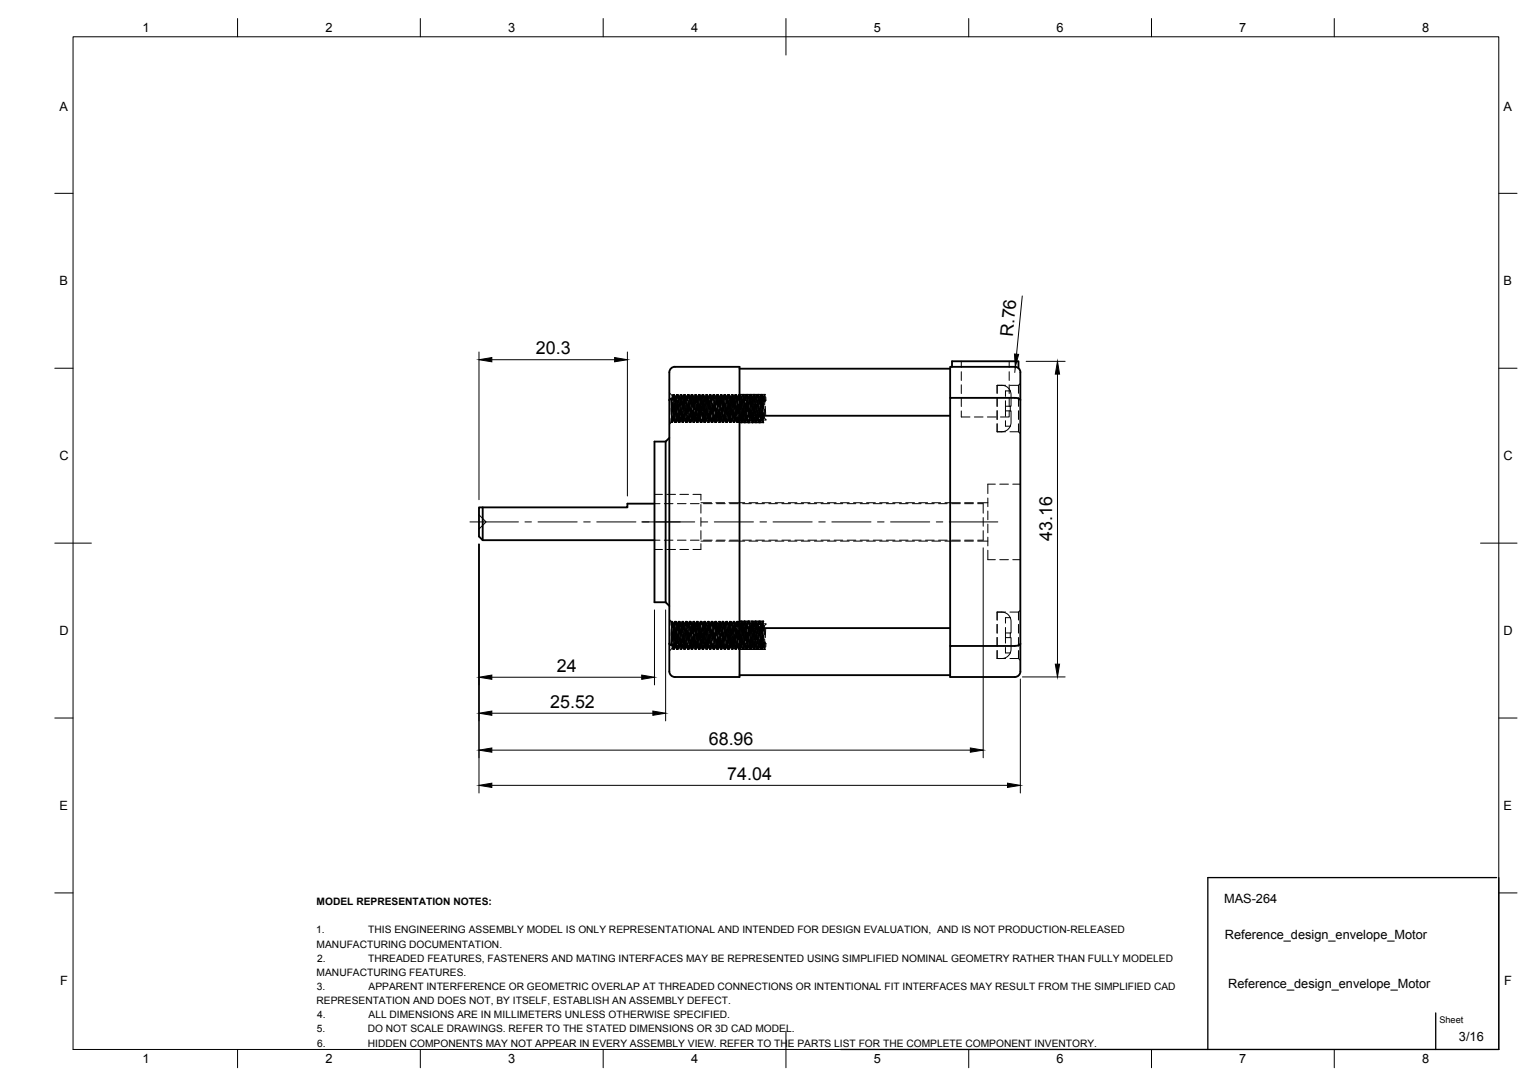
ISO-10303-21;
HEADER;
/* Generated by software containing ST-Developer
 * from STEP Tools, Inc. (www.steptools.com) 
 */

FILE_DESCRIPTION(
/* description */ (''),
/* implementation_level */ '2;1');

FILE_NAME(
/* name */ 'Reference_design_envelope_Motor.step',
/* time_stamp */ '2026-10-12T15:37:13-07:00',
/* author */ (''),
/* organization */ (''),
/* preprocessor_version */ 'ST-DEVELOPER v20.2',
/* originating_system */ 'Autodesk Translation Framework v15.15.0.0',
/* authorisation */ '');

FILE_SCHEMA (('AUTOMOTIVE_DESIGN { 1 0 10303 214 3 1 1 }'));
ENDSEC;

DATA;
#10=MECHANICAL_DESIGN_GEOMETRIC_PRESENTATION_REPRESENTATION('',(#326,#327,#328,#329,#330,#331,#332,#333),#36460);
#106=SHAPE_REPRESENTATION_RELATIONSHIP('SRR','None',#36517,#119);
#119=ADVANCED_BREP_SHAPE_REPRESENTATION('',(#358,#359,#360,#361,#362,#363,
#364,#365),#36446);
#132=FACE_BOUND('',#1845,.T.);
#133=FACE_BOUND('',#1846,.T.);
#134=FACE_BOUND('',#1847,.T.);
#135=FACE_BOUND('',#1848,.T.);
#136=FACE_BOUND('',#1849,.T.);
#137=FACE_BOUND('',#1863,.T.);
#138=FACE_BOUND('',#1865,.T.);
#139=FACE_BOUND('',#1883,.T.);
#140=FACE_BOUND('',#1884,.T.);
#141=FACE_BOUND('',#1885,.T.);
#142=FACE_BOUND('',#1886,.T.);
#143=FACE_BOUND('',#1887,.T.);
#144=FACE_BOUND('',#1893,.T.);
#145=FACE_BOUND('',#1917,.T.);
#146=FACE_BOUND('',#1920,.T.);
#147=FACE_BOUND('',#1921,.T.);
#148=FACE_BOUND('',#1922,.T.);
#149=FACE_BOUND('',#1923,.T.);
#150=FACE_BOUND('',#1924,.T.);
#151=FACE_BOUND('',#1945,.T.);
#152=FACE_BOUND('',#1947,.T.);
#153=FACE_BOUND('',#1954,.T.);
#154=FACE_BOUND('',#1956,.T.);
#155=FACE_BOUND('',#1957,.T.);
#156=FACE_BOUND('',#1958,.T.);
#157=FACE_BOUND('',#1959,.T.);
#158=FACE_BOUND('',#1960,.T.);
#265=(
BOUNDED_CURVE()
B_SPLINE_CURVE(2,(#24742,#24743,#24744,#24745,#24746,#24747,#24748,#24749,
#24750,#24751,#24752,#24753,#24754,#24755,#24756,#24757,#24758,#24759,#24760,
#24761,#24762,#24763,#24764,#24765,#24766,#24767,#24768,#24769,#24770,#24771,
#24772,#24773,#24774,#24775,#24776,#24777,#24778,#24779,#24780,#24781,#24782,
#24783,#24784,#24785,#24786,#24787,#24788,#24789,#24790,#24791,#24792,#24793,
#24794,#24795,#24796,#24797,#24798,#24799,#24800,#24801,#24802,#24803,#24804,
#24805,#24806,#24807,#24808,#24809,#24810,#24811,#24812,#24813,#24814,#24815,
#24816,#24817,#24818,#24819,#24820,#24821,#24822,#24823,#24824,#24825,#24826,
#24827,#24828,#24829,#24830,#24831,#24832,#24833,#24834,#24835,#24836,#24837,
#24838,#24839,#24840,#24841,#24842,#24843,#24844,#24845,#24846,#24847,#24848,
#24849,#24850,#24851,#24852,#24853,#24854,#24855,#24856,#24857,#24858,#24859,
#24860,#24861,#24862,#24863,#24864,#24865,#24866,#24867,#24868,#24869,#24870,
#24871,#24872,#24873,#24874,#24875,#24876,#24877,#24878,#24879,#24880,#24881,
#24882,#24883,#24884,#24885,#24886,#24887,#24888,#24889,#24890,#24891,#24892,
#24893,#24894,#24895,#24896,#24897,#24898,#24899,#24900,#24901,#24902,#24903,
#24904,#24905,#24906,#24907,#24908,#24909,#24910,#24911,#24912,#24913,#24914,
#24915,#24916,#24917,#24918,#24919,#24920,#24921,#24922,#24923,#24924,#24925,
#24926,#24927,#24928,#24929,#24930,#24931,#24932,#24933,#24934,#24935,#24936,
#24937,#24938,#24939,#24940,#24941,#24942,#24943,#24944,#24945,#24946,#24947,
#24948,#24949,#24950,#24951,#24952,#24953,#24954,#24955,#24956,#24957,#24958,
#24959,#24960,#24961,#24962,#24963,#24964,#24965,#24966,#24967,#24968,#24969,
#24970,#24971,#24972,#24973,#24974,#24975,#24976,#24977,#24978,#24979,#24980,
#24981,#24982,#24983,#24984,#24985,#24986,#24987,#24988,#24989,#24990,#24991,
#24992,#24993,#24994,#24995,#24996,#24997,#24998,#24999,#25000,#25001,#25002,
#25003,#25004,#25005,#25006,#25007,#25008,#25009,#25010,#25011,#25012,#25013,
#25014,#25015,#25016,#25017,#25018,#25019,#25020,#25021,#25022,#25023,#25024,
#25025,#25026,#25027,#25028,#25029,#25030,#25031,#25032,#25033,#25034,#25035,
#25036,#25037,#25038,#25039,#25040,#25041,#25042),.UNSPECIFIED.,.F.,.F.)
B_SPLINE_CURVE_WITH_KNOTS((3,2,2,2,2,2,2,2,2,2,2,2,2,2,2,2,2,2,2,2,2,2,
2,2,2,2,2,2,2,2,2,2,2,2,2,2,2,2,2,2,2,2,2,2,2,2,2,2,2,2,2,2,2,2,2,2,2,2,
2,2,2,2,2,2,2,2,2,2,2,2,2,2,2,2,2,2,2,2,2,2,2,2,2,2,2,2,2,2,2,2,2,2,2,2,
2,2,2,2,2,2,2,2,2,2,2,2,2,2,2,2,2,2,2,2,2,2,2,2,2,2,2,2,2,2,2,2,2,2,2,2,
2,2,2,2,2,2,2,2,2,2,2,2,2,2,2,2,2,2,2,2,3),(0.0578262804341777,0.063130434027066,
0.0694434774297724,0.0757565208324788,0.0820695642351851,0.0883826076378915,
0.0946956510405978,0.101008694443304,0.107321737846011,0.113634781248717,
0.119947824651423,0.12626086805413,0.132573911456836,0.138886954859542,
0.145199998262249,0.151513041664955,0.157826085067661,0.164139128470368,
0.170452171873074,0.17676521527578,0.183078258678487,0.189391302081193,
0.195704345483899,0.202017388886606,0.208330432289312,0.214643475692019,
0.220956519094725,0.227269562497431,0.233582605900138,0.239895649302844,
0.24620869270555,0.252521736108257,0.258834779510963,0.265147822913669,
0.271460866316376,0.277773909719082,0.284086953121788,0.290399996524495,
0.296713039927201,0.303026083329907,0.309339126732614,0.31565217013532,
0.321965213538027,0.328278256940733,0.334591300343439,0.340904343746146,
0.347217387148852,0.353530430551558,0.359843473954265,0.366156517356971,
0.372469560759677,0.378782604162384,0.38509564756509,0.391408690967797,
0.397721734370503,0.404034777773209,0.410347821175916,0.416660864578622,
0.422973907981328,0.429286951384035,0.435599994786741,0.441913038189447,
0.448226081592154,0.45453912499486,0.460852168397566,0.467165211800273,
0.473478255202979,0.479791298605685,0.486104342008392,0.492417385411098,
0.498730428813805,0.505043472216511,0.511356515619217,0.517669559021924,
0.52398260242463,0.530295645827336,0.536608689230043,0.542921732632749,
0.549234776035455,0.555547819438162,0.561860862840868,0.568173906243575,
0.574486949646281,0.580799993048987,0.587113036451693,0.5934260798544,0.599739123257106,
0.606052166659813,0.612365210062519,0.618678253465225,0.624991296867932,
0.631304340270638,0.637617383673344,0.643930427076051,0.650243470478757,
0.656556513881463,0.66286955728417,0.669182600686876,0.675495644089582,
0.681808687492289,0.688121730894995,0.694434774297702,0.700747817700408,
0.707060861103114,0.71337390450582,0.719686947908527,0.725999991311233,
0.732313034713939,0.738626078116646,0.744939121519352,0.751252164922059,
0.757565208324765,0.763878251727471,0.770191295130178,0.776504338532884,
0.78281738193559,0.789130425338297,0.795443468741003,0.80175651214371,0.808069555546416,
0.814382598949122,0.820695642351829,0.827008685754535,0.833321729157241,
0.839634772559948,0.845947815962654,0.85226085936536,0.858573902768067,
0.864886946170773,0.871199989573479,0.877513032976186,0.883826076378892,
0.890139119781598,0.896452163184305,0.902765206587011,0.909078249989718,
0.915391293392424,0.92170433679513,0.928017380197837,0.934330423600543,
0.940643467003249,0.946956510405956,0.953269553808662,0.959582597211368,
0.965895640614075,0.972208684016781,0.978521727419488,0.984834770822194,
0.9911478142249,0.997460857627607,1.),.UNSPECIFIED.)
CURVE()
GEOMETRIC_REPRESENTATION_ITEM()
RATIONAL_B_SPLINE_CURVE((0.964022189566827,0.887435933741894,1.,0.866025403784439,
1.,0.866025403784439,1.,0.866025403784439,1.,0.866025403784439,1.,0.866025403784439,
1.,0.866025403784439,1.,0.866025403784439,1.,0.866025403784439,1.,0.866025403784439,
1.,0.866025403784439,1.,0.866025403784439,1.,0.866025403784439,1.,0.866025403784439,
1.,0.866025403784439,1.,0.866025403784439,1.,0.866025403784439,1.,0.866025403784439,
1.,0.866025403784439,1.,0.866025403784439,1.,0.866025403784439,1.,0.866025403784439,
1.,0.866025403784439,1.,0.866025403784439,1.,0.866025403784439,1.,0.866025403784439,
1.,0.866025403784439,1.,0.866025403784439,1.,0.866025403784439,1.,0.866025403784439,
1.,0.866025403784439,1.,0.866025403784439,1.,0.866025403784439,1.,0.866025403784439,
1.,0.866025403784439,1.,0.866025403784439,1.,0.866025403784439,1.,0.866025403784439,
1.,0.866025403784439,1.,0.866025403784439,1.,0.866025403784439,1.,0.866025403784439,
1.,0.866025403784439,1.,0.866025403784439,1.,0.866025403784439,1.,0.866025403784439,
1.,0.866025403784439,1.,0.866025403784439,1.,0.866025403784439,1.,0.866025403784439,
1.,0.866025403784439,1.,0.866025403784439,1.,0.866025403784439,1.,0.866025403784439,
1.,0.866025403784439,1.,0.866025403784439,1.,0.866025403784439,1.,0.866025403784439,
1.,0.866025403784439,1.,0.866025403784439,1.,0.866025403784439,1.,0.866025403784439,
1.,0.866025403784439,1.,0.866025403784439,1.,0.866025403784439,1.,0.866025403784439,
1.,0.866025403784439,1.,0.866025403784439,1.,0.866025403784439,1.,0.866025403784439,
1.,0.866025403784439,1.,0.866025403784439,1.,0.866025403784439,1.,0.866025403784439,
1.,0.866025403784439,1.,0.866025403784439,1.,0.866025403784439,1.,0.866025403784439,
1.,0.866025403784439,1.,0.866025403784439,1.,0.866025403784439,1.,0.866025403784439,
1.,0.866025403784439,1.,0.866025403784439,1.,0.866025403784439,1.,0.866025403784439,
1.,0.866025403784439,1.,0.866025403784439,1.,0.866025403784439,1.,0.866025403784439,
1.,0.866025403784439,1.,0.866025403784439,1.,0.866025403784439,1.,0.866025403784439,
1.,0.866025403784439,1.,0.866025403784439,1.,0.866025403784439,1.,0.866025403784439,
1.,0.866025403784439,1.,0.866025403784439,1.,0.866025403784439,1.,0.866025403784439,
1.,0.866025403784439,1.,0.866025403784439,1.,0.866025403784439,1.,0.866025403784439,
1.,0.866025403784439,1.,0.866025403784439,1.,0.866025403784439,1.,0.866025403784439,
1.,0.866025403784439,1.,0.866025403784439,1.,0.866025403784439,1.,0.866025403784439,
1.,0.866025403784439,1.,0.866025403784439,1.,0.866025403784439,1.,0.866025403784439,
1.,0.866025403784439,1.,0.866025403784439,1.,0.866025403784439,1.,0.866025403784439,
1.,0.866025403784439,1.,0.866025403784439,1.,0.866025403784439,1.,0.866025403784439,
1.,0.866025403784439,1.,0.866025403784439,1.,0.866025403784439,1.,0.866025403784439,
1.,0.866025403784439,1.,0.866025403784439,1.,0.866025403784439,1.,0.866025403784439,
1.,0.866025403784439,1.,0.866025403784439,1.,0.866025403784439,1.,0.866025403784439,
1.,0.866025403784439,1.,0.866025403784439,1.,0.866025403784439,1.,0.866025403784439,
1.,0.866025403784439,1.,0.866025403784439,1.,0.866025403784439,1.,0.866025403784439,
1.,0.866025403784439,1.,0.866025403784439,1.,0.866025403784439,1.,0.946114646712328,
0.93557529156098))
REPRESENTATION_ITEM('')
);
#266=(
BOUNDED_CURVE()
B_SPLINE_CURVE(2,(#25685,#25686,#25687,#25688,#25689,#25690,#25691,#25692,
#25693,#25694,#25695,#25696,#25697,#25698,#25699,#25700,#25701,#25702,#25703,
#25704,#25705,#25706,#25707,#25708,#25709,#25710,#25711,#25712,#25713,#25714,
#25715,#25716,#25717,#25718,#25719,#25720,#25721,#25722,#25723,#25724,#25725,
#25726,#25727,#25728,#25729,#25730,#25731,#25732,#25733,#25734,#25735,#25736,
#25737,#25738,#25739,#25740,#25741,#25742,#25743,#25744,#25745,#25746,#25747,
#25748,#25749,#25750,#25751,#25752,#25753,#25754,#25755,#25756,#25757,#25758,
#25759,#25760,#25761,#25762,#25763,#25764,#25765,#25766,#25767,#25768,#25769,
#25770,#25771,#25772,#25773,#25774,#25775,#25776,#25777,#25778,#25779,#25780,
#25781,#25782,#25783,#25784,#25785,#25786,#25787,#25788,#25789,#25790,#25791,
#25792,#25793,#25794,#25795,#25796,#25797,#25798,#25799,#25800,#25801,#25802,
#25803,#25804,#25805,#25806,#25807,#25808,#25809,#25810,#25811,#25812,#25813,
#25814,#25815,#25816,#25817,#25818,#25819,#25820,#25821,#25822,#25823,#25824,
#25825,#25826,#25827,#25828,#25829,#25830,#25831,#25832,#25833,#25834,#25835,
#25836,#25837,#25838,#25839,#25840,#25841,#25842,#25843,#25844,#25845,#25846,
#25847,#25848,#25849,#25850,#25851,#25852,#25853,#25854,#25855,#25856,#25857,
#25858,#25859,#25860,#25861,#25862,#25863,#25864,#25865,#25866,#25867,#25868,
#25869,#25870,#25871,#25872,#25873,#25874,#25875,#25876,#25877,#25878,#25879,
#25880,#25881,#25882,#25883,#25884,#25885,#25886,#25887,#25888,#25889,#25890,
#25891,#25892,#25893,#25894,#25895,#25896,#25897,#25898,#25899,#25900,#25901,
#25902,#25903,#25904,#25905,#25906,#25907,#25908,#25909,#25910,#25911,#25912,
#25913,#25914,#25915,#25916,#25917,#25918,#25919,#25920,#25921,#25922,#25923,
#25924,#25925,#25926,#25927,#25928,#25929,#25930,#25931,#25932,#25933,#25934,
#25935,#25936,#25937,#25938,#25939,#25940,#25941,#25942,#25943,#25944,#25945,
#25946,#25947,#25948,#25949,#25950,#25951,#25952,#25953,#25954,#25955,#25956,
#25957,#25958,#25959,#25960,#25961,#25962,#25963,#25964,#25965,#25966,#25967,
#25968,#25969,#25970,#25971,#25972,#25973,#25974,#25975,#25976,#25977,#25978,
#25979,#25980,#25981,#25982,#25983,#25984,#25985),.UNSPECIFIED.,.F.,.F.)
B_SPLINE_CURVE_WITH_KNOTS((3,2,2,2,2,2,2,2,2,2,2,2,2,2,2,2,2,2,2,2,2,2,
2,2,2,2,2,2,2,2,2,2,2,2,2,2,2,2,2,2,2,2,2,2,2,2,2,2,2,2,2,2,2,2,2,2,2,2,
2,2,2,2,2,2,2,2,2,2,2,2,2,2,2,2,2,2,2,2,2,2,2,2,2,2,2,2,2,2,2,2,2,2,2,2,
2,2,2,2,2,2,2,2,2,2,2,2,2,2,2,2,2,2,2,2,2,2,2,2,2,2,2,2,2,2,2,2,2,2,2,2,
2,2,2,2,2,2,2,2,2,2,2,2,2,2,2,2,2,2,2,2,3),(0.0624132680173737,0.063130431687086,
0.0694434748554471,0.0757565180238082,0.0820695611921693,0.0883826043605304,
0.0946956475288915,0.101008690697253,0.107321733865614,0.113634777033975,
0.119947820202336,0.126260863370697,0.132573906539058,0.138886949707419,
0.14519999287578,0.151513036044142,0.157826079212503,0.164139122380864,
0.170452165549225,0.176765208717586,0.183078251885947,0.189391295054308,
0.195704338222669,0.20201738139103,0.208330424559392,0.214643467727753,
0.220956510896114,0.227269554064475,0.233582597232836,0.239895640401197,
0.246208683569558,0.252521726737919,0.258834769906281,0.265147813074642,
0.271460856243003,0.277773899411364,0.284086942579725,0.290399985748086,
0.296713028916447,0.303026072084808,0.309339115253169,0.31565215842153,
0.321965201589892,0.328278244758253,0.334591287926614,0.340904331094975,
0.347217374263336,0.353530417431697,0.359843460600058,0.366156503768419,
0.37246954693678,0.378782590105142,0.385095633273503,0.391408676441864,
0.397721719610225,0.404034762778586,0.410347805946947,0.416660849115308,
0.422973892283669,0.42928693545203,0.435599978620392,0.441913021788753,
0.448226064957114,0.454539108125475,0.460852151293836,0.467165194462197,
0.473478237630558,0.479791280798919,0.48610432396728,0.492417367135642,
0.498730410304003,0.505043453472364,0.511356496640725,0.517669539809086,
0.523982582977447,0.530295626145808,0.536608669314169,0.542921712482531,
0.549234755650892,0.555547798819253,0.561860841987614,0.568173885155975,
0.574486928324336,0.580799971492697,0.587113014661058,0.593426057829419,
0.599739100997781,0.606052144166142,0.612365187334503,0.618678230502864,
0.624991273671225,0.631304316839586,0.637617360007947,0.643930403176308,
0.650243446344669,0.656556489513031,0.662869532681392,0.669182575849753,
0.675495619018114,0.681808662186475,0.688121705354836,0.694434748523197,
0.700747791691558,0.707060834859919,0.713373878028281,0.719686921196642,
0.725999964365003,0.732313007533364,0.738626050701725,0.744939093870086,
0.751252137038447,0.757565180206808,0.763878223375169,0.770191266543531,
0.776504309711892,0.782817352880253,0.789130396048614,0.795443439216975,
0.801756482385336,0.808069525553697,0.814382568722058,0.820695611890419,
0.827008655058781,0.833321698227142,0.839634741395503,0.845947784563864,
0.852260827732225,0.858573870900586,0.864886914068947,0.871199957237308,
0.87751300040567,0.88382604357403,0.890139086742392,0.896452129910753,0.902765173079114,
0.909078216247475,0.915391259415836,0.921704302584197,0.928017345752558,
0.934330388920919,0.940643432089281,0.946956475257642,0.953269518426003,
0.959582561594364,0.965895604762725,0.972208647931086,0.978521691099447,
0.984834734267808,0.99114777743617,0.997460820604531,1.),.UNSPECIFIED.)
CURVE()
GEOMETRIC_REPRESENTATION_ITEM()
RATIONAL_B_SPLINE_CURVE((0.973018780871376,0.984780444152242,1.,0.866025403784439,
1.,0.866025403784439,1.,0.866025403784439,1.,0.866025403784439,1.,0.866025403784439,
1.,0.866025403784439,1.,0.866025403784439,1.,0.866025403784439,1.,0.866025403784439,
1.,0.866025403784439,1.,0.866025403784439,1.,0.866025403784439,1.,0.866025403784439,
1.,0.866025403784439,1.,0.866025403784439,1.,0.866025403784439,1.,0.866025403784439,
1.,0.866025403784439,1.,0.866025403784439,1.,0.866025403784439,1.,0.866025403784439,
1.,0.866025403784439,1.,0.866025403784439,1.,0.866025403784439,1.,0.866025403784439,
1.,0.866025403784439,1.,0.866025403784439,1.,0.866025403784439,1.,0.866025403784439,
1.,0.866025403784439,1.,0.866025403784439,1.,0.866025403784439,1.,0.866025403784439,
1.,0.866025403784439,1.,0.866025403784439,1.,0.866025403784439,1.,0.866025403784439,
1.,0.866025403784439,1.,0.866025403784439,1.,0.866025403784439,1.,0.866025403784439,
1.,0.866025403784439,1.,0.866025403784439,1.,0.866025403784439,1.,0.866025403784439,
1.,0.866025403784439,1.,0.866025403784439,1.,0.866025403784439,1.,0.866025403784439,
1.,0.866025403784439,1.,0.866025403784439,1.,0.866025403784439,1.,0.866025403784439,
1.,0.866025403784439,1.,0.866025403784439,1.,0.866025403784439,1.,0.866025403784439,
1.,0.866025403784439,1.,0.866025403784439,1.,0.866025403784439,1.,0.866025403784439,
1.,0.866025403784439,1.,0.866025403784439,1.,0.866025403784439,1.,0.866025403784439,
1.,0.866025403784439,1.,0.866025403784439,1.,0.866025403784439,1.,0.866025403784439,
1.,0.866025403784439,1.,0.866025403784439,1.,0.866025403784439,1.,0.866025403784439,
1.,0.866025403784439,1.,0.866025403784439,1.,0.866025403784439,1.,0.866025403784439,
1.,0.866025403784439,1.,0.866025403784439,1.,0.866025403784439,1.,0.866025403784439,
1.,0.866025403784439,1.,0.866025403784439,1.,0.866025403784439,1.,0.866025403784439,
1.,0.866025403784439,1.,0.866025403784439,1.,0.866025403784439,1.,0.866025403784439,
1.,0.866025403784439,1.,0.866025403784439,1.,0.866025403784439,1.,0.866025403784439,
1.,0.866025403784439,1.,0.866025403784439,1.,0.866025403784439,1.,0.866025403784439,
1.,0.866025403784439,1.,0.866025403784439,1.,0.866025403784439,1.,0.866025403784439,
1.,0.866025403784439,1.,0.866025403784439,1.,0.866025403784439,1.,0.866025403784439,
1.,0.866025403784439,1.,0.866025403784439,1.,0.866025403784439,1.,0.866025403784439,
1.,0.866025403784439,1.,0.866025403784439,1.,0.866025403784439,1.,0.866025403784439,
1.,0.866025403784439,1.,0.866025403784439,1.,0.866025403784439,1.,0.866025403784439,
1.,0.866025403784439,1.,0.866025403784439,1.,0.866025403784439,1.,0.866025403784439,
1.,0.866025403784439,1.,0.866025403784439,1.,0.866025403784439,1.,0.866025403784439,
1.,0.866025403784439,1.,0.866025403784439,1.,0.866025403784439,1.,0.866025403784439,
1.,0.866025403784439,1.,0.866025403784439,1.,0.866025403784439,1.,0.866025403784439,
1.,0.866025403784439,1.,0.866025403784439,1.,0.866025403784439,1.,0.866025403784439,
1.,0.866025403784439,1.,0.866025403784439,1.,0.866025403784439,1.,0.866025403784439,
1.,0.866025403784439,1.,0.866025403784439,1.,0.866025403784439,1.,0.866025403784439,
1.,0.866025403784439,1.,0.866025403784439,1.,0.866025403784439,1.,0.946114646713198,
0.93557529156132))
REPRESENTATION_ITEM('')
);
#267=(
BOUNDED_CURVE()
B_SPLINE_CURVE(2,(#27292,#27293,#27294,#27295,#27296,#27297,#27298,#27299,
#27300,#27301,#27302,#27303,#27304,#27305,#27306,#27307,#27308,#27309,#27310,
#27311,#27312,#27313,#27314,#27315,#27316,#27317,#27318,#27319,#27320,#27321,
#27322,#27323,#27324,#27325,#27326,#27327,#27328,#27329,#27330,#27331,#27332,
#27333,#27334,#27335,#27336,#27337,#27338,#27339,#27340,#27341,#27342,#27343,
#27344,#27345,#27346,#27347,#27348,#27349,#27350,#27351,#27352,#27353,#27354,
#27355,#27356,#27357,#27358,#27359,#27360,#27361,#27362,#27363,#27364,#27365,
#27366,#27367,#27368,#27369,#27370,#27371,#27372,#27373,#27374,#27375,#27376,
#27377,#27378,#27379,#27380,#27381,#27382,#27383,#27384,#27385,#27386,#27387,
#27388,#27389,#27390,#27391,#27392,#27393,#27394,#27395,#27396,#27397,#27398,
#27399,#27400,#27401,#27402,#27403,#27404,#27405,#27406,#27407,#27408,#27409,
#27410,#27411,#27412,#27413,#27414,#27415,#27416,#27417,#27418,#27419,#27420,
#27421,#27422,#27423,#27424,#27425,#27426,#27427,#27428,#27429,#27430,#27431,
#27432,#27433,#27434,#27435,#27436,#27437,#27438,#27439,#27440,#27441,#27442,
#27443,#27444,#27445,#27446,#27447,#27448,#27449,#27450,#27451,#27452,#27453,
#27454,#27455,#27456,#27457,#27458,#27459,#27460,#27461,#27462,#27463,#27464,
#27465,#27466,#27467,#27468,#27469,#27470,#27471,#27472,#27473,#27474,#27475,
#27476,#27477,#27478,#27479,#27480,#27481,#27482,#27483,#27484,#27485,#27486,
#27487,#27488,#27489,#27490,#27491,#27492,#27493,#27494,#27495,#27496,#27497,
#27498,#27499,#27500,#27501,#27502,#27503,#27504,#27505,#27506,#27507,#27508,
#27509,#27510,#27511,#27512,#27513,#27514,#27515,#27516,#27517,#27518,#27519,
#27520,#27521,#27522,#27523,#27524,#27525,#27526,#27527,#27528,#27529,#27530,
#27531,#27532,#27533,#27534,#27535,#27536,#27537,#27538,#27539,#27540,#27541,
#27542,#27543,#27544,#27545,#27546,#27547,#27548,#27549,#27550,#27551,#27552,
#27553,#27554,#27555,#27556,#27557,#27558,#27559,#27560,#27561,#27562,#27563,
#27564,#27565,#27566,#27567,#27568,#27569,#27570,#27571,#27572,#27573,#27574,
#27575,#27576,#27577,#27578,#27579,#27580,#27581,#27582,#27583,#27584,#27585,
#27586,#27587,#27588,#27589,#27590,#27591,#27592),.UNSPECIFIED.,.F.,.F.)
B_SPLINE_CURVE_WITH_KNOTS((3,2,2,2,2,2,2,2,2,2,2,2,2,2,2,2,2,2,2,2,2,2,
2,2,2,2,2,2,2,2,2,2,2,2,2,2,2,2,2,2,2,2,2,2,2,2,2,2,2,2,2,2,2,2,2,2,2,2,
2,2,2,2,2,2,2,2,2,2,2,2,2,2,2,2,2,2,2,2,2,2,2,2,2,2,2,2,2,2,2,2,2,2,2,2,
2,2,2,2,2,2,2,2,2,2,2,2,2,2,2,2,2,2,2,2,2,2,2,2,2,2,2,2,2,2,2,2,2,2,2,2,
2,2,2,2,2,2,2,2,2,2,2,2,2,2,2,2,2,2,2,2,3),(0.0578262804341777,0.0631304340270661,
0.0694434774297724,0.0757565208324788,0.0820695642351851,0.0883826076378915,
0.0946956510405978,0.101008694443304,0.107321737846011,0.113634781248717,
0.119947824651423,0.12626086805413,0.132573911456836,0.138886954859542,
0.145199998262249,0.151513041664955,0.157826085067661,0.164139128470368,
0.170452171873074,0.17676521527578,0.183078258678487,0.189391302081193,
0.195704345483899,0.202017388886606,0.208330432289312,0.214643475692019,
0.220956519094725,0.227269562497431,0.233582605900138,0.239895649302844,
0.24620869270555,0.252521736108257,0.258834779510963,0.265147822913669,
0.271460866316376,0.277773909719082,0.284086953121788,0.290399996524495,
0.296713039927201,0.303026083329908,0.309339126732614,0.31565217013532,
0.321965213538027,0.328278256940733,0.334591300343439,0.340904343746146,
0.347217387148852,0.353530430551558,0.359843473954265,0.366156517356971,
0.372469560759677,0.378782604162384,0.38509564756509,0.391408690967797,
0.397721734370503,0.404034777773209,0.410347821175916,0.416660864578622,
0.422973907981328,0.429286951384035,0.435599994786741,0.441913038189447,
0.448226081592154,0.45453912499486,0.460852168397566,0.467165211800273,
0.473478255202979,0.479791298605685,0.486104342008392,0.492417385411098,
0.498730428813805,0.505043472216511,0.511356515619217,0.517669559021924,
0.52398260242463,0.530295645827336,0.536608689230043,0.542921732632749,
0.549234776035455,0.555547819438162,0.561860862840868,0.568173906243575,
0.574486949646281,0.580799993048987,0.587113036451693,0.5934260798544,0.599739123257106,
0.606052166659813,0.612365210062519,0.618678253465225,0.624991296867932,
0.631304340270638,0.637617383673344,0.643930427076051,0.650243470478757,
0.656556513881463,0.66286955728417,0.669182600686876,0.675495644089582,
0.681808687492289,0.688121730894995,0.694434774297702,0.700747817700408,
0.707060861103114,0.71337390450582,0.719686947908527,0.725999991311233,
0.732313034713939,0.738626078116646,0.744939121519352,0.751252164922059,
0.757565208324765,0.763878251727471,0.770191295130178,0.776504338532884,
0.78281738193559,0.789130425338297,0.795443468741003,0.80175651214371,0.808069555546416,
0.814382598949122,0.820695642351829,0.827008685754535,0.833321729157241,
0.839634772559948,0.845947815962654,0.85226085936536,0.858573902768067,
0.864886946170773,0.871199989573479,0.877513032976186,0.883826076378892,
0.890139119781598,0.896452163184305,0.902765206587011,0.909078249989718,
0.915391293392424,0.92170433679513,0.928017380197837,0.934330423600543,
0.940643467003249,0.946956510405956,0.953269553808662,0.959582597211368,
0.965895640614075,0.972208684016781,0.978521727419488,0.984834770822194,
0.9911478142249,0.997460857627607,1.),.UNSPECIFIED.)
CURVE()
GEOMETRIC_REPRESENTATION_ITEM()
RATIONAL_B_SPLINE_CURVE((0.964022189566827,0.887435933741894,1.,0.866025403784439,
1.,0.866025403784439,1.,0.866025403784439,1.,0.866025403784439,1.,0.866025403784439,
1.,0.866025403784439,1.,0.866025403784439,1.,0.866025403784439,1.,0.866025403784439,
1.,0.866025403784439,1.,0.866025403784439,1.,0.866025403784439,1.,0.866025403784439,
1.,0.866025403784439,1.,0.866025403784439,1.,0.866025403784439,1.,0.866025403784439,
1.,0.866025403784439,1.,0.866025403784439,1.,0.866025403784439,1.,0.866025403784439,
1.,0.866025403784439,1.,0.866025403784439,1.,0.866025403784439,1.,0.866025403784439,
1.,0.866025403784439,1.,0.866025403784439,1.,0.866025403784439,1.,0.866025403784439,
1.,0.866025403784439,1.,0.866025403784439,1.,0.866025403784439,1.,0.866025403784439,
1.,0.866025403784439,1.,0.866025403784439,1.,0.866025403784439,1.,0.866025403784439,
1.,0.866025403784439,1.,0.866025403784439,1.,0.866025403784439,1.,0.866025403784439,
1.,0.866025403784439,1.,0.866025403784439,1.,0.866025403784439,1.,0.866025403784439,
1.,0.866025403784439,1.,0.866025403784439,1.,0.866025403784439,1.,0.866025403784439,
1.,0.866025403784439,1.,0.866025403784439,1.,0.866025403784439,1.,0.866025403784439,
1.,0.866025403784439,1.,0.866025403784439,1.,0.866025403784439,1.,0.866025403784439,
1.,0.866025403784439,1.,0.866025403784439,1.,0.866025403784439,1.,0.866025403784439,
1.,0.866025403784439,1.,0.866025403784439,1.,0.866025403784439,1.,0.866025403784439,
1.,0.866025403784439,1.,0.866025403784439,1.,0.866025403784439,1.,0.866025403784439,
1.,0.866025403784439,1.,0.866025403784439,1.,0.866025403784439,1.,0.866025403784439,
1.,0.866025403784439,1.,0.866025403784439,1.,0.866025403784439,1.,0.866025403784439,
1.,0.866025403784439,1.,0.866025403784439,1.,0.866025403784439,1.,0.866025403784439,
1.,0.866025403784439,1.,0.866025403784439,1.,0.866025403784439,1.,0.866025403784439,
1.,0.866025403784439,1.,0.866025403784439,1.,0.866025403784439,1.,0.866025403784439,
1.,0.866025403784439,1.,0.866025403784439,1.,0.866025403784439,1.,0.866025403784439,
1.,0.866025403784439,1.,0.866025403784439,1.,0.866025403784439,1.,0.866025403784439,
1.,0.866025403784439,1.,0.866025403784439,1.,0.866025403784439,1.,0.866025403784439,
1.,0.866025403784439,1.,0.866025403784439,1.,0.866025403784439,1.,0.866025403784439,
1.,0.866025403784439,1.,0.866025403784439,1.,0.866025403784439,1.,0.866025403784439,
1.,0.866025403784439,1.,0.866025403784439,1.,0.866025403784439,1.,0.866025403784439,
1.,0.866025403784439,1.,0.866025403784439,1.,0.866025403784439,1.,0.866025403784439,
1.,0.866025403784439,1.,0.866025403784439,1.,0.866025403784439,1.,0.866025403784439,
1.,0.866025403784439,1.,0.866025403784439,1.,0.866025403784439,1.,0.866025403784439,
1.,0.866025403784439,1.,0.866025403784439,1.,0.866025403784439,1.,0.866025403784439,
1.,0.866025403784439,1.,0.866025403784439,1.,0.866025403784439,1.,0.866025403784439,
1.,0.866025403784439,1.,0.866025403784439,1.,0.866025403784439,1.,0.866025403784439,
1.,0.866025403784439,1.,0.866025403784439,1.,0.866025403784439,1.,0.866025403784439,
1.,0.866025403784439,1.,0.866025403784439,1.,0.866025403784439,1.,0.866025403784439,
1.,0.866025403784439,1.,0.866025403784439,1.,0.866025403784439,1.,0.946114646712328,
0.93557529156098))
REPRESENTATION_ITEM('')
);
#268=(
BOUNDED_CURVE()
B_SPLINE_CURVE(2,(#28234,#28235,#28236,#28237,#28238,#28239,#28240,#28241,
#28242,#28243,#28244,#28245,#28246,#28247,#28248,#28249,#28250,#28251,#28252,
#28253,#28254,#28255,#28256,#28257,#28258,#28259,#28260,#28261,#28262,#28263,
#28264,#28265,#28266,#28267,#28268,#28269,#28270,#28271,#28272,#28273,#28274,
#28275,#28276,#28277,#28278,#28279,#28280,#28281,#28282,#28283,#28284,#28285,
#28286,#28287,#28288,#28289,#28290,#28291,#28292,#28293,#28294,#28295,#28296,
#28297,#28298,#28299,#28300,#28301,#28302,#28303,#28304,#28305,#28306,#28307,
#28308,#28309,#28310,#28311,#28312,#28313,#28314,#28315,#28316,#28317,#28318,
#28319,#28320,#28321,#28322,#28323,#28324,#28325,#28326,#28327,#28328,#28329,
#28330,#28331,#28332,#28333,#28334,#28335,#28336,#28337,#28338,#28339,#28340,
#28341,#28342,#28343,#28344,#28345,#28346,#28347,#28348,#28349,#28350,#28351,
#28352,#28353,#28354,#28355,#28356,#28357,#28358,#28359,#28360,#28361,#28362,
#28363,#28364,#28365,#28366,#28367,#28368,#28369,#28370,#28371,#28372,#28373,
#28374,#28375,#28376,#28377,#28378,#28379,#28380,#28381,#28382,#28383,#28384,
#28385,#28386,#28387,#28388,#28389,#28390,#28391,#28392,#28393,#28394,#28395,
#28396,#28397,#28398,#28399,#28400,#28401,#28402,#28403,#28404,#28405,#28406,
#28407,#28408,#28409,#28410,#28411,#28412,#28413,#28414,#28415,#28416,#28417,
#28418,#28419,#28420,#28421,#28422,#28423,#28424,#28425,#28426,#28427,#28428,
#28429,#28430,#28431,#28432,#28433,#28434,#28435,#28436,#28437,#28438,#28439,
#28440,#28441,#28442,#28443,#28444,#28445,#28446,#28447,#28448,#28449,#28450,
#28451,#28452,#28453,#28454,#28455,#28456,#28457,#28458,#28459,#28460,#28461,
#28462,#28463,#28464,#28465,#28466,#28467,#28468,#28469,#28470,#28471,#28472,
#28473,#28474,#28475,#28476,#28477,#28478,#28479,#28480,#28481,#28482,#28483,
#28484,#28485,#28486,#28487,#28488,#28489,#28490,#28491,#28492,#28493,#28494,
#28495,#28496,#28497,#28498,#28499,#28500,#28501,#28502,#28503,#28504,#28505,
#28506,#28507,#28508,#28509,#28510,#28511,#28512,#28513,#28514,#28515,#28516,
#28517,#28518,#28519,#28520,#28521,#28522,#28523,#28524,#28525,#28526,#28527,
#28528,#28529,#28530,#28531,#28532,#28533,#28534),.UNSPECIFIED.,.F.,.F.)
B_SPLINE_CURVE_WITH_KNOTS((3,2,2,2,2,2,2,2,2,2,2,2,2,2,2,2,2,2,2,2,2,2,
2,2,2,2,2,2,2,2,2,2,2,2,2,2,2,2,2,2,2,2,2,2,2,2,2,2,2,2,2,2,2,2,2,2,2,2,
2,2,2,2,2,2,2,2,2,2,2,2,2,2,2,2,2,2,2,2,2,2,2,2,2,2,2,2,2,2,2,2,2,2,2,2,
2,2,2,2,2,2,2,2,2,2,2,2,2,2,2,2,2,2,2,2,2,2,2,2,2,2,2,2,2,2,2,2,2,2,2,2,
2,2,2,2,2,2,2,2,2,2,2,2,2,2,2,2,2,2,2,2,3),(0.0624132680173737,0.0631304316871764,
0.0694434748563336,0.0757565180254908,0.082069561194648,0.0883826043638051,
0.0946956475329623,0.101008690702119,0.107321733871277,0.113634777040434,
0.119947820209591,0.126260863378748,0.132573906547905,0.138886949717063,
0.14519999288622,0.151513036055377,0.157826079224534,0.164139122393691,
0.170452165562848,0.176765208732006,0.183078251901163,0.18939129507032,
0.195704338239477,0.202017381408634,0.208330424577791,0.214643467746949,
0.220956510916106,0.227269554085263,0.23358259725442,0.239895640423577,
0.246208683592735,0.252521726761892,0.258834769931049,0.265147813100206,
0.271460856269363,0.27777389943852,0.284086942607678,0.290399985776835,
0.296713028945992,0.303026072115149,0.309339115284306,0.315652158453464,
0.321965201622621,0.328278244791778,0.334591287960935,0.340904331130092,
0.347217374299249,0.353530417468407,0.359843460637564,0.366156503806721,
0.372469546975878,0.378782590145035,0.385095633314192,0.39140867648335,
0.397721719652507,0.404034762821664,0.410347805990821,0.416660849159978,
0.422973892329136,0.429286935498293,0.43559997866745,0.441913021836607,
0.448226065005764,0.454539108174921,0.460852151344079,0.467165194513236,
0.473478237682393,0.47979128085155,0.486104324020707,0.492417367189865,
0.498730410359022,0.505043453528179,0.511356496697336,0.517669539866493,
0.52398258303565,0.530295626204808,0.536608669373965,0.542921712543122,
0.549234755712279,0.555547798881436,0.561860842050594,0.568173885219751,
0.574486928388908,0.580799971558065,0.587113014727222,0.593426057896379,
0.599739101065537,0.606052144234694,0.612365187403851,0.618678230573008,
0.624991273742165,0.631304316911322,0.63761736008048,0.643930403249637,
0.650243446418794,0.656556489587951,0.662869532757108,0.669182575926266,
0.675495619095423,0.68180866226458,0.688121705433737,0.694434748602894,
0.700747791772051,0.707060834941208,0.713373878110366,0.719686921279523,
0.72599996444868,0.732313007617837,0.738626050786994,0.744939093956152,
0.751252137125309,0.757565180294466,0.763878223463623,0.77019126663278,
0.776504309801938,0.782817352971095,0.789130396140252,0.795443439309409,
0.801756482478566,0.808069525647723,0.814382568816881,0.820695611986038,
0.827008655155195,0.833321698324352,0.839634741493509,0.845947784662667,
0.852260827831824,0.858573871000981,0.864886914170138,0.871199957339295,
0.877513000508452,0.883826043677609,0.890139086846767,0.896452130015924,
0.902765173185081,0.909078216354238,0.915391259523395,0.921704302692553,
0.92801734586171,0.934330389030867,0.940643432200024,0.946956475369181,
0.953269518538338,0.959582561707496,0.965895604876653,0.97220864804581,
0.978521691214967,0.984834734384124,0.991147777553281,0.997460820722439,
1.),.UNSPECIFIED.)
CURVE()
GEOMETRIC_REPRESENTATION_ITEM()
RATIONAL_B_SPLINE_CURVE((0.973018780871375,0.984780444152242,1.,0.866025403784439,
1.,0.866025403784439,1.,0.866025403784439,1.,0.866025403784439,1.,0.866025403784439,
1.,0.866025403784439,1.,0.866025403784439,1.,0.866025403784439,1.,0.866025403784439,
1.,0.866025403784439,1.,0.866025403784439,1.,0.866025403784439,1.,0.866025403784439,
1.,0.866025403784439,1.,0.866025403784439,1.,0.866025403784439,1.,0.866025403784439,
1.,0.866025403784439,1.,0.866025403784439,1.,0.866025403784439,1.,0.866025403784439,
1.,0.866025403784439,1.,0.866025403784439,1.,0.866025403784439,1.,0.866025403784439,
1.,0.866025403784439,1.,0.866025403784439,1.,0.866025403784439,1.,0.866025403784439,
1.,0.866025403784439,1.,0.866025403784439,1.,0.866025403784439,1.,0.866025403784439,
1.,0.866025403784439,1.,0.866025403784439,1.,0.866025403784439,1.,0.866025403784439,
1.,0.866025403784439,1.,0.866025403784439,1.,0.866025403784439,1.,0.866025403784439,
1.,0.866025403784439,1.,0.866025403784439,1.,0.866025403784439,1.,0.866025403784439,
1.,0.866025403784439,1.,0.866025403784439,1.,0.866025403784439,1.,0.866025403784439,
1.,0.866025403784439,1.,0.866025403784439,1.,0.866025403784439,1.,0.866025403784439,
1.,0.866025403784439,1.,0.866025403784439,1.,0.866025403784439,1.,0.866025403784439,
1.,0.866025403784439,1.,0.866025403784439,1.,0.866025403784439,1.,0.866025403784439,
1.,0.866025403784439,1.,0.866025403784439,1.,0.866025403784439,1.,0.866025403784439,
1.,0.866025403784439,1.,0.866025403784439,1.,0.866025403784439,1.,0.866025403784439,
1.,0.866025403784439,1.,0.866025403784439,1.,0.866025403784439,1.,0.866025403784439,
1.,0.866025403784439,1.,0.866025403784439,1.,0.866025403784439,1.,0.866025403784439,
1.,0.866025403784439,1.,0.866025403784439,1.,0.866025403784439,1.,0.866025403784439,
1.,0.866025403784439,1.,0.866025403784439,1.,0.866025403784439,1.,0.866025403784439,
1.,0.866025403784439,1.,0.866025403784439,1.,0.866025403784439,1.,0.866025403784439,
1.,0.866025403784439,1.,0.866025403784439,1.,0.866025403784439,1.,0.866025403784439,
1.,0.866025403784439,1.,0.866025403784439,1.,0.866025403784439,1.,0.866025403784439,
1.,0.866025403784439,1.,0.866025403784439,1.,0.866025403784439,1.,0.866025403784439,
1.,0.866025403784439,1.,0.866025403784439,1.,0.866025403784439,1.,0.866025403784439,
1.,0.866025403784439,1.,0.866025403784439,1.,0.866025403784439,1.,0.866025403784439,
1.,0.866025403784439,1.,0.866025403784439,1.,0.866025403784439,1.,0.866025403784439,
1.,0.866025403784439,1.,0.866025403784439,1.,0.866025403784439,1.,0.866025403784439,
1.,0.866025403784439,1.,0.866025403784439,1.,0.866025403784439,1.,0.866025403784439,
1.,0.866025403784439,1.,0.866025403784439,1.,0.866025403784439,1.,0.866025403784439,
1.,0.866025403784439,1.,0.866025403784439,1.,0.866025403784439,1.,0.866025403784439,
1.,0.866025403784439,1.,0.866025403784439,1.,0.866025403784439,1.,0.866025403784439,
1.,0.866025403784439,1.,0.866025403784439,1.,0.866025403784439,1.,0.866025403784439,
1.,0.866025403784439,1.,0.866025403784439,1.,0.866025403784439,1.,0.866025403784439,
1.,0.866025403784439,1.,0.866025403784439,1.,0.866025403784439,1.,0.866025403784439,
1.,0.866025403784439,1.,0.866025403784439,1.,0.866025403784439,1.,0.946114646713198,
0.93557529156132))
REPRESENTATION_ITEM('')
);
#269=(
BOUNDED_CURVE()
B_SPLINE_CURVE(2,(#29818,#29819,#29820,#29821,#29822,#29823,#29824,#29825,
#29826,#29827,#29828,#29829,#29830,#29831,#29832,#29833,#29834,#29835,#29836,
#29837,#29838,#29839,#29840,#29841,#29842,#29843,#29844,#29845,#29846,#29847,
#29848,#29849,#29850,#29851,#29852,#29853,#29854,#29855,#29856,#29857,#29858,
#29859,#29860,#29861,#29862,#29863,#29864,#29865,#29866,#29867,#29868,#29869,
#29870,#29871,#29872,#29873,#29874,#29875,#29876,#29877,#29878,#29879,#29880,
#29881,#29882,#29883,#29884,#29885,#29886,#29887,#29888,#29889,#29890,#29891,
#29892,#29893,#29894,#29895,#29896,#29897,#29898,#29899,#29900,#29901,#29902,
#29903,#29904,#29905,#29906,#29907,#29908,#29909,#29910,#29911,#29912,#29913,
#29914,#29915,#29916,#29917,#29918,#29919,#29920,#29921,#29922,#29923,#29924,
#29925,#29926,#29927,#29928,#29929,#29930,#29931,#29932,#29933,#29934,#29935,
#29936,#29937,#29938,#29939,#29940,#29941,#29942,#29943,#29944,#29945,#29946,
#29947,#29948,#29949,#29950,#29951,#29952,#29953,#29954,#29955,#29956,#29957,
#29958,#29959,#29960,#29961,#29962,#29963,#29964,#29965,#29966,#29967,#29968,
#29969,#29970,#29971,#29972,#29973,#29974,#29975,#29976,#29977,#29978,#29979,
#29980,#29981,#29982,#29983,#29984,#29985,#29986,#29987,#29988,#29989,#29990,
#29991,#29992,#29993,#29994,#29995,#29996,#29997,#29998,#29999,#30000,#30001,
#30002,#30003,#30004,#30005,#30006,#30007,#30008,#30009,#30010,#30011,#30012,
#30013,#30014,#30015,#30016,#30017,#30018,#30019,#30020,#30021,#30022,#30023,
#30024,#30025,#30026,#30027,#30028,#30029,#30030,#30031,#30032,#30033,#30034,
#30035,#30036,#30037,#30038,#30039,#30040,#30041,#30042,#30043,#30044,#30045,
#30046,#30047,#30048,#30049,#30050,#30051,#30052,#30053,#30054,#30055,#30056,
#30057,#30058,#30059,#30060,#30061,#30062,#30063,#30064,#30065,#30066,#30067,
#30068,#30069,#30070,#30071,#30072,#30073,#30074,#30075,#30076,#30077,#30078,
#30079,#30080,#30081,#30082,#30083,#30084,#30085,#30086,#30087,#30088,#30089,
#30090,#30091,#30092,#30093,#30094,#30095,#30096,#30097,#30098,#30099,#30100,
#30101,#30102,#30103,#30104,#30105,#30106,#30107,#30108,#30109,#30110,#30111,
#30112,#30113,#30114,#30115,#30116,#30117,#30118),.UNSPECIFIED.,.F.,.F.)
B_SPLINE_CURVE_WITH_KNOTS((3,2,2,2,2,2,2,2,2,2,2,2,2,2,2,2,2,2,2,2,2,2,
2,2,2,2,2,2,2,2,2,2,2,2,2,2,2,2,2,2,2,2,2,2,2,2,2,2,2,2,2,2,2,2,2,2,2,2,
2,2,2,2,2,2,2,2,2,2,2,2,2,2,2,2,2,2,2,2,2,2,2,2,2,2,2,2,2,2,2,2,2,2,2,2,
2,2,2,2,2,2,2,2,2,2,2,2,2,2,2,2,2,2,2,2,2,2,2,2,2,2,2,2,2,2,2,2,2,2,2,2,
2,2,2,2,2,2,2,2,2,2,2,2,2,2,2,2,2,2,2,2,3),(0.0578262804341777,0.063130434027066,
0.0694434774297724,0.0757565208324788,0.0820695642351851,0.0883826076378915,
0.0946956510405978,0.101008694443304,0.107321737846011,0.113634781248717,
0.119947824651423,0.12626086805413,0.132573911456836,0.138886954859542,
0.145199998262249,0.151513041664955,0.157826085067661,0.164139128470368,
0.170452171873074,0.17676521527578,0.183078258678487,0.189391302081193,
0.195704345483899,0.202017388886606,0.208330432289312,0.214643475692019,
0.220956519094725,0.227269562497431,0.233582605900138,0.239895649302844,
0.24620869270555,0.252521736108257,0.258834779510963,0.265147822913669,
0.271460866316376,0.277773909719082,0.284086953121788,0.290399996524495,
0.296713039927201,0.303026083329907,0.309339126732614,0.31565217013532,
0.321965213538027,0.328278256940733,0.334591300343439,0.340904343746146,
0.347217387148852,0.353530430551558,0.359843473954265,0.366156517356971,
0.372469560759677,0.378782604162384,0.38509564756509,0.391408690967797,
0.397721734370503,0.404034777773209,0.410347821175916,0.416660864578622,
0.422973907981328,0.429286951384035,0.435599994786741,0.441913038189447,
0.448226081592154,0.45453912499486,0.460852168397566,0.467165211800273,
0.473478255202979,0.479791298605685,0.486104342008392,0.492417385411098,
0.498730428813805,0.505043472216511,0.511356515619217,0.517669559021924,
0.52398260242463,0.530295645827336,0.536608689230043,0.542921732632749,
0.549234776035455,0.555547819438162,0.561860862840868,0.568173906243575,
0.574486949646281,0.580799993048987,0.587113036451693,0.5934260798544,0.599739123257106,
0.606052166659813,0.612365210062519,0.618678253465225,0.624991296867932,
0.631304340270638,0.637617383673344,0.643930427076051,0.650243470478757,
0.656556513881463,0.66286955728417,0.669182600686876,0.675495644089582,
0.681808687492289,0.688121730894995,0.694434774297702,0.700747817700408,
0.707060861103114,0.71337390450582,0.719686947908527,0.725999991311233,
0.732313034713939,0.738626078116646,0.744939121519352,0.751252164922059,
0.757565208324765,0.763878251727471,0.770191295130178,0.776504338532884,
0.78281738193559,0.789130425338297,0.795443468741003,0.80175651214371,0.808069555546416,
0.814382598949122,0.820695642351829,0.827008685754535,0.833321729157241,
0.839634772559948,0.845947815962654,0.85226085936536,0.858573902768067,
0.864886946170773,0.871199989573479,0.877513032976186,0.883826076378892,
0.890139119781598,0.896452163184305,0.902765206587011,0.909078249989718,
0.915391293392424,0.92170433679513,0.928017380197837,0.934330423600543,
0.940643467003249,0.946956510405956,0.953269553808662,0.959582597211368,
0.965895640614075,0.972208684016781,0.978521727419488,0.984834770822194,
0.9911478142249,0.997460857627607,1.),.UNSPECIFIED.)
CURVE()
GEOMETRIC_REPRESENTATION_ITEM()
RATIONAL_B_SPLINE_CURVE((0.964022189566827,0.887435933741894,1.,0.866025403784439,
1.,0.866025403784439,1.,0.866025403784439,1.,0.866025403784439,1.,0.866025403784439,
1.,0.866025403784439,1.,0.866025403784439,1.,0.866025403784439,1.,0.866025403784439,
1.,0.866025403784439,1.,0.866025403784439,1.,0.866025403784439,1.,0.866025403784439,
1.,0.866025403784439,1.,0.866025403784439,1.,0.866025403784439,1.,0.866025403784439,
1.,0.866025403784439,1.,0.866025403784439,1.,0.866025403784439,1.,0.866025403784439,
1.,0.866025403784439,1.,0.866025403784439,1.,0.866025403784439,1.,0.866025403784439,
1.,0.866025403784439,1.,0.866025403784439,1.,0.866025403784439,1.,0.866025403784439,
1.,0.866025403784439,1.,0.866025403784439,1.,0.866025403784439,1.,0.866025403784439,
1.,0.866025403784439,1.,0.866025403784439,1.,0.866025403784439,1.,0.866025403784439,
1.,0.866025403784439,1.,0.866025403784439,1.,0.866025403784439,1.,0.866025403784439,
1.,0.866025403784439,1.,0.866025403784439,1.,0.866025403784439,1.,0.866025403784439,
1.,0.866025403784439,1.,0.866025403784439,1.,0.866025403784439,1.,0.866025403784439,
1.,0.866025403784439,1.,0.866025403784439,1.,0.866025403784439,1.,0.866025403784439,
1.,0.866025403784439,1.,0.866025403784439,1.,0.866025403784439,1.,0.866025403784439,
1.,0.866025403784439,1.,0.866025403784439,1.,0.866025403784439,1.,0.866025403784439,
1.,0.866025403784439,1.,0.866025403784439,1.,0.866025403784439,1.,0.866025403784439,
1.,0.866025403784439,1.,0.866025403784439,1.,0.866025403784439,1.,0.866025403784439,
1.,0.866025403784439,1.,0.866025403784439,1.,0.866025403784439,1.,0.866025403784439,
1.,0.866025403784439,1.,0.866025403784439,1.,0.866025403784439,1.,0.866025403784439,
1.,0.866025403784439,1.,0.866025403784439,1.,0.866025403784439,1.,0.866025403784439,
1.,0.866025403784439,1.,0.866025403784439,1.,0.866025403784439,1.,0.866025403784439,
1.,0.866025403784439,1.,0.866025403784439,1.,0.866025403784439,1.,0.866025403784439,
1.,0.866025403784439,1.,0.866025403784439,1.,0.866025403784439,1.,0.866025403784439,
1.,0.866025403784439,1.,0.866025403784439,1.,0.866025403784439,1.,0.866025403784439,
1.,0.866025403784439,1.,0.866025403784439,1.,0.866025403784439,1.,0.866025403784439,
1.,0.866025403784439,1.,0.866025403784439,1.,0.866025403784439,1.,0.866025403784439,
1.,0.866025403784439,1.,0.866025403784439,1.,0.866025403784439,1.,0.866025403784439,
1.,0.866025403784439,1.,0.866025403784439,1.,0.866025403784439,1.,0.866025403784439,
1.,0.866025403784439,1.,0.866025403784439,1.,0.866025403784439,1.,0.866025403784439,
1.,0.866025403784439,1.,0.866025403784439,1.,0.866025403784439,1.,0.866025403784439,
1.,0.866025403784439,1.,0.866025403784439,1.,0.866025403784439,1.,0.866025403784439,
1.,0.866025403784439,1.,0.866025403784439,1.,0.866025403784439,1.,0.866025403784439,
1.,0.866025403784439,1.,0.866025403784439,1.,0.866025403784439,1.,0.866025403784439,
1.,0.866025403784439,1.,0.866025403784439,1.,0.866025403784439,1.,0.866025403784439,
1.,0.866025403784439,1.,0.866025403784439,1.,0.866025403784439,1.,0.866025403784439,
1.,0.866025403784439,1.,0.866025403784439,1.,0.866025403784439,1.,0.866025403784439,
1.,0.866025403784439,1.,0.866025403784439,1.,0.866025403784439,1.,0.946114646712328,
0.93557529156098))
REPRESENTATION_ITEM('')
);
#270=(
BOUNDED_CURVE()
B_SPLINE_CURVE(2,(#30760,#30761,#30762,#30763,#30764,#30765,#30766,#30767,
#30768,#30769,#30770,#30771,#30772,#30773,#30774,#30775,#30776,#30777,#30778,
#30779,#30780,#30781,#30782,#30783,#30784,#30785,#30786,#30787,#30788,#30789,
#30790,#30791,#30792,#30793,#30794,#30795,#30796,#30797,#30798,#30799,#30800,
#30801,#30802,#30803,#30804,#30805,#30806,#30807,#30808,#30809,#30810,#30811,
#30812,#30813,#30814,#30815,#30816,#30817,#30818,#30819,#30820,#30821,#30822,
#30823,#30824,#30825,#30826,#30827,#30828,#30829,#30830,#30831,#30832,#30833,
#30834,#30835,#30836,#30837,#30838,#30839,#30840,#30841,#30842,#30843,#30844,
#30845,#30846,#30847,#30848,#30849,#30850,#30851,#30852,#30853,#30854,#30855,
#30856,#30857,#30858,#30859,#30860,#30861,#30862,#30863,#30864,#30865,#30866,
#30867,#30868,#30869,#30870,#30871,#30872,#30873,#30874,#30875,#30876,#30877,
#30878,#30879,#30880,#30881,#30882,#30883,#30884,#30885,#30886,#30887,#30888,
#30889,#30890,#30891,#30892,#30893,#30894,#30895,#30896,#30897,#30898,#30899,
#30900,#30901,#30902,#30903,#30904,#30905,#30906,#30907,#30908,#30909,#30910,
#30911,#30912,#30913,#30914,#30915,#30916,#30917,#30918,#30919,#30920,#30921,
#30922,#30923,#30924,#30925,#30926,#30927,#30928,#30929,#30930,#30931,#30932,
#30933,#30934,#30935,#30936,#30937,#30938,#30939,#30940,#30941,#30942,#30943,
#30944,#30945,#30946,#30947,#30948,#30949,#30950,#30951,#30952,#30953,#30954,
#30955,#30956,#30957,#30958,#30959,#30960,#30961,#30962,#30963,#30964,#30965,
#30966,#30967,#30968,#30969,#30970,#30971,#30972,#30973,#30974,#30975,#30976,
#30977,#30978,#30979,#30980,#30981,#30982,#30983,#30984,#30985,#30986,#30987,
#30988,#30989,#30990,#30991,#30992,#30993,#30994,#30995,#30996,#30997,#30998,
#30999,#31000,#31001,#31002,#31003,#31004,#31005,#31006,#31007,#31008,#31009,
#31010,#31011,#31012,#31013,#31014,#31015,#31016,#31017,#31018,#31019,#31020,
#31021,#31022,#31023,#31024,#31025,#31026,#31027,#31028,#31029,#31030,#31031,
#31032,#31033,#31034,#31035,#31036,#31037,#31038,#31039,#31040,#31041,#31042,
#31043,#31044,#31045,#31046,#31047,#31048,#31049,#31050,#31051,#31052,#31053,
#31054,#31055,#31056,#31057,#31058,#31059,#31060),.UNSPECIFIED.,.F.,.F.)
B_SPLINE_CURVE_WITH_KNOTS((3,2,2,2,2,2,2,2,2,2,2,2,2,2,2,2,2,2,2,2,2,2,
2,2,2,2,2,2,2,2,2,2,2,2,2,2,2,2,2,2,2,2,2,2,2,2,2,2,2,2,2,2,2,2,2,2,2,2,
2,2,2,2,2,2,2,2,2,2,2,2,2,2,2,2,2,2,2,2,2,2,2,2,2,2,2,2,2,2,2,2,2,2,2,2,
2,2,2,2,2,2,2,2,2,2,2,2,2,2,2,2,2,2,2,2,2,2,2,2,2,2,2,2,2,2,2,2,2,2,2,2,
2,2,2,2,2,2,2,2,2,2,2,2,2,2,2,2,2,2,2,2,3),(0.0624132680173737,0.0631304316870872,
0.0694434748554592,0.0757565180238312,0.0820695611922032,0.0883826043605751,
0.0946956475289471,0.101008690697319,0.107321733865691,0.113634777034063,
0.119947820202435,0.126260863370807,0.132573906539179,0.138886949707551,
0.145199992875923,0.151513036044295,0.157826079212667,0.164139122381039,
0.170452165549411,0.176765208717783,0.183078251886155,0.189391295054527,
0.195704338222899,0.202017381391271,0.208330424559643,0.214643467728015,
0.220956510896387,0.227269554064759,0.233582597233131,0.239895640401503,
0.246208683569875,0.252521726738247,0.258834769906619,0.26514781307499,
0.271460856243362,0.277773899411734,0.284086942580106,0.290399985748478,
0.29671302891685,0.303026072085222,0.309339115253594,0.315652158421966,
0.321965201590338,0.32827824475871,0.334591287927082,0.340904331095454,
0.347217374263826,0.353530417432198,0.35984346060057,0.366156503768942,
0.372469546937314,0.378782590105686,0.385095633274058,0.39140867644243,
0.397721719610802,0.404034762779174,0.410347805947546,0.416660849115918,
0.42297389228429,0.429286935452662,0.435599978621034,0.441913021789406,
0.448226064957778,0.45453910812615,0.460852151294522,0.467165194462894,
0.473478237631266,0.479791280799638,0.48610432396801,0.492417367136382,
0.498730410304754,0.505043453473126,0.511356496641498,0.51766953980987,
0.523982582978242,0.530295626146613,0.536608669314985,0.542921712483357,
0.549234755651729,0.555547798820101,0.561860841988473,0.568173885156845,
0.574486928325217,0.580799971493589,0.587113014661961,0.593426057830333,
0.599739100998705,0.606052144167077,0.612365187335449,0.618678230503821,
0.624991273672193,0.631304316840565,0.637617360008937,0.643930403177309,
0.650243446345681,0.656556489514053,0.662869532682425,0.669182575850797,
0.675495619019169,0.681808662187541,0.688121705355913,0.694434748524285,
0.700747791692657,0.707060834861029,0.713373878029401,0.719686921197773,
0.725999964366145,0.732313007534517,0.738626050702889,0.744939093871261,
0.751252137039633,0.757565180208005,0.763878223376377,0.770191266544749,
0.776504309713121,0.782817352881493,0.789130396049865,0.795443439218236,
0.801756482386608,0.80806952555498,0.814382568723352,0.820695611891724,
0.827008655060096,0.833321698228468,0.83963474139684,0.845947784565212,
0.852260827733584,0.858573870901956,0.864886914070328,0.8711999572387,0.877513000407072,
0.883826043575444,0.890139086743816,0.896452129912188,0.90276517308056,
0.909078216248932,0.915391259417304,0.921704302585676,0.928017345754048,
0.93433038892242,0.940643432090792,0.946956475259164,0.953269518427536,
0.959582561595908,0.96589560476428,0.972208647932652,0.978521691101024,
0.984834734269396,0.991147777437768,0.99746082060614,1.),.UNSPECIFIED.)
CURVE()
GEOMETRIC_REPRESENTATION_ITEM()
RATIONAL_B_SPLINE_CURVE((0.973018780871376,0.984780444152242,1.,0.866025403784439,
1.,0.866025403784439,1.,0.866025403784439,1.,0.866025403784439,1.,0.866025403784439,
1.,0.866025403784439,1.,0.866025403784439,1.,0.866025403784439,1.,0.866025403784439,
1.,0.866025403784439,1.,0.866025403784439,1.,0.866025403784439,1.,0.866025403784439,
1.,0.866025403784439,1.,0.866025403784439,1.,0.866025403784439,1.,0.866025403784439,
1.,0.866025403784439,1.,0.866025403784439,1.,0.866025403784439,1.,0.866025403784439,
1.,0.866025403784439,1.,0.866025403784439,1.,0.866025403784439,1.,0.866025403784439,
1.,0.866025403784439,1.,0.866025403784439,1.,0.866025403784439,1.,0.866025403784439,
1.,0.866025403784439,1.,0.866025403784439,1.,0.866025403784439,1.,0.866025403784439,
1.,0.866025403784439,1.,0.866025403784439,1.,0.866025403784439,1.,0.866025403784439,
1.,0.866025403784439,1.,0.866025403784439,1.,0.866025403784439,1.,0.866025403784439,
1.,0.866025403784439,1.,0.866025403784439,1.,0.866025403784439,1.,0.866025403784439,
1.,0.866025403784439,1.,0.866025403784439,1.,0.866025403784439,1.,0.866025403784439,
1.,0.866025403784439,1.,0.866025403784439,1.,0.866025403784439,1.,0.866025403784439,
1.,0.866025403784439,1.,0.866025403784439,1.,0.866025403784439,1.,0.866025403784439,
1.,0.866025403784439,1.,0.866025403784439,1.,0.866025403784439,1.,0.866025403784439,
1.,0.866025403784439,1.,0.866025403784439,1.,0.866025403784439,1.,0.866025403784439,
1.,0.866025403784439,1.,0.866025403784439,1.,0.866025403784439,1.,0.866025403784439,
1.,0.866025403784439,1.,0.866025403784439,1.,0.866025403784439,1.,0.866025403784439,
1.,0.866025403784439,1.,0.866025403784439,1.,0.866025403784439,1.,0.866025403784439,
1.,0.866025403784439,1.,0.866025403784439,1.,0.866025403784439,1.,0.866025403784439,
1.,0.866025403784439,1.,0.866025403784439,1.,0.866025403784439,1.,0.866025403784439,
1.,0.866025403784439,1.,0.866025403784439,1.,0.866025403784439,1.,0.866025403784439,
1.,0.866025403784439,1.,0.866025403784439,1.,0.866025403784439,1.,0.866025403784439,
1.,0.866025403784439,1.,0.866025403784439,1.,0.866025403784439,1.,0.866025403784439,
1.,0.866025403784439,1.,0.866025403784439,1.,0.866025403784439,1.,0.866025403784439,
1.,0.866025403784439,1.,0.866025403784439,1.,0.866025403784439,1.,0.866025403784439,
1.,0.866025403784439,1.,0.866025403784439,1.,0.866025403784439,1.,0.866025403784439,
1.,0.866025403784439,1.,0.866025403784439,1.,0.866025403784439,1.,0.866025403784439,
1.,0.866025403784439,1.,0.866025403784439,1.,0.866025403784439,1.,0.866025403784439,
1.,0.866025403784439,1.,0.866025403784439,1.,0.866025403784439,1.,0.866025403784439,
1.,0.866025403784439,1.,0.866025403784439,1.,0.866025403784439,1.,0.866025403784439,
1.,0.866025403784439,1.,0.866025403784439,1.,0.866025403784439,1.,0.866025403784439,
1.,0.866025403784439,1.,0.866025403784439,1.,0.866025403784439,1.,0.866025403784439,
1.,0.866025403784439,1.,0.866025403784439,1.,0.866025403784439,1.,0.866025403784439,
1.,0.866025403784439,1.,0.866025403784439,1.,0.866025403784439,1.,0.866025403784439,
1.,0.866025403784439,1.,0.866025403784439,1.,0.866025403784439,1.,0.866025403784439,
1.,0.866025403784439,1.,0.866025403784439,1.,0.866025403784439,1.,0.946114646713198,
0.93557529156132))
REPRESENTATION_ITEM('')
);
#271=(
BOUNDED_CURVE()
B_SPLINE_CURVE(2,(#32344,#32345,#32346,#32347,#32348,#32349,#32350,#32351,
#32352,#32353,#32354,#32355,#32356,#32357,#32358,#32359,#32360,#32361,#32362,
#32363,#32364,#32365,#32366,#32367,#32368,#32369,#32370,#32371,#32372,#32373,
#32374,#32375,#32376,#32377,#32378,#32379,#32380,#32381,#32382,#32383,#32384,
#32385,#32386,#32387,#32388,#32389,#32390,#32391,#32392,#32393,#32394,#32395,
#32396,#32397,#32398,#32399,#32400,#32401,#32402,#32403,#32404,#32405,#32406,
#32407,#32408,#32409,#32410,#32411,#32412,#32413,#32414,#32415,#32416,#32417,
#32418,#32419,#32420,#32421,#32422,#32423,#32424,#32425,#32426,#32427,#32428,
#32429,#32430,#32431,#32432,#32433,#32434,#32435,#32436,#32437,#32438,#32439,
#32440,#32441,#32442,#32443,#32444,#32445,#32446,#32447,#32448,#32449,#32450,
#32451,#32452,#32453,#32454,#32455,#32456,#32457,#32458,#32459,#32460,#32461,
#32462,#32463,#32464,#32465,#32466,#32467,#32468,#32469,#32470,#32471,#32472,
#32473,#32474,#32475,#32476,#32477,#32478,#32479,#32480,#32481,#32482,#32483,
#32484,#32485,#32486,#32487,#32488,#32489,#32490,#32491,#32492,#32493,#32494,
#32495,#32496,#32497,#32498,#32499,#32500,#32501,#32502,#32503,#32504,#32505,
#32506,#32507,#32508,#32509,#32510,#32511,#32512,#32513,#32514,#32515,#32516,
#32517,#32518,#32519,#32520,#32521,#32522,#32523,#32524,#32525,#32526,#32527,
#32528,#32529,#32530,#32531,#32532,#32533,#32534,#32535,#32536,#32537,#32538,
#32539,#32540,#32541,#32542,#32543,#32544,#32545,#32546,#32547,#32548,#32549,
#32550,#32551,#32552,#32553,#32554,#32555,#32556,#32557,#32558,#32559,#32560,
#32561,#32562,#32563,#32564,#32565,#32566,#32567,#32568,#32569,#32570,#32571,
#32572,#32573,#32574,#32575,#32576,#32577,#32578,#32579,#32580,#32581,#32582,
#32583,#32584,#32585,#32586,#32587,#32588,#32589,#32590,#32591,#32592,#32593,
#32594,#32595,#32596,#32597,#32598,#32599,#32600,#32601,#32602,#32603,#32604,
#32605,#32606,#32607,#32608,#32609,#32610,#32611,#32612,#32613,#32614,#32615,
#32616,#32617,#32618,#32619,#32620,#32621,#32622,#32623,#32624,#32625,#32626,
#32627,#32628,#32629,#32630,#32631,#32632,#32633,#32634,#32635,#32636,#32637,
#32638,#32639,#32640,#32641,#32642,#32643,#32644),.UNSPECIFIED.,.F.,.F.)
B_SPLINE_CURVE_WITH_KNOTS((3,2,2,2,2,2,2,2,2,2,2,2,2,2,2,2,2,2,2,2,2,2,
2,2,2,2,2,2,2,2,2,2,2,2,2,2,2,2,2,2,2,2,2,2,2,2,2,2,2,2,2,2,2,2,2,2,2,2,
2,2,2,2,2,2,2,2,2,2,2,2,2,2,2,2,2,2,2,2,2,2,2,2,2,2,2,2,2,2,2,2,2,2,2,2,
2,2,2,2,2,2,2,2,2,2,2,2,2,2,2,2,2,2,2,2,2,2,2,2,2,2,2,2,2,2,2,2,2,2,2,2,
2,2,2,2,2,2,2,2,2,2,2,2,2,2,2,2,2,2,2,2,3),(0.0578262804341777,0.0631304340270661,
0.0694434774297724,0.0757565208324788,0.0820695642351851,0.0883826076378915,
0.0946956510405978,0.101008694443304,0.107321737846011,0.113634781248717,
0.119947824651423,0.12626086805413,0.132573911456836,0.138886954859542,
0.145199998262249,0.151513041664955,0.157826085067661,0.164139128470368,
0.170452171873074,0.17676521527578,0.183078258678487,0.189391302081193,
0.195704345483899,0.202017388886606,0.208330432289312,0.214643475692019,
0.220956519094725,0.227269562497431,0.233582605900138,0.239895649302844,
0.24620869270555,0.252521736108257,0.258834779510963,0.265147822913669,
0.271460866316376,0.277773909719082,0.284086953121788,0.290399996524495,
0.296713039927201,0.303026083329907,0.309339126732614,0.31565217013532,
0.321965213538027,0.328278256940733,0.334591300343439,0.340904343746146,
0.347217387148852,0.353530430551558,0.359843473954265,0.366156517356971,
0.372469560759677,0.378782604162384,0.38509564756509,0.391408690967796,
0.397721734370503,0.404034777773209,0.410347821175916,0.416660864578622,
0.422973907981328,0.429286951384035,0.435599994786741,0.441913038189447,
0.448226081592154,0.45453912499486,0.460852168397566,0.467165211800273,
0.473478255202979,0.479791298605685,0.486104342008392,0.492417385411098,
0.498730428813805,0.505043472216511,0.511356515619217,0.517669559021924,
0.52398260242463,0.530295645827336,0.536608689230043,0.542921732632749,
0.549234776035455,0.555547819438162,0.561860862840868,0.568173906243574,
0.574486949646281,0.580799993048987,0.587113036451694,0.5934260798544,0.599739123257106,
0.606052166659813,0.612365210062519,0.618678253465225,0.624991296867932,
0.631304340270638,0.637617383673344,0.643930427076051,0.650243470478757,
0.656556513881463,0.66286955728417,0.669182600686876,0.675495644089583,
0.681808687492289,0.688121730894995,0.694434774297702,0.700747817700408,
0.707060861103114,0.71337390450582,0.719686947908527,0.725999991311233,
0.73231303471394,0.738626078116646,0.744939121519352,0.751252164922059,
0.757565208324765,0.763878251727471,0.770191295130178,0.776504338532884,
0.78281738193559,0.789130425338297,0.795443468741003,0.80175651214371,0.808069555546416,
0.814382598949122,0.820695642351829,0.827008685754535,0.833321729157241,
0.839634772559948,0.845947815962654,0.85226085936536,0.858573902768067,
0.864886946170773,0.871199989573479,0.877513032976186,0.883826076378892,
0.890139119781598,0.896452163184305,0.902765206587011,0.909078249989718,
0.915391293392424,0.92170433679513,0.928017380197837,0.934330423600543,
0.940643467003249,0.946956510405956,0.953269553808662,0.959582597211368,
0.965895640614075,0.972208684016781,0.978521727419487,0.984834770822194,
0.9911478142249,0.997460857627607,1.),.UNSPECIFIED.)
CURVE()
GEOMETRIC_REPRESENTATION_ITEM()
RATIONAL_B_SPLINE_CURVE((0.964022189566828,0.887435933741894,1.,0.866025403784439,
1.,0.866025403784439,1.,0.866025403784439,1.,0.866025403784439,1.,0.866025403784439,
1.,0.866025403784439,1.,0.866025403784439,1.,0.866025403784439,1.,0.866025403784439,
1.,0.866025403784439,1.,0.866025403784439,1.,0.866025403784439,1.,0.866025403784439,
1.,0.866025403784439,1.,0.866025403784439,1.,0.866025403784439,1.,0.866025403784439,
1.,0.866025403784439,1.,0.866025403784439,1.,0.866025403784439,1.,0.866025403784439,
1.,0.866025403784439,1.,0.866025403784439,1.,0.866025403784439,1.,0.866025403784439,
1.,0.866025403784439,1.,0.866025403784439,1.,0.866025403784439,1.,0.866025403784439,
1.,0.866025403784439,1.,0.866025403784439,1.,0.866025403784439,1.,0.866025403784439,
1.,0.866025403784439,1.,0.866025403784439,1.,0.866025403784439,1.,0.866025403784439,
1.,0.866025403784439,1.,0.866025403784439,1.,0.866025403784439,1.,0.866025403784439,
1.,0.866025403784439,1.,0.866025403784439,1.,0.866025403784439,1.,0.866025403784439,
1.,0.866025403784439,1.,0.866025403784439,1.,0.866025403784439,1.,0.866025403784439,
1.,0.866025403784439,1.,0.866025403784439,1.,0.866025403784439,1.,0.866025403784439,
1.,0.866025403784439,1.,0.866025403784439,1.,0.866025403784439,1.,0.866025403784439,
1.,0.866025403784439,1.,0.866025403784439,1.,0.866025403784439,1.,0.866025403784439,
1.,0.866025403784439,1.,0.866025403784439,1.,0.866025403784439,1.,0.866025403784439,
1.,0.866025403784439,1.,0.866025403784439,1.,0.866025403784439,1.,0.866025403784439,
1.,0.866025403784439,1.,0.866025403784439,1.,0.866025403784439,1.,0.866025403784439,
1.,0.866025403784439,1.,0.866025403784439,1.,0.866025403784439,1.,0.866025403784439,
1.,0.866025403784439,1.,0.866025403784439,1.,0.866025403784439,1.,0.866025403784439,
1.,0.866025403784439,1.,0.866025403784439,1.,0.866025403784439,1.,0.866025403784439,
1.,0.866025403784439,1.,0.866025403784439,1.,0.866025403784439,1.,0.866025403784439,
1.,0.866025403784439,1.,0.866025403784439,1.,0.866025403784439,1.,0.866025403784439,
1.,0.866025403784439,1.,0.866025403784439,1.,0.866025403784439,1.,0.866025403784439,
1.,0.866025403784439,1.,0.866025403784439,1.,0.866025403784439,1.,0.866025403784439,
1.,0.866025403784439,1.,0.866025403784439,1.,0.866025403784439,1.,0.866025403784439,
1.,0.866025403784439,1.,0.866025403784439,1.,0.866025403784439,1.,0.866025403784439,
1.,0.866025403784439,1.,0.866025403784439,1.,0.866025403784439,1.,0.866025403784439,
1.,0.866025403784439,1.,0.866025403784439,1.,0.866025403784439,1.,0.866025403784439,
1.,0.866025403784439,1.,0.866025403784439,1.,0.866025403784439,1.,0.866025403784439,
1.,0.866025403784439,1.,0.866025403784439,1.,0.866025403784439,1.,0.866025403784439,
1.,0.866025403784439,1.,0.866025403784439,1.,0.866025403784439,1.,0.866025403784439,
1.,0.866025403784439,1.,0.866025403784439,1.,0.866025403784439,1.,0.866025403784439,
1.,0.866025403784439,1.,0.866025403784439,1.,0.866025403784439,1.,0.866025403784439,
1.,0.866025403784439,1.,0.866025403784439,1.,0.866025403784439,1.,0.866025403784439,
1.,0.866025403784439,1.,0.866025403784439,1.,0.866025403784439,1.,0.866025403784439,
1.,0.866025403784439,1.,0.866025403784439,1.,0.866025403784439,1.,0.946114646712328,
0.93557529156098))
REPRESENTATION_ITEM('')
);
#272=(
BOUNDED_CURVE()
B_SPLINE_CURVE(2,(#33286,#33287,#33288,#33289,#33290,#33291,#33292,#33293,
#33294,#33295,#33296,#33297,#33298,#33299,#33300,#33301,#33302,#33303,#33304,
#33305,#33306,#33307,#33308,#33309,#33310,#33311,#33312,#33313,#33314,#33315,
#33316,#33317,#33318,#33319,#33320,#33321,#33322,#33323,#33324,#33325,#33326,
#33327,#33328,#33329,#33330,#33331,#33332,#33333,#33334,#33335,#33336,#33337,
#33338,#33339,#33340,#33341,#33342,#33343,#33344,#33345,#33346,#33347,#33348,
#33349,#33350,#33351,#33352,#33353,#33354,#33355,#33356,#33357,#33358,#33359,
#33360,#33361,#33362,#33363,#33364,#33365,#33366,#33367,#33368,#33369,#33370,
#33371,#33372,#33373,#33374,#33375,#33376,#33377,#33378,#33379,#33380,#33381,
#33382,#33383,#33384,#33385,#33386,#33387,#33388,#33389,#33390,#33391,#33392,
#33393,#33394,#33395,#33396,#33397,#33398,#33399,#33400,#33401,#33402,#33403,
#33404,#33405,#33406,#33407,#33408,#33409,#33410,#33411,#33412,#33413,#33414,
#33415,#33416,#33417,#33418,#33419,#33420,#33421,#33422,#33423,#33424,#33425,
#33426,#33427,#33428,#33429,#33430,#33431,#33432,#33433,#33434,#33435,#33436,
#33437,#33438,#33439,#33440,#33441,#33442,#33443,#33444,#33445,#33446,#33447,
#33448,#33449,#33450,#33451,#33452,#33453,#33454,#33455,#33456,#33457,#33458,
#33459,#33460,#33461,#33462,#33463,#33464,#33465,#33466,#33467,#33468,#33469,
#33470,#33471,#33472,#33473,#33474,#33475,#33476,#33477,#33478,#33479,#33480,
#33481,#33482,#33483,#33484,#33485,#33486,#33487,#33488,#33489,#33490,#33491,
#33492,#33493,#33494,#33495,#33496,#33497,#33498,#33499,#33500,#33501,#33502,
#33503,#33504,#33505,#33506,#33507,#33508,#33509,#33510,#33511,#33512,#33513,
#33514,#33515,#33516,#33517,#33518,#33519,#33520,#33521,#33522,#33523,#33524,
#33525,#33526,#33527,#33528,#33529,#33530,#33531,#33532,#33533,#33534,#33535,
#33536,#33537,#33538,#33539,#33540,#33541,#33542,#33543,#33544,#33545,#33546,
#33547,#33548,#33549,#33550,#33551,#33552,#33553,#33554,#33555,#33556,#33557,
#33558,#33559,#33560,#33561,#33562,#33563,#33564,#33565,#33566,#33567,#33568,
#33569,#33570,#33571,#33572,#33573,#33574,#33575,#33576,#33577,#33578,#33579,
#33580,#33581,#33582,#33583,#33584,#33585,#33586),.UNSPECIFIED.,.F.,.F.)
B_SPLINE_CURVE_WITH_KNOTS((3,2,2,2,2,2,2,2,2,2,2,2,2,2,2,2,2,2,2,2,2,2,
2,2,2,2,2,2,2,2,2,2,2,2,2,2,2,2,2,2,2,2,2,2,2,2,2,2,2,2,2,2,2,2,2,2,2,2,
2,2,2,2,2,2,2,2,2,2,2,2,2,2,2,2,2,2,2,2,2,2,2,2,2,2,2,2,2,2,2,2,2,2,2,2,
2,2,2,2,2,2,2,2,2,2,2,2,2,2,2,2,2,2,2,2,2,2,2,2,2,2,2,2,2,2,2,2,2,2,2,2,
2,2,2,2,2,2,2,2,2,2,2,2,2,2,2,2,2,2,2,2,3),(0.0624132680173737,0.0631304316872321,
0.0694434748568796,0.0757565180265271,0.0820695611961746,0.088382604365822,
0.0946956475354695,0.101008690705117,0.107321733874764,0.113634777044412,
0.119947820214059,0.126260863383707,0.132573906553354,0.138886949723002,
0.145199992892649,0.151513036062297,0.157826079231944,0.164139122401592,
0.170452165571239,0.176765208740887,0.183078251910534,0.189391295080182,
0.195704338249829,0.202017381419477,0.208330424589124,0.214643467758772,
0.220956510928419,0.227269554098067,0.233582597267714,0.239895640437362,
0.246208683607009,0.252521726776657,0.258834769946304,0.265147813115952,
0.271460856285599,0.277773899455247,0.284086942624894,0.290399985794542,
0.296713028964189,0.303026072133836,0.309339115303484,0.315652158473131,
0.321965201642779,0.328278244812426,0.334591287982074,0.340904331151721,
0.347217374321369,0.353530417491016,0.359843460660664,0.366156503830311,
0.372469546999959,0.378782590169606,0.385095633339254,0.391408676508901,
0.397721719678549,0.404034762848196,0.410347806017844,0.416660849187491,
0.422973892357139,0.429286935526786,0.435599978696434,0.441913021866081,
0.448226065035729,0.454539108205376,0.460852151375024,0.467165194544671,
0.473478237714319,0.479791280883966,0.486104324053614,0.492417367223261,
0.498730410392908,0.505043453562556,0.511356496732204,0.517669539901851,
0.523982583071499,0.530295626241146,0.536608669410793,0.542921712580441,
0.549234755750089,0.555547798919736,0.561860842089383,0.568173885259031,
0.574486928428678,0.580799971598326,0.587113014767973,0.593426057937621,
0.599739101107268,0.606052144276916,0.612365187446563,0.618678230616211,
0.624991273785858,0.631304316955506,0.637617360125153,0.643930403294801,
0.650243446464448,0.656556489634096,0.662869532803743,0.669182575973391,
0.675495619143038,0.681808662312686,0.688121705482333,0.694434748651981,
0.700747791821628,0.707060834991275,0.713373878160923,0.719686921330571,
0.725999964500218,0.732313007669865,0.738626050839513,0.74493909400916,
0.751252137178808,0.757565180348455,0.763878223518103,0.77019126668775,
0.776504309857398,0.782817353027045,0.789130396196693,0.79544343936634,
0.801756482535988,0.808069525705635,0.814382568875283,0.82069561204493,
0.827008655214578,0.833321698384225,0.839634741553873,0.84594778472352,
0.852260827893168,0.858573871062815,0.864886914232463,0.87119995740211,
0.877513000571758,0.883826043741405,0.890139086911052,0.8964521300807,0.902765173250348,
0.909078216419995,0.915391259589642,0.92170430275929,0.928017345928937,
0.934330389098585,0.940643432268232,0.94695647543788,0.953269518607527,
0.959582561777175,0.965895604946822,0.97220864811647,0.978521691286117,
0.984834734455765,0.991147777625412,0.99746082079506,1.),.UNSPECIFIED.)
CURVE()
GEOMETRIC_REPRESENTATION_ITEM()
RATIONAL_B_SPLINE_CURVE((0.973018780871376,0.984780444152243,1.,0.866025403784439,
1.,0.866025403784439,1.,0.866025403784439,1.,0.866025403784439,1.,0.866025403784439,
1.,0.866025403784439,1.,0.866025403784439,1.,0.866025403784439,1.,0.866025403784439,
1.,0.866025403784439,1.,0.866025403784439,1.,0.866025403784439,1.,0.866025403784439,
1.,0.866025403784439,1.,0.866025403784439,1.,0.866025403784439,1.,0.866025403784439,
1.,0.866025403784439,1.,0.866025403784439,1.,0.866025403784439,1.,0.866025403784439,
1.,0.866025403784439,1.,0.866025403784439,1.,0.866025403784439,1.,0.866025403784439,
1.,0.866025403784439,1.,0.866025403784439,1.,0.866025403784439,1.,0.866025403784439,
1.,0.866025403784439,1.,0.866025403784439,1.,0.866025403784439,1.,0.866025403784439,
1.,0.866025403784439,1.,0.866025403784439,1.,0.866025403784439,1.,0.866025403784439,
1.,0.866025403784439,1.,0.866025403784439,1.,0.866025403784439,1.,0.866025403784439,
1.,0.866025403784439,1.,0.866025403784439,1.,0.866025403784439,1.,0.866025403784439,
1.,0.866025403784439,1.,0.866025403784439,1.,0.866025403784439,1.,0.866025403784439,
1.,0.866025403784439,1.,0.866025403784439,1.,0.866025403784439,1.,0.866025403784439,
1.,0.866025403784439,1.,0.866025403784439,1.,0.866025403784439,1.,0.866025403784439,
1.,0.866025403784439,1.,0.866025403784439,1.,0.866025403784439,1.,0.866025403784439,
1.,0.866025403784439,1.,0.866025403784439,1.,0.866025403784439,1.,0.866025403784439,
1.,0.866025403784439,1.,0.866025403784439,1.,0.866025403784439,1.,0.866025403784439,
1.,0.866025403784439,1.,0.866025403784439,1.,0.866025403784439,1.,0.866025403784439,
1.,0.866025403784439,1.,0.866025403784439,1.,0.866025403784439,1.,0.866025403784439,
1.,0.866025403784439,1.,0.866025403784439,1.,0.866025403784439,1.,0.866025403784439,
1.,0.866025403784439,1.,0.866025403784439,1.,0.866025403784439,1.,0.866025403784439,
1.,0.866025403784439,1.,0.866025403784439,1.,0.866025403784439,1.,0.866025403784439,
1.,0.866025403784439,1.,0.866025403784439,1.,0.866025403784439,1.,0.866025403784439,
1.,0.866025403784439,1.,0.866025403784439,1.,0.866025403784439,1.,0.866025403784439,
1.,0.866025403784439,1.,0.866025403784439,1.,0.866025403784439,1.,0.866025403784439,
1.,0.866025403784439,1.,0.866025403784439,1.,0.866025403784439,1.,0.866025403784439,
1.,0.866025403784439,1.,0.866025403784439,1.,0.866025403784439,1.,0.866025403784439,
1.,0.866025403784439,1.,0.866025403784439,1.,0.866025403784439,1.,0.866025403784439,
1.,0.866025403784439,1.,0.866025403784439,1.,0.866025403784439,1.,0.866025403784439,
1.,0.866025403784439,1.,0.866025403784439,1.,0.866025403784439,1.,0.866025403784439,
1.,0.866025403784439,1.,0.866025403784439,1.,0.866025403784439,1.,0.866025403784439,
1.,0.866025403784439,1.,0.866025403784439,1.,0.866025403784439,1.,0.866025403784439,
1.,0.866025403784439,1.,0.866025403784439,1.,0.866025403784439,1.,0.866025403784439,
1.,0.866025403784439,1.,0.866025403784439,1.,0.866025403784439,1.,0.866025403784439,
1.,0.866025403784439,1.,0.866025403784439,1.,0.866025403784439,1.,0.866025403784439,
1.,0.866025403784439,1.,0.866025403784439,1.,0.866025403784439,1.,0.866025403784439,
1.,0.866025403784439,1.,0.866025403784439,1.,0.866025403784439,1.,0.946114646713198,
0.93557529156132))
REPRESENTATION_ITEM('')
);
#273=(
BOUNDED_CURVE()
B_SPLINE_CURVE(2,(#34305,#34306,#34307),.UNSPECIFIED.,.F.,.F.)
B_SPLINE_CURVE_WITH_KNOTS((3,3),(3.14998285709622,4.30410895504795),
 .UNSPECIFIED.)
CURVE()
GEOMETRIC_REPRESENTATION_ITEM()
RATIONAL_B_SPLINE_CURVE((6.34638554216859,6.34638554216859,5.62867319679424))
REPRESENTATION_ITEM('')
);
#274=(
BOUNDED_CURVE()
B_SPLINE_CURVE(2,(#34312,#34313,#34314),.UNSPECIFIED.,.F.,.F.)
B_SPLINE_CURVE_WITH_KNOTS((3,3),(1.9958567591426,3.14998285709622),
 .UNSPECIFIED.)
CURVE()
GEOMETRIC_REPRESENTATION_ITEM()
RATIONAL_B_SPLINE_CURVE((5.62867319679188,6.34638554216859,6.34638554216859))
REPRESENTATION_ITEM('')
);
#289=(
BOUNDED_SURFACE()
B_SPLINE_SURFACE(1,2,((#24102,#24103,#24104,#24105,#24106,#24107,#24108,
#24109,#24110,#24111,#24112,#24113,#24114,#24115,#24116,#24117,#24118,#24119,
#24120,#24121,#24122,#24123,#24124,#24125,#24126,#24127,#24128,#24129,#24130,
#24131,#24132,#24133,#24134,#24135,#24136,#24137,#24138,#24139,#24140,#24141,
#24142,#24143,#24144,#24145,#24146,#24147,#24148,#24149,#24150,#24151,#24152,
#24153,#24154,#24155,#24156,#24157,#24158,#24159,#24160,#24161,#24162,#24163,
#24164,#24165,#24166,#24167,#24168,#24169,#24170,#24171,#24172,#24173,#24174,
#24175,#24176,#24177,#24178,#24179,#24180,#24181,#24182,#24183,#24184,#24185,
#24186,#24187,#24188,#24189,#24190,#24191,#24192,#24193,#24194,#24195,#24196,
#24197,#24198,#24199,#24200,#24201,#24202,#24203,#24204,#24205,#24206,#24207,
#24208,#24209,#24210,#24211,#24212,#24213,#24214,#24215,#24216,#24217,#24218,
#24219,#24220,#24221,#24222,#24223,#24224,#24225,#24226,#24227,#24228,#24229,
#24230,#24231,#24232,#24233,#24234,#24235,#24236,#24237,#24238,#24239,#24240,
#24241,#24242,#24243,#24244,#24245,#24246,#24247,#24248,#24249,#24250,#24251,
#24252,#24253,#24254,#24255,#24256,#24257,#24258,#24259,#24260,#24261,#24262,
#24263,#24264,#24265,#24266,#24267,#24268,#24269,#24270,#24271,#24272,#24273,
#24274,#24275,#24276,#24277,#24278,#24279,#24280,#24281,#24282,#24283,#24284,
#24285,#24286,#24287,#24288,#24289,#24290,#24291,#24292,#24293,#24294,#24295,
#24296,#24297,#24298,#24299,#24300,#24301,#24302,#24303,#24304,#24305,#24306,
#24307,#24308,#24309,#24310,#24311,#24312,#24313,#24314,#24315,#24316,#24317,
#24318,#24319,#24320,#24321,#24322,#24323,#24324,#24325,#24326,#24327,#24328,
#24329,#24330,#24331,#24332,#24333,#24334,#24335,#24336,#24337,#24338,#24339,
#24340,#24341,#24342,#24343,#24344,#24345,#24346,#24347,#24348,#24349,#24350,
#24351,#24352,#24353,#24354,#24355,#24356,#24357,#24358,#24359,#24360,#24361,
#24362,#24363,#24364,#24365,#24366,#24367,#24368,#24369,#24370,#24371,#24372,
#24373,#24374,#24375,#24376,#24377,#24378,#24379,#24380,#24381,#24382,#24383,
#24384,#24385,#24386,#24387,#24388,#24389,#24390,#24391,#24392,#24393,#24394,
#24395,#24396,#24397,#24398,#24399,#24400,#24401,#24402,#24403,#24404,#24405,
#24406,#24407,#24408,#24409,#24410,#24411,#24412,#24413,#24414,#24415,#24416,
#24417,#24418,#24419,#24420),(#24421,#24422,#24423,#24424,#24425,#24426,
#24427,#24428,#24429,#24430,#24431,#24432,#24433,#24434,#24435,#24436,#24437,
#24438,#24439,#24440,#24441,#24442,#24443,#24444,#24445,#24446,#24447,#24448,
#24449,#24450,#24451,#24452,#24453,#24454,#24455,#24456,#24457,#24458,#24459,
#24460,#24461,#24462,#24463,#24464,#24465,#24466,#24467,#24468,#24469,#24470,
#24471,#24472,#24473,#24474,#24475,#24476,#24477,#24478,#24479,#24480,#24481,
#24482,#24483,#24484,#24485,#24486,#24487,#24488,#24489,#24490,#24491,#24492,
#24493,#24494,#24495,#24496,#24497,#24498,#24499,#24500,#24501,#24502,#24503,
#24504,#24505,#24506,#24507,#24508,#24509,#24510,#24511,#24512,#24513,#24514,
#24515,#24516,#24517,#24518,#24519,#24520,#24521,#24522,#24523,#24524,#24525,
#24526,#24527,#24528,#24529,#24530,#24531,#24532,#24533,#24534,#24535,#24536,
#24537,#24538,#24539,#24540,#24541,#24542,#24543,#24544,#24545,#24546,#24547,
#24548,#24549,#24550,#24551,#24552,#24553,#24554,#24555,#24556,#24557,#24558,
#24559,#24560,#24561,#24562,#24563,#24564,#24565,#24566,#24567,#24568,#24569,
#24570,#24571,#24572,#24573,#24574,#24575,#24576,#24577,#24578,#24579,#24580,
#24581,#24582,#24583,#24584,#24585,#24586,#24587,#24588,#24589,#24590,#24591,
#24592,#24593,#24594,#24595,#24596,#24597,#24598,#24599,#24600,#24601,#24602,
#24603,#24604,#24605,#24606,#24607,#24608,#24609,#24610,#24611,#24612,#24613,
#24614,#24615,#24616,#24617,#24618,#24619,#24620,#24621,#24622,#24623,#24624,
#24625,#24626,#24627,#24628,#24629,#24630,#24631,#24632,#24633,#24634,#24635,
#24636,#24637,#24638,#24639,#24640,#24641,#24642,#24643,#24644,#24645,#24646,
#24647,#24648,#24649,#24650,#24651,#24652,#24653,#24654,#24655,#24656,#24657,
#24658,#24659,#24660,#24661,#24662,#24663,#24664,#24665,#24666,#24667,#24668,
#24669,#24670,#24671,#24672,#24673,#24674,#24675,#24676,#24677,#24678,#24679,
#24680,#24681,#24682,#24683,#24684,#24685,#24686,#24687,#24688,#24689,#24690,
#24691,#24692,#24693,#24694,#24695,#24696,#24697,#24698,#24699,#24700,#24701,
#24702,#24703,#24704,#24705,#24706,#24707,#24708,#24709,#24710,#24711,#24712,
#24713,#24714,#24715,#24716,#24717,#24718,#24719,#24720,#24721,#24722,#24723,
#24724,#24725,#24726,#24727,#24728,#24729,#24730,#24731,#24732,#24733,#24734,
#24735,#24736,#24737,#24738,#24739)),.UNSPECIFIED.,.F.,.F.,.F.)
B_SPLINE_SURFACE_WITH_KNOTS((2,2),(3,2,2,2,2,2,2,2,2,2,2,2,2,2,2,2,2,2,
2,2,2,2,2,2,2,2,2,2,2,2,2,2,2,2,2,2,2,2,2,2,2,2,2,2,2,2,2,2,2,2,2,2,2,2,
2,2,2,2,2,2,2,2,2,2,2,2,2,2,2,2,2,2,2,2,2,2,2,2,2,2,2,2,2,2,2,2,2,2,2,2,
2,2,2,2,2,2,2,2,2,2,2,2,2,2,2,2,2,2,2,2,2,2,2,2,2,2,2,2,2,2,2,2,2,2,2,2,
2,2,2,2,2,2,2,2,2,2,2,2,2,2,2,2,2,2,2,2,2,2,2,2,2,2,2,2,2,2,2,2,2,3),(-2.4733869132694E-5,
1.),(0.,0.00617283950617284,0.0123456790123457,0.0185185185185185,0.0246913580246914,
0.0308641975308642,0.037037037037037,0.0432098765432099,0.0493827160493827,
0.0555555555555556,0.0617283950617284,0.0679012345679012,0.0740740740740741,
0.0802469135802469,0.0864197530864197,0.0925925925925926,0.0987654320987654,
0.104938271604938,0.111111111111111,0.117283950617284,0.123456790123457,
0.12962962962963,0.135802469135802,0.141975308641975,0.148148148148148,
0.154320987654321,0.160493827160494,0.166666666666667,0.172839506172839,
0.179012345679012,0.185185185185185,0.191358024691358,0.197530864197531,
0.203703703703704,0.209876543209877,0.216049382716049,0.222222222222222,
0.228395061728395,0.234567901234568,0.240740740740741,0.246913580246914,
0.253086419753086,0.259259259259259,0.265432098765432,0.271604938271605,
0.277777777777778,0.283950617283951,0.290123456790123,0.296296296296296,
0.302469135802469,0.308641975308642,0.314814814814815,0.320987654320988,
0.327160493827161,0.333333333333333,0.339506172839506,0.345679012345679,
0.351851851851852,0.358024691358025,0.364197530864198,0.37037037037037,
0.376543209876543,0.382716049382716,0.388888888888889,0.395061728395062,
0.401234567901235,0.407407407407407,0.41358024691358,0.419753086419753,
0.425925925925926,0.432098765432099,0.438271604938272,0.444444444444444,
0.450617283950617,0.45679012345679,0.462962962962963,0.469135802469136,
0.475308641975309,0.481481481481481,0.487654320987654,0.493827160493827,
0.5,0.506172839506173,0.512345679012346,0.518518518518518,0.524691358024691,
0.530864197530864,0.537037037037037,0.54320987654321,0.549382716049383,
0.555555555555556,0.561728395061728,0.567901234567901,0.574074074074074,
0.580246913580247,0.58641975308642,0.592592592592593,0.598765432098765,
0.604938271604938,0.611111111111111,0.617283950617284,0.623456790123457,
0.62962962962963,0.635802469135803,0.641975308641975,0.648148148148148,
0.654320987654321,0.660493827160494,0.666666666666667,0.672839506172839,
0.679012345679012,0.685185185185185,0.691358024691358,0.697530864197531,
0.703703703703704,0.709876543209877,0.716049382716049,0.722222222222222,
0.728395061728395,0.734567901234568,0.740740740740741,0.746913580246914,
0.753086419753086,0.759259259259259,0.765432098765432,0.771604938271605,
0.777777777777778,0.783950617283951,0.790123456790123,0.796296296296296,
0.802469135802469,0.808641975308642,0.814814814814815,0.820987654320988,
0.827160493827161,0.833333333333333,0.839506172839506,0.845679012345679,
0.851851851851852,0.858024691358025,0.864197530864197,0.87037037037037,
0.876543209876543,0.882716049382716,0.888888888888889,0.895061728395062,
0.901234567901235,0.907407407407407,0.91358024691358,0.919753086419753,
0.925925925925926,0.932098765432099,0.938271604938272,0.944444444444444,
0.950617283950617,0.95679012345679,0.962962962962963,0.969135802469136,
0.975308641975309,0.977791447664447),.UNSPECIFIED.)
GEOMETRIC_REPRESENTATION_ITEM()
RATIONAL_B_SPLINE_SURFACE(((1.,0.866025403784439,1.,0.866025403784439,1.,
0.866025403784439,1.,0.866025403784439,1.,0.866025403784439,1.,0.866025403784439,
1.,0.866025403784439,1.,0.866025403784439,1.,0.866025403784439,1.,0.866025403784439,
1.,0.866025403784439,1.,0.866025403784439,1.,0.866025403784439,1.,0.866025403784439,
1.,0.866025403784439,1.,0.866025403784439,1.,0.866025403784439,1.,0.866025403784439,
1.,0.866025403784439,1.,0.866025403784439,1.,0.866025403784439,1.,0.866025403784439,
1.,0.866025403784439,1.,0.866025403784439,1.,0.866025403784439,1.,0.866025403784439,
1.,0.866025403784439,1.,0.866025403784439,1.,0.866025403784439,1.,0.866025403784439,
1.,0.866025403784439,1.,0.866025403784439,1.,0.866025403784439,1.,0.866025403784439,
1.,0.866025403784439,1.,0.866025403784439,1.,0.866025403784439,1.,0.866025403784439,
1.,0.866025403784439,1.,0.866025403784439,1.,0.866025403784439,1.,0.866025403784439,
1.,0.866025403784439,1.,0.866025403784439,1.,0.866025403784439,1.,0.866025403784439,
1.,0.866025403784439,1.,0.866025403784439,1.,0.866025403784439,1.,0.866025403784439,
1.,0.866025403784439,1.,0.866025403784439,1.,0.866025403784439,1.,0.866025403784439,
1.,0.866025403784439,1.,0.866025403784439,1.,0.866025403784439,1.,0.866025403784439,
1.,0.866025403784439,1.,0.866025403784439,1.,0.866025403784439,1.,0.866025403784439,
1.,0.866025403784439,1.,0.866025403784439,1.,0.866025403784439,1.,0.866025403784439,
1.,0.866025403784439,1.,0.866025403784439,1.,0.866025403784439,1.,0.866025403784439,
1.,0.866025403784439,1.,0.866025403784439,1.,0.866025403784439,1.,0.866025403784439,
1.,0.866025403784439,1.,0.866025403784439,1.,0.866025403784439,1.,0.866025403784439,
1.,0.866025403784439,1.,0.866025403784439,1.,0.866025403784439,1.,0.866025403784439,
1.,0.866025403784439,1.,0.866025403784439,1.,0.866025403784439,1.,0.866025403784439,
1.,0.866025403784439,1.,0.866025403784439,1.,0.866025403784439,1.,0.866025403784439,
1.,0.866025403784439,1.,0.866025403784439,1.,0.866025403784439,1.,0.866025403784439,
1.,0.866025403784439,1.,0.866025403784439,1.,0.866025403784439,1.,0.866025403784439,
1.,0.866025403784439,1.,0.866025403784439,1.,0.866025403784439,1.,0.866025403784439,
1.,0.866025403784439,1.,0.866025403784439,1.,0.866025403784439,1.,0.866025403784439,
1.,0.866025403784439,1.,0.866025403784439,1.,0.866025403784439,1.,0.866025403784439,
1.,0.866025403784439,1.,0.866025403784439,1.,0.866025403784439,1.,0.866025403784439,
1.,0.866025403784439,1.,0.866025403784439,1.,0.866025403784439,1.,0.866025403784439,
1.,0.866025403784439,1.,0.866025403784439,1.,0.866025403784439,1.,0.866025403784439,
1.,0.866025403784439,1.,0.866025403784439,1.,0.866025403784439,1.,0.866025403784439,
1.,0.866025403784439,1.,0.866025403784439,1.,0.866025403784439,1.,0.866025403784439,
1.,0.866025403784439,1.,0.866025403784439,1.,0.866025403784439,1.,0.866025403784439,
1.,0.866025403784439,1.,0.866025403784439,1.,0.866025403784439,1.,0.866025403784439,
1.,0.866025403784439,1.,0.866025403784439,1.,0.866025403784439,1.,0.866025403784439,
1.,0.866025403784439,1.,0.866025403784439,1.,0.866025403784439,1.,0.866025403784439,
1.,0.866025403784439,1.,0.866025403784439,1.,0.866025403784439,1.,0.866025403784439,
1.,0.866025403784439,1.,0.866025403784439,1.,0.866025403784439,1.,0.866025403784439,
1.,0.866025403784439,1.,0.866025403784439,1.,0.866025403784439,1.,0.866025403784439,
1.,0.9461134718712,0.935574832010768),(1.,0.866025403784439,1.,0.866025403784439,
1.,0.866025403784439,1.,0.866025403784439,1.,0.866025403784439,1.,0.866025403784439,
1.,0.866025403784439,1.,0.866025403784439,1.,0.866025403784439,1.,0.866025403784439,
1.,0.866025403784439,1.,0.866025403784439,1.,0.866025403784439,1.,0.866025403784439,
1.,0.866025403784439,1.,0.866025403784439,1.,0.866025403784439,1.,0.866025403784439,
1.,0.866025403784439,1.,0.866025403784439,1.,0.866025403784439,1.,0.866025403784439,
1.,0.866025403784439,1.,0.866025403784439,1.,0.866025403784439,1.,0.866025403784439,
1.,0.866025403784439,1.,0.866025403784439,1.,0.866025403784439,1.,0.866025403784439,
1.,0.866025403784439,1.,0.866025403784439,1.,0.866025403784439,1.,0.866025403784439,
1.,0.866025403784439,1.,0.866025403784439,1.,0.866025403784439,1.,0.866025403784439,
1.,0.866025403784439,1.,0.866025403784439,1.,0.866025403784439,1.,0.866025403784439,
1.,0.866025403784439,1.,0.866025403784439,1.,0.866025403784439,1.,0.866025403784439,
1.,0.866025403784439,1.,0.866025403784439,1.,0.866025403784439,1.,0.866025403784439,
1.,0.866025403784439,1.,0.866025403784439,1.,0.866025403784439,1.,0.866025403784439,
1.,0.866025403784439,1.,0.866025403784439,1.,0.866025403784439,1.,0.866025403784439,
1.,0.866025403784439,1.,0.866025403784439,1.,0.866025403784439,1.,0.866025403784439,
1.,0.866025403784439,1.,0.866025403784439,1.,0.866025403784439,1.,0.866025403784439,
1.,0.866025403784439,1.,0.866025403784439,1.,0.866025403784439,1.,0.866025403784439,
1.,0.866025403784439,1.,0.866025403784439,1.,0.866025403784439,1.,0.866025403784439,
1.,0.866025403784439,1.,0.866025403784439,1.,0.866025403784439,1.,0.866025403784439,
1.,0.866025403784439,1.,0.866025403784439,1.,0.866025403784439,1.,0.866025403784439,
1.,0.866025403784439,1.,0.866025403784439,1.,0.866025403784439,1.,0.866025403784439,
1.,0.866025403784439,1.,0.866025403784439,1.,0.866025403784439,1.,0.866025403784439,
1.,0.866025403784439,1.,0.866025403784439,1.,0.866025403784439,1.,0.866025403784439,
1.,0.866025403784439,1.,0.866025403784439,1.,0.866025403784439,1.,0.866025403784439,
1.,0.866025403784439,1.,0.866025403784439,1.,0.866025403784439,1.,0.866025403784439,
1.,0.866025403784439,1.,0.866025403784439,1.,0.866025403784439,1.,0.866025403784439,
1.,0.866025403784439,1.,0.866025403784439,1.,0.866025403784439,1.,0.866025403784439,
1.,0.866025403784439,1.,0.866025403784439,1.,0.866025403784439,1.,0.866025403784439,
1.,0.866025403784439,1.,0.866025403784439,1.,0.866025403784439,1.,0.866025403784439,
1.,0.866025403784439,1.,0.866025403784439,1.,0.866025403784439,1.,0.866025403784439,
1.,0.866025403784439,1.,0.866025403784439,1.,0.866025403784439,1.,0.866025403784439,
1.,0.866025403784439,1.,0.866025403784439,1.,0.866025403784439,1.,0.866025403784439,
1.,0.866025403784439,1.,0.866025403784439,1.,0.866025403784439,1.,0.866025403784439,
1.,0.866025403784439,1.,0.866025403784439,1.,0.866025403784439,1.,0.866025403784439,
1.,0.866025403784439,1.,0.866025403784439,1.,0.866025403784439,1.,0.866025403784439,
1.,0.866025403784439,1.,0.866025403784439,1.,0.866025403784439,1.,0.866025403784439,
1.,0.866025403784439,1.,0.866025403784439,1.,0.866025403784439,1.,0.866025403784439,
1.,0.866025403784439,1.,0.866025403784439,1.,0.866025403784439,1.,0.866025403784439,
1.,0.866025403784439,1.,0.866025403784439,1.,0.866025403784439,1.,0.866025403784439,
1.,0.9461134718712,0.935574832010768)))
REPRESENTATION_ITEM('')
SURFACE()
);
#290=(
BOUNDED_SURFACE()
B_SPLINE_SURFACE(1,2,((#25044,#25045,#25046,#25047,#25048,#25049,#25050,
#25051,#25052,#25053,#25054,#25055,#25056,#25057,#25058,#25059,#25060,#25061,
#25062,#25063,#25064,#25065,#25066,#25067,#25068,#25069,#25070,#25071,#25072,
#25073,#25074,#25075,#25076,#25077,#25078,#25079,#25080,#25081,#25082,#25083,
#25084,#25085,#25086,#25087,#25088,#25089,#25090,#25091,#25092,#25093,#25094,
#25095,#25096,#25097,#25098,#25099,#25100,#25101,#25102,#25103,#25104,#25105,
#25106,#25107,#25108,#25109,#25110,#25111,#25112,#25113,#25114,#25115,#25116,
#25117,#25118,#25119,#25120,#25121,#25122,#25123,#25124,#25125,#25126,#25127,
#25128,#25129,#25130,#25131,#25132,#25133,#25134,#25135,#25136,#25137,#25138,
#25139,#25140,#25141,#25142,#25143,#25144,#25145,#25146,#25147,#25148,#25149,
#25150,#25151,#25152,#25153,#25154,#25155,#25156,#25157,#25158,#25159,#25160,
#25161,#25162,#25163,#25164,#25165,#25166,#25167,#25168,#25169,#25170,#25171,
#25172,#25173,#25174,#25175,#25176,#25177,#25178,#25179,#25180,#25181,#25182,
#25183,#25184,#25185,#25186,#25187,#25188,#25189,#25190,#25191,#25192,#25193,
#25194,#25195,#25196,#25197,#25198,#25199,#25200,#25201,#25202,#25203,#25204,
#25205,#25206,#25207,#25208,#25209,#25210,#25211,#25212,#25213,#25214,#25215,
#25216,#25217,#25218,#25219,#25220,#25221,#25222,#25223,#25224,#25225,#25226,
#25227,#25228,#25229,#25230,#25231,#25232,#25233,#25234,#25235,#25236,#25237,
#25238,#25239,#25240,#25241,#25242,#25243,#25244,#25245,#25246,#25247,#25248,
#25249,#25250,#25251,#25252,#25253,#25254,#25255,#25256,#25257,#25258,#25259,
#25260,#25261,#25262,#25263,#25264,#25265,#25266,#25267,#25268,#25269,#25270,
#25271,#25272,#25273,#25274,#25275,#25276,#25277,#25278,#25279,#25280,#25281,
#25282,#25283,#25284,#25285,#25286,#25287,#25288,#25289,#25290,#25291,#25292,
#25293,#25294,#25295,#25296,#25297,#25298,#25299,#25300,#25301,#25302,#25303,
#25304,#25305,#25306,#25307,#25308,#25309,#25310,#25311,#25312,#25313,#25314,
#25315,#25316,#25317,#25318,#25319,#25320,#25321,#25322,#25323,#25324,#25325,
#25326,#25327,#25328,#25329,#25330,#25331,#25332,#25333,#25334,#25335,#25336,
#25337,#25338,#25339,#25340,#25341,#25342,#25343,#25344,#25345,#25346,#25347,
#25348,#25349,#25350,#25351,#25352,#25353,#25354,#25355,#25356,#25357,#25358,
#25359,#25360,#25361,#25362),(#25363,#25364,#25365,#25366,#25367,#25368,
#25369,#25370,#25371,#25372,#25373,#25374,#25375,#25376,#25377,#25378,#25379,
#25380,#25381,#25382,#25383,#25384,#25385,#25386,#25387,#25388,#25389,#25390,
#25391,#25392,#25393,#25394,#25395,#25396,#25397,#25398,#25399,#25400,#25401,
#25402,#25403,#25404,#25405,#25406,#25407,#25408,#25409,#25410,#25411,#25412,
#25413,#25414,#25415,#25416,#25417,#25418,#25419,#25420,#25421,#25422,#25423,
#25424,#25425,#25426,#25427,#25428,#25429,#25430,#25431,#25432,#25433,#25434,
#25435,#25436,#25437,#25438,#25439,#25440,#25441,#25442,#25443,#25444,#25445,
#25446,#25447,#25448,#25449,#25450,#25451,#25452,#25453,#25454,#25455,#25456,
#25457,#25458,#25459,#25460,#25461,#25462,#25463,#25464,#25465,#25466,#25467,
#25468,#25469,#25470,#25471,#25472,#25473,#25474,#25475,#25476,#25477,#25478,
#25479,#25480,#25481,#25482,#25483,#25484,#25485,#25486,#25487,#25488,#25489,
#25490,#25491,#25492,#25493,#25494,#25495,#25496,#25497,#25498,#25499,#25500,
#25501,#25502,#25503,#25504,#25505,#25506,#25507,#25508,#25509,#25510,#25511,
#25512,#25513,#25514,#25515,#25516,#25517,#25518,#25519,#25520,#25521,#25522,
#25523,#25524,#25525,#25526,#25527,#25528,#25529,#25530,#25531,#25532,#25533,
#25534,#25535,#25536,#25537,#25538,#25539,#25540,#25541,#25542,#25543,#25544,
#25545,#25546,#25547,#25548,#25549,#25550,#25551,#25552,#25553,#25554,#25555,
#25556,#25557,#25558,#25559,#25560,#25561,#25562,#25563,#25564,#25565,#25566,
#25567,#25568,#25569,#25570,#25571,#25572,#25573,#25574,#25575,#25576,#25577,
#25578,#25579,#25580,#25581,#25582,#25583,#25584,#25585,#25586,#25587,#25588,
#25589,#25590,#25591,#25592,#25593,#25594,#25595,#25596,#25597,#25598,#25599,
#25600,#25601,#25602,#25603,#25604,#25605,#25606,#25607,#25608,#25609,#25610,
#25611,#25612,#25613,#25614,#25615,#25616,#25617,#25618,#25619,#25620,#25621,
#25622,#25623,#25624,#25625,#25626,#25627,#25628,#25629,#25630,#25631,#25632,
#25633,#25634,#25635,#25636,#25637,#25638,#25639,#25640,#25641,#25642,#25643,
#25644,#25645,#25646,#25647,#25648,#25649,#25650,#25651,#25652,#25653,#25654,
#25655,#25656,#25657,#25658,#25659,#25660,#25661,#25662,#25663,#25664,#25665,
#25666,#25667,#25668,#25669,#25670,#25671,#25672,#25673,#25674,#25675,#25676,
#25677,#25678,#25679,#25680,#25681)),.UNSPECIFIED.,.F.,.F.,.F.)
B_SPLINE_SURFACE_WITH_KNOTS((2,2),(3,2,2,2,2,2,2,2,2,2,2,2,2,2,2,2,2,2,
2,2,2,2,2,2,2,2,2,2,2,2,2,2,2,2,2,2,2,2,2,2,2,2,2,2,2,2,2,2,2,2,2,2,2,2,
2,2,2,2,2,2,2,2,2,2,2,2,2,2,2,2,2,2,2,2,2,2,2,2,2,2,2,2,2,2,2,2,2,2,2,2,
2,2,2,2,2,2,2,2,2,2,2,2,2,2,2,2,2,2,2,2,2,2,2,2,2,2,2,2,2,2,2,2,2,2,2,2,
2,2,2,2,2,2,2,2,2,2,2,2,2,2,2,2,2,2,2,2,2,2,2,2,2,2,2,2,2,2,2,2,2,3),(0.,
1.),(0.,0.00617283950617284,0.0123456790123457,0.0185185185185185,0.0246913580246914,
0.0308641975308642,0.037037037037037,0.0432098765432099,0.0493827160493827,
0.0555555555555556,0.0617283950617284,0.0679012345679012,0.0740740740740741,
0.0802469135802469,0.0864197530864197,0.0925925925925926,0.0987654320987654,
0.104938271604938,0.111111111111111,0.117283950617284,0.123456790123457,
0.12962962962963,0.135802469135802,0.141975308641975,0.148148148148148,
0.154320987654321,0.160493827160494,0.166666666666667,0.172839506172839,
0.179012345679012,0.185185185185185,0.191358024691358,0.197530864197531,
0.203703703703704,0.209876543209877,0.216049382716049,0.222222222222222,
0.228395061728395,0.234567901234568,0.240740740740741,0.246913580246914,
0.253086419753086,0.259259259259259,0.265432098765432,0.271604938271605,
0.277777777777778,0.283950617283951,0.290123456790123,0.296296296296296,
0.302469135802469,0.308641975308642,0.314814814814815,0.320987654320988,
0.327160493827161,0.333333333333333,0.339506172839506,0.345679012345679,
0.351851851851852,0.358024691358025,0.364197530864198,0.37037037037037,
0.376543209876543,0.382716049382716,0.388888888888889,0.395061728395062,
0.401234567901235,0.407407407407407,0.41358024691358,0.419753086419753,
0.425925925925926,0.432098765432099,0.438271604938272,0.444444444444444,
0.450617283950617,0.45679012345679,0.462962962962963,0.469135802469136,
0.475308641975309,0.481481481481481,0.487654320987654,0.493827160493827,
0.5,0.506172839506173,0.512345679012346,0.518518518518518,0.524691358024691,
0.530864197530864,0.537037037037037,0.54320987654321,0.549382716049383,
0.555555555555556,0.561728395061728,0.567901234567901,0.574074074074074,
0.580246913580247,0.58641975308642,0.592592592592593,0.598765432098765,
0.604938271604938,0.611111111111111,0.617283950617284,0.623456790123457,
0.62962962962963,0.635802469135803,0.641975308641975,0.648148148148148,
0.654320987654321,0.660493827160494,0.666666666666667,0.672839506172839,
0.679012345679012,0.685185185185185,0.691358024691358,0.697530864197531,
0.703703703703704,0.709876543209877,0.716049382716049,0.722222222222222,
0.728395061728395,0.734567901234568,0.740740740740741,0.746913580246914,
0.753086419753086,0.759259259259259,0.765432098765432,0.771604938271605,
0.777777777777778,0.783950617283951,0.790123456790123,0.796296296296296,
0.802469135802469,0.808641975308642,0.814814814814815,0.820987654320988,
0.827160493827161,0.833333333333333,0.839506172839506,0.845679012345679,
0.851851851851852,0.858024691358025,0.864197530864197,0.87037037037037,
0.876543209876543,0.882716049382716,0.888888888888889,0.895061728395062,
0.901234567901235,0.907407407407407,0.91358024691358,0.919753086419753,
0.925925925925926,0.932098765432099,0.938271604938272,0.944444444444444,
0.950617283950617,0.95679012345679,0.962962962962963,0.969135802469136,
0.975308641975309,0.977791440774828),.UNSPECIFIED.)
GEOMETRIC_REPRESENTATION_ITEM()
RATIONAL_B_SPLINE_SURFACE(((1.,0.866025403784439,1.,0.866025403784439,1.,
0.866025403784439,1.,0.866025403784439,1.,0.866025403784439,1.,0.866025403784439,
1.,0.866025403784439,1.,0.866025403784439,1.,0.866025403784439,1.,0.866025403784439,
1.,0.866025403784439,1.,0.866025403784439,1.,0.866025403784439,1.,0.866025403784439,
1.,0.866025403784439,1.,0.866025403784439,1.,0.866025403784439,1.,0.866025403784439,
1.,0.866025403784439,1.,0.866025403784439,1.,0.866025403784439,1.,0.866025403784439,
1.,0.866025403784439,1.,0.866025403784439,1.,0.866025403784439,1.,0.866025403784439,
1.,0.866025403784439,1.,0.866025403784439,1.,0.866025403784439,1.,0.866025403784439,
1.,0.866025403784439,1.,0.866025403784439,1.,0.866025403784439,1.,0.866025403784439,
1.,0.866025403784439,1.,0.866025403784439,1.,0.866025403784439,1.,0.866025403784439,
1.,0.866025403784439,1.,0.866025403784439,1.,0.866025403784439,1.,0.866025403784439,
1.,0.866025403784439,1.,0.866025403784439,1.,0.866025403784439,1.,0.866025403784439,
1.,0.866025403784439,1.,0.866025403784439,1.,0.866025403784439,1.,0.866025403784439,
1.,0.866025403784439,1.,0.866025403784439,1.,0.866025403784439,1.,0.866025403784439,
1.,0.866025403784439,1.,0.866025403784439,1.,0.866025403784439,1.,0.866025403784439,
1.,0.866025403784439,1.,0.866025403784439,1.,0.866025403784439,1.,0.866025403784439,
1.,0.866025403784439,1.,0.866025403784439,1.,0.866025403784439,1.,0.866025403784439,
1.,0.866025403784439,1.,0.866025403784439,1.,0.866025403784439,1.,0.866025403784439,
1.,0.866025403784439,1.,0.866025403784439,1.,0.866025403784439,1.,0.866025403784439,
1.,0.866025403784439,1.,0.866025403784439,1.,0.866025403784439,1.,0.866025403784439,
1.,0.866025403784439,1.,0.866025403784439,1.,0.866025403784439,1.,0.866025403784439,
1.,0.866025403784439,1.,0.866025403784439,1.,0.866025403784439,1.,0.866025403784439,
1.,0.866025403784439,1.,0.866025403784439,1.,0.866025403784439,1.,0.866025403784439,
1.,0.866025403784439,1.,0.866025403784439,1.,0.866025403784439,1.,0.866025403784439,
1.,0.866025403784439,1.,0.866025403784439,1.,0.866025403784439,1.,0.866025403784439,
1.,0.866025403784439,1.,0.866025403784439,1.,0.866025403784439,1.,0.866025403784439,
1.,0.866025403784439,1.,0.866025403784439,1.,0.866025403784439,1.,0.866025403784439,
1.,0.866025403784439,1.,0.866025403784439,1.,0.866025403784439,1.,0.866025403784439,
1.,0.866025403784439,1.,0.866025403784439,1.,0.866025403784439,1.,0.866025403784439,
1.,0.866025403784439,1.,0.866025403784439,1.,0.866025403784439,1.,0.866025403784439,
1.,0.866025403784439,1.,0.866025403784439,1.,0.866025403784439,1.,0.866025403784439,
1.,0.866025403784439,1.,0.866025403784439,1.,0.866025403784439,1.,0.866025403784439,
1.,0.866025403784439,1.,0.866025403784439,1.,0.866025403784439,1.,0.866025403784439,
1.,0.866025403784439,1.,0.866025403784439,1.,0.866025403784439,1.,0.866025403784439,
1.,0.866025403784439,1.,0.866025403784439,1.,0.866025403784439,1.,0.866025403784439,
1.,0.866025403784439,1.,0.866025403784439,1.,0.866025403784439,1.,0.866025403784439,
1.,0.866025403784439,1.,0.866025403784439,1.,0.866025403784439,1.,0.866025403784439,
1.,0.866025403784439,1.,0.866025403784439,1.,0.866025403784439,1.,0.866025403784439,
1.,0.866025403784439,1.,0.866025403784439,1.,0.866025403784439,1.,0.866025403784439,
1.,0.866025403784439,1.,0.866025403784439,1.,0.866025403784439,1.,0.866025403784439,
1.,0.946113621402695,0.935574890499137),(1.,0.866025403784439,1.,0.866025403784439,
1.,0.866025403784439,1.,0.866025403784439,1.,0.866025403784439,1.,0.866025403784439,
1.,0.866025403784439,1.,0.866025403784439,1.,0.866025403784439,1.,0.866025403784439,
1.,0.866025403784439,1.,0.866025403784439,1.,0.866025403784439,1.,0.866025403784439,
1.,0.866025403784439,1.,0.866025403784439,1.,0.866025403784439,1.,0.866025403784439,
1.,0.866025403784439,1.,0.866025403784439,1.,0.866025403784439,1.,0.866025403784439,
1.,0.866025403784439,1.,0.866025403784439,1.,0.866025403784439,1.,0.866025403784439,
1.,0.866025403784439,1.,0.866025403784439,1.,0.866025403784439,1.,0.866025403784439,
1.,0.866025403784439,1.,0.866025403784439,1.,0.866025403784439,1.,0.866025403784439,
1.,0.866025403784439,1.,0.866025403784439,1.,0.866025403784439,1.,0.866025403784439,
1.,0.866025403784439,1.,0.866025403784439,1.,0.866025403784439,1.,0.866025403784439,
1.,0.866025403784439,1.,0.866025403784439,1.,0.866025403784439,1.,0.866025403784439,
1.,0.866025403784439,1.,0.866025403784439,1.,0.866025403784439,1.,0.866025403784439,
1.,0.866025403784439,1.,0.866025403784439,1.,0.866025403784439,1.,0.866025403784439,
1.,0.866025403784439,1.,0.866025403784439,1.,0.866025403784439,1.,0.866025403784439,
1.,0.866025403784439,1.,0.866025403784439,1.,0.866025403784439,1.,0.866025403784439,
1.,0.866025403784439,1.,0.866025403784439,1.,0.866025403784439,1.,0.866025403784439,
1.,0.866025403784439,1.,0.866025403784439,1.,0.866025403784439,1.,0.866025403784439,
1.,0.866025403784439,1.,0.866025403784439,1.,0.866025403784439,1.,0.866025403784439,
1.,0.866025403784439,1.,0.866025403784439,1.,0.866025403784439,1.,0.866025403784439,
1.,0.866025403784439,1.,0.866025403784439,1.,0.866025403784439,1.,0.866025403784439,
1.,0.866025403784439,1.,0.866025403784439,1.,0.866025403784439,1.,0.866025403784439,
1.,0.866025403784439,1.,0.866025403784439,1.,0.866025403784439,1.,0.866025403784439,
1.,0.866025403784439,1.,0.866025403784439,1.,0.866025403784439,1.,0.866025403784439,
1.,0.866025403784439,1.,0.866025403784439,1.,0.866025403784439,1.,0.866025403784439,
1.,0.866025403784439,1.,0.866025403784439,1.,0.866025403784439,1.,0.866025403784439,
1.,0.866025403784439,1.,0.866025403784439,1.,0.866025403784439,1.,0.866025403784439,
1.,0.866025403784439,1.,0.866025403784439,1.,0.866025403784439,1.,0.866025403784439,
1.,0.866025403784439,1.,0.866025403784439,1.,0.866025403784439,1.,0.866025403784439,
1.,0.866025403784439,1.,0.866025403784439,1.,0.866025403784439,1.,0.866025403784439,
1.,0.866025403784439,1.,0.866025403784439,1.,0.866025403784439,1.,0.866025403784439,
1.,0.866025403784439,1.,0.866025403784439,1.,0.866025403784439,1.,0.866025403784439,
1.,0.866025403784439,1.,0.866025403784439,1.,0.866025403784439,1.,0.866025403784439,
1.,0.866025403784439,1.,0.866025403784439,1.,0.866025403784439,1.,0.866025403784439,
1.,0.866025403784439,1.,0.866025403784439,1.,0.866025403784439,1.,0.866025403784439,
1.,0.866025403784439,1.,0.866025403784439,1.,0.866025403784439,1.,0.866025403784439,
1.,0.866025403784439,1.,0.866025403784439,1.,0.866025403784439,1.,0.866025403784439,
1.,0.866025403784439,1.,0.866025403784439,1.,0.866025403784439,1.,0.866025403784439,
1.,0.866025403784439,1.,0.866025403784439,1.,0.866025403784439,1.,0.866025403784439,
1.,0.866025403784439,1.,0.866025403784439,1.,0.866025403784439,1.,0.866025403784439,
1.,0.946113621402695,0.935574890499137)))
REPRESENTATION_ITEM('')
SURFACE()
);
#291=(
BOUNDED_SURFACE()
B_SPLINE_SURFACE(1,2,((#25988,#25989,#25990,#25991,#25992,#25993,#25994,
#25995,#25996,#25997,#25998,#25999,#26000,#26001,#26002,#26003,#26004,#26005,
#26006,#26007,#26008,#26009,#26010,#26011,#26012,#26013,#26014,#26015,#26016,
#26017,#26018,#26019,#26020,#26021,#26022,#26023,#26024,#26025,#26026,#26027,
#26028,#26029,#26030,#26031,#26032,#26033,#26034,#26035,#26036,#26037,#26038,
#26039,#26040,#26041,#26042,#26043,#26044,#26045,#26046,#26047,#26048,#26049,
#26050,#26051,#26052,#26053,#26054,#26055,#26056,#26057,#26058,#26059,#26060,
#26061,#26062,#26063,#26064,#26065,#26066,#26067,#26068,#26069,#26070,#26071,
#26072,#26073,#26074,#26075,#26076,#26077,#26078,#26079,#26080,#26081,#26082,
#26083,#26084,#26085,#26086,#26087,#26088,#26089,#26090,#26091,#26092,#26093,
#26094,#26095,#26096,#26097,#26098,#26099,#26100,#26101,#26102,#26103,#26104,
#26105,#26106,#26107,#26108,#26109,#26110,#26111,#26112,#26113,#26114,#26115,
#26116,#26117,#26118,#26119,#26120,#26121,#26122,#26123,#26124,#26125,#26126,
#26127,#26128,#26129,#26130,#26131,#26132,#26133,#26134,#26135,#26136,#26137,
#26138,#26139,#26140,#26141,#26142,#26143,#26144,#26145,#26146,#26147,#26148,
#26149,#26150,#26151,#26152,#26153,#26154,#26155,#26156,#26157,#26158,#26159,
#26160,#26161,#26162,#26163,#26164,#26165,#26166,#26167,#26168,#26169,#26170,
#26171,#26172,#26173,#26174,#26175,#26176,#26177,#26178,#26179,#26180,#26181,
#26182,#26183,#26184,#26185,#26186,#26187,#26188,#26189,#26190,#26191,#26192,
#26193,#26194,#26195,#26196,#26197,#26198,#26199,#26200,#26201,#26202,#26203,
#26204,#26205,#26206,#26207,#26208,#26209,#26210,#26211,#26212,#26213,#26214,
#26215,#26216,#26217,#26218,#26219,#26220,#26221,#26222,#26223,#26224,#26225,
#26226,#26227,#26228,#26229,#26230,#26231,#26232,#26233,#26234,#26235,#26236,
#26237,#26238,#26239,#26240,#26241,#26242,#26243,#26244,#26245,#26246,#26247,
#26248,#26249,#26250,#26251,#26252,#26253,#26254,#26255,#26256,#26257,#26258,
#26259,#26260,#26261,#26262,#26263,#26264,#26265,#26266,#26267,#26268,#26269,
#26270,#26271,#26272,#26273,#26274,#26275,#26276,#26277,#26278,#26279,#26280,
#26281,#26282,#26283,#26284,#26285,#26286,#26287,#26288,#26289,#26290,#26291,
#26292,#26293,#26294,#26295,#26296,#26297,#26298,#26299,#26300,#26301,#26302,
#26303,#26304,#26305,#26306,#26307,#26308),(#26309,#26310,#26311,#26312,
#26313,#26314,#26315,#26316,#26317,#26318,#26319,#26320,#26321,#26322,#26323,
#26324,#26325,#26326,#26327,#26328,#26329,#26330,#26331,#26332,#26333,#26334,
#26335,#26336,#26337,#26338,#26339,#26340,#26341,#26342,#26343,#26344,#26345,
#26346,#26347,#26348,#26349,#26350,#26351,#26352,#26353,#26354,#26355,#26356,
#26357,#26358,#26359,#26360,#26361,#26362,#26363,#26364,#26365,#26366,#26367,
#26368,#26369,#26370,#26371,#26372,#26373,#26374,#26375,#26376,#26377,#26378,
#26379,#26380,#26381,#26382,#26383,#26384,#26385,#26386,#26387,#26388,#26389,
#26390,#26391,#26392,#26393,#26394,#26395,#26396,#26397,#26398,#26399,#26400,
#26401,#26402,#26403,#26404,#26405,#26406,#26407,#26408,#26409,#26410,#26411,
#26412,#26413,#26414,#26415,#26416,#26417,#26418,#26419,#26420,#26421,#26422,
#26423,#26424,#26425,#26426,#26427,#26428,#26429,#26430,#26431,#26432,#26433,
#26434,#26435,#26436,#26437,#26438,#26439,#26440,#26441,#26442,#26443,#26444,
#26445,#26446,#26447,#26448,#26449,#26450,#26451,#26452,#26453,#26454,#26455,
#26456,#26457,#26458,#26459,#26460,#26461,#26462,#26463,#26464,#26465,#26466,
#26467,#26468,#26469,#26470,#26471,#26472,#26473,#26474,#26475,#26476,#26477,
#26478,#26479,#26480,#26481,#26482,#26483,#26484,#26485,#26486,#26487,#26488,
#26489,#26490,#26491,#26492,#26493,#26494,#26495,#26496,#26497,#26498,#26499,
#26500,#26501,#26502,#26503,#26504,#26505,#26506,#26507,#26508,#26509,#26510,
#26511,#26512,#26513,#26514,#26515,#26516,#26517,#26518,#26519,#26520,#26521,
#26522,#26523,#26524,#26525,#26526,#26527,#26528,#26529,#26530,#26531,#26532,
#26533,#26534,#26535,#26536,#26537,#26538,#26539,#26540,#26541,#26542,#26543,
#26544,#26545,#26546,#26547,#26548,#26549,#26550,#26551,#26552,#26553,#26554,
#26555,#26556,#26557,#26558,#26559,#26560,#26561,#26562,#26563,#26564,#26565,
#26566,#26567,#26568,#26569,#26570,#26571,#26572,#26573,#26574,#26575,#26576,
#26577,#26578,#26579,#26580,#26581,#26582,#26583,#26584,#26585,#26586,#26587,
#26588,#26589,#26590,#26591,#26592,#26593,#26594,#26595,#26596,#26597,#26598,
#26599,#26600,#26601,#26602,#26603,#26604,#26605,#26606,#26607,#26608,#26609,
#26610,#26611,#26612,#26613,#26614,#26615,#26616,#26617,#26618,#26619,#26620,
#26621,#26622,#26623,#26624,#26625,#26626,#26627,#26628,#26629)),
 .UNSPECIFIED.,.F.,.F.,.F.)
B_SPLINE_SURFACE_WITH_KNOTS((2,2),(3,2,2,2,2,2,2,2,2,2,2,2,2,2,2,2,2,2,
2,2,2,2,2,2,2,2,2,2,2,2,2,2,2,2,2,2,2,2,2,2,2,2,2,2,2,2,2,2,2,2,2,2,2,2,
2,2,2,2,2,2,2,2,2,2,2,2,2,2,2,2,2,2,2,2,2,2,2,2,2,2,2,2,2,2,2,2,2,2,2,2,
2,2,2,2,2,2,2,2,2,2,2,2,2,2,2,2,2,2,2,2,2,2,2,2,2,2,2,2,2,2,2,2,2,2,2,2,
2,2,2,2,2,2,2,2,2,2,2,2,2,2,2,2,2,2,2,2,2,2,2,2,2,2,2,2,2,2,2,2,2,2,3),
(-0.000321975171232605,1.),(0.,0.00617283950617284,0.0123456790123457,0.0185185185185185,
0.0246913580246914,0.0308641975308642,0.037037037037037,0.0432098765432099,
0.0493827160493827,0.0555555555555556,0.0617283950617284,0.0679012345679012,
0.0740740740740741,0.0802469135802469,0.0864197530864197,0.0925925925925926,
0.0987654320987654,0.104938271604938,0.111111111111111,0.117283950617284,
0.123456790123457,0.12962962962963,0.135802469135802,0.141975308641975,
0.148148148148148,0.154320987654321,0.160493827160494,0.166666666666667,
0.172839506172839,0.179012345679012,0.185185185185185,0.191358024691358,
0.197530864197531,0.203703703703704,0.209876543209877,0.216049382716049,
0.222222222222222,0.228395061728395,0.234567901234568,0.240740740740741,
0.246913580246914,0.253086419753086,0.259259259259259,0.265432098765432,
0.271604938271605,0.277777777777778,0.283950617283951,0.290123456790123,
0.296296296296296,0.302469135802469,0.308641975308642,0.314814814814815,
0.320987654320988,0.327160493827161,0.333333333333333,0.339506172839506,
0.345679012345679,0.351851851851852,0.358024691358025,0.364197530864198,
0.37037037037037,0.376543209876543,0.382716049382716,0.388888888888889,
0.395061728395062,0.401234567901235,0.407407407407407,0.41358024691358,
0.419753086419753,0.425925925925926,0.432098765432099,0.438271604938272,
0.444444444444444,0.450617283950617,0.45679012345679,0.462962962962963,
0.469135802469136,0.475308641975309,0.481481481481481,0.487654320987654,
0.493827160493827,0.5,0.506172839506173,0.512345679012346,0.518518518518518,
0.524691358024691,0.530864197530864,0.537037037037037,0.54320987654321,
0.549382716049383,0.555555555555556,0.561728395061728,0.567901234567901,
0.574074074074074,0.580246913580247,0.58641975308642,0.592592592592593,
0.598765432098765,0.604938271604938,0.611111111111111,0.617283950617284,
0.623456790123457,0.62962962962963,0.635802469135803,0.641975308641975,
0.648148148148148,0.654320987654321,0.660493827160494,0.666666666666667,
0.672839506172839,0.679012345679012,0.685185185185185,0.691358024691358,
0.697530864197531,0.703703703703704,0.709876543209877,0.716049382716049,
0.722222222222222,0.728395061728395,0.734567901234568,0.740740740740741,
0.746913580246914,0.753086419753086,0.759259259259259,0.765432098765432,
0.771604938271605,0.777777777777778,0.783950617283951,0.790123456790123,
0.796296296296296,0.802469135802469,0.808641975308642,0.814814814814815,
0.820987654320988,0.827160493827161,0.833333333333333,0.839506172839506,
0.845679012345679,0.851851851851852,0.858024691358025,0.864197530864197,
0.87037037037037,0.876543209876543,0.882716049382716,0.888888888888889,
0.895061728395062,0.901234567901235,0.907407407407407,0.91358024691358,
0.919753086419753,0.925925925925926,0.932098765432099,0.938271604938272,
0.944444444444444,0.950617283950617,0.95679012345679,0.962962962962963,
0.969135802469136,0.975308641975309,0.977791393533952,0.987569307469292),
 .UNSPECIFIED.)
GEOMETRIC_REPRESENTATION_ITEM()
RATIONAL_B_SPLINE_SURFACE(((1.,0.866025403784439,1.,0.866025403784439,1.,
0.866025403784439,1.,0.866025403784439,1.,0.866025403784439,1.,0.866025403784439,
1.,0.866025403784439,1.,0.866025403784439,1.,0.866025403784439,1.,0.866025403784439,
1.,0.866025403784439,1.,0.866025403784439,1.,0.866025403784439,1.,0.866025403784439,
1.,0.866025403784439,1.,0.866025403784439,1.,0.866025403784439,1.,0.866025403784439,
1.,0.866025403784439,1.,0.866025403784439,1.,0.866025403784439,1.,0.866025403784439,
1.,0.866025403784439,1.,0.866025403784439,1.,0.866025403784439,1.,0.866025403784439,
1.,0.866025403784439,1.,0.866025403784439,1.,0.866025403784439,1.,0.866025403784439,
1.,0.866025403784439,1.,0.866025403784439,1.,0.866025403784439,1.,0.866025403784439,
1.,0.866025403784439,1.,0.866025403784439,1.,0.866025403784439,1.,0.866025403784439,
1.,0.866025403784439,1.,0.866025403784439,1.,0.866025403784439,1.,0.866025403784439,
1.,0.866025403784439,1.,0.866025403784439,1.,0.866025403784439,1.,0.866025403784439,
1.,0.866025403784439,1.,0.866025403784439,1.,0.866025403784439,1.,0.866025403784439,
1.,0.866025403784439,1.,0.866025403784439,1.,0.866025403784439,1.,0.866025403784439,
1.,0.866025403784439,1.,0.866025403784439,1.,0.866025403784439,1.,0.866025403784439,
1.,0.866025403784439,1.,0.866025403784439,1.,0.866025403784439,1.,0.866025403784439,
1.,0.866025403784439,1.,0.866025403784439,1.,0.866025403784439,1.,0.866025403784439,
1.,0.866025403784439,1.,0.866025403784439,1.,0.866025403784439,1.,0.866025403784439,
1.,0.866025403784439,1.,0.866025403784439,1.,0.866025403784439,1.,0.866025403784439,
1.,0.866025403784439,1.,0.866025403784439,1.,0.866025403784439,1.,0.866025403784439,
1.,0.866025403784439,1.,0.866025403784439,1.,0.866025403784439,1.,0.866025403784439,
1.,0.866025403784439,1.,0.866025403784439,1.,0.866025403784439,1.,0.866025403784439,
1.,0.866025403784439,1.,0.866025403784439,1.,0.866025403784439,1.,0.866025403784439,
1.,0.866025403784439,1.,0.866025403784439,1.,0.866025403784439,1.,0.866025403784439,
1.,0.866025403784439,1.,0.866025403784439,1.,0.866025403784439,1.,0.866025403784439,
1.,0.866025403784439,1.,0.866025403784439,1.,0.866025403784439,1.,0.866025403784439,
1.,0.866025403784439,1.,0.866025403784439,1.,0.866025403784439,1.,0.866025403784439,
1.,0.866025403784439,1.,0.866025403784439,1.,0.866025403784439,1.,0.866025403784439,
1.,0.866025403784439,1.,0.866025403784439,1.,0.866025403784439,1.,0.866025403784439,
1.,0.866025403784439,1.,0.866025403784439,1.,0.866025403784439,1.,0.866025403784439,
1.,0.866025403784439,1.,0.866025403784439,1.,0.866025403784439,1.,0.866025403784439,
1.,0.866025403784439,1.,0.866025403784439,1.,0.866025403784439,1.,0.866025403784439,
1.,0.866025403784439,1.,0.866025403784439,1.,0.866025403784439,1.,0.866025403784439,
1.,0.866025403784439,1.,0.866025403784439,1.,0.866025403784439,1.,0.866025403784439,
1.,0.866025403784439,1.,0.866025403784439,1.,0.866025403784439,1.,0.866025403784439,
1.,0.866025403784439,1.,0.866025403784439,1.,0.866025403784439,1.,0.866025403784439,
1.,0.866025403784439,1.,0.866025403784439,1.,0.866025403784439,1.,0.866025403784439,
1.,0.866025403784439,1.,0.866025403784439,1.,0.866025403784439,1.,0.866025403784439,
1.,0.866025403784439,1.,0.866025403784439,1.,0.866025403784439,1.,0.866025403784439,
1.,0.866025403784439,1.,0.866025403784439,1.,0.866025403784439,1.,0.866025403784439,
1.,0.946114646713198,0.93557529156132,0.93557529156132,0.93557529156132),
(1.,0.866025403784439,1.,0.866025403784439,1.,0.866025403784439,1.,0.866025403784439,
1.,0.866025403784439,1.,0.866025403784439,1.,0.866025403784439,1.,0.866025403784439,
1.,0.866025403784439,1.,0.866025403784439,1.,0.866025403784439,1.,0.866025403784439,
1.,0.866025403784439,1.,0.866025403784439,1.,0.866025403784439,1.,0.866025403784439,
1.,0.866025403784439,1.,0.866025403784439,1.,0.866025403784439,1.,0.866025403784439,
1.,0.866025403784439,1.,0.866025403784439,1.,0.866025403784439,1.,0.866025403784439,
1.,0.866025403784439,1.,0.866025403784439,1.,0.866025403784439,1.,0.866025403784439,
1.,0.866025403784439,1.,0.866025403784439,1.,0.866025403784439,1.,0.866025403784439,
1.,0.866025403784439,1.,0.866025403784439,1.,0.866025403784439,1.,0.866025403784439,
1.,0.866025403784439,1.,0.866025403784439,1.,0.866025403784439,1.,0.866025403784439,
1.,0.866025403784439,1.,0.866025403784439,1.,0.866025403784439,1.,0.866025403784439,
1.,0.866025403784439,1.,0.866025403784439,1.,0.866025403784439,1.,0.866025403784439,
1.,0.866025403784439,1.,0.866025403784439,1.,0.866025403784439,1.,0.866025403784439,
1.,0.866025403784439,1.,0.866025403784439,1.,0.866025403784439,1.,0.866025403784439,
1.,0.866025403784439,1.,0.866025403784439,1.,0.866025403784439,1.,0.866025403784439,
1.,0.866025403784439,1.,0.866025403784439,1.,0.866025403784439,1.,0.866025403784439,
1.,0.866025403784439,1.,0.866025403784439,1.,0.866025403784439,1.,0.866025403784439,
1.,0.866025403784439,1.,0.866025403784439,1.,0.866025403784439,1.,0.866025403784439,
1.,0.866025403784439,1.,0.866025403784439,1.,0.866025403784439,1.,0.866025403784439,
1.,0.866025403784439,1.,0.866025403784439,1.,0.866025403784439,1.,0.866025403784439,
1.,0.866025403784439,1.,0.866025403784439,1.,0.866025403784439,1.,0.866025403784439,
1.,0.866025403784439,1.,0.866025403784439,1.,0.866025403784439,1.,0.866025403784439,
1.,0.866025403784439,1.,0.866025403784439,1.,0.866025403784439,1.,0.866025403784439,
1.,0.866025403784439,1.,0.866025403784439,1.,0.866025403784439,1.,0.866025403784439,
1.,0.866025403784439,1.,0.866025403784439,1.,0.866025403784439,1.,0.866025403784439,
1.,0.866025403784439,1.,0.866025403784439,1.,0.866025403784439,1.,0.866025403784439,
1.,0.866025403784439,1.,0.866025403784439,1.,0.866025403784439,1.,0.866025403784439,
1.,0.866025403784439,1.,0.866025403784439,1.,0.866025403784439,1.,0.866025403784439,
1.,0.866025403784439,1.,0.866025403784439,1.,0.866025403784439,1.,0.866025403784439,
1.,0.866025403784439,1.,0.866025403784439,1.,0.866025403784439,1.,0.866025403784439,
1.,0.866025403784439,1.,0.866025403784439,1.,0.866025403784439,1.,0.866025403784439,
1.,0.866025403784439,1.,0.866025403784439,1.,0.866025403784439,1.,0.866025403784439,
1.,0.866025403784439,1.,0.866025403784439,1.,0.866025403784439,1.,0.866025403784439,
1.,0.866025403784439,1.,0.866025403784439,1.,0.866025403784439,1.,0.866025403784439,
1.,0.866025403784439,1.,0.866025403784439,1.,0.866025403784439,1.,0.866025403784439,
1.,0.866025403784439,1.,0.866025403784439,1.,0.866025403784439,1.,0.866025403784439,
1.,0.866025403784439,1.,0.866025403784439,1.,0.866025403784439,1.,0.866025403784439,
1.,0.866025403784439,1.,0.866025403784439,1.,0.866025403784439,1.,0.866025403784439,
1.,0.866025403784439,1.,0.866025403784439,1.,0.866025403784439,1.,0.866025403784439,
1.,0.866025403784439,1.,0.866025403784439,1.,0.946114646713198,0.93557529156132,
0.93557529156132,0.93557529156132)))
REPRESENTATION_ITEM('')
SURFACE()
);
#292=(
BOUNDED_SURFACE()
B_SPLINE_SURFACE(1,2,((#26653,#26654,#26655,#26656,#26657,#26658,#26659,
#26660,#26661,#26662,#26663,#26664,#26665,#26666,#26667,#26668,#26669,#26670,
#26671,#26672,#26673,#26674,#26675,#26676,#26677,#26678,#26679,#26680,#26681,
#26682,#26683,#26684,#26685,#26686,#26687,#26688,#26689,#26690,#26691,#26692,
#26693,#26694,#26695,#26696,#26697,#26698,#26699,#26700,#26701,#26702,#26703,
#26704,#26705,#26706,#26707,#26708,#26709,#26710,#26711,#26712,#26713,#26714,
#26715,#26716,#26717,#26718,#26719,#26720,#26721,#26722,#26723,#26724,#26725,
#26726,#26727,#26728,#26729,#26730,#26731,#26732,#26733,#26734,#26735,#26736,
#26737,#26738,#26739,#26740,#26741,#26742,#26743,#26744,#26745,#26746,#26747,
#26748,#26749,#26750,#26751,#26752,#26753,#26754,#26755,#26756,#26757,#26758,
#26759,#26760,#26761,#26762,#26763,#26764,#26765,#26766,#26767,#26768,#26769,
#26770,#26771,#26772,#26773,#26774,#26775,#26776,#26777,#26778,#26779,#26780,
#26781,#26782,#26783,#26784,#26785,#26786,#26787,#26788,#26789,#26790,#26791,
#26792,#26793,#26794,#26795,#26796,#26797,#26798,#26799,#26800,#26801,#26802,
#26803,#26804,#26805,#26806,#26807,#26808,#26809,#26810,#26811,#26812,#26813,
#26814,#26815,#26816,#26817,#26818,#26819,#26820,#26821,#26822,#26823,#26824,
#26825,#26826,#26827,#26828,#26829,#26830,#26831,#26832,#26833,#26834,#26835,
#26836,#26837,#26838,#26839,#26840,#26841,#26842,#26843,#26844,#26845,#26846,
#26847,#26848,#26849,#26850,#26851,#26852,#26853,#26854,#26855,#26856,#26857,
#26858,#26859,#26860,#26861,#26862,#26863,#26864,#26865,#26866,#26867,#26868,
#26869,#26870,#26871,#26872,#26873,#26874,#26875,#26876,#26877,#26878,#26879,
#26880,#26881,#26882,#26883,#26884,#26885,#26886,#26887,#26888,#26889,#26890,
#26891,#26892,#26893,#26894,#26895,#26896,#26897,#26898,#26899,#26900,#26901,
#26902,#26903,#26904,#26905,#26906,#26907,#26908,#26909,#26910,#26911,#26912,
#26913,#26914,#26915,#26916,#26917,#26918,#26919,#26920,#26921,#26922,#26923,
#26924,#26925,#26926,#26927,#26928,#26929,#26930,#26931,#26932,#26933,#26934,
#26935,#26936,#26937,#26938,#26939,#26940,#26941,#26942,#26943,#26944,#26945,
#26946,#26947,#26948,#26949,#26950,#26951,#26952,#26953,#26954,#26955,#26956,
#26957,#26958,#26959,#26960,#26961,#26962,#26963,#26964,#26965,#26966,#26967,
#26968,#26969,#26970,#26971),(#26972,#26973,#26974,#26975,#26976,#26977,
#26978,#26979,#26980,#26981,#26982,#26983,#26984,#26985,#26986,#26987,#26988,
#26989,#26990,#26991,#26992,#26993,#26994,#26995,#26996,#26997,#26998,#26999,
#27000,#27001,#27002,#27003,#27004,#27005,#27006,#27007,#27008,#27009,#27010,
#27011,#27012,#27013,#27014,#27015,#27016,#27017,#27018,#27019,#27020,#27021,
#27022,#27023,#27024,#27025,#27026,#27027,#27028,#27029,#27030,#27031,#27032,
#27033,#27034,#27035,#27036,#27037,#27038,#27039,#27040,#27041,#27042,#27043,
#27044,#27045,#27046,#27047,#27048,#27049,#27050,#27051,#27052,#27053,#27054,
#27055,#27056,#27057,#27058,#27059,#27060,#27061,#27062,#27063,#27064,#27065,
#27066,#27067,#27068,#27069,#27070,#27071,#27072,#27073,#27074,#27075,#27076,
#27077,#27078,#27079,#27080,#27081,#27082,#27083,#27084,#27085,#27086,#27087,
#27088,#27089,#27090,#27091,#27092,#27093,#27094,#27095,#27096,#27097,#27098,
#27099,#27100,#27101,#27102,#27103,#27104,#27105,#27106,#27107,#27108,#27109,
#27110,#27111,#27112,#27113,#27114,#27115,#27116,#27117,#27118,#27119,#27120,
#27121,#27122,#27123,#27124,#27125,#27126,#27127,#27128,#27129,#27130,#27131,
#27132,#27133,#27134,#27135,#27136,#27137,#27138,#27139,#27140,#27141,#27142,
#27143,#27144,#27145,#27146,#27147,#27148,#27149,#27150,#27151,#27152,#27153,
#27154,#27155,#27156,#27157,#27158,#27159,#27160,#27161,#27162,#27163,#27164,
#27165,#27166,#27167,#27168,#27169,#27170,#27171,#27172,#27173,#27174,#27175,
#27176,#27177,#27178,#27179,#27180,#27181,#27182,#27183,#27184,#27185,#27186,
#27187,#27188,#27189,#27190,#27191,#27192,#27193,#27194,#27195,#27196,#27197,
#27198,#27199,#27200,#27201,#27202,#27203,#27204,#27205,#27206,#27207,#27208,
#27209,#27210,#27211,#27212,#27213,#27214,#27215,#27216,#27217,#27218,#27219,
#27220,#27221,#27222,#27223,#27224,#27225,#27226,#27227,#27228,#27229,#27230,
#27231,#27232,#27233,#27234,#27235,#27236,#27237,#27238,#27239,#27240,#27241,
#27242,#27243,#27244,#27245,#27246,#27247,#27248,#27249,#27250,#27251,#27252,
#27253,#27254,#27255,#27256,#27257,#27258,#27259,#27260,#27261,#27262,#27263,
#27264,#27265,#27266,#27267,#27268,#27269,#27270,#27271,#27272,#27273,#27274,
#27275,#27276,#27277,#27278,#27279,#27280,#27281,#27282,#27283,#27284,#27285,
#27286,#27287,#27288,#27289,#27290)),.UNSPECIFIED.,.F.,.F.,.F.)
B_SPLINE_SURFACE_WITH_KNOTS((2,2),(3,2,2,2,2,2,2,2,2,2,2,2,2,2,2,2,2,2,
2,2,2,2,2,2,2,2,2,2,2,2,2,2,2,2,2,2,2,2,2,2,2,2,2,2,2,2,2,2,2,2,2,2,2,2,
2,2,2,2,2,2,2,2,2,2,2,2,2,2,2,2,2,2,2,2,2,2,2,2,2,2,2,2,2,2,2,2,2,2,2,2,
2,2,2,2,2,2,2,2,2,2,2,2,2,2,2,2,2,2,2,2,2,2,2,2,2,2,2,2,2,2,2,2,2,2,2,2,
2,2,2,2,2,2,2,2,2,2,2,2,2,2,2,2,2,2,2,2,2,2,2,2,2,2,2,2,2,2,2,2,2,3),(-2.47338691325004E-5,
1.),(0.,0.00617283950617284,0.0123456790123457,0.0185185185185185,0.0246913580246914,
0.0308641975308642,0.037037037037037,0.0432098765432099,0.0493827160493827,
0.0555555555555556,0.0617283950617284,0.0679012345679012,0.0740740740740741,
0.0802469135802469,0.0864197530864197,0.0925925925925926,0.0987654320987654,
0.104938271604938,0.111111111111111,0.117283950617284,0.123456790123457,
0.12962962962963,0.135802469135802,0.141975308641975,0.148148148148148,
0.154320987654321,0.160493827160494,0.166666666666667,0.172839506172839,
0.179012345679012,0.185185185185185,0.191358024691358,0.197530864197531,
0.203703703703704,0.209876543209877,0.216049382716049,0.222222222222222,
0.228395061728395,0.234567901234568,0.240740740740741,0.246913580246914,
0.253086419753086,0.259259259259259,0.265432098765432,0.271604938271605,
0.277777777777778,0.283950617283951,0.290123456790123,0.296296296296296,
0.302469135802469,0.308641975308642,0.314814814814815,0.320987654320988,
0.327160493827161,0.333333333333333,0.339506172839506,0.345679012345679,
0.351851851851852,0.358024691358025,0.364197530864198,0.37037037037037,
0.376543209876543,0.382716049382716,0.388888888888889,0.395061728395062,
0.401234567901235,0.407407407407407,0.41358024691358,0.419753086419753,
0.425925925925926,0.432098765432099,0.438271604938272,0.444444444444444,
0.450617283950617,0.45679012345679,0.462962962962963,0.469135802469136,
0.475308641975309,0.481481481481481,0.487654320987654,0.493827160493827,
0.5,0.506172839506173,0.512345679012346,0.518518518518518,0.524691358024691,
0.530864197530864,0.537037037037037,0.54320987654321,0.549382716049383,
0.555555555555556,0.561728395061728,0.567901234567901,0.574074074074074,
0.580246913580247,0.58641975308642,0.592592592592593,0.598765432098765,
0.604938271604938,0.611111111111111,0.617283950617284,0.623456790123457,
0.62962962962963,0.635802469135803,0.641975308641975,0.648148148148148,
0.654320987654321,0.660493827160494,0.666666666666667,0.672839506172839,
0.679012345679012,0.685185185185185,0.691358024691358,0.697530864197531,
0.703703703703704,0.709876543209877,0.716049382716049,0.722222222222222,
0.728395061728395,0.734567901234568,0.740740740740741,0.746913580246914,
0.753086419753086,0.759259259259259,0.765432098765432,0.771604938271605,
0.777777777777778,0.783950617283951,0.790123456790123,0.796296296296296,
0.802469135802469,0.808641975308642,0.814814814814815,0.820987654320988,
0.827160493827161,0.833333333333333,0.839506172839506,0.845679012345679,
0.851851851851852,0.858024691358025,0.864197530864197,0.87037037037037,
0.876543209876543,0.882716049382716,0.888888888888889,0.895061728395062,
0.901234567901235,0.907407407407407,0.91358024691358,0.919753086419753,
0.925925925925926,0.932098765432099,0.938271604938272,0.944444444444444,
0.950617283950617,0.95679012345679,0.962962962962963,0.969135802469136,
0.975308641975309,0.977791447664447),.UNSPECIFIED.)
GEOMETRIC_REPRESENTATION_ITEM()
RATIONAL_B_SPLINE_SURFACE(((1.,0.866025403784439,1.,0.866025403784439,1.,
0.866025403784439,1.,0.866025403784439,1.,0.866025403784439,1.,0.866025403784439,
1.,0.866025403784439,1.,0.866025403784439,1.,0.866025403784439,1.,0.866025403784439,
1.,0.866025403784439,1.,0.866025403784439,1.,0.866025403784439,1.,0.866025403784439,
1.,0.866025403784439,1.,0.866025403784439,1.,0.866025403784439,1.,0.866025403784439,
1.,0.866025403784439,1.,0.866025403784439,1.,0.866025403784439,1.,0.866025403784439,
1.,0.866025403784439,1.,0.866025403784439,1.,0.866025403784439,1.,0.866025403784439,
1.,0.866025403784439,1.,0.866025403784439,1.,0.866025403784439,1.,0.866025403784439,
1.,0.866025403784439,1.,0.866025403784439,1.,0.866025403784439,1.,0.866025403784439,
1.,0.866025403784439,1.,0.866025403784439,1.,0.866025403784439,1.,0.866025403784439,
1.,0.866025403784439,1.,0.866025403784439,1.,0.866025403784439,1.,0.866025403784439,
1.,0.866025403784439,1.,0.866025403784439,1.,0.866025403784439,1.,0.866025403784439,
1.,0.866025403784439,1.,0.866025403784439,1.,0.866025403784439,1.,0.866025403784439,
1.,0.866025403784439,1.,0.866025403784439,1.,0.866025403784439,1.,0.866025403784439,
1.,0.866025403784439,1.,0.866025403784439,1.,0.866025403784439,1.,0.866025403784439,
1.,0.866025403784439,1.,0.866025403784439,1.,0.866025403784439,1.,0.866025403784439,
1.,0.866025403784439,1.,0.866025403784439,1.,0.866025403784439,1.,0.866025403784439,
1.,0.866025403784439,1.,0.866025403784439,1.,0.866025403784439,1.,0.866025403784439,
1.,0.866025403784439,1.,0.866025403784439,1.,0.866025403784439,1.,0.866025403784439,
1.,0.866025403784439,1.,0.866025403784439,1.,0.866025403784439,1.,0.866025403784439,
1.,0.866025403784439,1.,0.866025403784439,1.,0.866025403784439,1.,0.866025403784439,
1.,0.866025403784439,1.,0.866025403784439,1.,0.866025403784439,1.,0.866025403784439,
1.,0.866025403784439,1.,0.866025403784439,1.,0.866025403784439,1.,0.866025403784439,
1.,0.866025403784439,1.,0.866025403784439,1.,0.866025403784439,1.,0.866025403784439,
1.,0.866025403784439,1.,0.866025403784439,1.,0.866025403784439,1.,0.866025403784439,
1.,0.866025403784439,1.,0.866025403784439,1.,0.866025403784439,1.,0.866025403784439,
1.,0.866025403784439,1.,0.866025403784439,1.,0.866025403784439,1.,0.866025403784439,
1.,0.866025403784439,1.,0.866025403784439,1.,0.866025403784439,1.,0.866025403784439,
1.,0.866025403784439,1.,0.866025403784439,1.,0.866025403784439,1.,0.866025403784439,
1.,0.866025403784439,1.,0.866025403784439,1.,0.866025403784439,1.,0.866025403784439,
1.,0.866025403784439,1.,0.866025403784439,1.,0.866025403784439,1.,0.866025403784439,
1.,0.866025403784439,1.,0.866025403784439,1.,0.866025403784439,1.,0.866025403784439,
1.,0.866025403784439,1.,0.866025403784439,1.,0.866025403784439,1.,0.866025403784439,
1.,0.866025403784439,1.,0.866025403784439,1.,0.866025403784439,1.,0.866025403784439,
1.,0.866025403784439,1.,0.866025403784439,1.,0.866025403784439,1.,0.866025403784439,
1.,0.866025403784439,1.,0.866025403784439,1.,0.866025403784439,1.,0.866025403784439,
1.,0.866025403784439,1.,0.866025403784439,1.,0.866025403784439,1.,0.866025403784439,
1.,0.866025403784439,1.,0.866025403784439,1.,0.866025403784439,1.,0.866025403784439,
1.,0.866025403784439,1.,0.866025403784439,1.,0.866025403784439,1.,0.866025403784439,
1.,0.866025403784439,1.,0.866025403784439,1.,0.866025403784439,1.,0.866025403784439,
1.,0.9461134718712,0.935574832010768),(1.,0.866025403784439,1.,0.866025403784439,
1.,0.866025403784439,1.,0.866025403784439,1.,0.866025403784439,1.,0.866025403784439,
1.,0.866025403784439,1.,0.866025403784439,1.,0.866025403784439,1.,0.866025403784439,
1.,0.866025403784439,1.,0.866025403784439,1.,0.866025403784439,1.,0.866025403784439,
1.,0.866025403784439,1.,0.866025403784439,1.,0.866025403784439,1.,0.866025403784439,
1.,0.866025403784439,1.,0.866025403784439,1.,0.866025403784439,1.,0.866025403784439,
1.,0.866025403784439,1.,0.866025403784439,1.,0.866025403784439,1.,0.866025403784439,
1.,0.866025403784439,1.,0.866025403784439,1.,0.866025403784439,1.,0.866025403784439,
1.,0.866025403784439,1.,0.866025403784439,1.,0.866025403784439,1.,0.866025403784439,
1.,0.866025403784439,1.,0.866025403784439,1.,0.866025403784439,1.,0.866025403784439,
1.,0.866025403784439,1.,0.866025403784439,1.,0.866025403784439,1.,0.866025403784439,
1.,0.866025403784439,1.,0.866025403784439,1.,0.866025403784439,1.,0.866025403784439,
1.,0.866025403784439,1.,0.866025403784439,1.,0.866025403784439,1.,0.866025403784439,
1.,0.866025403784439,1.,0.866025403784439,1.,0.866025403784439,1.,0.866025403784439,
1.,0.866025403784439,1.,0.866025403784439,1.,0.866025403784439,1.,0.866025403784439,
1.,0.866025403784439,1.,0.866025403784439,1.,0.866025403784439,1.,0.866025403784439,
1.,0.866025403784439,1.,0.866025403784439,1.,0.866025403784439,1.,0.866025403784439,
1.,0.866025403784439,1.,0.866025403784439,1.,0.866025403784439,1.,0.866025403784439,
1.,0.866025403784439,1.,0.866025403784439,1.,0.866025403784439,1.,0.866025403784439,
1.,0.866025403784439,1.,0.866025403784439,1.,0.866025403784439,1.,0.866025403784439,
1.,0.866025403784439,1.,0.866025403784439,1.,0.866025403784439,1.,0.866025403784439,
1.,0.866025403784439,1.,0.866025403784439,1.,0.866025403784439,1.,0.866025403784439,
1.,0.866025403784439,1.,0.866025403784439,1.,0.866025403784439,1.,0.866025403784439,
1.,0.866025403784439,1.,0.866025403784439,1.,0.866025403784439,1.,0.866025403784439,
1.,0.866025403784439,1.,0.866025403784439,1.,0.866025403784439,1.,0.866025403784439,
1.,0.866025403784439,1.,0.866025403784439,1.,0.866025403784439,1.,0.866025403784439,
1.,0.866025403784439,1.,0.866025403784439,1.,0.866025403784439,1.,0.866025403784439,
1.,0.866025403784439,1.,0.866025403784439,1.,0.866025403784439,1.,0.866025403784439,
1.,0.866025403784439,1.,0.866025403784439,1.,0.866025403784439,1.,0.866025403784439,
1.,0.866025403784439,1.,0.866025403784439,1.,0.866025403784439,1.,0.866025403784439,
1.,0.866025403784439,1.,0.866025403784439,1.,0.866025403784439,1.,0.866025403784439,
1.,0.866025403784439,1.,0.866025403784439,1.,0.866025403784439,1.,0.866025403784439,
1.,0.866025403784439,1.,0.866025403784439,1.,0.866025403784439,1.,0.866025403784439,
1.,0.866025403784439,1.,0.866025403784439,1.,0.866025403784439,1.,0.866025403784439,
1.,0.866025403784439,1.,0.866025403784439,1.,0.866025403784439,1.,0.866025403784439,
1.,0.866025403784439,1.,0.866025403784439,1.,0.866025403784439,1.,0.866025403784439,
1.,0.866025403784439,1.,0.866025403784439,1.,0.866025403784439,1.,0.866025403784439,
1.,0.866025403784439,1.,0.866025403784439,1.,0.866025403784439,1.,0.866025403784439,
1.,0.866025403784439,1.,0.866025403784439,1.,0.866025403784439,1.,0.866025403784439,
1.,0.866025403784439,1.,0.866025403784439,1.,0.866025403784439,1.,0.866025403784439,
1.,0.9461134718712,0.935574832010768)))
REPRESENTATION_ITEM('')
SURFACE()
);
#293=(
BOUNDED_SURFACE()
B_SPLINE_SURFACE(1,2,((#27594,#27595,#27596,#27597,#27598,#27599,#27600,
#27601,#27602,#27603,#27604,#27605,#27606,#27607,#27608,#27609,#27610,#27611,
#27612,#27613,#27614,#27615,#27616,#27617,#27618,#27619,#27620,#27621,#27622,
#27623,#27624,#27625,#27626,#27627,#27628,#27629,#27630,#27631,#27632,#27633,
#27634,#27635,#27636,#27637,#27638,#27639,#27640,#27641,#27642,#27643,#27644,
#27645,#27646,#27647,#27648,#27649,#27650,#27651,#27652,#27653,#27654,#27655,
#27656,#27657,#27658,#27659,#27660,#27661,#27662,#27663,#27664,#27665,#27666,
#27667,#27668,#27669,#27670,#27671,#27672,#27673,#27674,#27675,#27676,#27677,
#27678,#27679,#27680,#27681,#27682,#27683,#27684,#27685,#27686,#27687,#27688,
#27689,#27690,#27691,#27692,#27693,#27694,#27695,#27696,#27697,#27698,#27699,
#27700,#27701,#27702,#27703,#27704,#27705,#27706,#27707,#27708,#27709,#27710,
#27711,#27712,#27713,#27714,#27715,#27716,#27717,#27718,#27719,#27720,#27721,
#27722,#27723,#27724,#27725,#27726,#27727,#27728,#27729,#27730,#27731,#27732,
#27733,#27734,#27735,#27736,#27737,#27738,#27739,#27740,#27741,#27742,#27743,
#27744,#27745,#27746,#27747,#27748,#27749,#27750,#27751,#27752,#27753,#27754,
#27755,#27756,#27757,#27758,#27759,#27760,#27761,#27762,#27763,#27764,#27765,
#27766,#27767,#27768,#27769,#27770,#27771,#27772,#27773,#27774,#27775,#27776,
#27777,#27778,#27779,#27780,#27781,#27782,#27783,#27784,#27785,#27786,#27787,
#27788,#27789,#27790,#27791,#27792,#27793,#27794,#27795,#27796,#27797,#27798,
#27799,#27800,#27801,#27802,#27803,#27804,#27805,#27806,#27807,#27808,#27809,
#27810,#27811,#27812,#27813,#27814,#27815,#27816,#27817,#27818,#27819,#27820,
#27821,#27822,#27823,#27824,#27825,#27826,#27827,#27828,#27829,#27830,#27831,
#27832,#27833,#27834,#27835,#27836,#27837,#27838,#27839,#27840,#27841,#27842,
#27843,#27844,#27845,#27846,#27847,#27848,#27849,#27850,#27851,#27852,#27853,
#27854,#27855,#27856,#27857,#27858,#27859,#27860,#27861,#27862,#27863,#27864,
#27865,#27866,#27867,#27868,#27869,#27870,#27871,#27872,#27873,#27874,#27875,
#27876,#27877,#27878,#27879,#27880,#27881,#27882,#27883,#27884,#27885,#27886,
#27887,#27888,#27889,#27890,#27891,#27892,#27893,#27894,#27895,#27896,#27897,
#27898,#27899,#27900,#27901,#27902,#27903,#27904,#27905,#27906,#27907,#27908,
#27909,#27910,#27911,#27912),(#27913,#27914,#27915,#27916,#27917,#27918,
#27919,#27920,#27921,#27922,#27923,#27924,#27925,#27926,#27927,#27928,#27929,
#27930,#27931,#27932,#27933,#27934,#27935,#27936,#27937,#27938,#27939,#27940,
#27941,#27942,#27943,#27944,#27945,#27946,#27947,#27948,#27949,#27950,#27951,
#27952,#27953,#27954,#27955,#27956,#27957,#27958,#27959,#27960,#27961,#27962,
#27963,#27964,#27965,#27966,#27967,#27968,#27969,#27970,#27971,#27972,#27973,
#27974,#27975,#27976,#27977,#27978,#27979,#27980,#27981,#27982,#27983,#27984,
#27985,#27986,#27987,#27988,#27989,#27990,#27991,#27992,#27993,#27994,#27995,
#27996,#27997,#27998,#27999,#28000,#28001,#28002,#28003,#28004,#28005,#28006,
#28007,#28008,#28009,#28010,#28011,#28012,#28013,#28014,#28015,#28016,#28017,
#28018,#28019,#28020,#28021,#28022,#28023,#28024,#28025,#28026,#28027,#28028,
#28029,#28030,#28031,#28032,#28033,#28034,#28035,#28036,#28037,#28038,#28039,
#28040,#28041,#28042,#28043,#28044,#28045,#28046,#28047,#28048,#28049,#28050,
#28051,#28052,#28053,#28054,#28055,#28056,#28057,#28058,#28059,#28060,#28061,
#28062,#28063,#28064,#28065,#28066,#28067,#28068,#28069,#28070,#28071,#28072,
#28073,#28074,#28075,#28076,#28077,#28078,#28079,#28080,#28081,#28082,#28083,
#28084,#28085,#28086,#28087,#28088,#28089,#28090,#28091,#28092,#28093,#28094,
#28095,#28096,#28097,#28098,#28099,#28100,#28101,#28102,#28103,#28104,#28105,
#28106,#28107,#28108,#28109,#28110,#28111,#28112,#28113,#28114,#28115,#28116,
#28117,#28118,#28119,#28120,#28121,#28122,#28123,#28124,#28125,#28126,#28127,
#28128,#28129,#28130,#28131,#28132,#28133,#28134,#28135,#28136,#28137,#28138,
#28139,#28140,#28141,#28142,#28143,#28144,#28145,#28146,#28147,#28148,#28149,
#28150,#28151,#28152,#28153,#28154,#28155,#28156,#28157,#28158,#28159,#28160,
#28161,#28162,#28163,#28164,#28165,#28166,#28167,#28168,#28169,#28170,#28171,
#28172,#28173,#28174,#28175,#28176,#28177,#28178,#28179,#28180,#28181,#28182,
#28183,#28184,#28185,#28186,#28187,#28188,#28189,#28190,#28191,#28192,#28193,
#28194,#28195,#28196,#28197,#28198,#28199,#28200,#28201,#28202,#28203,#28204,
#28205,#28206,#28207,#28208,#28209,#28210,#28211,#28212,#28213,#28214,#28215,
#28216,#28217,#28218,#28219,#28220,#28221,#28222,#28223,#28224,#28225,#28226,
#28227,#28228,#28229,#28230,#28231)),.UNSPECIFIED.,.F.,.F.,.F.)
B_SPLINE_SURFACE_WITH_KNOTS((2,2),(3,2,2,2,2,2,2,2,2,2,2,2,2,2,2,2,2,2,
2,2,2,2,2,2,2,2,2,2,2,2,2,2,2,2,2,2,2,2,2,2,2,2,2,2,2,2,2,2,2,2,2,2,2,2,
2,2,2,2,2,2,2,2,2,2,2,2,2,2,2,2,2,2,2,2,2,2,2,2,2,2,2,2,2,2,2,2,2,2,2,2,
2,2,2,2,2,2,2,2,2,2,2,2,2,2,2,2,2,2,2,2,2,2,2,2,2,2,2,2,2,2,2,2,2,2,2,2,
2,2,2,2,2,2,2,2,2,2,2,2,2,2,2,2,2,2,2,2,2,2,2,2,2,2,2,2,2,2,2,2,2,3),(0.,
1.00001332089208),(0.,0.00617283950617284,0.0123456790123457,0.0185185185185185,
0.0246913580246914,0.0308641975308642,0.037037037037037,0.0432098765432099,
0.0493827160493827,0.0555555555555556,0.0617283950617284,0.0679012345679012,
0.0740740740740741,0.0802469135802469,0.0864197530864197,0.0925925925925926,
0.0987654320987654,0.104938271604938,0.111111111111111,0.117283950617284,
0.123456790123457,0.12962962962963,0.135802469135802,0.141975308641975,
0.148148148148148,0.154320987654321,0.160493827160494,0.166666666666667,
0.172839506172839,0.179012345679012,0.185185185185185,0.191358024691358,
0.197530864197531,0.203703703703704,0.209876543209877,0.216049382716049,
0.222222222222222,0.228395061728395,0.234567901234568,0.240740740740741,
0.246913580246914,0.253086419753086,0.259259259259259,0.265432098765432,
0.271604938271605,0.277777777777778,0.283950617283951,0.290123456790123,
0.296296296296296,0.302469135802469,0.308641975308642,0.314814814814815,
0.320987654320988,0.327160493827161,0.333333333333333,0.339506172839506,
0.345679012345679,0.351851851851852,0.358024691358025,0.364197530864198,
0.37037037037037,0.376543209876543,0.382716049382716,0.388888888888889,
0.395061728395062,0.401234567901235,0.407407407407407,0.41358024691358,
0.419753086419753,0.425925925925926,0.432098765432099,0.438271604938272,
0.444444444444444,0.450617283950617,0.45679012345679,0.462962962962963,
0.469135802469136,0.475308641975309,0.481481481481481,0.487654320987654,
0.493827160493827,0.5,0.506172839506173,0.512345679012346,0.518518518518518,
0.524691358024691,0.530864197530864,0.537037037037037,0.54320987654321,
0.549382716049383,0.555555555555556,0.561728395061728,0.567901234567901,
0.574074074074074,0.580246913580247,0.58641975308642,0.592592592592593,
0.598765432098765,0.604938271604938,0.611111111111111,0.617283950617284,
0.623456790123457,0.62962962962963,0.635802469135803,0.641975308641975,
0.648148148148148,0.654320987654321,0.660493827160494,0.666666666666667,
0.672839506172839,0.679012345679012,0.685185185185185,0.691358024691358,
0.697530864197531,0.703703703703704,0.709876543209877,0.716049382716049,
0.722222222222222,0.728395061728395,0.734567901234568,0.740740740740741,
0.746913580246914,0.753086419753086,0.759259259259259,0.765432098765432,
0.771604938271605,0.777777777777778,0.783950617283951,0.790123456790123,
0.796296296296296,0.802469135802469,0.808641975308642,0.814814814814815,
0.820987654320988,0.827160493827161,0.833333333333333,0.839506172839506,
0.845679012345679,0.851851851851852,0.858024691358025,0.864197530864197,
0.87037037037037,0.876543209876543,0.882716049382716,0.888888888888889,
0.895061728395062,0.901234567901235,0.907407407407407,0.91358024691358,
0.919753086419753,0.925925925925926,0.932098765432099,0.938271604938272,
0.944444444444444,0.950617283950617,0.95679012345679,0.962962962962963,
0.969135802469136,0.975308641975309,0.977791440774828),.UNSPECIFIED.)
GEOMETRIC_REPRESENTATION_ITEM()
RATIONAL_B_SPLINE_SURFACE(((1.,0.866025403784439,1.,0.866025403784439,1.,
0.866025403784439,1.,0.866025403784439,1.,0.866025403784439,1.,0.866025403784439,
1.,0.866025403784439,1.,0.866025403784439,1.,0.866025403784439,1.,0.866025403784439,
1.,0.866025403784439,1.,0.866025403784439,1.,0.866025403784439,1.,0.866025403784439,
1.,0.866025403784439,1.,0.866025403784439,1.,0.866025403784439,1.,0.866025403784439,
1.,0.866025403784439,1.,0.866025403784439,1.,0.866025403784439,1.,0.866025403784439,
1.,0.866025403784439,1.,0.866025403784439,1.,0.866025403784439,1.,0.866025403784439,
1.,0.866025403784439,1.,0.866025403784439,1.,0.866025403784439,1.,0.866025403784439,
1.,0.866025403784439,1.,0.866025403784439,1.,0.866025403784439,1.,0.866025403784439,
1.,0.866025403784439,1.,0.866025403784439,1.,0.866025403784439,1.,0.866025403784439,
1.,0.866025403784439,1.,0.866025403784439,1.,0.866025403784439,1.,0.866025403784439,
1.,0.866025403784439,1.,0.866025403784439,1.,0.866025403784439,1.,0.866025403784439,
1.,0.866025403784439,1.,0.866025403784439,1.,0.866025403784439,1.,0.866025403784439,
1.,0.866025403784439,1.,0.866025403784439,1.,0.866025403784439,1.,0.866025403784439,
1.,0.866025403784439,1.,0.866025403784439,1.,0.866025403784439,1.,0.866025403784439,
1.,0.866025403784439,1.,0.866025403784439,1.,0.866025403784439,1.,0.866025403784439,
1.,0.866025403784439,1.,0.866025403784439,1.,0.866025403784439,1.,0.866025403784439,
1.,0.866025403784439,1.,0.866025403784439,1.,0.866025403784439,1.,0.866025403784439,
1.,0.866025403784439,1.,0.866025403784439,1.,0.866025403784439,1.,0.866025403784439,
1.,0.866025403784439,1.,0.866025403784439,1.,0.866025403784439,1.,0.866025403784439,
1.,0.866025403784439,1.,0.866025403784439,1.,0.866025403784439,1.,0.866025403784439,
1.,0.866025403784439,1.,0.866025403784439,1.,0.866025403784439,1.,0.866025403784439,
1.,0.866025403784439,1.,0.866025403784439,1.,0.866025403784439,1.,0.866025403784439,
1.,0.866025403784439,1.,0.866025403784439,1.,0.866025403784439,1.,0.866025403784439,
1.,0.866025403784439,1.,0.866025403784439,1.,0.866025403784439,1.,0.866025403784439,
1.,0.866025403784439,1.,0.866025403784439,1.,0.866025403784439,1.,0.866025403784439,
1.,0.866025403784439,1.,0.866025403784439,1.,0.866025403784439,1.,0.866025403784439,
1.,0.866025403784439,1.,0.866025403784439,1.,0.866025403784439,1.,0.866025403784439,
1.,0.866025403784439,1.,0.866025403784439,1.,0.866025403784439,1.,0.866025403784439,
1.,0.866025403784439,1.,0.866025403784439,1.,0.866025403784439,1.,0.866025403784439,
1.,0.866025403784439,1.,0.866025403784439,1.,0.866025403784439,1.,0.866025403784439,
1.,0.866025403784439,1.,0.866025403784439,1.,0.866025403784439,1.,0.866025403784439,
1.,0.866025403784439,1.,0.866025403784439,1.,0.866025403784439,1.,0.866025403784439,
1.,0.866025403784439,1.,0.866025403784439,1.,0.866025403784439,1.,0.866025403784439,
1.,0.866025403784439,1.,0.866025403784439,1.,0.866025403784439,1.,0.866025403784439,
1.,0.866025403784439,1.,0.866025403784439,1.,0.866025403784439,1.,0.866025403784439,
1.,0.866025403784439,1.,0.866025403784439,1.,0.866025403784439,1.,0.866025403784439,
1.,0.866025403784439,1.,0.866025403784439,1.,0.866025403784439,1.,0.866025403784439,
1.,0.866025403784439,1.,0.866025403784439,1.,0.866025403784439,1.,0.866025403784439,
1.,0.866025403784439,1.,0.866025403784439,1.,0.866025403784439,1.,0.866025403784439,
1.,0.946113621402695,0.935574890499137),(1.,0.866025403784439,1.,0.866025403784439,
1.,0.866025403784439,1.,0.866025403784439,1.,0.866025403784439,1.,0.866025403784439,
1.,0.866025403784439,1.,0.866025403784439,1.,0.866025403784439,1.,0.866025403784439,
1.,0.866025403784439,1.,0.866025403784439,1.,0.866025403784439,1.,0.866025403784439,
1.,0.866025403784439,1.,0.866025403784439,1.,0.866025403784439,1.,0.866025403784439,
1.,0.866025403784439,1.,0.866025403784439,1.,0.866025403784439,1.,0.866025403784439,
1.,0.866025403784439,1.,0.866025403784439,1.,0.866025403784439,1.,0.866025403784439,
1.,0.866025403784439,1.,0.866025403784439,1.,0.866025403784439,1.,0.866025403784439,
1.,0.866025403784439,1.,0.866025403784439,1.,0.866025403784439,1.,0.866025403784439,
1.,0.866025403784439,1.,0.866025403784439,1.,0.866025403784439,1.,0.866025403784439,
1.,0.866025403784439,1.,0.866025403784439,1.,0.866025403784439,1.,0.866025403784439,
1.,0.866025403784439,1.,0.866025403784439,1.,0.866025403784439,1.,0.866025403784439,
1.,0.866025403784439,1.,0.866025403784439,1.,0.866025403784439,1.,0.866025403784439,
1.,0.866025403784439,1.,0.866025403784439,1.,0.866025403784439,1.,0.866025403784439,
1.,0.866025403784439,1.,0.866025403784439,1.,0.866025403784439,1.,0.866025403784439,
1.,0.866025403784439,1.,0.866025403784439,1.,0.866025403784439,1.,0.866025403784439,
1.,0.866025403784439,1.,0.866025403784439,1.,0.866025403784439,1.,0.866025403784439,
1.,0.866025403784439,1.,0.866025403784439,1.,0.866025403784439,1.,0.866025403784439,
1.,0.866025403784439,1.,0.866025403784439,1.,0.866025403784439,1.,0.866025403784439,
1.,0.866025403784439,1.,0.866025403784439,1.,0.866025403784439,1.,0.866025403784439,
1.,0.866025403784439,1.,0.866025403784439,1.,0.866025403784439,1.,0.866025403784439,
1.,0.866025403784439,1.,0.866025403784439,1.,0.866025403784439,1.,0.866025403784439,
1.,0.866025403784439,1.,0.866025403784439,1.,0.866025403784439,1.,0.866025403784439,
1.,0.866025403784439,1.,0.866025403784439,1.,0.866025403784439,1.,0.866025403784439,
1.,0.866025403784439,1.,0.866025403784439,1.,0.866025403784439,1.,0.866025403784439,
1.,0.866025403784439,1.,0.866025403784439,1.,0.866025403784439,1.,0.866025403784439,
1.,0.866025403784439,1.,0.866025403784439,1.,0.866025403784439,1.,0.866025403784439,
1.,0.866025403784439,1.,0.866025403784439,1.,0.866025403784439,1.,0.866025403784439,
1.,0.866025403784439,1.,0.866025403784439,1.,0.866025403784439,1.,0.866025403784439,
1.,0.866025403784439,1.,0.866025403784439,1.,0.866025403784439,1.,0.866025403784439,
1.,0.866025403784439,1.,0.866025403784439,1.,0.866025403784439,1.,0.866025403784439,
1.,0.866025403784439,1.,0.866025403784439,1.,0.866025403784439,1.,0.866025403784439,
1.,0.866025403784439,1.,0.866025403784439,1.,0.866025403784439,1.,0.866025403784439,
1.,0.866025403784439,1.,0.866025403784439,1.,0.866025403784439,1.,0.866025403784439,
1.,0.866025403784439,1.,0.866025403784439,1.,0.866025403784439,1.,0.866025403784439,
1.,0.866025403784439,1.,0.866025403784439,1.,0.866025403784439,1.,0.866025403784439,
1.,0.866025403784439,1.,0.866025403784439,1.,0.866025403784439,1.,0.866025403784439,
1.,0.866025403784439,1.,0.866025403784439,1.,0.866025403784439,1.,0.866025403784439,
1.,0.866025403784439,1.,0.866025403784439,1.,0.866025403784439,1.,0.866025403784439,
1.,0.866025403784439,1.,0.866025403784439,1.,0.866025403784439,1.,0.866025403784439,
1.,0.946113621402695,0.935574890499137)))
REPRESENTATION_ITEM('')
SURFACE()
);
#294=(
BOUNDED_SURFACE()
B_SPLINE_SURFACE(1,2,((#28537,#28538,#28539,#28540,#28541,#28542,#28543,
#28544,#28545,#28546,#28547,#28548,#28549,#28550,#28551,#28552,#28553,#28554,
#28555,#28556,#28557,#28558,#28559,#28560,#28561,#28562,#28563,#28564,#28565,
#28566,#28567,#28568,#28569,#28570,#28571,#28572,#28573,#28574,#28575,#28576,
#28577,#28578,#28579,#28580,#28581,#28582,#28583,#28584,#28585,#28586,#28587,
#28588,#28589,#28590,#28591,#28592,#28593,#28594,#28595,#28596,#28597,#28598,
#28599,#28600,#28601,#28602,#28603,#28604,#28605,#28606,#28607,#28608,#28609,
#28610,#28611,#28612,#28613,#28614,#28615,#28616,#28617,#28618,#28619,#28620,
#28621,#28622,#28623,#28624,#28625,#28626,#28627,#28628,#28629,#28630,#28631,
#28632,#28633,#28634,#28635,#28636,#28637,#28638,#28639,#28640,#28641,#28642,
#28643,#28644,#28645,#28646,#28647,#28648,#28649,#28650,#28651,#28652,#28653,
#28654,#28655,#28656,#28657,#28658,#28659,#28660,#28661,#28662,#28663,#28664,
#28665,#28666,#28667,#28668,#28669,#28670,#28671,#28672,#28673,#28674,#28675,
#28676,#28677,#28678,#28679,#28680,#28681,#28682,#28683,#28684,#28685,#28686,
#28687,#28688,#28689,#28690,#28691,#28692,#28693,#28694,#28695,#28696,#28697,
#28698,#28699,#28700,#28701,#28702,#28703,#28704,#28705,#28706,#28707,#28708,
#28709,#28710,#28711,#28712,#28713,#28714,#28715,#28716,#28717,#28718,#28719,
#28720,#28721,#28722,#28723,#28724,#28725,#28726,#28727,#28728,#28729,#28730,
#28731,#28732,#28733,#28734,#28735,#28736,#28737,#28738,#28739,#28740,#28741,
#28742,#28743,#28744,#28745,#28746,#28747,#28748,#28749,#28750,#28751,#28752,
#28753,#28754,#28755,#28756,#28757,#28758,#28759,#28760,#28761,#28762,#28763,
#28764,#28765,#28766,#28767,#28768,#28769,#28770,#28771,#28772,#28773,#28774,
#28775,#28776,#28777,#28778,#28779,#28780,#28781,#28782,#28783,#28784,#28785,
#28786,#28787,#28788,#28789,#28790,#28791,#28792,#28793,#28794,#28795,#28796,
#28797,#28798,#28799,#28800,#28801,#28802,#28803,#28804,#28805,#28806,#28807,
#28808,#28809,#28810,#28811,#28812,#28813,#28814,#28815,#28816,#28817,#28818,
#28819,#28820,#28821,#28822,#28823,#28824,#28825,#28826,#28827,#28828,#28829,
#28830,#28831,#28832,#28833,#28834,#28835,#28836,#28837,#28838,#28839,#28840,
#28841,#28842,#28843,#28844,#28845,#28846,#28847,#28848,#28849,#28850,#28851,
#28852,#28853,#28854,#28855,#28856,#28857),(#28858,#28859,#28860,#28861,
#28862,#28863,#28864,#28865,#28866,#28867,#28868,#28869,#28870,#28871,#28872,
#28873,#28874,#28875,#28876,#28877,#28878,#28879,#28880,#28881,#28882,#28883,
#28884,#28885,#28886,#28887,#28888,#28889,#28890,#28891,#28892,#28893,#28894,
#28895,#28896,#28897,#28898,#28899,#28900,#28901,#28902,#28903,#28904,#28905,
#28906,#28907,#28908,#28909,#28910,#28911,#28912,#28913,#28914,#28915,#28916,
#28917,#28918,#28919,#28920,#28921,#28922,#28923,#28924,#28925,#28926,#28927,
#28928,#28929,#28930,#28931,#28932,#28933,#28934,#28935,#28936,#28937,#28938,
#28939,#28940,#28941,#28942,#28943,#28944,#28945,#28946,#28947,#28948,#28949,
#28950,#28951,#28952,#28953,#28954,#28955,#28956,#28957,#28958,#28959,#28960,
#28961,#28962,#28963,#28964,#28965,#28966,#28967,#28968,#28969,#28970,#28971,
#28972,#28973,#28974,#28975,#28976,#28977,#28978,#28979,#28980,#28981,#28982,
#28983,#28984,#28985,#28986,#28987,#28988,#28989,#28990,#28991,#28992,#28993,
#28994,#28995,#28996,#28997,#28998,#28999,#29000,#29001,#29002,#29003,#29004,
#29005,#29006,#29007,#29008,#29009,#29010,#29011,#29012,#29013,#29014,#29015,
#29016,#29017,#29018,#29019,#29020,#29021,#29022,#29023,#29024,#29025,#29026,
#29027,#29028,#29029,#29030,#29031,#29032,#29033,#29034,#29035,#29036,#29037,
#29038,#29039,#29040,#29041,#29042,#29043,#29044,#29045,#29046,#29047,#29048,
#29049,#29050,#29051,#29052,#29053,#29054,#29055,#29056,#29057,#29058,#29059,
#29060,#29061,#29062,#29063,#29064,#29065,#29066,#29067,#29068,#29069,#29070,
#29071,#29072,#29073,#29074,#29075,#29076,#29077,#29078,#29079,#29080,#29081,
#29082,#29083,#29084,#29085,#29086,#29087,#29088,#29089,#29090,#29091,#29092,
#29093,#29094,#29095,#29096,#29097,#29098,#29099,#29100,#29101,#29102,#29103,
#29104,#29105,#29106,#29107,#29108,#29109,#29110,#29111,#29112,#29113,#29114,
#29115,#29116,#29117,#29118,#29119,#29120,#29121,#29122,#29123,#29124,#29125,
#29126,#29127,#29128,#29129,#29130,#29131,#29132,#29133,#29134,#29135,#29136,
#29137,#29138,#29139,#29140,#29141,#29142,#29143,#29144,#29145,#29146,#29147,
#29148,#29149,#29150,#29151,#29152,#29153,#29154,#29155,#29156,#29157,#29158,
#29159,#29160,#29161,#29162,#29163,#29164,#29165,#29166,#29167,#29168,#29169,
#29170,#29171,#29172,#29173,#29174,#29175,#29176,#29177,#29178)),
 .UNSPECIFIED.,.F.,.F.,.F.)
B_SPLINE_SURFACE_WITH_KNOTS((2,2),(3,2,2,2,2,2,2,2,2,2,2,2,2,2,2,2,2,2,
2,2,2,2,2,2,2,2,2,2,2,2,2,2,2,2,2,2,2,2,2,2,2,2,2,2,2,2,2,2,2,2,2,2,2,2,
2,2,2,2,2,2,2,2,2,2,2,2,2,2,2,2,2,2,2,2,2,2,2,2,2,2,2,2,2,2,2,2,2,2,2,2,
2,2,2,2,2,2,2,2,2,2,2,2,2,2,2,2,2,2,2,2,2,2,2,2,2,2,2,2,2,2,2,2,2,2,2,2,
2,2,2,2,2,2,2,2,2,2,2,2,2,2,2,2,2,2,2,2,2,2,2,2,2,2,2,2,2,2,2,2,2,2,3),
(-0.000321975171239186,1.),(0.,0.00617283950617284,0.0123456790123457,0.0185185185185185,
0.0246913580246914,0.0308641975308642,0.037037037037037,0.0432098765432099,
0.0493827160493827,0.0555555555555556,0.0617283950617284,0.0679012345679012,
0.0740740740740741,0.0802469135802469,0.0864197530864197,0.0925925925925926,
0.0987654320987654,0.104938271604938,0.111111111111111,0.117283950617284,
0.123456790123457,0.12962962962963,0.135802469135802,0.141975308641975,
0.148148148148148,0.154320987654321,0.160493827160494,0.166666666666667,
0.172839506172839,0.179012345679012,0.185185185185185,0.191358024691358,
0.197530864197531,0.203703703703704,0.209876543209877,0.216049382716049,
0.222222222222222,0.228395061728395,0.234567901234568,0.240740740740741,
0.246913580246914,0.253086419753086,0.259259259259259,0.265432098765432,
0.271604938271605,0.277777777777778,0.283950617283951,0.290123456790123,
0.296296296296296,0.302469135802469,0.308641975308642,0.314814814814815,
0.320987654320988,0.327160493827161,0.333333333333333,0.339506172839506,
0.345679012345679,0.351851851851852,0.358024691358025,0.364197530864198,
0.37037037037037,0.376543209876543,0.382716049382716,0.388888888888889,
0.395061728395062,0.401234567901235,0.407407407407407,0.41358024691358,
0.419753086419753,0.425925925925926,0.432098765432099,0.438271604938272,
0.444444444444444,0.450617283950617,0.45679012345679,0.462962962962963,
0.469135802469136,0.475308641975309,0.481481481481481,0.487654320987654,
0.493827160493827,0.5,0.506172839506173,0.512345679012346,0.518518518518518,
0.524691358024691,0.530864197530864,0.537037037037037,0.54320987654321,
0.549382716049383,0.555555555555556,0.561728395061728,0.567901234567901,
0.574074074074074,0.580246913580247,0.58641975308642,0.592592592592593,
0.598765432098765,0.604938271604938,0.611111111111111,0.617283950617284,
0.623456790123457,0.62962962962963,0.635802469135803,0.641975308641975,
0.648148148148148,0.654320987654321,0.660493827160494,0.666666666666667,
0.672839506172839,0.679012345679012,0.685185185185185,0.691358024691358,
0.697530864197531,0.703703703703704,0.709876543209877,0.716049382716049,
0.722222222222222,0.728395061728395,0.734567901234568,0.740740740740741,
0.746913580246914,0.753086419753086,0.759259259259259,0.765432098765432,
0.771604938271605,0.777777777777778,0.783950617283951,0.790123456790123,
0.796296296296296,0.802469135802469,0.808641975308642,0.814814814814815,
0.820987654320988,0.827160493827161,0.833333333333333,0.839506172839506,
0.845679012345679,0.851851851851852,0.858024691358025,0.864197530864197,
0.87037037037037,0.876543209876543,0.882716049382716,0.888888888888889,
0.895061728395062,0.901234567901235,0.907407407407407,0.91358024691358,
0.919753086419753,0.925925925925926,0.932098765432099,0.938271604938272,
0.944444444444444,0.950617283950617,0.95679012345679,0.962962962962963,
0.969135802469136,0.975308641975309,0.977791393533952,0.987569307469292),
 .UNSPECIFIED.)
GEOMETRIC_REPRESENTATION_ITEM()
RATIONAL_B_SPLINE_SURFACE(((1.,0.866025403784439,1.,0.866025403784439,1.,
0.866025403784439,1.,0.866025403784439,1.,0.866025403784439,1.,0.866025403784439,
1.,0.866025403784439,1.,0.866025403784439,1.,0.866025403784439,1.,0.866025403784439,
1.,0.866025403784439,1.,0.866025403784439,1.,0.866025403784439,1.,0.866025403784439,
1.,0.866025403784439,1.,0.866025403784439,1.,0.866025403784439,1.,0.866025403784439,
1.,0.866025403784439,1.,0.866025403784439,1.,0.866025403784439,1.,0.866025403784439,
1.,0.866025403784439,1.,0.866025403784439,1.,0.866025403784439,1.,0.866025403784439,
1.,0.866025403784439,1.,0.866025403784439,1.,0.866025403784439,1.,0.866025403784439,
1.,0.866025403784439,1.,0.866025403784439,1.,0.866025403784439,1.,0.866025403784439,
1.,0.866025403784439,1.,0.866025403784439,1.,0.866025403784439,1.,0.866025403784439,
1.,0.866025403784439,1.,0.866025403784439,1.,0.866025403784439,1.,0.866025403784439,
1.,0.866025403784439,1.,0.866025403784439,1.,0.866025403784439,1.,0.866025403784439,
1.,0.866025403784439,1.,0.866025403784439,1.,0.866025403784439,1.,0.866025403784439,
1.,0.866025403784439,1.,0.866025403784439,1.,0.866025403784439,1.,0.866025403784439,
1.,0.866025403784439,1.,0.866025403784439,1.,0.866025403784439,1.,0.866025403784439,
1.,0.866025403784439,1.,0.866025403784439,1.,0.866025403784439,1.,0.866025403784439,
1.,0.866025403784439,1.,0.866025403784439,1.,0.866025403784439,1.,0.866025403784439,
1.,0.866025403784439,1.,0.866025403784439,1.,0.866025403784439,1.,0.866025403784439,
1.,0.866025403784439,1.,0.866025403784439,1.,0.866025403784439,1.,0.866025403784439,
1.,0.866025403784439,1.,0.866025403784439,1.,0.866025403784439,1.,0.866025403784439,
1.,0.866025403784439,1.,0.866025403784439,1.,0.866025403784439,1.,0.866025403784439,
1.,0.866025403784439,1.,0.866025403784439,1.,0.866025403784439,1.,0.866025403784439,
1.,0.866025403784439,1.,0.866025403784439,1.,0.866025403784439,1.,0.866025403784439,
1.,0.866025403784439,1.,0.866025403784439,1.,0.866025403784439,1.,0.866025403784439,
1.,0.866025403784439,1.,0.866025403784439,1.,0.866025403784439,1.,0.866025403784439,
1.,0.866025403784439,1.,0.866025403784439,1.,0.866025403784439,1.,0.866025403784439,
1.,0.866025403784439,1.,0.866025403784439,1.,0.866025403784439,1.,0.866025403784439,
1.,0.866025403784439,1.,0.866025403784439,1.,0.866025403784439,1.,0.866025403784439,
1.,0.866025403784439,1.,0.866025403784439,1.,0.866025403784439,1.,0.866025403784439,
1.,0.866025403784439,1.,0.866025403784439,1.,0.866025403784439,1.,0.866025403784439,
1.,0.866025403784439,1.,0.866025403784439,1.,0.866025403784439,1.,0.866025403784439,
1.,0.866025403784439,1.,0.866025403784439,1.,0.866025403784439,1.,0.866025403784439,
1.,0.866025403784439,1.,0.866025403784439,1.,0.866025403784439,1.,0.866025403784439,
1.,0.866025403784439,1.,0.866025403784439,1.,0.866025403784439,1.,0.866025403784439,
1.,0.866025403784439,1.,0.866025403784439,1.,0.866025403784439,1.,0.866025403784439,
1.,0.866025403784439,1.,0.866025403784439,1.,0.866025403784439,1.,0.866025403784439,
1.,0.866025403784439,1.,0.866025403784439,1.,0.866025403784439,1.,0.866025403784439,
1.,0.866025403784439,1.,0.866025403784439,1.,0.866025403784439,1.,0.866025403784439,
1.,0.866025403784439,1.,0.866025403784439,1.,0.866025403784439,1.,0.866025403784439,
1.,0.866025403784439,1.,0.866025403784439,1.,0.866025403784439,1.,0.866025403784439,
1.,0.946114646713198,0.93557529156132,0.93557529156132,0.93557529156132),
(1.,0.866025403784439,1.,0.866025403784439,1.,0.866025403784439,1.,0.866025403784439,
1.,0.866025403784439,1.,0.866025403784439,1.,0.866025403784439,1.,0.866025403784439,
1.,0.866025403784439,1.,0.866025403784439,1.,0.866025403784439,1.,0.866025403784439,
1.,0.866025403784439,1.,0.866025403784439,1.,0.866025403784439,1.,0.866025403784439,
1.,0.866025403784439,1.,0.866025403784439,1.,0.866025403784439,1.,0.866025403784439,
1.,0.866025403784439,1.,0.866025403784439,1.,0.866025403784439,1.,0.866025403784439,
1.,0.866025403784439,1.,0.866025403784439,1.,0.866025403784439,1.,0.866025403784439,
1.,0.866025403784439,1.,0.866025403784439,1.,0.866025403784439,1.,0.866025403784439,
1.,0.866025403784439,1.,0.866025403784439,1.,0.866025403784439,1.,0.866025403784439,
1.,0.866025403784439,1.,0.866025403784439,1.,0.866025403784439,1.,0.866025403784439,
1.,0.866025403784439,1.,0.866025403784439,1.,0.866025403784439,1.,0.866025403784439,
1.,0.866025403784439,1.,0.866025403784439,1.,0.866025403784439,1.,0.866025403784439,
1.,0.866025403784439,1.,0.866025403784439,1.,0.866025403784439,1.,0.866025403784439,
1.,0.866025403784439,1.,0.866025403784439,1.,0.866025403784439,1.,0.866025403784439,
1.,0.866025403784439,1.,0.866025403784439,1.,0.866025403784439,1.,0.866025403784439,
1.,0.866025403784439,1.,0.866025403784439,1.,0.866025403784439,1.,0.866025403784439,
1.,0.866025403784439,1.,0.866025403784439,1.,0.866025403784439,1.,0.866025403784439,
1.,0.866025403784439,1.,0.866025403784439,1.,0.866025403784439,1.,0.866025403784439,
1.,0.866025403784439,1.,0.866025403784439,1.,0.866025403784439,1.,0.866025403784439,
1.,0.866025403784439,1.,0.866025403784439,1.,0.866025403784439,1.,0.866025403784439,
1.,0.866025403784439,1.,0.866025403784439,1.,0.866025403784439,1.,0.866025403784439,
1.,0.866025403784439,1.,0.866025403784439,1.,0.866025403784439,1.,0.866025403784439,
1.,0.866025403784439,1.,0.866025403784439,1.,0.866025403784439,1.,0.866025403784439,
1.,0.866025403784439,1.,0.866025403784439,1.,0.866025403784439,1.,0.866025403784439,
1.,0.866025403784439,1.,0.866025403784439,1.,0.866025403784439,1.,0.866025403784439,
1.,0.866025403784439,1.,0.866025403784439,1.,0.866025403784439,1.,0.866025403784439,
1.,0.866025403784439,1.,0.866025403784439,1.,0.866025403784439,1.,0.866025403784439,
1.,0.866025403784439,1.,0.866025403784439,1.,0.866025403784439,1.,0.866025403784439,
1.,0.866025403784439,1.,0.866025403784439,1.,0.866025403784439,1.,0.866025403784439,
1.,0.866025403784439,1.,0.866025403784439,1.,0.866025403784439,1.,0.866025403784439,
1.,0.866025403784439,1.,0.866025403784439,1.,0.866025403784439,1.,0.866025403784439,
1.,0.866025403784439,1.,0.866025403784439,1.,0.866025403784439,1.,0.866025403784439,
1.,0.866025403784439,1.,0.866025403784439,1.,0.866025403784439,1.,0.866025403784439,
1.,0.866025403784439,1.,0.866025403784439,1.,0.866025403784439,1.,0.866025403784439,
1.,0.866025403784439,1.,0.866025403784439,1.,0.866025403784439,1.,0.866025403784439,
1.,0.866025403784439,1.,0.866025403784439,1.,0.866025403784439,1.,0.866025403784439,
1.,0.866025403784439,1.,0.866025403784439,1.,0.866025403784439,1.,0.866025403784439,
1.,0.866025403784439,1.,0.866025403784439,1.,0.866025403784439,1.,0.866025403784439,
1.,0.866025403784439,1.,0.866025403784439,1.,0.866025403784439,1.,0.866025403784439,
1.,0.866025403784439,1.,0.866025403784439,1.,0.946114646713198,0.93557529156132,
0.93557529156132,0.93557529156132)))
REPRESENTATION_ITEM('')
SURFACE()
);
#295=(
BOUNDED_SURFACE()
B_SPLINE_SURFACE(1,2,((#29179,#29180,#29181,#29182,#29183,#29184,#29185,
#29186,#29187,#29188,#29189,#29190,#29191,#29192,#29193,#29194,#29195,#29196,
#29197,#29198,#29199,#29200,#29201,#29202,#29203,#29204,#29205,#29206,#29207,
#29208,#29209,#29210,#29211,#29212,#29213,#29214,#29215,#29216,#29217,#29218,
#29219,#29220,#29221,#29222,#29223,#29224,#29225,#29226,#29227,#29228,#29229,
#29230,#29231,#29232,#29233,#29234,#29235,#29236,#29237,#29238,#29239,#29240,
#29241,#29242,#29243,#29244,#29245,#29246,#29247,#29248,#29249,#29250,#29251,
#29252,#29253,#29254,#29255,#29256,#29257,#29258,#29259,#29260,#29261,#29262,
#29263,#29264,#29265,#29266,#29267,#29268,#29269,#29270,#29271,#29272,#29273,
#29274,#29275,#29276,#29277,#29278,#29279,#29280,#29281,#29282,#29283,#29284,
#29285,#29286,#29287,#29288,#29289,#29290,#29291,#29292,#29293,#29294,#29295,
#29296,#29297,#29298,#29299,#29300,#29301,#29302,#29303,#29304,#29305,#29306,
#29307,#29308,#29309,#29310,#29311,#29312,#29313,#29314,#29315,#29316,#29317,
#29318,#29319,#29320,#29321,#29322,#29323,#29324,#29325,#29326,#29327,#29328,
#29329,#29330,#29331,#29332,#29333,#29334,#29335,#29336,#29337,#29338,#29339,
#29340,#29341,#29342,#29343,#29344,#29345,#29346,#29347,#29348,#29349,#29350,
#29351,#29352,#29353,#29354,#29355,#29356,#29357,#29358,#29359,#29360,#29361,
#29362,#29363,#29364,#29365,#29366,#29367,#29368,#29369,#29370,#29371,#29372,
#29373,#29374,#29375,#29376,#29377,#29378,#29379,#29380,#29381,#29382,#29383,
#29384,#29385,#29386,#29387,#29388,#29389,#29390,#29391,#29392,#29393,#29394,
#29395,#29396,#29397,#29398,#29399,#29400,#29401,#29402,#29403,#29404,#29405,
#29406,#29407,#29408,#29409,#29410,#29411,#29412,#29413,#29414,#29415,#29416,
#29417,#29418,#29419,#29420,#29421,#29422,#29423,#29424,#29425,#29426,#29427,
#29428,#29429,#29430,#29431,#29432,#29433,#29434,#29435,#29436,#29437,#29438,
#29439,#29440,#29441,#29442,#29443,#29444,#29445,#29446,#29447,#29448,#29449,
#29450,#29451,#29452,#29453,#29454,#29455,#29456,#29457,#29458,#29459,#29460,
#29461,#29462,#29463,#29464,#29465,#29466,#29467,#29468,#29469,#29470,#29471,
#29472,#29473,#29474,#29475,#29476,#29477,#29478,#29479,#29480,#29481,#29482,
#29483,#29484,#29485,#29486,#29487,#29488,#29489,#29490,#29491,#29492,#29493,
#29494,#29495,#29496,#29497),(#29498,#29499,#29500,#29501,#29502,#29503,
#29504,#29505,#29506,#29507,#29508,#29509,#29510,#29511,#29512,#29513,#29514,
#29515,#29516,#29517,#29518,#29519,#29520,#29521,#29522,#29523,#29524,#29525,
#29526,#29527,#29528,#29529,#29530,#29531,#29532,#29533,#29534,#29535,#29536,
#29537,#29538,#29539,#29540,#29541,#29542,#29543,#29544,#29545,#29546,#29547,
#29548,#29549,#29550,#29551,#29552,#29553,#29554,#29555,#29556,#29557,#29558,
#29559,#29560,#29561,#29562,#29563,#29564,#29565,#29566,#29567,#29568,#29569,
#29570,#29571,#29572,#29573,#29574,#29575,#29576,#29577,#29578,#29579,#29580,
#29581,#29582,#29583,#29584,#29585,#29586,#29587,#29588,#29589,#29590,#29591,
#29592,#29593,#29594,#29595,#29596,#29597,#29598,#29599,#29600,#29601,#29602,
#29603,#29604,#29605,#29606,#29607,#29608,#29609,#29610,#29611,#29612,#29613,
#29614,#29615,#29616,#29617,#29618,#29619,#29620,#29621,#29622,#29623,#29624,
#29625,#29626,#29627,#29628,#29629,#29630,#29631,#29632,#29633,#29634,#29635,
#29636,#29637,#29638,#29639,#29640,#29641,#29642,#29643,#29644,#29645,#29646,
#29647,#29648,#29649,#29650,#29651,#29652,#29653,#29654,#29655,#29656,#29657,
#29658,#29659,#29660,#29661,#29662,#29663,#29664,#29665,#29666,#29667,#29668,
#29669,#29670,#29671,#29672,#29673,#29674,#29675,#29676,#29677,#29678,#29679,
#29680,#29681,#29682,#29683,#29684,#29685,#29686,#29687,#29688,#29689,#29690,
#29691,#29692,#29693,#29694,#29695,#29696,#29697,#29698,#29699,#29700,#29701,
#29702,#29703,#29704,#29705,#29706,#29707,#29708,#29709,#29710,#29711,#29712,
#29713,#29714,#29715,#29716,#29717,#29718,#29719,#29720,#29721,#29722,#29723,
#29724,#29725,#29726,#29727,#29728,#29729,#29730,#29731,#29732,#29733,#29734,
#29735,#29736,#29737,#29738,#29739,#29740,#29741,#29742,#29743,#29744,#29745,
#29746,#29747,#29748,#29749,#29750,#29751,#29752,#29753,#29754,#29755,#29756,
#29757,#29758,#29759,#29760,#29761,#29762,#29763,#29764,#29765,#29766,#29767,
#29768,#29769,#29770,#29771,#29772,#29773,#29774,#29775,#29776,#29777,#29778,
#29779,#29780,#29781,#29782,#29783,#29784,#29785,#29786,#29787,#29788,#29789,
#29790,#29791,#29792,#29793,#29794,#29795,#29796,#29797,#29798,#29799,#29800,
#29801,#29802,#29803,#29804,#29805,#29806,#29807,#29808,#29809,#29810,#29811,
#29812,#29813,#29814,#29815,#29816)),.UNSPECIFIED.,.F.,.F.,.F.)
B_SPLINE_SURFACE_WITH_KNOTS((2,2),(3,2,2,2,2,2,2,2,2,2,2,2,2,2,2,2,2,2,
2,2,2,2,2,2,2,2,2,2,2,2,2,2,2,2,2,2,2,2,2,2,2,2,2,2,2,2,2,2,2,2,2,2,2,2,
2,2,2,2,2,2,2,2,2,2,2,2,2,2,2,2,2,2,2,2,2,2,2,2,2,2,2,2,2,2,2,2,2,2,2,2,
2,2,2,2,2,2,2,2,2,2,2,2,2,2,2,2,2,2,2,2,2,2,2,2,2,2,2,2,2,2,2,2,2,2,2,2,
2,2,2,2,2,2,2,2,2,2,2,2,2,2,2,2,2,2,2,2,2,2,2,2,2,2,2,2,2,2,2,2,2,3),(-2.4733869132694E-5,
1.),(0.,0.00617283950617284,0.0123456790123457,0.0185185185185185,0.0246913580246914,
0.0308641975308642,0.037037037037037,0.0432098765432099,0.0493827160493827,
0.0555555555555556,0.0617283950617284,0.0679012345679012,0.0740740740740741,
0.0802469135802469,0.0864197530864197,0.0925925925925926,0.0987654320987654,
0.104938271604938,0.111111111111111,0.117283950617284,0.123456790123457,
0.12962962962963,0.135802469135802,0.141975308641975,0.148148148148148,
0.154320987654321,0.160493827160494,0.166666666666667,0.172839506172839,
0.179012345679012,0.185185185185185,0.191358024691358,0.197530864197531,
0.203703703703704,0.209876543209877,0.216049382716049,0.222222222222222,
0.228395061728395,0.234567901234568,0.240740740740741,0.246913580246914,
0.253086419753086,0.259259259259259,0.265432098765432,0.271604938271605,
0.277777777777778,0.283950617283951,0.290123456790123,0.296296296296296,
0.302469135802469,0.308641975308642,0.314814814814815,0.320987654320988,
0.327160493827161,0.333333333333333,0.339506172839506,0.345679012345679,
0.351851851851852,0.358024691358025,0.364197530864198,0.37037037037037,
0.376543209876543,0.382716049382716,0.388888888888889,0.395061728395062,
0.401234567901235,0.407407407407407,0.41358024691358,0.419753086419753,
0.425925925925926,0.432098765432099,0.438271604938272,0.444444444444444,
0.450617283950617,0.45679012345679,0.462962962962963,0.469135802469136,
0.475308641975309,0.481481481481481,0.487654320987654,0.493827160493827,
0.5,0.506172839506173,0.512345679012346,0.518518518518518,0.524691358024691,
0.530864197530864,0.537037037037037,0.54320987654321,0.549382716049383,
0.555555555555556,0.561728395061728,0.567901234567901,0.574074074074074,
0.580246913580247,0.58641975308642,0.592592592592593,0.598765432098765,
0.604938271604938,0.611111111111111,0.617283950617284,0.623456790123457,
0.62962962962963,0.635802469135803,0.641975308641975,0.648148148148148,
0.654320987654321,0.660493827160494,0.666666666666667,0.672839506172839,
0.679012345679012,0.685185185185185,0.691358024691358,0.697530864197531,
0.703703703703704,0.709876543209877,0.716049382716049,0.722222222222222,
0.728395061728395,0.734567901234568,0.740740740740741,0.746913580246914,
0.753086419753086,0.759259259259259,0.765432098765432,0.771604938271605,
0.777777777777778,0.783950617283951,0.790123456790123,0.796296296296296,
0.802469135802469,0.808641975308642,0.814814814814815,0.820987654320988,
0.827160493827161,0.833333333333333,0.839506172839506,0.845679012345679,
0.851851851851852,0.858024691358025,0.864197530864197,0.87037037037037,
0.876543209876543,0.882716049382716,0.888888888888889,0.895061728395062,
0.901234567901235,0.907407407407407,0.91358024691358,0.919753086419753,
0.925925925925926,0.932098765432099,0.938271604938272,0.944444444444444,
0.950617283950617,0.95679012345679,0.962962962962963,0.969135802469136,
0.975308641975309,0.977791447664447),.UNSPECIFIED.)
GEOMETRIC_REPRESENTATION_ITEM()
RATIONAL_B_SPLINE_SURFACE(((1.,0.866025403784439,1.,0.866025403784439,1.,
0.866025403784439,1.,0.866025403784439,1.,0.866025403784439,1.,0.866025403784439,
1.,0.866025403784439,1.,0.866025403784439,1.,0.866025403784439,1.,0.866025403784439,
1.,0.866025403784439,1.,0.866025403784439,1.,0.866025403784439,1.,0.866025403784439,
1.,0.866025403784439,1.,0.866025403784439,1.,0.866025403784439,1.,0.866025403784439,
1.,0.866025403784439,1.,0.866025403784439,1.,0.866025403784439,1.,0.866025403784439,
1.,0.866025403784439,1.,0.866025403784439,1.,0.866025403784439,1.,0.866025403784439,
1.,0.866025403784439,1.,0.866025403784439,1.,0.866025403784439,1.,0.866025403784439,
1.,0.866025403784439,1.,0.866025403784439,1.,0.866025403784439,1.,0.866025403784439,
1.,0.866025403784439,1.,0.866025403784439,1.,0.866025403784439,1.,0.866025403784439,
1.,0.866025403784439,1.,0.866025403784439,1.,0.866025403784439,1.,0.866025403784439,
1.,0.866025403784439,1.,0.866025403784439,1.,0.866025403784439,1.,0.866025403784439,
1.,0.866025403784439,1.,0.866025403784439,1.,0.866025403784439,1.,0.866025403784439,
1.,0.866025403784439,1.,0.866025403784439,1.,0.866025403784439,1.,0.866025403784439,
1.,0.866025403784439,1.,0.866025403784439,1.,0.866025403784439,1.,0.866025403784439,
1.,0.866025403784439,1.,0.866025403784439,1.,0.866025403784439,1.,0.866025403784439,
1.,0.866025403784439,1.,0.866025403784439,1.,0.866025403784439,1.,0.866025403784439,
1.,0.866025403784439,1.,0.866025403784439,1.,0.866025403784439,1.,0.866025403784439,
1.,0.866025403784439,1.,0.866025403784439,1.,0.866025403784439,1.,0.866025403784439,
1.,0.866025403784439,1.,0.866025403784439,1.,0.866025403784439,1.,0.866025403784439,
1.,0.866025403784439,1.,0.866025403784439,1.,0.866025403784439,1.,0.866025403784439,
1.,0.866025403784439,1.,0.866025403784439,1.,0.866025403784439,1.,0.866025403784439,
1.,0.866025403784439,1.,0.866025403784439,1.,0.866025403784439,1.,0.866025403784439,
1.,0.866025403784439,1.,0.866025403784439,1.,0.866025403784439,1.,0.866025403784439,
1.,0.866025403784439,1.,0.866025403784439,1.,0.866025403784439,1.,0.866025403784439,
1.,0.866025403784439,1.,0.866025403784439,1.,0.866025403784439,1.,0.866025403784439,
1.,0.866025403784439,1.,0.866025403784439,1.,0.866025403784439,1.,0.866025403784439,
1.,0.866025403784439,1.,0.866025403784439,1.,0.866025403784439,1.,0.866025403784439,
1.,0.866025403784439,1.,0.866025403784439,1.,0.866025403784439,1.,0.866025403784439,
1.,0.866025403784439,1.,0.866025403784439,1.,0.866025403784439,1.,0.866025403784439,
1.,0.866025403784439,1.,0.866025403784439,1.,0.866025403784439,1.,0.866025403784439,
1.,0.866025403784439,1.,0.866025403784439,1.,0.866025403784439,1.,0.866025403784439,
1.,0.866025403784439,1.,0.866025403784439,1.,0.866025403784439,1.,0.866025403784439,
1.,0.866025403784439,1.,0.866025403784439,1.,0.866025403784439,1.,0.866025403784439,
1.,0.866025403784439,1.,0.866025403784439,1.,0.866025403784439,1.,0.866025403784439,
1.,0.866025403784439,1.,0.866025403784439,1.,0.866025403784439,1.,0.866025403784439,
1.,0.866025403784439,1.,0.866025403784439,1.,0.866025403784439,1.,0.866025403784439,
1.,0.866025403784439,1.,0.866025403784439,1.,0.866025403784439,1.,0.866025403784439,
1.,0.866025403784439,1.,0.866025403784439,1.,0.866025403784439,1.,0.866025403784439,
1.,0.866025403784439,1.,0.866025403784439,1.,0.866025403784439,1.,0.866025403784439,
1.,0.9461134718712,0.935574832010768),(1.,0.866025403784439,1.,0.866025403784439,
1.,0.866025403784439,1.,0.866025403784439,1.,0.866025403784439,1.,0.866025403784439,
1.,0.866025403784439,1.,0.866025403784439,1.,0.866025403784439,1.,0.866025403784439,
1.,0.866025403784439,1.,0.866025403784439,1.,0.866025403784439,1.,0.866025403784439,
1.,0.866025403784439,1.,0.866025403784439,1.,0.866025403784439,1.,0.866025403784439,
1.,0.866025403784439,1.,0.866025403784439,1.,0.866025403784439,1.,0.866025403784439,
1.,0.866025403784439,1.,0.866025403784439,1.,0.866025403784439,1.,0.866025403784439,
1.,0.866025403784439,1.,0.866025403784439,1.,0.866025403784439,1.,0.866025403784439,
1.,0.866025403784439,1.,0.866025403784439,1.,0.866025403784439,1.,0.866025403784439,
1.,0.866025403784439,1.,0.866025403784439,1.,0.866025403784439,1.,0.866025403784439,
1.,0.866025403784439,1.,0.866025403784439,1.,0.866025403784439,1.,0.866025403784439,
1.,0.866025403784439,1.,0.866025403784439,1.,0.866025403784439,1.,0.866025403784439,
1.,0.866025403784439,1.,0.866025403784439,1.,0.866025403784439,1.,0.866025403784439,
1.,0.866025403784439,1.,0.866025403784439,1.,0.866025403784439,1.,0.866025403784439,
1.,0.866025403784439,1.,0.866025403784439,1.,0.866025403784439,1.,0.866025403784439,
1.,0.866025403784439,1.,0.866025403784439,1.,0.866025403784439,1.,0.866025403784439,
1.,0.866025403784439,1.,0.866025403784439,1.,0.866025403784439,1.,0.866025403784439,
1.,0.866025403784439,1.,0.866025403784439,1.,0.866025403784439,1.,0.866025403784439,
1.,0.866025403784439,1.,0.866025403784439,1.,0.866025403784439,1.,0.866025403784439,
1.,0.866025403784439,1.,0.866025403784439,1.,0.866025403784439,1.,0.866025403784439,
1.,0.866025403784439,1.,0.866025403784439,1.,0.866025403784439,1.,0.866025403784439,
1.,0.866025403784439,1.,0.866025403784439,1.,0.866025403784439,1.,0.866025403784439,
1.,0.866025403784439,1.,0.866025403784439,1.,0.866025403784439,1.,0.866025403784439,
1.,0.866025403784439,1.,0.866025403784439,1.,0.866025403784439,1.,0.866025403784439,
1.,0.866025403784439,1.,0.866025403784439,1.,0.866025403784439,1.,0.866025403784439,
1.,0.866025403784439,1.,0.866025403784439,1.,0.866025403784439,1.,0.866025403784439,
1.,0.866025403784439,1.,0.866025403784439,1.,0.866025403784439,1.,0.866025403784439,
1.,0.866025403784439,1.,0.866025403784439,1.,0.866025403784439,1.,0.866025403784439,
1.,0.866025403784439,1.,0.866025403784439,1.,0.866025403784439,1.,0.866025403784439,
1.,0.866025403784439,1.,0.866025403784439,1.,0.866025403784439,1.,0.866025403784439,
1.,0.866025403784439,1.,0.866025403784439,1.,0.866025403784439,1.,0.866025403784439,
1.,0.866025403784439,1.,0.866025403784439,1.,0.866025403784439,1.,0.866025403784439,
1.,0.866025403784439,1.,0.866025403784439,1.,0.866025403784439,1.,0.866025403784439,
1.,0.866025403784439,1.,0.866025403784439,1.,0.866025403784439,1.,0.866025403784439,
1.,0.866025403784439,1.,0.866025403784439,1.,0.866025403784439,1.,0.866025403784439,
1.,0.866025403784439,1.,0.866025403784439,1.,0.866025403784439,1.,0.866025403784439,
1.,0.866025403784439,1.,0.866025403784439,1.,0.866025403784439,1.,0.866025403784439,
1.,0.866025403784439,1.,0.866025403784439,1.,0.866025403784439,1.,0.866025403784439,
1.,0.866025403784439,1.,0.866025403784439,1.,0.866025403784439,1.,0.866025403784439,
1.,0.866025403784439,1.,0.866025403784439,1.,0.866025403784439,1.,0.866025403784439,
1.,0.9461134718712,0.935574832010768)))
REPRESENTATION_ITEM('')
SURFACE()
);
#296=(
BOUNDED_SURFACE()
B_SPLINE_SURFACE(1,2,((#30120,#30121,#30122,#30123,#30124,#30125,#30126,
#30127,#30128,#30129,#30130,#30131,#30132,#30133,#30134,#30135,#30136,#30137,
#30138,#30139,#30140,#30141,#30142,#30143,#30144,#30145,#30146,#30147,#30148,
#30149,#30150,#30151,#30152,#30153,#30154,#30155,#30156,#30157,#30158,#30159,
#30160,#30161,#30162,#30163,#30164,#30165,#30166,#30167,#30168,#30169,#30170,
#30171,#30172,#30173,#30174,#30175,#30176,#30177,#30178,#30179,#30180,#30181,
#30182,#30183,#30184,#30185,#30186,#30187,#30188,#30189,#30190,#30191,#30192,
#30193,#30194,#30195,#30196,#30197,#30198,#30199,#30200,#30201,#30202,#30203,
#30204,#30205,#30206,#30207,#30208,#30209,#30210,#30211,#30212,#30213,#30214,
#30215,#30216,#30217,#30218,#30219,#30220,#30221,#30222,#30223,#30224,#30225,
#30226,#30227,#30228,#30229,#30230,#30231,#30232,#30233,#30234,#30235,#30236,
#30237,#30238,#30239,#30240,#30241,#30242,#30243,#30244,#30245,#30246,#30247,
#30248,#30249,#30250,#30251,#30252,#30253,#30254,#30255,#30256,#30257,#30258,
#30259,#30260,#30261,#30262,#30263,#30264,#30265,#30266,#30267,#30268,#30269,
#30270,#30271,#30272,#30273,#30274,#30275,#30276,#30277,#30278,#30279,#30280,
#30281,#30282,#30283,#30284,#30285,#30286,#30287,#30288,#30289,#30290,#30291,
#30292,#30293,#30294,#30295,#30296,#30297,#30298,#30299,#30300,#30301,#30302,
#30303,#30304,#30305,#30306,#30307,#30308,#30309,#30310,#30311,#30312,#30313,
#30314,#30315,#30316,#30317,#30318,#30319,#30320,#30321,#30322,#30323,#30324,
#30325,#30326,#30327,#30328,#30329,#30330,#30331,#30332,#30333,#30334,#30335,
#30336,#30337,#30338,#30339,#30340,#30341,#30342,#30343,#30344,#30345,#30346,
#30347,#30348,#30349,#30350,#30351,#30352,#30353,#30354,#30355,#30356,#30357,
#30358,#30359,#30360,#30361,#30362,#30363,#30364,#30365,#30366,#30367,#30368,
#30369,#30370,#30371,#30372,#30373,#30374,#30375,#30376,#30377,#30378,#30379,
#30380,#30381,#30382,#30383,#30384,#30385,#30386,#30387,#30388,#30389,#30390,
#30391,#30392,#30393,#30394,#30395,#30396,#30397,#30398,#30399,#30400,#30401,
#30402,#30403,#30404,#30405,#30406,#30407,#30408,#30409,#30410,#30411,#30412,
#30413,#30414,#30415,#30416,#30417,#30418,#30419,#30420,#30421,#30422,#30423,
#30424,#30425,#30426,#30427,#30428,#30429,#30430,#30431,#30432,#30433,#30434,
#30435,#30436,#30437,#30438),(#30439,#30440,#30441,#30442,#30443,#30444,
#30445,#30446,#30447,#30448,#30449,#30450,#30451,#30452,#30453,#30454,#30455,
#30456,#30457,#30458,#30459,#30460,#30461,#30462,#30463,#30464,#30465,#30466,
#30467,#30468,#30469,#30470,#30471,#30472,#30473,#30474,#30475,#30476,#30477,
#30478,#30479,#30480,#30481,#30482,#30483,#30484,#30485,#30486,#30487,#30488,
#30489,#30490,#30491,#30492,#30493,#30494,#30495,#30496,#30497,#30498,#30499,
#30500,#30501,#30502,#30503,#30504,#30505,#30506,#30507,#30508,#30509,#30510,
#30511,#30512,#30513,#30514,#30515,#30516,#30517,#30518,#30519,#30520,#30521,
#30522,#30523,#30524,#30525,#30526,#30527,#30528,#30529,#30530,#30531,#30532,
#30533,#30534,#30535,#30536,#30537,#30538,#30539,#30540,#30541,#30542,#30543,
#30544,#30545,#30546,#30547,#30548,#30549,#30550,#30551,#30552,#30553,#30554,
#30555,#30556,#30557,#30558,#30559,#30560,#30561,#30562,#30563,#30564,#30565,
#30566,#30567,#30568,#30569,#30570,#30571,#30572,#30573,#30574,#30575,#30576,
#30577,#30578,#30579,#30580,#30581,#30582,#30583,#30584,#30585,#30586,#30587,
#30588,#30589,#30590,#30591,#30592,#30593,#30594,#30595,#30596,#30597,#30598,
#30599,#30600,#30601,#30602,#30603,#30604,#30605,#30606,#30607,#30608,#30609,
#30610,#30611,#30612,#30613,#30614,#30615,#30616,#30617,#30618,#30619,#30620,
#30621,#30622,#30623,#30624,#30625,#30626,#30627,#30628,#30629,#30630,#30631,
#30632,#30633,#30634,#30635,#30636,#30637,#30638,#30639,#30640,#30641,#30642,
#30643,#30644,#30645,#30646,#30647,#30648,#30649,#30650,#30651,#30652,#30653,
#30654,#30655,#30656,#30657,#30658,#30659,#30660,#30661,#30662,#30663,#30664,
#30665,#30666,#30667,#30668,#30669,#30670,#30671,#30672,#30673,#30674,#30675,
#30676,#30677,#30678,#30679,#30680,#30681,#30682,#30683,#30684,#30685,#30686,
#30687,#30688,#30689,#30690,#30691,#30692,#30693,#30694,#30695,#30696,#30697,
#30698,#30699,#30700,#30701,#30702,#30703,#30704,#30705,#30706,#30707,#30708,
#30709,#30710,#30711,#30712,#30713,#30714,#30715,#30716,#30717,#30718,#30719,
#30720,#30721,#30722,#30723,#30724,#30725,#30726,#30727,#30728,#30729,#30730,
#30731,#30732,#30733,#30734,#30735,#30736,#30737,#30738,#30739,#30740,#30741,
#30742,#30743,#30744,#30745,#30746,#30747,#30748,#30749,#30750,#30751,#30752,
#30753,#30754,#30755,#30756,#30757)),.UNSPECIFIED.,.F.,.F.,.F.)
B_SPLINE_SURFACE_WITH_KNOTS((2,2),(3,2,2,2,2,2,2,2,2,2,2,2,2,2,2,2,2,2,
2,2,2,2,2,2,2,2,2,2,2,2,2,2,2,2,2,2,2,2,2,2,2,2,2,2,2,2,2,2,2,2,2,2,2,2,
2,2,2,2,2,2,2,2,2,2,2,2,2,2,2,2,2,2,2,2,2,2,2,2,2,2,2,2,2,2,2,2,2,2,2,2,
2,2,2,2,2,2,2,2,2,2,2,2,2,2,2,2,2,2,2,2,2,2,2,2,2,2,2,2,2,2,2,2,2,2,2,2,
2,2,2,2,2,2,2,2,2,2,2,2,2,2,2,2,2,2,2,2,2,2,2,2,2,2,2,2,2,2,2,2,2,3),(0.,
1.00001332089206),(0.,0.00617283950617284,0.0123456790123457,0.0185185185185185,
0.0246913580246914,0.0308641975308642,0.037037037037037,0.0432098765432099,
0.0493827160493827,0.0555555555555556,0.0617283950617284,0.0679012345679012,
0.0740740740740741,0.0802469135802469,0.0864197530864197,0.0925925925925926,
0.0987654320987654,0.104938271604938,0.111111111111111,0.117283950617284,
0.123456790123457,0.12962962962963,0.135802469135802,0.141975308641975,
0.148148148148148,0.154320987654321,0.160493827160494,0.166666666666667,
0.172839506172839,0.179012345679012,0.185185185185185,0.191358024691358,
0.197530864197531,0.203703703703704,0.209876543209877,0.216049382716049,
0.222222222222222,0.228395061728395,0.234567901234568,0.240740740740741,
0.246913580246914,0.253086419753086,0.259259259259259,0.265432098765432,
0.271604938271605,0.277777777777778,0.283950617283951,0.290123456790123,
0.296296296296296,0.302469135802469,0.308641975308642,0.314814814814815,
0.320987654320988,0.327160493827161,0.333333333333333,0.339506172839506,
0.345679012345679,0.351851851851852,0.358024691358025,0.364197530864198,
0.37037037037037,0.376543209876543,0.382716049382716,0.388888888888889,
0.395061728395062,0.401234567901235,0.407407407407407,0.41358024691358,
0.419753086419753,0.425925925925926,0.432098765432099,0.438271604938272,
0.444444444444444,0.450617283950617,0.45679012345679,0.462962962962963,
0.469135802469136,0.475308641975309,0.481481481481481,0.487654320987654,
0.493827160493827,0.5,0.506172839506173,0.512345679012346,0.518518518518518,
0.524691358024691,0.530864197530864,0.537037037037037,0.54320987654321,
0.549382716049383,0.555555555555556,0.561728395061728,0.567901234567901,
0.574074074074074,0.580246913580247,0.58641975308642,0.592592592592593,
0.598765432098765,0.604938271604938,0.611111111111111,0.617283950617284,
0.623456790123457,0.62962962962963,0.635802469135803,0.641975308641975,
0.648148148148148,0.654320987654321,0.660493827160494,0.666666666666667,
0.672839506172839,0.679012345679012,0.685185185185185,0.691358024691358,
0.697530864197531,0.703703703703704,0.709876543209877,0.716049382716049,
0.722222222222222,0.728395061728395,0.734567901234568,0.740740740740741,
0.746913580246914,0.753086419753086,0.759259259259259,0.765432098765432,
0.771604938271605,0.777777777777778,0.783950617283951,0.790123456790123,
0.796296296296296,0.802469135802469,0.808641975308642,0.814814814814815,
0.820987654320988,0.827160493827161,0.833333333333333,0.839506172839506,
0.845679012345679,0.851851851851852,0.858024691358025,0.864197530864197,
0.87037037037037,0.876543209876543,0.882716049382716,0.888888888888889,
0.895061728395062,0.901234567901235,0.907407407407407,0.91358024691358,
0.919753086419753,0.925925925925926,0.932098765432099,0.938271604938272,
0.944444444444444,0.950617283950617,0.95679012345679,0.962962962962963,
0.969135802469136,0.975308641975309,0.977791440774828),.UNSPECIFIED.)
GEOMETRIC_REPRESENTATION_ITEM()
RATIONAL_B_SPLINE_SURFACE(((1.,0.866025403784439,1.,0.866025403784439,1.,
0.866025403784439,1.,0.866025403784439,1.,0.866025403784439,1.,0.866025403784439,
1.,0.866025403784439,1.,0.866025403784439,1.,0.866025403784439,1.,0.866025403784439,
1.,0.866025403784439,1.,0.866025403784439,1.,0.866025403784439,1.,0.866025403784439,
1.,0.866025403784439,1.,0.866025403784439,1.,0.866025403784439,1.,0.866025403784439,
1.,0.866025403784439,1.,0.866025403784439,1.,0.866025403784439,1.,0.866025403784439,
1.,0.866025403784439,1.,0.866025403784439,1.,0.866025403784439,1.,0.866025403784439,
1.,0.866025403784439,1.,0.866025403784439,1.,0.866025403784439,1.,0.866025403784439,
1.,0.866025403784439,1.,0.866025403784439,1.,0.866025403784439,1.,0.866025403784439,
1.,0.866025403784439,1.,0.866025403784439,1.,0.866025403784439,1.,0.866025403784439,
1.,0.866025403784439,1.,0.866025403784439,1.,0.866025403784439,1.,0.866025403784439,
1.,0.866025403784439,1.,0.866025403784439,1.,0.866025403784439,1.,0.866025403784439,
1.,0.866025403784439,1.,0.866025403784439,1.,0.866025403784439,1.,0.866025403784439,
1.,0.866025403784439,1.,0.866025403784439,1.,0.866025403784439,1.,0.866025403784439,
1.,0.866025403784439,1.,0.866025403784439,1.,0.866025403784439,1.,0.866025403784439,
1.,0.866025403784439,1.,0.866025403784439,1.,0.866025403784439,1.,0.866025403784439,
1.,0.866025403784439,1.,0.866025403784439,1.,0.866025403784439,1.,0.866025403784439,
1.,0.866025403784439,1.,0.866025403784439,1.,0.866025403784439,1.,0.866025403784439,
1.,0.866025403784439,1.,0.866025403784439,1.,0.866025403784439,1.,0.866025403784439,
1.,0.866025403784439,1.,0.866025403784439,1.,0.866025403784439,1.,0.866025403784439,
1.,0.866025403784439,1.,0.866025403784439,1.,0.866025403784439,1.,0.866025403784439,
1.,0.866025403784439,1.,0.866025403784439,1.,0.866025403784439,1.,0.866025403784439,
1.,0.866025403784439,1.,0.866025403784439,1.,0.866025403784439,1.,0.866025403784439,
1.,0.866025403784439,1.,0.866025403784439,1.,0.866025403784439,1.,0.866025403784439,
1.,0.866025403784439,1.,0.866025403784439,1.,0.866025403784439,1.,0.866025403784439,
1.,0.866025403784439,1.,0.866025403784439,1.,0.866025403784439,1.,0.866025403784439,
1.,0.866025403784439,1.,0.866025403784439,1.,0.866025403784439,1.,0.866025403784439,
1.,0.866025403784439,1.,0.866025403784439,1.,0.866025403784439,1.,0.866025403784439,
1.,0.866025403784439,1.,0.866025403784439,1.,0.866025403784439,1.,0.866025403784439,
1.,0.866025403784439,1.,0.866025403784439,1.,0.866025403784439,1.,0.866025403784439,
1.,0.866025403784439,1.,0.866025403784439,1.,0.866025403784439,1.,0.866025403784439,
1.,0.866025403784439,1.,0.866025403784439,1.,0.866025403784439,1.,0.866025403784439,
1.,0.866025403784439,1.,0.866025403784439,1.,0.866025403784439,1.,0.866025403784439,
1.,0.866025403784439,1.,0.866025403784439,1.,0.866025403784439,1.,0.866025403784439,
1.,0.866025403784439,1.,0.866025403784439,1.,0.866025403784439,1.,0.866025403784439,
1.,0.866025403784439,1.,0.866025403784439,1.,0.866025403784439,1.,0.866025403784439,
1.,0.866025403784439,1.,0.866025403784439,1.,0.866025403784439,1.,0.866025403784439,
1.,0.866025403784439,1.,0.866025403784439,1.,0.866025403784439,1.,0.866025403784439,
1.,0.866025403784439,1.,0.866025403784439,1.,0.866025403784439,1.,0.866025403784439,
1.,0.866025403784439,1.,0.866025403784439,1.,0.866025403784439,1.,0.866025403784439,
1.,0.946113621402695,0.935574890499137),(1.,0.866025403784439,1.,0.866025403784439,
1.,0.866025403784439,1.,0.866025403784439,1.,0.866025403784439,1.,0.866025403784439,
1.,0.866025403784439,1.,0.866025403784439,1.,0.866025403784439,1.,0.866025403784439,
1.,0.866025403784439,1.,0.866025403784439,1.,0.866025403784439,1.,0.866025403784439,
1.,0.866025403784439,1.,0.866025403784439,1.,0.866025403784439,1.,0.866025403784439,
1.,0.866025403784439,1.,0.866025403784439,1.,0.866025403784439,1.,0.866025403784439,
1.,0.866025403784439,1.,0.866025403784439,1.,0.866025403784439,1.,0.866025403784439,
1.,0.866025403784439,1.,0.866025403784439,1.,0.866025403784439,1.,0.866025403784439,
1.,0.866025403784439,1.,0.866025403784439,1.,0.866025403784439,1.,0.866025403784439,
1.,0.866025403784439,1.,0.866025403784439,1.,0.866025403784439,1.,0.866025403784439,
1.,0.866025403784439,1.,0.866025403784439,1.,0.866025403784439,1.,0.866025403784439,
1.,0.866025403784439,1.,0.866025403784439,1.,0.866025403784439,1.,0.866025403784439,
1.,0.866025403784439,1.,0.866025403784439,1.,0.866025403784439,1.,0.866025403784439,
1.,0.866025403784439,1.,0.866025403784439,1.,0.866025403784439,1.,0.866025403784439,
1.,0.866025403784439,1.,0.866025403784439,1.,0.866025403784439,1.,0.866025403784439,
1.,0.866025403784439,1.,0.866025403784439,1.,0.866025403784439,1.,0.866025403784439,
1.,0.866025403784439,1.,0.866025403784439,1.,0.866025403784439,1.,0.866025403784439,
1.,0.866025403784439,1.,0.866025403784439,1.,0.866025403784439,1.,0.866025403784439,
1.,0.866025403784439,1.,0.866025403784439,1.,0.866025403784439,1.,0.866025403784439,
1.,0.866025403784439,1.,0.866025403784439,1.,0.866025403784439,1.,0.866025403784439,
1.,0.866025403784439,1.,0.866025403784439,1.,0.866025403784439,1.,0.866025403784439,
1.,0.866025403784439,1.,0.866025403784439,1.,0.866025403784439,1.,0.866025403784439,
1.,0.866025403784439,1.,0.866025403784439,1.,0.866025403784439,1.,0.866025403784439,
1.,0.866025403784439,1.,0.866025403784439,1.,0.866025403784439,1.,0.866025403784439,
1.,0.866025403784439,1.,0.866025403784439,1.,0.866025403784439,1.,0.866025403784439,
1.,0.866025403784439,1.,0.866025403784439,1.,0.866025403784439,1.,0.866025403784439,
1.,0.866025403784439,1.,0.866025403784439,1.,0.866025403784439,1.,0.866025403784439,
1.,0.866025403784439,1.,0.866025403784439,1.,0.866025403784439,1.,0.866025403784439,
1.,0.866025403784439,1.,0.866025403784439,1.,0.866025403784439,1.,0.866025403784439,
1.,0.866025403784439,1.,0.866025403784439,1.,0.866025403784439,1.,0.866025403784439,
1.,0.866025403784439,1.,0.866025403784439,1.,0.866025403784439,1.,0.866025403784439,
1.,0.866025403784439,1.,0.866025403784439,1.,0.866025403784439,1.,0.866025403784439,
1.,0.866025403784439,1.,0.866025403784439,1.,0.866025403784439,1.,0.866025403784439,
1.,0.866025403784439,1.,0.866025403784439,1.,0.866025403784439,1.,0.866025403784439,
1.,0.866025403784439,1.,0.866025403784439,1.,0.866025403784439,1.,0.866025403784439,
1.,0.866025403784439,1.,0.866025403784439,1.,0.866025403784439,1.,0.866025403784439,
1.,0.866025403784439,1.,0.866025403784439,1.,0.866025403784439,1.,0.866025403784439,
1.,0.866025403784439,1.,0.866025403784439,1.,0.866025403784439,1.,0.866025403784439,
1.,0.866025403784439,1.,0.866025403784439,1.,0.866025403784439,1.,0.866025403784439,
1.,0.866025403784439,1.,0.866025403784439,1.,0.866025403784439,1.,0.866025403784439,
1.,0.946113621402695,0.935574890499137)))
REPRESENTATION_ITEM('')
SURFACE()
);
#297=(
BOUNDED_SURFACE()
B_SPLINE_SURFACE(1,2,((#31063,#31064,#31065,#31066,#31067,#31068,#31069,
#31070,#31071,#31072,#31073,#31074,#31075,#31076,#31077,#31078,#31079,#31080,
#31081,#31082,#31083,#31084,#31085,#31086,#31087,#31088,#31089,#31090,#31091,
#31092,#31093,#31094,#31095,#31096,#31097,#31098,#31099,#31100,#31101,#31102,
#31103,#31104,#31105,#31106,#31107,#31108,#31109,#31110,#31111,#31112,#31113,
#31114,#31115,#31116,#31117,#31118,#31119,#31120,#31121,#31122,#31123,#31124,
#31125,#31126,#31127,#31128,#31129,#31130,#31131,#31132,#31133,#31134,#31135,
#31136,#31137,#31138,#31139,#31140,#31141,#31142,#31143,#31144,#31145,#31146,
#31147,#31148,#31149,#31150,#31151,#31152,#31153,#31154,#31155,#31156,#31157,
#31158,#31159,#31160,#31161,#31162,#31163,#31164,#31165,#31166,#31167,#31168,
#31169,#31170,#31171,#31172,#31173,#31174,#31175,#31176,#31177,#31178,#31179,
#31180,#31181,#31182,#31183,#31184,#31185,#31186,#31187,#31188,#31189,#31190,
#31191,#31192,#31193,#31194,#31195,#31196,#31197,#31198,#31199,#31200,#31201,
#31202,#31203,#31204,#31205,#31206,#31207,#31208,#31209,#31210,#31211,#31212,
#31213,#31214,#31215,#31216,#31217,#31218,#31219,#31220,#31221,#31222,#31223,
#31224,#31225,#31226,#31227,#31228,#31229,#31230,#31231,#31232,#31233,#31234,
#31235,#31236,#31237,#31238,#31239,#31240,#31241,#31242,#31243,#31244,#31245,
#31246,#31247,#31248,#31249,#31250,#31251,#31252,#31253,#31254,#31255,#31256,
#31257,#31258,#31259,#31260,#31261,#31262,#31263,#31264,#31265,#31266,#31267,
#31268,#31269,#31270,#31271,#31272,#31273,#31274,#31275,#31276,#31277,#31278,
#31279,#31280,#31281,#31282,#31283,#31284,#31285,#31286,#31287,#31288,#31289,
#31290,#31291,#31292,#31293,#31294,#31295,#31296,#31297,#31298,#31299,#31300,
#31301,#31302,#31303,#31304,#31305,#31306,#31307,#31308,#31309,#31310,#31311,
#31312,#31313,#31314,#31315,#31316,#31317,#31318,#31319,#31320,#31321,#31322,
#31323,#31324,#31325,#31326,#31327,#31328,#31329,#31330,#31331,#31332,#31333,
#31334,#31335,#31336,#31337,#31338,#31339,#31340,#31341,#31342,#31343,#31344,
#31345,#31346,#31347,#31348,#31349,#31350,#31351,#31352,#31353,#31354,#31355,
#31356,#31357,#31358,#31359,#31360,#31361,#31362,#31363,#31364,#31365,#31366,
#31367,#31368,#31369,#31370,#31371,#31372,#31373,#31374,#31375,#31376,#31377,
#31378,#31379,#31380,#31381,#31382,#31383),(#31384,#31385,#31386,#31387,
#31388,#31389,#31390,#31391,#31392,#31393,#31394,#31395,#31396,#31397,#31398,
#31399,#31400,#31401,#31402,#31403,#31404,#31405,#31406,#31407,#31408,#31409,
#31410,#31411,#31412,#31413,#31414,#31415,#31416,#31417,#31418,#31419,#31420,
#31421,#31422,#31423,#31424,#31425,#31426,#31427,#31428,#31429,#31430,#31431,
#31432,#31433,#31434,#31435,#31436,#31437,#31438,#31439,#31440,#31441,#31442,
#31443,#31444,#31445,#31446,#31447,#31448,#31449,#31450,#31451,#31452,#31453,
#31454,#31455,#31456,#31457,#31458,#31459,#31460,#31461,#31462,#31463,#31464,
#31465,#31466,#31467,#31468,#31469,#31470,#31471,#31472,#31473,#31474,#31475,
#31476,#31477,#31478,#31479,#31480,#31481,#31482,#31483,#31484,#31485,#31486,
#31487,#31488,#31489,#31490,#31491,#31492,#31493,#31494,#31495,#31496,#31497,
#31498,#31499,#31500,#31501,#31502,#31503,#31504,#31505,#31506,#31507,#31508,
#31509,#31510,#31511,#31512,#31513,#31514,#31515,#31516,#31517,#31518,#31519,
#31520,#31521,#31522,#31523,#31524,#31525,#31526,#31527,#31528,#31529,#31530,
#31531,#31532,#31533,#31534,#31535,#31536,#31537,#31538,#31539,#31540,#31541,
#31542,#31543,#31544,#31545,#31546,#31547,#31548,#31549,#31550,#31551,#31552,
#31553,#31554,#31555,#31556,#31557,#31558,#31559,#31560,#31561,#31562,#31563,
#31564,#31565,#31566,#31567,#31568,#31569,#31570,#31571,#31572,#31573,#31574,
#31575,#31576,#31577,#31578,#31579,#31580,#31581,#31582,#31583,#31584,#31585,
#31586,#31587,#31588,#31589,#31590,#31591,#31592,#31593,#31594,#31595,#31596,
#31597,#31598,#31599,#31600,#31601,#31602,#31603,#31604,#31605,#31606,#31607,
#31608,#31609,#31610,#31611,#31612,#31613,#31614,#31615,#31616,#31617,#31618,
#31619,#31620,#31621,#31622,#31623,#31624,#31625,#31626,#31627,#31628,#31629,
#31630,#31631,#31632,#31633,#31634,#31635,#31636,#31637,#31638,#31639,#31640,
#31641,#31642,#31643,#31644,#31645,#31646,#31647,#31648,#31649,#31650,#31651,
#31652,#31653,#31654,#31655,#31656,#31657,#31658,#31659,#31660,#31661,#31662,
#31663,#31664,#31665,#31666,#31667,#31668,#31669,#31670,#31671,#31672,#31673,
#31674,#31675,#31676,#31677,#31678,#31679,#31680,#31681,#31682,#31683,#31684,
#31685,#31686,#31687,#31688,#31689,#31690,#31691,#31692,#31693,#31694,#31695,
#31696,#31697,#31698,#31699,#31700,#31701,#31702,#31703,#31704)),
 .UNSPECIFIED.,.F.,.F.,.F.)
B_SPLINE_SURFACE_WITH_KNOTS((2,2),(3,2,2,2,2,2,2,2,2,2,2,2,2,2,2,2,2,2,
2,2,2,2,2,2,2,2,2,2,2,2,2,2,2,2,2,2,2,2,2,2,2,2,2,2,2,2,2,2,2,2,2,2,2,2,
2,2,2,2,2,2,2,2,2,2,2,2,2,2,2,2,2,2,2,2,2,2,2,2,2,2,2,2,2,2,2,2,2,2,2,2,
2,2,2,2,2,2,2,2,2,2,2,2,2,2,2,2,2,2,2,2,2,2,2,2,2,2,2,2,2,2,2,2,2,2,2,2,
2,2,2,2,2,2,2,2,2,2,2,2,2,2,2,2,2,2,2,2,2,2,2,2,2,2,2,2,2,2,2,2,2,2,3),
(-0.000321975171240591,1.),(0.,0.00617283950617284,0.0123456790123457,0.0185185185185185,
0.0246913580246914,0.0308641975308642,0.037037037037037,0.0432098765432099,
0.0493827160493827,0.0555555555555556,0.0617283950617284,0.0679012345679012,
0.0740740740740741,0.0802469135802469,0.0864197530864197,0.0925925925925926,
0.0987654320987654,0.104938271604938,0.111111111111111,0.117283950617284,
0.123456790123457,0.12962962962963,0.135802469135802,0.141975308641975,
0.148148148148148,0.154320987654321,0.160493827160494,0.166666666666667,
0.172839506172839,0.179012345679012,0.185185185185185,0.191358024691358,
0.197530864197531,0.203703703703704,0.209876543209877,0.216049382716049,
0.222222222222222,0.228395061728395,0.234567901234568,0.240740740740741,
0.246913580246914,0.253086419753086,0.259259259259259,0.265432098765432,
0.271604938271605,0.277777777777778,0.283950617283951,0.290123456790123,
0.296296296296296,0.302469135802469,0.308641975308642,0.314814814814815,
0.320987654320988,0.327160493827161,0.333333333333333,0.339506172839506,
0.345679012345679,0.351851851851852,0.358024691358025,0.364197530864198,
0.37037037037037,0.376543209876543,0.382716049382716,0.388888888888889,
0.395061728395062,0.401234567901235,0.407407407407407,0.41358024691358,
0.419753086419753,0.425925925925926,0.432098765432099,0.438271604938272,
0.444444444444444,0.450617283950617,0.45679012345679,0.462962962962963,
0.469135802469136,0.475308641975309,0.481481481481481,0.487654320987654,
0.493827160493827,0.5,0.506172839506173,0.512345679012346,0.518518518518518,
0.524691358024691,0.530864197530864,0.537037037037037,0.54320987654321,
0.549382716049383,0.555555555555556,0.561728395061728,0.567901234567901,
0.574074074074074,0.580246913580247,0.58641975308642,0.592592592592593,
0.598765432098765,0.604938271604938,0.611111111111111,0.617283950617284,
0.623456790123457,0.62962962962963,0.635802469135803,0.641975308641975,
0.648148148148148,0.654320987654321,0.660493827160494,0.666666666666667,
0.672839506172839,0.679012345679012,0.685185185185185,0.691358024691358,
0.697530864197531,0.703703703703704,0.709876543209877,0.716049382716049,
0.722222222222222,0.728395061728395,0.734567901234568,0.740740740740741,
0.746913580246914,0.753086419753086,0.759259259259259,0.765432098765432,
0.771604938271605,0.777777777777778,0.783950617283951,0.790123456790123,
0.796296296296296,0.802469135802469,0.808641975308642,0.814814814814815,
0.820987654320988,0.827160493827161,0.833333333333333,0.839506172839506,
0.845679012345679,0.851851851851852,0.858024691358025,0.864197530864197,
0.87037037037037,0.876543209876543,0.882716049382716,0.888888888888889,
0.895061728395062,0.901234567901235,0.907407407407407,0.91358024691358,
0.919753086419753,0.925925925925926,0.932098765432099,0.938271604938272,
0.944444444444444,0.950617283950617,0.95679012345679,0.962962962962963,
0.969135802469136,0.975308641975309,0.977791393533952,0.987569307469292),
 .UNSPECIFIED.)
GEOMETRIC_REPRESENTATION_ITEM()
RATIONAL_B_SPLINE_SURFACE(((1.,0.866025403784439,1.,0.866025403784439,1.,
0.866025403784439,1.,0.866025403784439,1.,0.866025403784439,1.,0.866025403784439,
1.,0.866025403784439,1.,0.866025403784439,1.,0.866025403784439,1.,0.866025403784439,
1.,0.866025403784439,1.,0.866025403784439,1.,0.866025403784439,1.,0.866025403784439,
1.,0.866025403784439,1.,0.866025403784439,1.,0.866025403784439,1.,0.866025403784439,
1.,0.866025403784439,1.,0.866025403784439,1.,0.866025403784439,1.,0.866025403784439,
1.,0.866025403784439,1.,0.866025403784439,1.,0.866025403784439,1.,0.866025403784439,
1.,0.866025403784439,1.,0.866025403784439,1.,0.866025403784439,1.,0.866025403784439,
1.,0.866025403784439,1.,0.866025403784439,1.,0.866025403784439,1.,0.866025403784439,
1.,0.866025403784439,1.,0.866025403784439,1.,0.866025403784439,1.,0.866025403784439,
1.,0.866025403784439,1.,0.866025403784439,1.,0.866025403784439,1.,0.866025403784439,
1.,0.866025403784439,1.,0.866025403784439,1.,0.866025403784439,1.,0.866025403784439,
1.,0.866025403784439,1.,0.866025403784439,1.,0.866025403784439,1.,0.866025403784439,
1.,0.866025403784439,1.,0.866025403784439,1.,0.866025403784439,1.,0.866025403784439,
1.,0.866025403784439,1.,0.866025403784439,1.,0.866025403784439,1.,0.866025403784439,
1.,0.866025403784439,1.,0.866025403784439,1.,0.866025403784439,1.,0.866025403784439,
1.,0.866025403784439,1.,0.866025403784439,1.,0.866025403784439,1.,0.866025403784439,
1.,0.866025403784439,1.,0.866025403784439,1.,0.866025403784439,1.,0.866025403784439,
1.,0.866025403784439,1.,0.866025403784439,1.,0.866025403784439,1.,0.866025403784439,
1.,0.866025403784439,1.,0.866025403784439,1.,0.866025403784439,1.,0.866025403784439,
1.,0.866025403784439,1.,0.866025403784439,1.,0.866025403784439,1.,0.866025403784439,
1.,0.866025403784439,1.,0.866025403784439,1.,0.866025403784439,1.,0.866025403784439,
1.,0.866025403784439,1.,0.866025403784439,1.,0.866025403784439,1.,0.866025403784439,
1.,0.866025403784439,1.,0.866025403784439,1.,0.866025403784439,1.,0.866025403784439,
1.,0.866025403784439,1.,0.866025403784439,1.,0.866025403784439,1.,0.866025403784439,
1.,0.866025403784439,1.,0.866025403784439,1.,0.866025403784439,1.,0.866025403784439,
1.,0.866025403784439,1.,0.866025403784439,1.,0.866025403784439,1.,0.866025403784439,
1.,0.866025403784439,1.,0.866025403784439,1.,0.866025403784439,1.,0.866025403784439,
1.,0.866025403784439,1.,0.866025403784439,1.,0.866025403784439,1.,0.866025403784439,
1.,0.866025403784439,1.,0.866025403784439,1.,0.866025403784439,1.,0.866025403784439,
1.,0.866025403784439,1.,0.866025403784439,1.,0.866025403784439,1.,0.866025403784439,
1.,0.866025403784439,1.,0.866025403784439,1.,0.866025403784439,1.,0.866025403784439,
1.,0.866025403784439,1.,0.866025403784439,1.,0.866025403784439,1.,0.866025403784439,
1.,0.866025403784439,1.,0.866025403784439,1.,0.866025403784439,1.,0.866025403784439,
1.,0.866025403784439,1.,0.866025403784439,1.,0.866025403784439,1.,0.866025403784439,
1.,0.866025403784439,1.,0.866025403784439,1.,0.866025403784439,1.,0.866025403784439,
1.,0.866025403784439,1.,0.866025403784439,1.,0.866025403784439,1.,0.866025403784439,
1.,0.866025403784439,1.,0.866025403784439,1.,0.866025403784439,1.,0.866025403784439,
1.,0.866025403784439,1.,0.866025403784439,1.,0.866025403784439,1.,0.866025403784439,
1.,0.866025403784439,1.,0.866025403784439,1.,0.866025403784439,1.,0.866025403784439,
1.,0.946114646713198,0.93557529156132,0.93557529156132,0.93557529156132),
(1.,0.866025403784439,1.,0.866025403784439,1.,0.866025403784439,1.,0.866025403784439,
1.,0.866025403784439,1.,0.866025403784439,1.,0.866025403784439,1.,0.866025403784439,
1.,0.866025403784439,1.,0.866025403784439,1.,0.866025403784439,1.,0.866025403784439,
1.,0.866025403784439,1.,0.866025403784439,1.,0.866025403784439,1.,0.866025403784439,
1.,0.866025403784439,1.,0.866025403784439,1.,0.866025403784439,1.,0.866025403784439,
1.,0.866025403784439,1.,0.866025403784439,1.,0.866025403784439,1.,0.866025403784439,
1.,0.866025403784439,1.,0.866025403784439,1.,0.866025403784439,1.,0.866025403784439,
1.,0.866025403784439,1.,0.866025403784439,1.,0.866025403784439,1.,0.866025403784439,
1.,0.866025403784439,1.,0.866025403784439,1.,0.866025403784439,1.,0.866025403784439,
1.,0.866025403784439,1.,0.866025403784439,1.,0.866025403784439,1.,0.866025403784439,
1.,0.866025403784439,1.,0.866025403784439,1.,0.866025403784439,1.,0.866025403784439,
1.,0.866025403784439,1.,0.866025403784439,1.,0.866025403784439,1.,0.866025403784439,
1.,0.866025403784439,1.,0.866025403784439,1.,0.866025403784439,1.,0.866025403784439,
1.,0.866025403784439,1.,0.866025403784439,1.,0.866025403784439,1.,0.866025403784439,
1.,0.866025403784439,1.,0.866025403784439,1.,0.866025403784439,1.,0.866025403784439,
1.,0.866025403784439,1.,0.866025403784439,1.,0.866025403784439,1.,0.866025403784439,
1.,0.866025403784439,1.,0.866025403784439,1.,0.866025403784439,1.,0.866025403784439,
1.,0.866025403784439,1.,0.866025403784439,1.,0.866025403784439,1.,0.866025403784439,
1.,0.866025403784439,1.,0.866025403784439,1.,0.866025403784439,1.,0.866025403784439,
1.,0.866025403784439,1.,0.866025403784439,1.,0.866025403784439,1.,0.866025403784439,
1.,0.866025403784439,1.,0.866025403784439,1.,0.866025403784439,1.,0.866025403784439,
1.,0.866025403784439,1.,0.866025403784439,1.,0.866025403784439,1.,0.866025403784439,
1.,0.866025403784439,1.,0.866025403784439,1.,0.866025403784439,1.,0.866025403784439,
1.,0.866025403784439,1.,0.866025403784439,1.,0.866025403784439,1.,0.866025403784439,
1.,0.866025403784439,1.,0.866025403784439,1.,0.866025403784439,1.,0.866025403784439,
1.,0.866025403784439,1.,0.866025403784439,1.,0.866025403784439,1.,0.866025403784439,
1.,0.866025403784439,1.,0.866025403784439,1.,0.866025403784439,1.,0.866025403784439,
1.,0.866025403784439,1.,0.866025403784439,1.,0.866025403784439,1.,0.866025403784439,
1.,0.866025403784439,1.,0.866025403784439,1.,0.866025403784439,1.,0.866025403784439,
1.,0.866025403784439,1.,0.866025403784439,1.,0.866025403784439,1.,0.866025403784439,
1.,0.866025403784439,1.,0.866025403784439,1.,0.866025403784439,1.,0.866025403784439,
1.,0.866025403784439,1.,0.866025403784439,1.,0.866025403784439,1.,0.866025403784439,
1.,0.866025403784439,1.,0.866025403784439,1.,0.866025403784439,1.,0.866025403784439,
1.,0.866025403784439,1.,0.866025403784439,1.,0.866025403784439,1.,0.866025403784439,
1.,0.866025403784439,1.,0.866025403784439,1.,0.866025403784439,1.,0.866025403784439,
1.,0.866025403784439,1.,0.866025403784439,1.,0.866025403784439,1.,0.866025403784439,
1.,0.866025403784439,1.,0.866025403784439,1.,0.866025403784439,1.,0.866025403784439,
1.,0.866025403784439,1.,0.866025403784439,1.,0.866025403784439,1.,0.866025403784439,
1.,0.866025403784439,1.,0.866025403784439,1.,0.866025403784439,1.,0.866025403784439,
1.,0.866025403784439,1.,0.866025403784439,1.,0.946114646713198,0.93557529156132,
0.93557529156132,0.93557529156132)))
REPRESENTATION_ITEM('')
SURFACE()
);
#298=(
BOUNDED_SURFACE()
B_SPLINE_SURFACE(1,2,((#31705,#31706,#31707,#31708,#31709,#31710,#31711,
#31712,#31713,#31714,#31715,#31716,#31717,#31718,#31719,#31720,#31721,#31722,
#31723,#31724,#31725,#31726,#31727,#31728,#31729,#31730,#31731,#31732,#31733,
#31734,#31735,#31736,#31737,#31738,#31739,#31740,#31741,#31742,#31743,#31744,
#31745,#31746,#31747,#31748,#31749,#31750,#31751,#31752,#31753,#31754,#31755,
#31756,#31757,#31758,#31759,#31760,#31761,#31762,#31763,#31764,#31765,#31766,
#31767,#31768,#31769,#31770,#31771,#31772,#31773,#31774,#31775,#31776,#31777,
#31778,#31779,#31780,#31781,#31782,#31783,#31784,#31785,#31786,#31787,#31788,
#31789,#31790,#31791,#31792,#31793,#31794,#31795,#31796,#31797,#31798,#31799,
#31800,#31801,#31802,#31803,#31804,#31805,#31806,#31807,#31808,#31809,#31810,
#31811,#31812,#31813,#31814,#31815,#31816,#31817,#31818,#31819,#31820,#31821,
#31822,#31823,#31824,#31825,#31826,#31827,#31828,#31829,#31830,#31831,#31832,
#31833,#31834,#31835,#31836,#31837,#31838,#31839,#31840,#31841,#31842,#31843,
#31844,#31845,#31846,#31847,#31848,#31849,#31850,#31851,#31852,#31853,#31854,
#31855,#31856,#31857,#31858,#31859,#31860,#31861,#31862,#31863,#31864,#31865,
#31866,#31867,#31868,#31869,#31870,#31871,#31872,#31873,#31874,#31875,#31876,
#31877,#31878,#31879,#31880,#31881,#31882,#31883,#31884,#31885,#31886,#31887,
#31888,#31889,#31890,#31891,#31892,#31893,#31894,#31895,#31896,#31897,#31898,
#31899,#31900,#31901,#31902,#31903,#31904,#31905,#31906,#31907,#31908,#31909,
#31910,#31911,#31912,#31913,#31914,#31915,#31916,#31917,#31918,#31919,#31920,
#31921,#31922,#31923,#31924,#31925,#31926,#31927,#31928,#31929,#31930,#31931,
#31932,#31933,#31934,#31935,#31936,#31937,#31938,#31939,#31940,#31941,#31942,
#31943,#31944,#31945,#31946,#31947,#31948,#31949,#31950,#31951,#31952,#31953,
#31954,#31955,#31956,#31957,#31958,#31959,#31960,#31961,#31962,#31963,#31964,
#31965,#31966,#31967,#31968,#31969,#31970,#31971,#31972,#31973,#31974,#31975,
#31976,#31977,#31978,#31979,#31980,#31981,#31982,#31983,#31984,#31985,#31986,
#31987,#31988,#31989,#31990,#31991,#31992,#31993,#31994,#31995,#31996,#31997,
#31998,#31999,#32000,#32001,#32002,#32003,#32004,#32005,#32006,#32007,#32008,
#32009,#32010,#32011,#32012,#32013,#32014,#32015,#32016,#32017,#32018,#32019,
#32020,#32021,#32022,#32023),(#32024,#32025,#32026,#32027,#32028,#32029,
#32030,#32031,#32032,#32033,#32034,#32035,#32036,#32037,#32038,#32039,#32040,
#32041,#32042,#32043,#32044,#32045,#32046,#32047,#32048,#32049,#32050,#32051,
#32052,#32053,#32054,#32055,#32056,#32057,#32058,#32059,#32060,#32061,#32062,
#32063,#32064,#32065,#32066,#32067,#32068,#32069,#32070,#32071,#32072,#32073,
#32074,#32075,#32076,#32077,#32078,#32079,#32080,#32081,#32082,#32083,#32084,
#32085,#32086,#32087,#32088,#32089,#32090,#32091,#32092,#32093,#32094,#32095,
#32096,#32097,#32098,#32099,#32100,#32101,#32102,#32103,#32104,#32105,#32106,
#32107,#32108,#32109,#32110,#32111,#32112,#32113,#32114,#32115,#32116,#32117,
#32118,#32119,#32120,#32121,#32122,#32123,#32124,#32125,#32126,#32127,#32128,
#32129,#32130,#32131,#32132,#32133,#32134,#32135,#32136,#32137,#32138,#32139,
#32140,#32141,#32142,#32143,#32144,#32145,#32146,#32147,#32148,#32149,#32150,
#32151,#32152,#32153,#32154,#32155,#32156,#32157,#32158,#32159,#32160,#32161,
#32162,#32163,#32164,#32165,#32166,#32167,#32168,#32169,#32170,#32171,#32172,
#32173,#32174,#32175,#32176,#32177,#32178,#32179,#32180,#32181,#32182,#32183,
#32184,#32185,#32186,#32187,#32188,#32189,#32190,#32191,#32192,#32193,#32194,
#32195,#32196,#32197,#32198,#32199,#32200,#32201,#32202,#32203,#32204,#32205,
#32206,#32207,#32208,#32209,#32210,#32211,#32212,#32213,#32214,#32215,#32216,
#32217,#32218,#32219,#32220,#32221,#32222,#32223,#32224,#32225,#32226,#32227,
#32228,#32229,#32230,#32231,#32232,#32233,#32234,#32235,#32236,#32237,#32238,
#32239,#32240,#32241,#32242,#32243,#32244,#32245,#32246,#32247,#32248,#32249,
#32250,#32251,#32252,#32253,#32254,#32255,#32256,#32257,#32258,#32259,#32260,
#32261,#32262,#32263,#32264,#32265,#32266,#32267,#32268,#32269,#32270,#32271,
#32272,#32273,#32274,#32275,#32276,#32277,#32278,#32279,#32280,#32281,#32282,
#32283,#32284,#32285,#32286,#32287,#32288,#32289,#32290,#32291,#32292,#32293,
#32294,#32295,#32296,#32297,#32298,#32299,#32300,#32301,#32302,#32303,#32304,
#32305,#32306,#32307,#32308,#32309,#32310,#32311,#32312,#32313,#32314,#32315,
#32316,#32317,#32318,#32319,#32320,#32321,#32322,#32323,#32324,#32325,#32326,
#32327,#32328,#32329,#32330,#32331,#32332,#32333,#32334,#32335,#32336,#32337,
#32338,#32339,#32340,#32341,#32342)),.UNSPECIFIED.,.F.,.F.,.F.)
B_SPLINE_SURFACE_WITH_KNOTS((2,2),(3,2,2,2,2,2,2,2,2,2,2,2,2,2,2,2,2,2,
2,2,2,2,2,2,2,2,2,2,2,2,2,2,2,2,2,2,2,2,2,2,2,2,2,2,2,2,2,2,2,2,2,2,2,2,
2,2,2,2,2,2,2,2,2,2,2,2,2,2,2,2,2,2,2,2,2,2,2,2,2,2,2,2,2,2,2,2,2,2,2,2,
2,2,2,2,2,2,2,2,2,2,2,2,2,2,2,2,2,2,2,2,2,2,2,2,2,2,2,2,2,2,2,2,2,2,2,2,
2,2,2,2,2,2,2,2,2,2,2,2,2,2,2,2,2,2,2,2,2,2,2,2,2,2,2,2,2,2,2,2,2,3),(-2.473386913217E-5,
1.),(0.,0.00617283950617284,0.0123456790123457,0.0185185185185185,0.0246913580246914,
0.0308641975308642,0.037037037037037,0.0432098765432099,0.0493827160493827,
0.0555555555555556,0.0617283950617284,0.0679012345679012,0.0740740740740741,
0.0802469135802469,0.0864197530864197,0.0925925925925926,0.0987654320987654,
0.104938271604938,0.111111111111111,0.117283950617284,0.123456790123457,
0.12962962962963,0.135802469135802,0.141975308641975,0.148148148148148,
0.154320987654321,0.160493827160494,0.166666666666667,0.172839506172839,
0.179012345679012,0.185185185185185,0.191358024691358,0.197530864197531,
0.203703703703704,0.209876543209877,0.216049382716049,0.222222222222222,
0.228395061728395,0.234567901234568,0.240740740740741,0.246913580246914,
0.253086419753086,0.259259259259259,0.265432098765432,0.271604938271605,
0.277777777777778,0.283950617283951,0.290123456790123,0.296296296296296,
0.302469135802469,0.308641975308642,0.314814814814815,0.320987654320988,
0.327160493827161,0.333333333333333,0.339506172839506,0.345679012345679,
0.351851851851852,0.358024691358025,0.364197530864198,0.37037037037037,
0.376543209876543,0.382716049382716,0.388888888888889,0.395061728395062,
0.401234567901235,0.407407407407407,0.41358024691358,0.419753086419753,
0.425925925925926,0.432098765432099,0.438271604938272,0.444444444444444,
0.450617283950617,0.45679012345679,0.462962962962963,0.469135802469136,
0.475308641975309,0.481481481481481,0.487654320987654,0.493827160493827,
0.5,0.506172839506173,0.512345679012346,0.518518518518518,0.524691358024691,
0.530864197530864,0.537037037037037,0.54320987654321,0.549382716049383,
0.555555555555556,0.561728395061728,0.567901234567901,0.574074074074074,
0.580246913580247,0.58641975308642,0.592592592592593,0.598765432098765,
0.604938271604938,0.611111111111111,0.617283950617284,0.623456790123457,
0.62962962962963,0.635802469135803,0.641975308641975,0.648148148148148,
0.654320987654321,0.660493827160494,0.666666666666667,0.672839506172839,
0.679012345679012,0.685185185185185,0.691358024691358,0.697530864197531,
0.703703703703704,0.709876543209877,0.716049382716049,0.722222222222222,
0.728395061728395,0.734567901234568,0.740740740740741,0.746913580246914,
0.753086419753086,0.759259259259259,0.765432098765432,0.771604938271605,
0.777777777777778,0.783950617283951,0.790123456790123,0.796296296296296,
0.802469135802469,0.808641975308642,0.814814814814815,0.820987654320988,
0.827160493827161,0.833333333333333,0.839506172839506,0.845679012345679,
0.851851851851852,0.858024691358025,0.864197530864197,0.87037037037037,
0.876543209876543,0.882716049382716,0.888888888888889,0.895061728395062,
0.901234567901235,0.907407407407407,0.91358024691358,0.919753086419753,
0.925925925925926,0.932098765432099,0.938271604938272,0.944444444444444,
0.950617283950617,0.95679012345679,0.962962962962963,0.969135802469136,
0.975308641975309,0.977791447664447),.UNSPECIFIED.)
GEOMETRIC_REPRESENTATION_ITEM()
RATIONAL_B_SPLINE_SURFACE(((1.,0.866025403784439,1.,0.866025403784439,1.,
0.866025403784439,1.,0.866025403784439,1.,0.866025403784439,1.,0.866025403784439,
1.,0.866025403784439,1.,0.866025403784439,1.,0.866025403784439,1.,0.866025403784439,
1.,0.866025403784439,1.,0.866025403784439,1.,0.866025403784439,1.,0.866025403784439,
1.,0.866025403784439,1.,0.866025403784439,1.,0.866025403784439,1.,0.866025403784439,
1.,0.866025403784439,1.,0.866025403784439,1.,0.866025403784439,1.,0.866025403784439,
1.,0.866025403784439,1.,0.866025403784439,1.,0.866025403784439,1.,0.866025403784439,
1.,0.866025403784439,1.,0.866025403784439,1.,0.866025403784439,1.,0.866025403784439,
1.,0.866025403784439,1.,0.866025403784439,1.,0.866025403784439,1.,0.866025403784439,
1.,0.866025403784439,1.,0.866025403784439,1.,0.866025403784439,1.,0.866025403784439,
1.,0.866025403784439,1.,0.866025403784439,1.,0.866025403784439,1.,0.866025403784439,
1.,0.866025403784439,1.,0.866025403784439,1.,0.866025403784439,1.,0.866025403784439,
1.,0.866025403784439,1.,0.866025403784439,1.,0.866025403784439,1.,0.866025403784439,
1.,0.866025403784439,1.,0.866025403784439,1.,0.866025403784439,1.,0.866025403784439,
1.,0.866025403784439,1.,0.866025403784439,1.,0.866025403784439,1.,0.866025403784439,
1.,0.866025403784439,1.,0.866025403784439,1.,0.866025403784439,1.,0.866025403784439,
1.,0.866025403784439,1.,0.866025403784439,1.,0.866025403784439,1.,0.866025403784439,
1.,0.866025403784439,1.,0.866025403784439,1.,0.866025403784439,1.,0.866025403784439,
1.,0.866025403784439,1.,0.866025403784439,1.,0.866025403784439,1.,0.866025403784439,
1.,0.866025403784439,1.,0.866025403784439,1.,0.866025403784439,1.,0.866025403784439,
1.,0.866025403784439,1.,0.866025403784439,1.,0.866025403784439,1.,0.866025403784439,
1.,0.866025403784439,1.,0.866025403784439,1.,0.866025403784439,1.,0.866025403784439,
1.,0.866025403784439,1.,0.866025403784439,1.,0.866025403784439,1.,0.866025403784439,
1.,0.866025403784439,1.,0.866025403784439,1.,0.866025403784439,1.,0.866025403784439,
1.,0.866025403784439,1.,0.866025403784439,1.,0.866025403784439,1.,0.866025403784439,
1.,0.866025403784439,1.,0.866025403784439,1.,0.866025403784439,1.,0.866025403784439,
1.,0.866025403784439,1.,0.866025403784439,1.,0.866025403784439,1.,0.866025403784439,
1.,0.866025403784439,1.,0.866025403784439,1.,0.866025403784439,1.,0.866025403784439,
1.,0.866025403784439,1.,0.866025403784439,1.,0.866025403784439,1.,0.866025403784439,
1.,0.866025403784439,1.,0.866025403784439,1.,0.866025403784439,1.,0.866025403784439,
1.,0.866025403784439,1.,0.866025403784439,1.,0.866025403784439,1.,0.866025403784439,
1.,0.866025403784439,1.,0.866025403784439,1.,0.866025403784439,1.,0.866025403784439,
1.,0.866025403784439,1.,0.866025403784439,1.,0.866025403784439,1.,0.866025403784439,
1.,0.866025403784439,1.,0.866025403784439,1.,0.866025403784439,1.,0.866025403784439,
1.,0.866025403784439,1.,0.866025403784439,1.,0.866025403784439,1.,0.866025403784439,
1.,0.866025403784439,1.,0.866025403784439,1.,0.866025403784439,1.,0.866025403784439,
1.,0.866025403784439,1.,0.866025403784439,1.,0.866025403784439,1.,0.866025403784439,
1.,0.866025403784439,1.,0.866025403784439,1.,0.866025403784439,1.,0.866025403784439,
1.,0.866025403784439,1.,0.866025403784439,1.,0.866025403784439,1.,0.866025403784439,
1.,0.866025403784439,1.,0.866025403784439,1.,0.866025403784439,1.,0.866025403784439,
1.,0.9461134718712,0.935574832010768),(1.,0.866025403784439,1.,0.866025403784439,
1.,0.866025403784439,1.,0.866025403784439,1.,0.866025403784439,1.,0.866025403784439,
1.,0.866025403784439,1.,0.866025403784439,1.,0.866025403784439,1.,0.866025403784439,
1.,0.866025403784439,1.,0.866025403784439,1.,0.866025403784439,1.,0.866025403784439,
1.,0.866025403784439,1.,0.866025403784439,1.,0.866025403784439,1.,0.866025403784439,
1.,0.866025403784439,1.,0.866025403784439,1.,0.866025403784439,1.,0.866025403784439,
1.,0.866025403784439,1.,0.866025403784439,1.,0.866025403784439,1.,0.866025403784439,
1.,0.866025403784439,1.,0.866025403784439,1.,0.866025403784439,1.,0.866025403784439,
1.,0.866025403784439,1.,0.866025403784439,1.,0.866025403784439,1.,0.866025403784439,
1.,0.866025403784439,1.,0.866025403784439,1.,0.866025403784439,1.,0.866025403784439,
1.,0.866025403784439,1.,0.866025403784439,1.,0.866025403784439,1.,0.866025403784439,
1.,0.866025403784439,1.,0.866025403784439,1.,0.866025403784439,1.,0.866025403784439,
1.,0.866025403784439,1.,0.866025403784439,1.,0.866025403784439,1.,0.866025403784439,
1.,0.866025403784439,1.,0.866025403784439,1.,0.866025403784439,1.,0.866025403784439,
1.,0.866025403784439,1.,0.866025403784439,1.,0.866025403784439,1.,0.866025403784439,
1.,0.866025403784439,1.,0.866025403784439,1.,0.866025403784439,1.,0.866025403784439,
1.,0.866025403784439,1.,0.866025403784439,1.,0.866025403784439,1.,0.866025403784439,
1.,0.866025403784439,1.,0.866025403784439,1.,0.866025403784439,1.,0.866025403784439,
1.,0.866025403784439,1.,0.866025403784439,1.,0.866025403784439,1.,0.866025403784439,
1.,0.866025403784439,1.,0.866025403784439,1.,0.866025403784439,1.,0.866025403784439,
1.,0.866025403784439,1.,0.866025403784439,1.,0.866025403784439,1.,0.866025403784439,
1.,0.866025403784439,1.,0.866025403784439,1.,0.866025403784439,1.,0.866025403784439,
1.,0.866025403784439,1.,0.866025403784439,1.,0.866025403784439,1.,0.866025403784439,
1.,0.866025403784439,1.,0.866025403784439,1.,0.866025403784439,1.,0.866025403784439,
1.,0.866025403784439,1.,0.866025403784439,1.,0.866025403784439,1.,0.866025403784439,
1.,0.866025403784439,1.,0.866025403784439,1.,0.866025403784439,1.,0.866025403784439,
1.,0.866025403784439,1.,0.866025403784439,1.,0.866025403784439,1.,0.866025403784439,
1.,0.866025403784439,1.,0.866025403784439,1.,0.866025403784439,1.,0.866025403784439,
1.,0.866025403784439,1.,0.866025403784439,1.,0.866025403784439,1.,0.866025403784439,
1.,0.866025403784439,1.,0.866025403784439,1.,0.866025403784439,1.,0.866025403784439,
1.,0.866025403784439,1.,0.866025403784439,1.,0.866025403784439,1.,0.866025403784439,
1.,0.866025403784439,1.,0.866025403784439,1.,0.866025403784439,1.,0.866025403784439,
1.,0.866025403784439,1.,0.866025403784439,1.,0.866025403784439,1.,0.866025403784439,
1.,0.866025403784439,1.,0.866025403784439,1.,0.866025403784439,1.,0.866025403784439,
1.,0.866025403784439,1.,0.866025403784439,1.,0.866025403784439,1.,0.866025403784439,
1.,0.866025403784439,1.,0.866025403784439,1.,0.866025403784439,1.,0.866025403784439,
1.,0.866025403784439,1.,0.866025403784439,1.,0.866025403784439,1.,0.866025403784439,
1.,0.866025403784439,1.,0.866025403784439,1.,0.866025403784439,1.,0.866025403784439,
1.,0.866025403784439,1.,0.866025403784439,1.,0.866025403784439,1.,0.866025403784439,
1.,0.866025403784439,1.,0.866025403784439,1.,0.866025403784439,1.,0.866025403784439,
1.,0.9461134718712,0.935574832010768)))
REPRESENTATION_ITEM('')
SURFACE()
);
#299=(
BOUNDED_SURFACE()
B_SPLINE_SURFACE(1,2,((#32646,#32647,#32648,#32649,#32650,#32651,#32652,
#32653,#32654,#32655,#32656,#32657,#32658,#32659,#32660,#32661,#32662,#32663,
#32664,#32665,#32666,#32667,#32668,#32669,#32670,#32671,#32672,#32673,#32674,
#32675,#32676,#32677,#32678,#32679,#32680,#32681,#32682,#32683,#32684,#32685,
#32686,#32687,#32688,#32689,#32690,#32691,#32692,#32693,#32694,#32695,#32696,
#32697,#32698,#32699,#32700,#32701,#32702,#32703,#32704,#32705,#32706,#32707,
#32708,#32709,#32710,#32711,#32712,#32713,#32714,#32715,#32716,#32717,#32718,
#32719,#32720,#32721,#32722,#32723,#32724,#32725,#32726,#32727,#32728,#32729,
#32730,#32731,#32732,#32733,#32734,#32735,#32736,#32737,#32738,#32739,#32740,
#32741,#32742,#32743,#32744,#32745,#32746,#32747,#32748,#32749,#32750,#32751,
#32752,#32753,#32754,#32755,#32756,#32757,#32758,#32759,#32760,#32761,#32762,
#32763,#32764,#32765,#32766,#32767,#32768,#32769,#32770,#32771,#32772,#32773,
#32774,#32775,#32776,#32777,#32778,#32779,#32780,#32781,#32782,#32783,#32784,
#32785,#32786,#32787,#32788,#32789,#32790,#32791,#32792,#32793,#32794,#32795,
#32796,#32797,#32798,#32799,#32800,#32801,#32802,#32803,#32804,#32805,#32806,
#32807,#32808,#32809,#32810,#32811,#32812,#32813,#32814,#32815,#32816,#32817,
#32818,#32819,#32820,#32821,#32822,#32823,#32824,#32825,#32826,#32827,#32828,
#32829,#32830,#32831,#32832,#32833,#32834,#32835,#32836,#32837,#32838,#32839,
#32840,#32841,#32842,#32843,#32844,#32845,#32846,#32847,#32848,#32849,#32850,
#32851,#32852,#32853,#32854,#32855,#32856,#32857,#32858,#32859,#32860,#32861,
#32862,#32863,#32864,#32865,#32866,#32867,#32868,#32869,#32870,#32871,#32872,
#32873,#32874,#32875,#32876,#32877,#32878,#32879,#32880,#32881,#32882,#32883,
#32884,#32885,#32886,#32887,#32888,#32889,#32890,#32891,#32892,#32893,#32894,
#32895,#32896,#32897,#32898,#32899,#32900,#32901,#32902,#32903,#32904,#32905,
#32906,#32907,#32908,#32909,#32910,#32911,#32912,#32913,#32914,#32915,#32916,
#32917,#32918,#32919,#32920,#32921,#32922,#32923,#32924,#32925,#32926,#32927,
#32928,#32929,#32930,#32931,#32932,#32933,#32934,#32935,#32936,#32937,#32938,
#32939,#32940,#32941,#32942,#32943,#32944,#32945,#32946,#32947,#32948,#32949,
#32950,#32951,#32952,#32953,#32954,#32955,#32956,#32957,#32958,#32959,#32960,
#32961,#32962,#32963,#32964),(#32965,#32966,#32967,#32968,#32969,#32970,
#32971,#32972,#32973,#32974,#32975,#32976,#32977,#32978,#32979,#32980,#32981,
#32982,#32983,#32984,#32985,#32986,#32987,#32988,#32989,#32990,#32991,#32992,
#32993,#32994,#32995,#32996,#32997,#32998,#32999,#33000,#33001,#33002,#33003,
#33004,#33005,#33006,#33007,#33008,#33009,#33010,#33011,#33012,#33013,#33014,
#33015,#33016,#33017,#33018,#33019,#33020,#33021,#33022,#33023,#33024,#33025,
#33026,#33027,#33028,#33029,#33030,#33031,#33032,#33033,#33034,#33035,#33036,
#33037,#33038,#33039,#33040,#33041,#33042,#33043,#33044,#33045,#33046,#33047,
#33048,#33049,#33050,#33051,#33052,#33053,#33054,#33055,#33056,#33057,#33058,
#33059,#33060,#33061,#33062,#33063,#33064,#33065,#33066,#33067,#33068,#33069,
#33070,#33071,#33072,#33073,#33074,#33075,#33076,#33077,#33078,#33079,#33080,
#33081,#33082,#33083,#33084,#33085,#33086,#33087,#33088,#33089,#33090,#33091,
#33092,#33093,#33094,#33095,#33096,#33097,#33098,#33099,#33100,#33101,#33102,
#33103,#33104,#33105,#33106,#33107,#33108,#33109,#33110,#33111,#33112,#33113,
#33114,#33115,#33116,#33117,#33118,#33119,#33120,#33121,#33122,#33123,#33124,
#33125,#33126,#33127,#33128,#33129,#33130,#33131,#33132,#33133,#33134,#33135,
#33136,#33137,#33138,#33139,#33140,#33141,#33142,#33143,#33144,#33145,#33146,
#33147,#33148,#33149,#33150,#33151,#33152,#33153,#33154,#33155,#33156,#33157,
#33158,#33159,#33160,#33161,#33162,#33163,#33164,#33165,#33166,#33167,#33168,
#33169,#33170,#33171,#33172,#33173,#33174,#33175,#33176,#33177,#33178,#33179,
#33180,#33181,#33182,#33183,#33184,#33185,#33186,#33187,#33188,#33189,#33190,
#33191,#33192,#33193,#33194,#33195,#33196,#33197,#33198,#33199,#33200,#33201,
#33202,#33203,#33204,#33205,#33206,#33207,#33208,#33209,#33210,#33211,#33212,
#33213,#33214,#33215,#33216,#33217,#33218,#33219,#33220,#33221,#33222,#33223,
#33224,#33225,#33226,#33227,#33228,#33229,#33230,#33231,#33232,#33233,#33234,
#33235,#33236,#33237,#33238,#33239,#33240,#33241,#33242,#33243,#33244,#33245,
#33246,#33247,#33248,#33249,#33250,#33251,#33252,#33253,#33254,#33255,#33256,
#33257,#33258,#33259,#33260,#33261,#33262,#33263,#33264,#33265,#33266,#33267,
#33268,#33269,#33270,#33271,#33272,#33273,#33274,#33275,#33276,#33277,#33278,
#33279,#33280,#33281,#33282,#33283)),.UNSPECIFIED.,.F.,.F.,.F.)
B_SPLINE_SURFACE_WITH_KNOTS((2,2),(3,2,2,2,2,2,2,2,2,2,2,2,2,2,2,2,2,2,
2,2,2,2,2,2,2,2,2,2,2,2,2,2,2,2,2,2,2,2,2,2,2,2,2,2,2,2,2,2,2,2,2,2,2,2,
2,2,2,2,2,2,2,2,2,2,2,2,2,2,2,2,2,2,2,2,2,2,2,2,2,2,2,2,2,2,2,2,2,2,2,2,
2,2,2,2,2,2,2,2,2,2,2,2,2,2,2,2,2,2,2,2,2,2,2,2,2,2,2,2,2,2,2,2,2,2,2,2,
2,2,2,2,2,2,2,2,2,2,2,2,2,2,2,2,2,2,2,2,2,2,2,2,2,2,2,2,2,2,2,2,2,3),(0.,
1.00001332089252),(0.,0.00617283950617284,0.0123456790123457,0.0185185185185185,
0.0246913580246914,0.0308641975308642,0.037037037037037,0.0432098765432099,
0.0493827160493827,0.0555555555555556,0.0617283950617284,0.0679012345679012,
0.0740740740740741,0.0802469135802469,0.0864197530864197,0.0925925925925926,
0.0987654320987654,0.104938271604938,0.111111111111111,0.117283950617284,
0.123456790123457,0.12962962962963,0.135802469135802,0.141975308641975,
0.148148148148148,0.154320987654321,0.160493827160494,0.166666666666667,
0.172839506172839,0.179012345679012,0.185185185185185,0.191358024691358,
0.197530864197531,0.203703703703704,0.209876543209877,0.216049382716049,
0.222222222222222,0.228395061728395,0.234567901234568,0.240740740740741,
0.246913580246914,0.253086419753086,0.259259259259259,0.265432098765432,
0.271604938271605,0.277777777777778,0.283950617283951,0.290123456790123,
0.296296296296296,0.302469135802469,0.308641975308642,0.314814814814815,
0.320987654320988,0.327160493827161,0.333333333333333,0.339506172839506,
0.345679012345679,0.351851851851852,0.358024691358025,0.364197530864198,
0.37037037037037,0.376543209876543,0.382716049382716,0.388888888888889,
0.395061728395062,0.401234567901235,0.407407407407407,0.41358024691358,
0.419753086419753,0.425925925925926,0.432098765432099,0.438271604938272,
0.444444444444444,0.450617283950617,0.45679012345679,0.462962962962963,
0.469135802469136,0.475308641975309,0.481481481481481,0.487654320987654,
0.493827160493827,0.5,0.506172839506173,0.512345679012346,0.518518518518518,
0.524691358024691,0.530864197530864,0.537037037037037,0.54320987654321,
0.549382716049383,0.555555555555556,0.561728395061728,0.567901234567901,
0.574074074074074,0.580246913580247,0.58641975308642,0.592592592592593,
0.598765432098765,0.604938271604938,0.611111111111111,0.617283950617284,
0.623456790123457,0.62962962962963,0.635802469135803,0.641975308641975,
0.648148148148148,0.654320987654321,0.660493827160494,0.666666666666667,
0.672839506172839,0.679012345679012,0.685185185185185,0.691358024691358,
0.697530864197531,0.703703703703704,0.709876543209877,0.716049382716049,
0.722222222222222,0.728395061728395,0.734567901234568,0.740740740740741,
0.746913580246914,0.753086419753086,0.759259259259259,0.765432098765432,
0.771604938271605,0.777777777777778,0.783950617283951,0.790123456790123,
0.796296296296296,0.802469135802469,0.808641975308642,0.814814814814815,
0.820987654320988,0.827160493827161,0.833333333333333,0.839506172839506,
0.845679012345679,0.851851851851852,0.858024691358025,0.864197530864197,
0.87037037037037,0.876543209876543,0.882716049382716,0.888888888888889,
0.895061728395062,0.901234567901235,0.907407407407407,0.91358024691358,
0.919753086419753,0.925925925925926,0.932098765432099,0.938271604938272,
0.944444444444444,0.950617283950617,0.95679012345679,0.962962962962963,
0.969135802469136,0.975308641975309,0.977791440774828),.UNSPECIFIED.)
GEOMETRIC_REPRESENTATION_ITEM()
RATIONAL_B_SPLINE_SURFACE(((1.,0.866025403784439,1.,0.866025403784439,1.,
0.866025403784439,1.,0.866025403784439,1.,0.866025403784439,1.,0.866025403784439,
1.,0.866025403784439,1.,0.866025403784439,1.,0.866025403784439,1.,0.866025403784439,
1.,0.866025403784439,1.,0.866025403784439,1.,0.866025403784439,1.,0.866025403784439,
1.,0.866025403784439,1.,0.866025403784439,1.,0.866025403784439,1.,0.866025403784439,
1.,0.866025403784439,1.,0.866025403784439,1.,0.866025403784439,1.,0.866025403784439,
1.,0.866025403784439,1.,0.866025403784439,1.,0.866025403784439,1.,0.866025403784439,
1.,0.866025403784439,1.,0.866025403784439,1.,0.866025403784439,1.,0.866025403784439,
1.,0.866025403784439,1.,0.866025403784439,1.,0.866025403784439,1.,0.866025403784439,
1.,0.866025403784439,1.,0.866025403784439,1.,0.866025403784439,1.,0.866025403784439,
1.,0.866025403784439,1.,0.866025403784439,1.,0.866025403784439,1.,0.866025403784439,
1.,0.866025403784439,1.,0.866025403784439,1.,0.866025403784439,1.,0.866025403784439,
1.,0.866025403784439,1.,0.866025403784439,1.,0.866025403784439,1.,0.866025403784439,
1.,0.866025403784439,1.,0.866025403784439,1.,0.866025403784439,1.,0.866025403784439,
1.,0.866025403784439,1.,0.866025403784439,1.,0.866025403784439,1.,0.866025403784439,
1.,0.866025403784439,1.,0.866025403784439,1.,0.866025403784439,1.,0.866025403784439,
1.,0.866025403784439,1.,0.866025403784439,1.,0.866025403784439,1.,0.866025403784439,
1.,0.866025403784439,1.,0.866025403784439,1.,0.866025403784439,1.,0.866025403784439,
1.,0.866025403784439,1.,0.866025403784439,1.,0.866025403784439,1.,0.866025403784439,
1.,0.866025403784439,1.,0.866025403784439,1.,0.866025403784439,1.,0.866025403784439,
1.,0.866025403784439,1.,0.866025403784439,1.,0.866025403784439,1.,0.866025403784439,
1.,0.866025403784439,1.,0.866025403784439,1.,0.866025403784439,1.,0.866025403784439,
1.,0.866025403784439,1.,0.866025403784439,1.,0.866025403784439,1.,0.866025403784439,
1.,0.866025403784439,1.,0.866025403784439,1.,0.866025403784439,1.,0.866025403784439,
1.,0.866025403784439,1.,0.866025403784439,1.,0.866025403784439,1.,0.866025403784439,
1.,0.866025403784439,1.,0.866025403784439,1.,0.866025403784439,1.,0.866025403784439,
1.,0.866025403784439,1.,0.866025403784439,1.,0.866025403784439,1.,0.866025403784439,
1.,0.866025403784439,1.,0.866025403784439,1.,0.866025403784439,1.,0.866025403784439,
1.,0.866025403784439,1.,0.866025403784439,1.,0.866025403784439,1.,0.866025403784439,
1.,0.866025403784439,1.,0.866025403784439,1.,0.866025403784439,1.,0.866025403784439,
1.,0.866025403784439,1.,0.866025403784439,1.,0.866025403784439,1.,0.866025403784439,
1.,0.866025403784439,1.,0.866025403784439,1.,0.866025403784439,1.,0.866025403784439,
1.,0.866025403784439,1.,0.866025403784439,1.,0.866025403784439,1.,0.866025403784439,
1.,0.866025403784439,1.,0.866025403784439,1.,0.866025403784439,1.,0.866025403784439,
1.,0.866025403784439,1.,0.866025403784439,1.,0.866025403784439,1.,0.866025403784439,
1.,0.866025403784439,1.,0.866025403784439,1.,0.866025403784439,1.,0.866025403784439,
1.,0.866025403784439,1.,0.866025403784439,1.,0.866025403784439,1.,0.866025403784439,
1.,0.866025403784439,1.,0.866025403784439,1.,0.866025403784439,1.,0.866025403784439,
1.,0.866025403784439,1.,0.866025403784439,1.,0.866025403784439,1.,0.866025403784439,
1.,0.866025403784439,1.,0.866025403784439,1.,0.866025403784439,1.,0.866025403784439,
1.,0.946113621402695,0.935574890499137),(1.,0.866025403784439,1.,0.866025403784439,
1.,0.866025403784439,1.,0.866025403784439,1.,0.866025403784439,1.,0.866025403784439,
1.,0.866025403784439,1.,0.866025403784439,1.,0.866025403784439,1.,0.866025403784439,
1.,0.866025403784439,1.,0.866025403784439,1.,0.866025403784439,1.,0.866025403784439,
1.,0.866025403784439,1.,0.866025403784439,1.,0.866025403784439,1.,0.866025403784439,
1.,0.866025403784439,1.,0.866025403784439,1.,0.866025403784439,1.,0.866025403784439,
1.,0.866025403784439,1.,0.866025403784439,1.,0.866025403784439,1.,0.866025403784439,
1.,0.866025403784439,1.,0.866025403784439,1.,0.866025403784439,1.,0.866025403784439,
1.,0.866025403784439,1.,0.866025403784439,1.,0.866025403784439,1.,0.866025403784439,
1.,0.866025403784439,1.,0.866025403784439,1.,0.866025403784439,1.,0.866025403784439,
1.,0.866025403784439,1.,0.866025403784439,1.,0.866025403784439,1.,0.866025403784439,
1.,0.866025403784439,1.,0.866025403784439,1.,0.866025403784439,1.,0.866025403784439,
1.,0.866025403784439,1.,0.866025403784439,1.,0.866025403784439,1.,0.866025403784439,
1.,0.866025403784439,1.,0.866025403784439,1.,0.866025403784439,1.,0.866025403784439,
1.,0.866025403784439,1.,0.866025403784439,1.,0.866025403784439,1.,0.866025403784439,
1.,0.866025403784439,1.,0.866025403784439,1.,0.866025403784439,1.,0.866025403784439,
1.,0.866025403784439,1.,0.866025403784439,1.,0.866025403784439,1.,0.866025403784439,
1.,0.866025403784439,1.,0.866025403784439,1.,0.866025403784439,1.,0.866025403784439,
1.,0.866025403784439,1.,0.866025403784439,1.,0.866025403784439,1.,0.866025403784439,
1.,0.866025403784439,1.,0.866025403784439,1.,0.866025403784439,1.,0.866025403784439,
1.,0.866025403784439,1.,0.866025403784439,1.,0.866025403784439,1.,0.866025403784439,
1.,0.866025403784439,1.,0.866025403784439,1.,0.866025403784439,1.,0.866025403784439,
1.,0.866025403784439,1.,0.866025403784439,1.,0.866025403784439,1.,0.866025403784439,
1.,0.866025403784439,1.,0.866025403784439,1.,0.866025403784439,1.,0.866025403784439,
1.,0.866025403784439,1.,0.866025403784439,1.,0.866025403784439,1.,0.866025403784439,
1.,0.866025403784439,1.,0.866025403784439,1.,0.866025403784439,1.,0.866025403784439,
1.,0.866025403784439,1.,0.866025403784439,1.,0.866025403784439,1.,0.866025403784439,
1.,0.866025403784439,1.,0.866025403784439,1.,0.866025403784439,1.,0.866025403784439,
1.,0.866025403784439,1.,0.866025403784439,1.,0.866025403784439,1.,0.866025403784439,
1.,0.866025403784439,1.,0.866025403784439,1.,0.866025403784439,1.,0.866025403784439,
1.,0.866025403784439,1.,0.866025403784439,1.,0.866025403784439,1.,0.866025403784439,
1.,0.866025403784439,1.,0.866025403784439,1.,0.866025403784439,1.,0.866025403784439,
1.,0.866025403784439,1.,0.866025403784439,1.,0.866025403784439,1.,0.866025403784439,
1.,0.866025403784439,1.,0.866025403784439,1.,0.866025403784439,1.,0.866025403784439,
1.,0.866025403784439,1.,0.866025403784439,1.,0.866025403784439,1.,0.866025403784439,
1.,0.866025403784439,1.,0.866025403784439,1.,0.866025403784439,1.,0.866025403784439,
1.,0.866025403784439,1.,0.866025403784439,1.,0.866025403784439,1.,0.866025403784439,
1.,0.866025403784439,1.,0.866025403784439,1.,0.866025403784439,1.,0.866025403784439,
1.,0.866025403784439,1.,0.866025403784439,1.,0.866025403784439,1.,0.866025403784439,
1.,0.866025403784439,1.,0.866025403784439,1.,0.866025403784439,1.,0.866025403784439,
1.,0.946113621402695,0.935574890499137)))
REPRESENTATION_ITEM('')
SURFACE()
);
#300=(
BOUNDED_SURFACE()
B_SPLINE_SURFACE(1,2,((#33589,#33590,#33591,#33592,#33593,#33594,#33595,
#33596,#33597,#33598,#33599,#33600,#33601,#33602,#33603,#33604,#33605,#33606,
#33607,#33608,#33609,#33610,#33611,#33612,#33613,#33614,#33615,#33616,#33617,
#33618,#33619,#33620,#33621,#33622,#33623,#33624,#33625,#33626,#33627,#33628,
#33629,#33630,#33631,#33632,#33633,#33634,#33635,#33636,#33637,#33638,#33639,
#33640,#33641,#33642,#33643,#33644,#33645,#33646,#33647,#33648,#33649,#33650,
#33651,#33652,#33653,#33654,#33655,#33656,#33657,#33658,#33659,#33660,#33661,
#33662,#33663,#33664,#33665,#33666,#33667,#33668,#33669,#33670,#33671,#33672,
#33673,#33674,#33675,#33676,#33677,#33678,#33679,#33680,#33681,#33682,#33683,
#33684,#33685,#33686,#33687,#33688,#33689,#33690,#33691,#33692,#33693,#33694,
#33695,#33696,#33697,#33698,#33699,#33700,#33701,#33702,#33703,#33704,#33705,
#33706,#33707,#33708,#33709,#33710,#33711,#33712,#33713,#33714,#33715,#33716,
#33717,#33718,#33719,#33720,#33721,#33722,#33723,#33724,#33725,#33726,#33727,
#33728,#33729,#33730,#33731,#33732,#33733,#33734,#33735,#33736,#33737,#33738,
#33739,#33740,#33741,#33742,#33743,#33744,#33745,#33746,#33747,#33748,#33749,
#33750,#33751,#33752,#33753,#33754,#33755,#33756,#33757,#33758,#33759,#33760,
#33761,#33762,#33763,#33764,#33765,#33766,#33767,#33768,#33769,#33770,#33771,
#33772,#33773,#33774,#33775,#33776,#33777,#33778,#33779,#33780,#33781,#33782,
#33783,#33784,#33785,#33786,#33787,#33788,#33789,#33790,#33791,#33792,#33793,
#33794,#33795,#33796,#33797,#33798,#33799,#33800,#33801,#33802,#33803,#33804,
#33805,#33806,#33807,#33808,#33809,#33810,#33811,#33812,#33813,#33814,#33815,
#33816,#33817,#33818,#33819,#33820,#33821,#33822,#33823,#33824,#33825,#33826,
#33827,#33828,#33829,#33830,#33831,#33832,#33833,#33834,#33835,#33836,#33837,
#33838,#33839,#33840,#33841,#33842,#33843,#33844,#33845,#33846,#33847,#33848,
#33849,#33850,#33851,#33852,#33853,#33854,#33855,#33856,#33857,#33858,#33859,
#33860,#33861,#33862,#33863,#33864,#33865,#33866,#33867,#33868,#33869,#33870,
#33871,#33872,#33873,#33874,#33875,#33876,#33877,#33878,#33879,#33880,#33881,
#33882,#33883,#33884,#33885,#33886,#33887,#33888,#33889,#33890,#33891,#33892,
#33893,#33894,#33895,#33896,#33897,#33898,#33899,#33900,#33901,#33902,#33903,
#33904,#33905,#33906,#33907,#33908,#33909),(#33910,#33911,#33912,#33913,
#33914,#33915,#33916,#33917,#33918,#33919,#33920,#33921,#33922,#33923,#33924,
#33925,#33926,#33927,#33928,#33929,#33930,#33931,#33932,#33933,#33934,#33935,
#33936,#33937,#33938,#33939,#33940,#33941,#33942,#33943,#33944,#33945,#33946,
#33947,#33948,#33949,#33950,#33951,#33952,#33953,#33954,#33955,#33956,#33957,
#33958,#33959,#33960,#33961,#33962,#33963,#33964,#33965,#33966,#33967,#33968,
#33969,#33970,#33971,#33972,#33973,#33974,#33975,#33976,#33977,#33978,#33979,
#33980,#33981,#33982,#33983,#33984,#33985,#33986,#33987,#33988,#33989,#33990,
#33991,#33992,#33993,#33994,#33995,#33996,#33997,#33998,#33999,#34000,#34001,
#34002,#34003,#34004,#34005,#34006,#34007,#34008,#34009,#34010,#34011,#34012,
#34013,#34014,#34015,#34016,#34017,#34018,#34019,#34020,#34021,#34022,#34023,
#34024,#34025,#34026,#34027,#34028,#34029,#34030,#34031,#34032,#34033,#34034,
#34035,#34036,#34037,#34038,#34039,#34040,#34041,#34042,#34043,#34044,#34045,
#34046,#34047,#34048,#34049,#34050,#34051,#34052,#34053,#34054,#34055,#34056,
#34057,#34058,#34059,#34060,#34061,#34062,#34063,#34064,#34065,#34066,#34067,
#34068,#34069,#34070,#34071,#34072,#34073,#34074,#34075,#34076,#34077,#34078,
#34079,#34080,#34081,#34082,#34083,#34084,#34085,#34086,#34087,#34088,#34089,
#34090,#34091,#34092,#34093,#34094,#34095,#34096,#34097,#34098,#34099,#34100,
#34101,#34102,#34103,#34104,#34105,#34106,#34107,#34108,#34109,#34110,#34111,
#34112,#34113,#34114,#34115,#34116,#34117,#34118,#34119,#34120,#34121,#34122,
#34123,#34124,#34125,#34126,#34127,#34128,#34129,#34130,#34131,#34132,#34133,
#34134,#34135,#34136,#34137,#34138,#34139,#34140,#34141,#34142,#34143,#34144,
#34145,#34146,#34147,#34148,#34149,#34150,#34151,#34152,#34153,#34154,#34155,
#34156,#34157,#34158,#34159,#34160,#34161,#34162,#34163,#34164,#34165,#34166,
#34167,#34168,#34169,#34170,#34171,#34172,#34173,#34174,#34175,#34176,#34177,
#34178,#34179,#34180,#34181,#34182,#34183,#34184,#34185,#34186,#34187,#34188,
#34189,#34190,#34191,#34192,#34193,#34194,#34195,#34196,#34197,#34198,#34199,
#34200,#34201,#34202,#34203,#34204,#34205,#34206,#34207,#34208,#34209,#34210,
#34211,#34212,#34213,#34214,#34215,#34216,#34217,#34218,#34219,#34220,#34221,
#34222,#34223,#34224,#34225,#34226,#34227,#34228,#34229,#34230)),
 .UNSPECIFIED.,.F.,.F.,.F.)
B_SPLINE_SURFACE_WITH_KNOTS((2,2),(3,2,2,2,2,2,2,2,2,2,2,2,2,2,2,2,2,2,
2,2,2,2,2,2,2,2,2,2,2,2,2,2,2,2,2,2,2,2,2,2,2,2,2,2,2,2,2,2,2,2,2,2,2,2,
2,2,2,2,2,2,2,2,2,2,2,2,2,2,2,2,2,2,2,2,2,2,2,2,2,2,2,2,2,2,2,2,2,2,2,2,
2,2,2,2,2,2,2,2,2,2,2,2,2,2,2,2,2,2,2,2,2,2,2,2,2,2,2,2,2,2,2,2,2,2,2,2,
2,2,2,2,2,2,2,2,2,2,2,2,2,2,2,2,2,2,2,2,2,2,2,2,2,2,2,2,2,2,2,2,2,2,3),
(-0.000321975171240205,1.),(0.,0.00617283950617284,0.0123456790123457,0.0185185185185185,
0.0246913580246914,0.0308641975308642,0.037037037037037,0.0432098765432099,
0.0493827160493827,0.0555555555555556,0.0617283950617284,0.0679012345679012,
0.0740740740740741,0.0802469135802469,0.0864197530864197,0.0925925925925926,
0.0987654320987654,0.104938271604938,0.111111111111111,0.117283950617284,
0.123456790123457,0.12962962962963,0.135802469135802,0.141975308641975,
0.148148148148148,0.154320987654321,0.160493827160494,0.166666666666667,
0.172839506172839,0.179012345679012,0.185185185185185,0.191358024691358,
0.197530864197531,0.203703703703704,0.209876543209877,0.216049382716049,
0.222222222222222,0.228395061728395,0.234567901234568,0.240740740740741,
0.246913580246914,0.253086419753086,0.259259259259259,0.265432098765432,
0.271604938271605,0.277777777777778,0.283950617283951,0.290123456790123,
0.296296296296296,0.302469135802469,0.308641975308642,0.314814814814815,
0.320987654320988,0.327160493827161,0.333333333333333,0.339506172839506,
0.345679012345679,0.351851851851852,0.358024691358025,0.364197530864198,
0.37037037037037,0.376543209876543,0.382716049382716,0.388888888888889,
0.395061728395062,0.401234567901235,0.407407407407407,0.41358024691358,
0.419753086419753,0.425925925925926,0.432098765432099,0.438271604938272,
0.444444444444444,0.450617283950617,0.45679012345679,0.462962962962963,
0.469135802469136,0.475308641975309,0.481481481481481,0.487654320987654,
0.493827160493827,0.5,0.506172839506173,0.512345679012346,0.518518518518518,
0.524691358024691,0.530864197530864,0.537037037037037,0.54320987654321,
0.549382716049383,0.555555555555556,0.561728395061728,0.567901234567901,
0.574074074074074,0.580246913580247,0.58641975308642,0.592592592592593,
0.598765432098765,0.604938271604938,0.611111111111111,0.617283950617284,
0.623456790123457,0.62962962962963,0.635802469135803,0.641975308641975,
0.648148148148148,0.654320987654321,0.660493827160494,0.666666666666667,
0.672839506172839,0.679012345679012,0.685185185185185,0.691358024691358,
0.697530864197531,0.703703703703704,0.709876543209877,0.716049382716049,
0.722222222222222,0.728395061728395,0.734567901234568,0.740740740740741,
0.746913580246914,0.753086419753086,0.759259259259259,0.765432098765432,
0.771604938271605,0.777777777777778,0.783950617283951,0.790123456790123,
0.796296296296296,0.802469135802469,0.808641975308642,0.814814814814815,
0.820987654320988,0.827160493827161,0.833333333333333,0.839506172839506,
0.845679012345679,0.851851851851852,0.858024691358025,0.864197530864197,
0.87037037037037,0.876543209876543,0.882716049382716,0.888888888888889,
0.895061728395062,0.901234567901235,0.907407407407407,0.91358024691358,
0.919753086419753,0.925925925925926,0.932098765432099,0.938271604938272,
0.944444444444444,0.950617283950617,0.95679012345679,0.962962962962963,
0.969135802469136,0.975308641975309,0.977791393533952,0.987569307469292),
 .UNSPECIFIED.)
GEOMETRIC_REPRESENTATION_ITEM()
RATIONAL_B_SPLINE_SURFACE(((1.,0.866025403784439,1.,0.866025403784439,1.,
0.866025403784439,1.,0.866025403784439,1.,0.866025403784439,1.,0.866025403784439,
1.,0.866025403784439,1.,0.866025403784439,1.,0.866025403784439,1.,0.866025403784439,
1.,0.866025403784439,1.,0.866025403784439,1.,0.866025403784439,1.,0.866025403784439,
1.,0.866025403784439,1.,0.866025403784439,1.,0.866025403784439,1.,0.866025403784439,
1.,0.866025403784439,1.,0.866025403784439,1.,0.866025403784439,1.,0.866025403784439,
1.,0.866025403784439,1.,0.866025403784439,1.,0.866025403784439,1.,0.866025403784439,
1.,0.866025403784439,1.,0.866025403784439,1.,0.866025403784439,1.,0.866025403784439,
1.,0.866025403784439,1.,0.866025403784439,1.,0.866025403784439,1.,0.866025403784439,
1.,0.866025403784439,1.,0.866025403784439,1.,0.866025403784439,1.,0.866025403784439,
1.,0.866025403784439,1.,0.866025403784439,1.,0.866025403784439,1.,0.866025403784439,
1.,0.866025403784439,1.,0.866025403784439,1.,0.866025403784439,1.,0.866025403784439,
1.,0.866025403784439,1.,0.866025403784439,1.,0.866025403784439,1.,0.866025403784439,
1.,0.866025403784439,1.,0.866025403784439,1.,0.866025403784439,1.,0.866025403784439,
1.,0.866025403784439,1.,0.866025403784439,1.,0.866025403784439,1.,0.866025403784439,
1.,0.866025403784439,1.,0.866025403784439,1.,0.866025403784439,1.,0.866025403784439,
1.,0.866025403784439,1.,0.866025403784439,1.,0.866025403784439,1.,0.866025403784439,
1.,0.866025403784439,1.,0.866025403784439,1.,0.866025403784439,1.,0.866025403784439,
1.,0.866025403784439,1.,0.866025403784439,1.,0.866025403784439,1.,0.866025403784439,
1.,0.866025403784439,1.,0.866025403784439,1.,0.866025403784439,1.,0.866025403784439,
1.,0.866025403784439,1.,0.866025403784439,1.,0.866025403784439,1.,0.866025403784439,
1.,0.866025403784439,1.,0.866025403784439,1.,0.866025403784439,1.,0.866025403784439,
1.,0.866025403784439,1.,0.866025403784439,1.,0.866025403784439,1.,0.866025403784439,
1.,0.866025403784439,1.,0.866025403784439,1.,0.866025403784439,1.,0.866025403784439,
1.,0.866025403784439,1.,0.866025403784439,1.,0.866025403784439,1.,0.866025403784439,
1.,0.866025403784439,1.,0.866025403784439,1.,0.866025403784439,1.,0.866025403784439,
1.,0.866025403784439,1.,0.866025403784439,1.,0.866025403784439,1.,0.866025403784439,
1.,0.866025403784439,1.,0.866025403784439,1.,0.866025403784439,1.,0.866025403784439,
1.,0.866025403784439,1.,0.866025403784439,1.,0.866025403784439,1.,0.866025403784439,
1.,0.866025403784439,1.,0.866025403784439,1.,0.866025403784439,1.,0.866025403784439,
1.,0.866025403784439,1.,0.866025403784439,1.,0.866025403784439,1.,0.866025403784439,
1.,0.866025403784439,1.,0.866025403784439,1.,0.866025403784439,1.,0.866025403784439,
1.,0.866025403784439,1.,0.866025403784439,1.,0.866025403784439,1.,0.866025403784439,
1.,0.866025403784439,1.,0.866025403784439,1.,0.866025403784439,1.,0.866025403784439,
1.,0.866025403784439,1.,0.866025403784439,1.,0.866025403784439,1.,0.866025403784439,
1.,0.866025403784439,1.,0.866025403784439,1.,0.866025403784439,1.,0.866025403784439,
1.,0.866025403784439,1.,0.866025403784439,1.,0.866025403784439,1.,0.866025403784439,
1.,0.866025403784439,1.,0.866025403784439,1.,0.866025403784439,1.,0.866025403784439,
1.,0.866025403784439,1.,0.866025403784439,1.,0.866025403784439,1.,0.866025403784439,
1.,0.866025403784439,1.,0.866025403784439,1.,0.866025403784439,1.,0.866025403784439,
1.,0.946114646713198,0.93557529156132,0.93557529156132,0.93557529156132),
(1.,0.866025403784439,1.,0.866025403784439,1.,0.866025403784439,1.,0.866025403784439,
1.,0.866025403784439,1.,0.866025403784439,1.,0.866025403784439,1.,0.866025403784439,
1.,0.866025403784439,1.,0.866025403784439,1.,0.866025403784439,1.,0.866025403784439,
1.,0.866025403784439,1.,0.866025403784439,1.,0.866025403784439,1.,0.866025403784439,
1.,0.866025403784439,1.,0.866025403784439,1.,0.866025403784439,1.,0.866025403784439,
1.,0.866025403784439,1.,0.866025403784439,1.,0.866025403784439,1.,0.866025403784439,
1.,0.866025403784439,1.,0.866025403784439,1.,0.866025403784439,1.,0.866025403784439,
1.,0.866025403784439,1.,0.866025403784439,1.,0.866025403784439,1.,0.866025403784439,
1.,0.866025403784439,1.,0.866025403784439,1.,0.866025403784439,1.,0.866025403784439,
1.,0.866025403784439,1.,0.866025403784439,1.,0.866025403784439,1.,0.866025403784439,
1.,0.866025403784439,1.,0.866025403784439,1.,0.866025403784439,1.,0.866025403784439,
1.,0.866025403784439,1.,0.866025403784439,1.,0.866025403784439,1.,0.866025403784439,
1.,0.866025403784439,1.,0.866025403784439,1.,0.866025403784439,1.,0.866025403784439,
1.,0.866025403784439,1.,0.866025403784439,1.,0.866025403784439,1.,0.866025403784439,
1.,0.866025403784439,1.,0.866025403784439,1.,0.866025403784439,1.,0.866025403784439,
1.,0.866025403784439,1.,0.866025403784439,1.,0.866025403784439,1.,0.866025403784439,
1.,0.866025403784439,1.,0.866025403784439,1.,0.866025403784439,1.,0.866025403784439,
1.,0.866025403784439,1.,0.866025403784439,1.,0.866025403784439,1.,0.866025403784439,
1.,0.866025403784439,1.,0.866025403784439,1.,0.866025403784439,1.,0.866025403784439,
1.,0.866025403784439,1.,0.866025403784439,1.,0.866025403784439,1.,0.866025403784439,
1.,0.866025403784439,1.,0.866025403784439,1.,0.866025403784439,1.,0.866025403784439,
1.,0.866025403784439,1.,0.866025403784439,1.,0.866025403784439,1.,0.866025403784439,
1.,0.866025403784439,1.,0.866025403784439,1.,0.866025403784439,1.,0.866025403784439,
1.,0.866025403784439,1.,0.866025403784439,1.,0.866025403784439,1.,0.866025403784439,
1.,0.866025403784439,1.,0.866025403784439,1.,0.866025403784439,1.,0.866025403784439,
1.,0.866025403784439,1.,0.866025403784439,1.,0.866025403784439,1.,0.866025403784439,
1.,0.866025403784439,1.,0.866025403784439,1.,0.866025403784439,1.,0.866025403784439,
1.,0.866025403784439,1.,0.866025403784439,1.,0.866025403784439,1.,0.866025403784439,
1.,0.866025403784439,1.,0.866025403784439,1.,0.866025403784439,1.,0.866025403784439,
1.,0.866025403784439,1.,0.866025403784439,1.,0.866025403784439,1.,0.866025403784439,
1.,0.866025403784439,1.,0.866025403784439,1.,0.866025403784439,1.,0.866025403784439,
1.,0.866025403784439,1.,0.866025403784439,1.,0.866025403784439,1.,0.866025403784439,
1.,0.866025403784439,1.,0.866025403784439,1.,0.866025403784439,1.,0.866025403784439,
1.,0.866025403784439,1.,0.866025403784439,1.,0.866025403784439,1.,0.866025403784439,
1.,0.866025403784439,1.,0.866025403784439,1.,0.866025403784439,1.,0.866025403784439,
1.,0.866025403784439,1.,0.866025403784439,1.,0.866025403784439,1.,0.866025403784439,
1.,0.866025403784439,1.,0.866025403784439,1.,0.866025403784439,1.,0.866025403784439,
1.,0.866025403784439,1.,0.866025403784439,1.,0.866025403784439,1.,0.866025403784439,
1.,0.866025403784439,1.,0.866025403784439,1.,0.866025403784439,1.,0.866025403784439,
1.,0.866025403784439,1.,0.866025403784439,1.,0.946114646713198,0.93557529156132,
0.93557529156132,0.93557529156132)))
REPRESENTATION_ITEM('')
SURFACE()
);
#301=CONICAL_SURFACE('',#11717,10.985,0.785398163397459);
#302=CONICAL_SURFACE('',#11722,2.155,0.78539816339745);
#303=CONICAL_SURFACE('',#11725,2.155,0.78539816339745);
#304=CONICAL_SURFACE('',#11728,2.155,0.78539816339745);
#305=CONICAL_SURFACE('',#11731,2.155,0.78539816339745);
#306=CONICAL_SURFACE('',#11774,1.99200000000004,0.785398163397448);
#307=CONICAL_SURFACE('',#11777,1.99200000000004,0.785398163397448);
#308=CONICAL_SURFACE('',#11780,0.975999999999995,0.78539816339745);
#309=CONICAL_SURFACE('',#11792,3.175,0.785398163397427);
#310=CONICAL_SURFACE('',#11795,3.175,0.785398163397427);
#311=CONICAL_SURFACE('',#11798,3.175,0.785398163397427);
#312=CONICAL_SURFACE('',#11801,3.175,0.785398163397427);
#326=STYLED_ITEM('',(#36596),#358);
#327=STYLED_ITEM('',(#36596),#359);
#328=STYLED_ITEM('',(#36596),#360);
#329=STYLED_ITEM('',(#36596),#361);
#330=STYLED_ITEM('',(#36596),#362);
#331=STYLED_ITEM('',(#36596),#363);
#332=STYLED_ITEM('',(#36596),#364);
#333=STYLED_ITEM('',(#36596),#365);
#358=MANIFOLD_SOLID_BREP('Body1',#11262);
#359=MANIFOLD_SOLID_BREP('Body2',#11263);
#360=MANIFOLD_SOLID_BREP('Body3',#11264);
#361=MANIFOLD_SOLID_BREP('Body4',#11265);
#362=MANIFOLD_SOLID_BREP('Body5',#11266);
#363=MANIFOLD_SOLID_BREP('Body6',#11267);
#364=MANIFOLD_SOLID_BREP('Body7',#11268);
#365=MANIFOLD_SOLID_BREP('Body8',#11269);
#390=PLANE('',#11458);
#391=PLANE('',#11459);
#392=PLANE('',#11460);
#393=PLANE('',#11461);
#394=PLANE('',#11462);
#395=PLANE('',#11463);
#396=PLANE('',#11464);
#397=PLANE('',#11465);
#398=PLANE('',#11466);
#399=PLANE('',#11467);
#400=PLANE('',#11468);
#401=PLANE('',#11469);
#402=PLANE('',#11470);
#403=PLANE('',#11471);
#404=PLANE('',#11472);
#405=PLANE('',#11473);
#406=PLANE('',#11474);
#407=PLANE('',#11475);
#408=PLANE('',#11494);
#409=PLANE('',#11495);
#410=PLANE('',#11496);
#411=PLANE('',#11497);
#412=PLANE('',#11498);
#413=PLANE('',#11499);
#414=PLANE('',#11500);
#415=PLANE('',#11501);
#416=PLANE('',#11502);
#417=PLANE('',#11503);
#418=PLANE('',#11504);
#419=PLANE('',#11505);
#420=PLANE('',#11506);
#421=PLANE('',#11507);
#422=PLANE('',#11508);
#423=PLANE('',#11509);
#424=PLANE('',#11510);
#425=PLANE('',#11511);
#426=PLANE('',#11530);
#427=PLANE('',#11531);
#428=PLANE('',#11532);
#429=PLANE('',#11533);
#430=PLANE('',#11534);
#431=PLANE('',#11535);
#432=PLANE('',#11536);
#433=PLANE('',#11537);
#434=PLANE('',#11538);
#435=PLANE('',#11539);
#436=PLANE('',#11540);
#437=PLANE('',#11541);
#438=PLANE('',#11542);
#439=PLANE('',#11543);
#440=PLANE('',#11544);
#441=PLANE('',#11545);
#442=PLANE('',#11546);
#443=PLANE('',#11547);
#444=PLANE('',#11566);
#445=PLANE('',#11567);
#446=PLANE('',#11568);
#447=PLANE('',#11569);
#448=PLANE('',#11570);
#449=PLANE('',#11571);
#450=PLANE('',#11572);
#451=PLANE('',#11573);
#452=PLANE('',#11574);
#453=PLANE('',#11575);
#454=PLANE('',#11576);
#455=PLANE('',#11577);
#456=PLANE('',#11578);
#457=PLANE('',#11579);
#458=PLANE('',#11580);
#459=PLANE('',#11581);
#460=PLANE('',#11582);
#461=PLANE('',#11583);
#462=PLANE('',#11736);
#463=PLANE('',#11737);
#464=PLANE('',#11744);
#465=PLANE('',#11745);
#466=PLANE('',#11746);
#467=PLANE('',#11747);
#468=PLANE('',#11748);
#469=PLANE('',#11749);
#470=PLANE('',#11750);
#471=PLANE('',#11754);
#472=PLANE('',#11755);
#473=PLANE('',#11758);
#474=PLANE('',#11761);
#475=PLANE('',#11764);
#476=PLANE('',#11767);
#477=PLANE('',#11773);
#478=PLANE('',#11785);
#479=PLANE('',#11786);
#480=PLANE('',#11787);
#481=PLANE('',#11788);
#482=PLANE('',#11815);
#483=PLANE('',#11816);
#484=PLANE('',#11817);
#485=PLANE('',#11818);
#486=PLANE('',#11819);
#487=PLANE('',#11820);
#488=PLANE('',#11821);
#489=PLANE('',#11822);
#490=PLANE('',#11823);
#491=PLANE('',#11824);
#492=PLANE('',#11825);
#493=PLANE('',#11826);
#494=PLANE('',#11834);
#495=PLANE('',#11837);
#496=PLANE('',#11840);
#497=PLANE('',#11843);
#498=PLANE('',#11846);
#499=PLANE('',#11847);
#500=PLANE('',#11848);
#501=PLANE('',#11850);
#502=PLANE('',#11851);
#503=PLANE('',#11854);
#504=PLANE('',#11855);
#505=PLANE('',#11856);
#506=PLANE('',#11857);
#507=PLANE('',#11873);
#508=PLANE('',#11874);
#509=PLANE('',#11875);
#510=PLANE('',#11876);
#511=PLANE('',#11877);
#512=PLANE('',#11878);
#513=PLANE('',#11879);
#514=PLANE('',#11880);
#515=PLANE('',#11881);
#516=PLANE('',#11882);
#517=PLANE('',#11883);
#518=PLANE('',#11884);
#519=PLANE('',#11885);
#520=PLANE('',#11886);
#714=ELLIPSE('',#11446,1.32158737874913,1.29894133639841);
#715=ELLIPSE('',#11448,1.32158737875847,1.29894133640388);
#716=ELLIPSE('',#11449,1.32158737877034,1.2989413364124);
#717=ELLIPSE('',#11451,1.32594775747344,1.30189938329286);
#718=ELLIPSE('',#11452,1.32594775747545,1.30189938329438);
#719=ELLIPSE('',#11454,1.32594775748252,1.30189938329882);
#720=ELLIPSE('',#11455,1.3259477575257,1.30189938332617);
#721=ELLIPSE('',#11457,1.32158737873925,1.29894133639057);
#722=ELLIPSE('',#11482,1.32158737875113,1.29894133639988);
#723=ELLIPSE('',#11484,1.32158737869327,1.29894133635907);
#724=ELLIPSE('',#11485,1.32158737875922,1.29894133640477);
#725=ELLIPSE('',#11487,1.32594775746793,1.3018993832892);
#726=ELLIPSE('',#11488,1.32594775746135,1.3018993832848);
#727=ELLIPSE('',#11490,1.32594775747089,1.30189938329139);
#728=ELLIPSE('',#11491,1.32594775751682,1.30189938332048);
#729=ELLIPSE('',#11493,1.32158737872551,1.29894133638101);
#730=ELLIPSE('',#11518,1.32158737874913,1.29894133639841);
#731=ELLIPSE('',#11520,1.32158737875847,1.29894133640388);
#732=ELLIPSE('',#11521,1.32158737877034,1.2989413364124);
#733=ELLIPSE('',#11523,1.32594775747344,1.30189938329286);
#734=ELLIPSE('',#11524,1.32594775747545,1.30189938329438);
#735=ELLIPSE('',#11526,1.32594775748252,1.30189938329882);
#736=ELLIPSE('',#11527,1.3259477575257,1.30189938332617);
#737=ELLIPSE('',#11529,1.32158737873925,1.29894133639057);
#738=ELLIPSE('',#11554,1.32158737871208,1.29894133637222);
#739=ELLIPSE('',#11556,1.32158737876063,1.29894133640545);
#740=ELLIPSE('',#11557,1.3215873787679,1.29894133641094);
#741=ELLIPSE('',#11559,1.32594775747229,1.30189938329206);
#742=ELLIPSE('',#11560,1.32594775746355,1.30189938328618);
#743=ELLIPSE('',#11562,1.3259477575216,1.30189938332397);
#744=ELLIPSE('',#11563,1.32594775751662,1.30189938332021);
#745=ELLIPSE('',#11565,1.32158737874161,1.29894133639227);
#746=ELLIPSE('',#11752,0.824782856622966,0.762000000000211);
#747=ELLIPSE('',#11753,0.824782856622431,0.761999999999637);
#748=ELLIPSE('',#11757,0.824782856622448,0.761999999999701);
#749=ELLIPSE('',#11760,0.824782856623037,0.762000000000206);
#750=ELLIPSE('',#11763,0.82478285662272,0.761999999999946);
#751=ELLIPSE('',#11766,0.824782856622662,0.761999999999831);
#752=ELLIPSE('',#11769,0.824782856622382,0.761999999999617);
#753=ELLIPSE('',#11771,0.824782856622497,0.761999999999736);
#754=ELLIPSE('',#11828,0.8247828566222,0.761999999999463);
#755=ELLIPSE('',#11829,0.824782856621912,0.761999999999204);
#756=ELLIPSE('',#11831,0.824782856622183,0.761999999999485);
#757=ELLIPSE('',#11833,0.824782856621664,0.761999999998966);
#758=ELLIPSE('',#11836,0.824782856622583,0.761999999999779);
#759=ELLIPSE('',#11839,0.824782856622534,0.761999999999738);
#760=ELLIPSE('',#11842,0.824782856623014,0.762000000000189);
#761=ELLIPSE('',#11845,0.824782856623095,0.762000000000223);
#762=B_SPLINE_CURVE_WITH_KNOTS('',3,(#15394,#15395,#15396,#15397),
 .UNSPECIFIED.,.F.,.F.,(4,4),(-0.496042203551295,-0.465357569002963),
 .UNSPECIFIED.);
#763=B_SPLINE_CURVE_WITH_KNOTS('',3,(#15400,#15401,#15402,#15403),
 .UNSPECIFIED.,.F.,.F.,(4,4),(-0.526726838099626,-0.496042203551295),
 .UNSPECIFIED.);
#764=B_SPLINE_CURVE_WITH_KNOTS('',3,(#15411,#15412,#15413,#15414,#15415,
#15416),.UNSPECIFIED.,.F.,.F.,(4,2,4),(0.465357569002967,0.496042203551295,
0.526726838099618),.UNSPECIFIED.);
#765=B_SPLINE_CURVE_WITH_KNOTS('',3,(#15424,#15425,#15426,#15427,#15428,
#15429),.UNSPECIFIED.,.F.,.F.,(4,2,4),(-0.526726838099624,-0.496042203551295,
-0.465357569002967),.UNSPECIFIED.);
#766=B_SPLINE_CURVE_WITH_KNOTS('',3,(#15437,#15438,#15439,#15440,#15441,
#15442),.UNSPECIFIED.,.F.,.F.,(4,2,4),(0.465357569002967,0.496042203551295,
0.526726838099618),.UNSPECIFIED.);
#767=B_SPLINE_CURVE_WITH_KNOTS('',3,(#15525,#15526,#15527,#15528),
 .UNSPECIFIED.,.F.,.F.,(4,4),(-0.496042203551295,-0.465357569002962),
 .UNSPECIFIED.);
#768=B_SPLINE_CURVE_WITH_KNOTS('',3,(#15531,#15532,#15533,#15534),
 .UNSPECIFIED.,.F.,.F.,(4,4),(-0.526726838099626,-0.496042203551295),
 .UNSPECIFIED.);
#769=B_SPLINE_CURVE_WITH_KNOTS('',3,(#15542,#15543,#15544,#15545,#15546,
#15547),.UNSPECIFIED.,.F.,.F.,(4,2,4),(0.465357569002975,0.496042203551295,
0.526726838099626),.UNSPECIFIED.);
#770=B_SPLINE_CURVE_WITH_KNOTS('',3,(#15555,#15556,#15557,#15558,#15559,
#15560),.UNSPECIFIED.,.F.,.F.,(4,2,4),(-0.526726838099632,-0.496042203551295,
-0.465357569002975),.UNSPECIFIED.);
#771=B_SPLINE_CURVE_WITH_KNOTS('',3,(#15568,#15569,#15570,#15571,#15572,
#15573),.UNSPECIFIED.,.F.,.F.,(4,2,4),(0.465357569002966,0.496042203551295,
0.526726838099617),.UNSPECIFIED.);
#772=B_SPLINE_CURVE_WITH_KNOTS('',3,(#15656,#15657,#15658,#15659),
 .UNSPECIFIED.,.F.,.F.,(4,4),(-0.496042203551295,-0.465357569002963),
 .UNSPECIFIED.);
#773=B_SPLINE_CURVE_WITH_KNOTS('',3,(#15662,#15663,#15664,#15665),
 .UNSPECIFIED.,.F.,.F.,(4,4),(-0.526726838099626,-0.496042203551295),
 .UNSPECIFIED.);
#774=B_SPLINE_CURVE_WITH_KNOTS('',3,(#15673,#15674,#15675,#15676,#15677,
#15678),.UNSPECIFIED.,.F.,.F.,(4,2,4),(0.465357569002967,0.496042203551295,
0.526726838099618),.UNSPECIFIED.);
#775=B_SPLINE_CURVE_WITH_KNOTS('',3,(#15686,#15687,#15688,#15689,#15690,
#15691),.UNSPECIFIED.,.F.,.F.,(4,2,4),(-0.526726838099624,-0.496042203551295,
-0.465357569002967),.UNSPECIFIED.);
#776=B_SPLINE_CURVE_WITH_KNOTS('',3,(#15699,#15700,#15701,#15702,#15703,
#15704),.UNSPECIFIED.,.F.,.F.,(4,2,4),(0.465357569002967,0.496042203551295,
0.526726838099618),.UNSPECIFIED.);
#777=B_SPLINE_CURVE_WITH_KNOTS('',3,(#15787,#15788,#15789,#15790),
 .UNSPECIFIED.,.F.,.F.,(4,4),(-0.496042203551296,-0.465357569002961),
 .UNSPECIFIED.);
#778=B_SPLINE_CURVE_WITH_KNOTS('',3,(#15793,#15794,#15795,#15796),
 .UNSPECIFIED.,.F.,.F.,(4,4),(-0.526726838099625,-0.496042203551296),
 .UNSPECIFIED.);
#779=B_SPLINE_CURVE_WITH_KNOTS('',3,(#15804,#15805,#15806,#15807,#15808,
#15809),.UNSPECIFIED.,.F.,.F.,(4,2,4),(0.465357569002966,0.496042203551297,
0.526726838099617),.UNSPECIFIED.);
#780=B_SPLINE_CURVE_WITH_KNOTS('',3,(#15817,#15818,#15819,#15820,#15821,
#15822),.UNSPECIFIED.,.F.,.F.,(4,2,4),(-0.526726838099632,-0.496042203551297,
-0.465357569002976),.UNSPECIFIED.);
#781=B_SPLINE_CURVE_WITH_KNOTS('',3,(#15830,#15831,#15832,#15833,#15834,
#15835),.UNSPECIFIED.,.F.,.F.,(4,2,4),(0.465357569002975,0.496042203551296,
0.526726838099625),.UNSPECIFIED.);
#782=B_SPLINE_CURVE_WITH_KNOTS('',3,(#15912,#15913,#15914,#15915,#15916,
#15917,#15918,#15919,#15920,#15921,#15922,#15923,#15924,#15925,#15926,#15927,
#15928,#15929,#15930,#15931,#15932,#15933,#15934,#15935),.UNSPECIFIED.,
 .F.,.F.,(4,2,2,2,2,2,2,2,2,2,2,4),(21.735148043229,21.8036569750145,21.87839314446,
21.9507157433963,22.0264533977592,22.1003572095216,22.1735114412091,22.2494464904211,
22.3225068859442,22.3979222493655,22.4408998473177,22.4837420617588),
 .UNSPECIFIED.);
#783=B_SPLINE_CURVE_WITH_KNOTS('',3,(#15938,#15939,#15940,#15941,#15942,
#15943,#15944,#15945,#15946,#15947,#15948,#15949,#15950,#15951,#15952,#15953,
#15954,#15955,#15956,#15957),.UNSPECIFIED.,.F.,.F.,(4,2,2,2,2,2,2,2,2,4),
(9.99999992566316E-7,0.073261775877382,0.148517640224947,0.222784465371623,
0.296220695153182,0.372581441669242,0.445206623942385,0.519494682665066,
0.595216703454685,0.600517325493893),.UNSPECIFIED.);
#784=B_SPLINE_CURVE_WITH_KNOTS('',3,(#15962,#15963,#15964,#15965,#15966,
#15967,#15968,#15969,#15970,#15971,#15972,#15973,#15974,#15975,#15976,#15977,
#15978,#15979,#15980,#15981,#15982,#15983,#15984,#15985,#15986,#15987,#15988,
#15989,#15990,#15991,#15992,#15993,#15994,#15995,#15996,#15997,#15998,#15999),
 .UNSPECIFIED.,.F.,.F.,(4,2,2,2,2,2,2,2,2,2,2,2,2,2,2,2,2,2,4),(20.5336633202875,
20.5379028397142,20.6136758540443,20.6880566488837,20.7606931637132,20.8371521629564,
20.9106790831678,20.9848948112315,21.0603960074604,21.133073065851,21.2088134892057,
21.2833596437299,21.3557824762703,21.4315489590993,21.5052648239699,21.578854096748,
21.654575937,21.7274478848722,21.735148043229),.UNSPECIFIED.);
#785=B_SPLINE_CURVE_WITH_KNOTS('',3,(#16000,#16001,#16002,#16003,#16004,
#16005,#16006,#16007,#16008,#16009,#16010,#16011,#16012,#16013,#16014,#16015,
#16016,#16017,#16018,#16019,#16020,#16021,#16022,#16023,#16024,#16025,#16026,
#16027,#16028,#16029,#16030,#16031,#16032,#16033,#16034,#16035),
 .UNSPECIFIED.,.F.,.F.,(4,2,2,2,2,2,2,2,2,2,2,2,2,2,2,2,2,4),(0.600517325493893,
0.667612278651497,0.742740731622242,0.817626982135437,0.890823747292109,
0.966914372473297,1.03979849673016,1.11384065879918,1.18955318544221,1.26185304627361,
1.33673011198806,1.41235250817445,1.48533685995812,1.56118752270884,1.63444336293204,
1.70827064836793,1.78399660279134,1.8010716495484),.UNSPECIFIED.);
#786=B_SPLINE_CURVE_WITH_KNOTS('',3,(#16040,#16041,#16042,#16043,#16044,
#16045,#16046,#16047,#16048,#16049,#16050,#16051,#16052,#16053,#16054,#16055,
#16056,#16057,#16058,#16059,#16060,#16061,#16062,#16063,#16064,#16065,#16066,
#16067,#16068,#16069,#16070,#16071,#16072,#16073,#16074,#16075),
 .UNSPECIFIED.,.F.,.F.,(4,2,2,2,2,2,2,2,2,2,2,2,2,2,2,2,2,4),(19.3323573209819,
19.3484147961251,19.4241832189873,19.4980919040389,19.5713184805846,19.647256341792,
19.7203214434773,19.7958507281764,19.8708169249353,19.9431693074854,20.0189283058273,
20.0930582366082,20.1659315565263,20.2421156550342,20.3153987855463,20.3902097385234,
20.4654324286821,20.5336633202875),.UNSPECIFIED.);
#787=B_SPLINE_CURVE_WITH_KNOTS('',3,(#16076,#16077,#16078,#16079,#16080,
#16081,#16082,#16083,#16084,#16085,#16086,#16087,#16088,#16089,#16090,#16091,
#16092,#16093,#16094,#16095,#16096,#16097,#16098,#16099,#16100,#16101,#16102,
#16103,#16104,#16105,#16106,#16107,#16108,#16109,#16110,#16111),
 .UNSPECIFIED.,.F.,.F.,(4,2,2,2,2,2,2,2,2,2,2,2,2,2,2,2,2,4),(1.8010716495484,
1.85632097173359,1.93097958702412,2.00669544898473,2.07947671745479,2.15509765889709,
2.22887534865907,2.30250174281485,2.37826575306116,2.45073970736901,2.52519594000083,
2.60090396558053,2.6734198270398,2.7487208613376,2.82307768483266,2.89642023960164,
2.97267867831249,3.00178463538),.UNSPECIFIED.);
#788=B_SPLINE_CURVE_WITH_KNOTS('',3,(#16116,#16117,#16118,#16119,#16120,
#16121,#16122,#16123,#16124,#16125,#16126,#16127,#16128,#16129,#16130,#16131,
#16132,#16133,#16134,#16135,#16136,#16137,#16138,#16139,#16140,#16141,#16142,
#16143,#16144,#16145,#16146,#16147,#16148,#16149,#16150,#16151),
 .UNSPECIFIED.,.F.,.F.,(4,2,2,2,2,2,2,2,2,2,2,2,2,2,2,2,2,4),(18.1305008749428,
18.1578726481782,18.2343411588787,18.3078795059063,18.3821918466053,18.4577019685292,
18.5303892204231,18.6061604943215,18.6807161398418,18.7531832580321,18.8289827839731,
18.9027079219705,18.9763779108492,19.0521069660884,19.1249875630571,19.201317714322,
19.2760587308964,19.3323573209819),.UNSPECIFIED.);
#789=B_SPLINE_CURVE_WITH_KNOTS('',3,(#16152,#16153,#16154,#16155,#16156,
#16157,#16158,#16159,#16160,#16161,#16162,#16163,#16164,#16165,#16166,#16167,
#16168,#16169,#16170,#16171,#16172,#16173,#16174,#16175,#16176,#16177,#16178,
#16179,#16180,#16181,#16182,#16183,#16184,#16185,#16186,#16187),
 .UNSPECIFIED.,.F.,.F.,(4,2,2,2,2,2,2,2,2,2,2,2,2,2,2,2,2,4),(3.00178463538,
3.04531437320501,3.11950655772365,3.19518552285788,3.26751148643464,3.34254217247711,
3.41754738871303,3.49065592253175,3.56665029446013,3.63957183128242,3.71352440520342,
3.78919914579688,3.86145728333581,3.9362433503504,4.01200521216688,4.08490867151133,
4.16067128180272,4.20177247101643),.UNSPECIFIED.);
#790=B_SPLINE_CURVE_WITH_KNOTS('',3,(#16192,#16193,#16194,#16195,#16196,
#16197,#16198,#16199,#16200,#16201,#16202,#16203,#16204,#16205,#16206,#16207,
#16208,#16209,#16210,#16211,#16212,#16213,#16214,#16215,#16216,#16217,#16218,
#16219,#16220,#16221,#16222,#16223,#16224,#16225,#16226,#16227),
 .UNSPECIFIED.,.F.,.F.,(4,2,2,2,2,2,2,2,2,2,2,2,2,2,2,2,2,4),(16.9284782926901,
16.9678976750472,17.0438510669624,17.1169330115821,17.1925854820866,17.2675652039096,
17.3399503832518,17.4157492456997,17.4898927769109,17.5628373804741,17.6390334998648,
17.7123303300565,17.7872529716401,17.8624863899118,17.9349763255315,18.0107865695245,
18.0851783175673,18.1305008749428),.UNSPECIFIED.);
#791=B_SPLINE_CURVE_WITH_KNOTS('',3,(#16228,#16229,#16230,#16231,#16232,
#16233,#16234,#16235,#16236,#16237,#16238,#16239,#16240,#16241,#16242,#16243,
#16244,#16245,#16246,#16247,#16248,#16249,#16250,#16251,#16252,#16253,#16254,
#16255,#16256,#16257,#16258,#16259,#16260,#16261,#16262,#16263),
 .UNSPECIFIED.,.F.,.F.,(4,2,2,2,2,2,2,2,2,2,2,2,2,2,2,2,2,4),(4.20177247101643,
4.23398639776024,4.30773238538011,4.38342550182221,4.45573344091213,4.53030981628678,
4.60598738978255,4.67869011646994,4.75422560786203,4.82809657464004,4.90164519382672,
4.97813761619202,5.05060070132551,5.12500656732537,5.20068772705914,5.27315693915424,
5.34840666656873,5.40206337156151),.UNSPECIFIED.);
#792=B_SPLINE_CURVE_WITH_KNOTS('',3,(#16268,#16269,#16270,#16271,#16272,
#16273,#16274,#16275,#16276,#16277,#16278,#16279,#16280,#16281,#16282,#16283,
#16284,#16285,#16286,#16287,#16288,#16289,#16290,#16291,#16292,#16293,#16294,
#16295,#16296,#16297,#16298,#16299,#16300,#16301,#16302,#16303),
 .UNSPECIFIED.,.F.,.F.,(4,2,2,2,2,2,2,2,2,2,2,2,2,2,2,2,2,4),(15.726117824467,
15.7780750192724,15.853606763511,15.9263163363047,16.0021301582733,16.0767077486258,
16.1492304547217,16.2250745456645,16.2988212561443,16.3725818347547,16.448330814818,
16.5212321990517,16.5976919639176,16.6724503083522,16.7448517316063,16.8206624353022,
16.8945883123486,16.9284782926901),.UNSPECIFIED.);
#793=B_SPLINE_CURVE_WITH_KNOTS('',3,(#16304,#16305,#16306,#16307,#16308,
#16309,#16310,#16311,#16312,#16313,#16314,#16315,#16316,#16317,#16318,#16319,
#16320,#16321,#16322,#16323,#16324,#16325,#16326,#16327,#16328,#16329,#16330,
#16331,#16332,#16333,#16334,#16335,#16336,#16337,#16338,#16339),
 .UNSPECIFIED.,.F.,.F.,(4,2,2,2,2,2,2,2,2,2,2,2,2,2,2,2,2,4),(5.40206337156151,
5.42280202682982,5.49609741893041,5.57230460411098,5.64494245529769,5.71908647523217,
5.79474126674104,5.86703289445559,5.94201457649685,6.01707103049025,6.09013508828157,
6.16608119732253,6.23901689966539,6.31292439432828,6.38857738200078,6.46081383727264,
6.5355541601915,6.60170135024484),.UNSPECIFIED.);
#794=B_SPLINE_CURVE_WITH_KNOTS('',3,(#16344,#16345,#16346,#16347,#16348,
#16349,#16350,#16351,#16352,#16353,#16354,#16355,#16356,#16357,#16358,#16359,
#16360,#16361,#16362,#16363,#16364,#16365,#16366,#16367,#16368,#16369,#16370,
#16371,#16372,#16373,#16374,#16375,#16376,#16377,#16378,#16379),
 .UNSPECIFIED.,.F.,.F.,(4,2,2,2,2,2,2,2,2,2,2,2,2,2,2,2,2,4),(14.5232480602204,
14.587720826004,14.6627266216289,14.7351566206077,14.8110065122084,14.8851760254236,
14.9582018706076,15.0344228221103,15.1077455393524,15.1827880426445,15.2580448317048,
15.330567041737,15.4064258517686,15.4808410268554,15.5536039491834,15.6300948676244,
15.7036569101188,15.726117824467),.UNSPECIFIED.);
#795=B_SPLINE_CURVE_WITH_KNOTS('',3,(#16380,#16381,#16382,#16383,#16384,
#16385,#16386,#16387,#16388,#16389,#16390,#16391,#16392,#16393,#16394,#16395,
#16396,#16397,#16398,#16399,#16400,#16401,#16402,#16403,#16404,#16405,#16406,
#16407,#16408,#16409,#16410,#16411,#16412,#16413,#16414,#16415,#16416,#16417),
 .UNSPECIFIED.,.F.,.F.,(4,2,2,2,2,2,2,2,2,2,2,2,2,2,2,2,2,2,4),(6.60170135024484,
6.61137577552695,6.68423824543049,6.75995648832746,6.83329516983099,6.90699999888082,
6.98267359184862,7.05497103331607,7.12950580421754,7.20516147352223,7.27782441678246,
7.35331687836184,7.42722660556652,7.50073581542755,7.57718483813595,7.64964990352041,
7.72401516242666,7.79968082938935,7.80168454737663),.UNSPECIFIED.);
#796=B_SPLINE_CURVE_WITH_KNOTS('',3,(#16422,#16423,#16424,#16425,#16426,
#16427,#16428,#16429,#16430,#16431,#16432,#16433,#16434,#16435,#16436,#16437,
#16438,#16439,#16440,#16441,#16442,#16443,#16444,#16445,#16446,#16447,#16448,
#16449,#16450,#16451,#16452,#16453,#16454,#16455,#16456,#16457,#16458,#16459),
 .UNSPECIFIED.,.F.,.F.,(4,2,2,2,2,2,2,2,2,2,2,2,2,2,2,2,2,2,4),(13.3202804103381,
13.3204858332824,13.396327946239,13.4709396564183,13.5435282910564,13.6194278366413,
13.6932081483868,13.7670676615046,13.842849038861,13.9157830966167,13.992378939387,
14.0671670071756,14.139624957434,14.2154889603696,14.2894442653871,14.3628455045441,
14.4388271007212,14.5119379522483,14.5232480602204),.UNSPECIFIED.);
#797=B_SPLINE_CURVE_WITH_KNOTS('',3,(#16460,#16461,#16462,#16463,#16464,
#16465,#16466,#16467,#16468,#16469,#16470,#16471,#16472,#16473,#16474,#16475,
#16476,#16477,#16478,#16479,#16480,#16481,#16482,#16483,#16484,#16485,#16486,
#16487,#16488,#16489,#16490,#16491,#16492,#16493,#16494,#16495),
 .UNSPECIFIED.,.F.,.F.,(4,2,2,2,2,2,2,2,2,2,2,2,2,2,2,2,2,4),(7.80168454737663,
7.87211413102601,7.94732240677868,8.02177231494539,8.09503035135967,8.17119637492625,
8.24384995772828,8.31795574584409,8.39359784723522,8.46586665716587,8.54080937647058,
8.61593349998142,8.68896308906026,8.76487125310207,8.83783517633463,8.91170775389988,
8.98735057902809,9.00117105879399),.UNSPECIFIED.);
#798=B_SPLINE_CURVE_WITH_KNOTS('',3,(#16500,#16501,#16502,#16503,#16504,
#16505,#16506,#16507,#16508,#16509,#16510,#16511,#16512,#16513,#16514,#16515,
#16516,#16517,#16518,#16519,#16520,#16521,#16522,#16523,#16524,#16525,#16526,
#16527,#16528,#16529,#16530,#16531,#16532,#16533,#16534,#16535),
 .UNSPECIFIED.,.F.,.F.,(4,2,2,2,2,2,2,2,2,2,2,2,2,2,2,2,2,4),(12.1180952064906,
12.1300964327481,12.2059000950361,12.2800023729485,12.3530142433209,12.429164356048,
12.5024207579045,12.577482546649,12.6526682733113,12.7251319418283,12.8009422564708,
12.8752874494255,12.9480251561944,13.0244425760833,13.0979359086261,13.1723612965324,
13.2478199418432,13.3202804103381),.UNSPECIFIED.);
#799=B_SPLINE_CURVE_WITH_KNOTS('',3,(#16536,#16537,#16538,#16539,#16540,
#16541,#16542,#16543,#16544,#16545,#16546,#16547,#16548,#16549,#16550,#16551,
#16552,#16553,#16554,#16555,#16556,#16557,#16558,#16559,#16560,#16561,#16562,
#16563,#16564,#16565,#16566,#16567,#16568,#16569,#16570,#16571),
 .UNSPECIFIED.,.F.,.F.,(4,2,2,2,2,2,2,2,2,2,2,2,2,2,2,2,2,4),(9.00117105879399,
9.05957747650006,9.13428234170321,9.21018018815867,9.28301191789558,9.35869638013789,
9.43207287871308,9.50574697566939,9.58141274520128,9.65371218182695,9.72821591324838,
9.80386132341097,9.87649484644817,9.95195499133692,10.0259184544355,10.0993988305648,
10.1758153751141,10.2009145729997),.UNSPECIFIED.);
#800=B_SPLINE_CURVE_WITH_KNOTS('',3,(#16576,#16577,#16578,#16579,#16580,
#16581,#16582,#16583,#16584,#16585,#16586,#16587,#16588,#16589,#16590,#16591,
#16592,#16593,#16594,#16595,#16596,#16597,#16598,#16599,#16600,#16601,#16602,
#16603,#16604,#16605,#16606,#16607,#16608,#16609,#16610,#16611),
 .UNSPECIFIED.,.F.,.F.,(4,2,2,2,2,2,2,2,2,2,2,2,2,2,2,2,2,4),(10.9159048894311,
10.9417285685803,11.0153840118466,11.0919857331349,11.1645843892562,11.2390977710806,
11.3119432957782,11.3877499955148,11.4624736172065,11.5348953545546,11.6107151951244,
11.6846067885645,11.7580031449498,11.8339173959719,11.9069650575345,11.9827756411443,
12.0577132709042,12.1180952064906),.UNSPECIFIED.);
#801=B_SPLINE_CURVE_WITH_KNOTS('',3,(#16612,#16613,#16614,#16615,#16616,
#16617,#16618,#16619,#16620,#16621,#16622,#16623,#16624,#16625,#16626,#16627,
#16628,#16629,#16630,#16631,#16632,#16633,#16634,#16635,#16636,#16637,#16638,
#16639,#16640,#16641,#16642,#16643,#16644,#16645,#16646,#16647),
 .UNSPECIFIED.,.F.,.F.,(4,2,2,2,2,2,2,2,2,2,2,2,2,2,2,2,2,4),(10.2009145729997,
10.2482956163185,10.322630969213,10.3982930177132,10.4707021613456,10.5458798011778,
10.6203996650247,10.6936310413183,10.7697669637686,10.8424499299129,10.9165283318329,
10.9921696743595,11.0644279598046,11.1393426885537,11.2145500048589,11.2901931117698,
11.3640626377355,11.4005300405451),.UNSPECIFIED.);
#802=B_SPLINE_CURVE_WITH_KNOTS('',3,(#16652,#16653,#16654,#16655,#16656,
#16657,#16658,#16659,#16660,#16661,#16662,#16663,#16664,#16665,#16666,#16667,
#16668,#16669,#16670,#16671,#16672,#16673,#16674,#16675,#16676,#16677,#16678,
#16679,#16680,#16681,#16682,#16683,#16684,#16685,#16686,#16687),
 .UNSPECIFIED.,.F.,.F.,(4,2,2,2,2,2,2,2,2,2,2,2,2,2,2,2,2,4),(9.71384447846264,
9.75123807372611,9.82529401484089,9.90109268520411,9.97346838049563,10.0483588614417,
10.1243054415182,10.1973133659223,10.2731832176365,10.3466515722912,10.4205034552055,
10.4963221962313,10.5687561318069,10.6434396061474,10.7192409968005,10.7920487072417,
10.8676920069456,10.9159048894311),.UNSPECIFIED.);
#803=B_SPLINE_CURVE_WITH_KNOTS('',3,(#16688,#16689,#16690,#16691,#16692,
#16693,#16694,#16695,#16696,#16697,#16698,#16699,#16700,#16701,#16702,#16703,
#16704,#16705,#16706,#16707,#16708,#16709,#16710,#16711,#16712,#16713,#16714,
#16715,#16716,#16717,#16718,#16719,#16720,#16721,#16722,#16723),
 .UNSPECIFIED.,.F.,.F.,(4,2,2,2,2,2,2,2,2,2,2,2,2,2,2,2,2,4),(11.4005300405451,
11.4370319883629,11.512936739381,11.5859633149398,11.66109817641,11.7360373201757,
11.8083047404636,11.8839467877415,11.9580490787634,12.0307064288464,12.1068686070501,
12.1801232420663,12.2545821520692,12.3297865173144,12.4022166746571,12.4778819161449,
12.5522433586879,12.6001780638435),.UNSPECIFIED.);
#804=B_SPLINE_CURVE_WITH_KNOTS('',3,(#16728,#16729,#16730,#16731,#16732,
#16733,#16734,#16735,#16736,#16737,#16738,#16739,#16740,#16741,#16742,#16743,
#16744,#16745,#16746,#16747,#16748,#16749,#16750,#16751,#16752,#16753,#16754,
#16755,#16756,#16757,#16758,#16759,#16760,#16761,#16762,#16763),
 .UNSPECIFIED.,.F.,.F.,(4,2,2,2,2,2,2,2,2,2,2,2,2,2,2,2,2,4),(8.51163684764714,
8.56051488014775,8.63507149460952,8.71089970093124,8.78351502133584,8.85891730151577,
8.93344036889881,9.00688362281223,9.08324511353396,9.15601680140874,9.2303105092999,
9.30611160804312,9.37854583103873,9.45367896715513,9.52886111434057,9.60207190548669,
9.67817105698719,9.71384447846264),.UNSPECIFIED.);
#805=B_SPLINE_CURVE_WITH_KNOTS('',3,(#16764,#16765,#16766,#16767,#16768,
#16769,#16770,#16771,#16772,#16773,#16774,#16775,#16776,#16777,#16778,#16779,
#16780,#16781,#16782,#16783,#16784,#16785,#16786,#16787,#16788,#16789,#16790,
#16791,#16792,#16793,#16794,#16795,#16796,#16797,#16798,#16799),
 .UNSPECIFIED.,.F.,.F.,(4,2,2,2,2,2,2,2,2,2,2,2,2,2,2,2,2,4),(12.6001780638435,
12.6247103529074,12.7011552296179,12.7746607626844,12.8485773844421,12.9240657240679,
12.9967249178213,13.0723793041668,13.1469101199023,13.2192078014959,13.2948804280115,
13.3685813421806,13.4419248676146,13.5176388064005,13.5904973625241,13.6663287520978,
13.7410645591005,13.8000330191523),.UNSPECIFIED.);
#806=B_SPLINE_CURVE_WITH_KNOTS('',3,(#16804,#16805,#16806,#16807,#16808,
#16809,#16810,#16811,#16812,#16813,#16814,#16815,#16816,#16817,#16818,#16819,
#16820,#16821,#16822,#16823,#16824,#16825,#16826,#16827,#16828,#16829,#16830,
#16831,#16832,#16833,#16834,#16835,#16836,#16837,#16838,#16839),
 .UNSPECIFIED.,.F.,.F.,(4,2,2,2,2,2,2,2,2,2,2,2,2,2,2,2,2,4),(7.30910491909639,
7.36904466691905,7.44398341398191,7.51987439067294,7.59292582087003,7.66884263680248,
7.74229098745011,7.81618658837825,7.89202775292298,7.96447527526033,8.03920294715864,
8.11502912392363,8.18787916176048,8.26356811876647,8.33756968006074,8.41126712892377,
8.48791492770604,8.51163684764714),.UNSPECIFIED.);
#807=B_SPLINE_CURVE_WITH_KNOTS('',3,(#16840,#16841,#16842,#16843,#16844,
#16845,#16846,#16847,#16848,#16849,#16850,#16851,#16852,#16853,#16854,#16855,
#16856,#16857,#16858,#16859,#16860,#16861,#16862,#16863,#16864,#16865,#16866,
#16867,#16868,#16869,#16870,#16871,#16872,#16873,#16874,#16875),
 .UNSPECIFIED.,.F.,.F.,(4,2,2,2,2,2,2,2,2,2,2,2,2,2,2,2,2,4),(13.8000330191523,
13.8132997602596,13.8889514810619,13.9628545298081,14.0357938247276,14.1117351018702,
14.1847947733853,14.2598598732388,14.3348365968016,14.4071252676432,14.4827784672019,
14.5569176226292,14.6295574535427,14.7057594011558,14.7790500427128,14.8534523457235,
14.928696802142,14.9997046922138),.UNSPECIFIED.);
#808=B_SPLINE_CURVE_WITH_KNOTS('',3,(#16880,#16881,#16882,#16883,#16884,
#16885,#16886,#16887,#16888,#16889,#16890,#16891,#16892,#16893,#16894,#16895,
#16896,#16897,#16898,#16899,#16900,#16901,#16902,#16903,#16904,#16905,#16906,
#16907,#16908,#16909,#16910,#16911,#16912,#16913,#16914,#16915),
 .UNSPECIFIED.,.F.,.F.,(4,2,2,2,2,2,2,2,2,2,2,2,2,2,2,2,2,4),(6.10664536118632,
6.17866461342232,6.25412061574428,6.32860913795001,6.40210195980943,6.47851717655568,
6.55129006619227,6.62563437348072,6.70146248771766,6.77393386191794,6.84911846281497,
6.9242534903129,6.99751121258825,7.07366115565623,7.1467175018577,7.2208210143513,
7.29664430841493,7.30910491909639),.UNSPECIFIED.);
#809=B_SPLINE_CURVE_WITH_KNOTS('',3,(#16916,#16917,#16918,#16919,#16920,
#16921,#16922,#16923,#16924,#16925,#16926,#16927,#16928,#16929,#16930,#16931,
#16932,#16933,#16934,#16935,#16936,#16937,#16938,#16939,#16940,#16941,#16942,
#16943,#16944,#16945,#16946,#16947,#16948,#16949,#16950,#16951,#16952,#16953),
 .UNSPECIFIED.,.F.,.F.,(4,2,2,2,2,2,2,2,2,2,2,2,2,2,2,2,2,2,4),(14.9997046922138,
15.0011613882487,15.0768405953163,15.1512412983625,15.2237046008859,15.3001915049673,
15.3737351155337,15.4476109939679,15.5231410173751,15.5958386903706,15.6715134909765,
15.7460845825,15.8183911548274,15.8940818044762,15.9678225658965,16.0411406541614,
16.1168976313948,16.1897958881647,16.1999526159265),.UNSPECIFIED.);
#810=B_SPLINE_CURVE_WITH_KNOTS('',3,(#16958,#16959,#16960,#16961,#16962,
#16963,#16964,#16965,#16966,#16967,#16968,#16969,#16970,#16971,#16972,#16973,
#16974,#16975,#16976,#16977,#16978,#16979,#16980,#16981,#16982,#16983,#16984,
#16985,#16986,#16987,#16988,#16989,#16990,#16991,#16992,#16993,#16994,#16995),
 .UNSPECIFIED.,.F.,.F.,(4,2,2,2,2,2,2,2,2,2,2,2,2,2,2,2,2,2,4),(4.90346669291888,
4.91506870236462,4.98820357266399,5.0642110881259,5.13760351086168,5.21158300924342,
5.28745976927761,5.35992685538553,5.43473940551762,5.51060663707254,5.58353780541342,
5.65931490562363,5.73322660979942,5.80700448229846,5.88291878918759,5.95553277454454,
6.03014214800553,6.10600003177494,6.10664536118632),.UNSPECIFIED.);
#811=B_SPLINE_CURVE_WITH_KNOTS('',3,(#16996,#16997,#16998,#16999,#17000,
#17001,#17002,#17003,#17004,#17005,#17006,#17007,#17008,#17009,#17010,#17011,
#17012,#17013,#17014,#17015,#17016,#17017,#17018,#17019,#17020,#17021,#17022,
#17023,#17024,#17025,#17026,#17027,#17028,#17029,#17030,#17031),
 .UNSPECIFIED.,.F.,.F.,(4,2,2,2,2,2,2,2,2,2,2,2,2,2,2,2,2,4),(16.1999526159265,
16.2655653257236,16.3403455878608,16.4126009260191,16.4882729159108,16.5622197702428,
16.6351430664402,16.7111313156308,16.7842342086322,16.8592458915388,16.9342703643616,
17.006591918744,17.0822678244985,17.1564539028843,17.2290898213618,17.305341763104,
17.3786783406879,17.3999243091323),.UNSPECIFIED.);
#812=B_SPLINE_CURVE_WITH_KNOTS('',3,(#17036,#17037,#17038,#17039,#17040,
#17041,#17042,#17043,#17044,#17045,#17046,#17047,#17048,#17049,#17050,#17051,
#17052,#17053,#17054,#17055,#17056,#17057,#17058,#17059,#17060,#17061,#17062,
#17063,#17064,#17065,#17066,#17067,#17068,#17069,#17070,#17071),
 .UNSPECIFIED.,.F.,.F.,(4,2,2,2,2,2,2,2,2,2,2,2,2,2,2,2,2,4),(3.70035601869793,
3.72311624650954,3.79670529484639,3.87322545967511,3.94599134340126,4.02043411786514,
4.09630815185354,4.16885219107272,4.24413705849594,4.31915694699897,4.39250538571124,
4.46875415936413,4.54177650959524,4.61597214318868,4.6918359692238,4.76428118831078,
4.83931350214248,4.90346669291888),.UNSPECIFIED.);
#813=B_SPLINE_CURVE_WITH_KNOTS('',3,(#17072,#17073,#17074,#17075,#17076,
#17077,#17078,#17079,#17080,#17081,#17082,#17083,#17084,#17085,#17086,#17087,
#17088,#17089,#17090,#17091,#17092,#17093,#17094,#17095,#17096,#17097,#17098,
#17099,#17100,#17101,#17102,#17103,#17104,#17105,#17106,#17107),
 .UNSPECIFIED.,.F.,.F.,(4,2,2,2,2,2,2,2,2,2,2,2,2,2,2,2,2,4),(17.3999243091323,
17.4530399991148,17.5283345331806,17.6008444296539,17.6765490523624,17.7509989042253,
17.823471428145,17.9000104222439,17.9736018979823,18.0474522767511,18.1230338545409,
18.1957795858358,18.2714859169376,18.3461070373767,18.4184345339858,18.4941544247165,
18.5679446597149,18.6006226277154),.UNSPECIFIED.);
#814=B_SPLINE_CURVE_WITH_KNOTS('',3,(#17112,#17113,#17114,#17115,#17116,
#17117,#17118,#17119,#17120,#17121,#17122,#17123,#17124,#17125,#17126,#17127,
#17128,#17129,#17130,#17131,#17132,#17133,#17134,#17135,#17136,#17137,#17138,
#17139,#17140,#17141,#17142,#17143,#17144,#17145,#17146,#17147),
 .UNSPECIFIED.,.F.,.F.,(4,2,2,2,2,2,2,2,2,2,2,2,2,2,2,2,2,4),(2.49771244823052,
2.53192367017835,2.60588018236931,2.6817093794774,2.75412572335012,2.82891507571771,
2.90534779569656,2.97827737294551,3.05405652257629,3.12780907401846,3.20158401386577,
3.27744541782065,3.34997777562528,3.42458384305547,3.500416008436,3.57315285646769,
3.64871375186048,3.70035601869793),.UNSPECIFIED.);
#815=B_SPLINE_CURVE_WITH_KNOTS('',3,(#17148,#17149,#17150,#17151,#17152,
#17153,#17154,#17155,#17156,#17157,#17158,#17159,#17160,#17161,#17162,#17163,
#17164,#17165,#17166,#17167,#17168,#17169,#17170,#17171,#17172,#17173,#17174,
#17175,#17176,#17177,#17178,#17179,#17180,#17181,#17182,#17183),
 .UNSPECIFIED.,.F.,.F.,(4,2,2,2,2,2,2,2,2,2,2,2,2,2,2,2,2,4),(18.6006226277154,
18.6412515943291,18.7170613483601,18.7900087657457,18.8657332626392,18.9405674102812,
19.0128543569302,19.088557693505,19.162557674121,19.2354788720627,19.3115235235351,
19.3846788212928,19.4596538548932,19.5347352341894,19.6071003449551,19.6828098930783,
19.7570519591634,19.8010822666473),.UNSPECIFIED.);
#816=B_SPLINE_CURVE_WITH_KNOTS('',3,(#17188,#17189,#17190,#17191,#17192,
#17193,#17194,#17195,#17196,#17197,#17198,#17199,#17200,#17201,#17202,#17203,
#17204,#17205,#17206,#17207,#17208,#17209,#17210,#17211,#17212,#17213,#17214,
#17215,#17216,#17217,#17218,#17219,#17220,#17221,#17222,#17223),
 .UNSPECIFIED.,.F.,.F.,(4,2,2,2,2,2,2,2,2,2,2,2,2,2,2,2,2,4),(1.29536360785537,
1.3410237414506,1.41544967668057,1.49128106098848,1.56379951471133,1.6390676891521,
1.71397174076513,1.78730072016975,1.86353142409529,1.93647760847481,2.01065379022671,
2.08647240671551,2.15887907340395,2.233891932145,2.30952022673612,2.38263254256176,
2.45861853204788,2.49771244823052),.UNSPECIFIED.);
#817=B_SPLINE_CURVE_WITH_KNOTS('',3,(#17224,#17225,#17226,#17227,#17228,
#17229,#17230,#17231,#17232,#17233,#17234,#17235,#17236,#17237,#17238,#17239,
#17240,#17241,#17242,#17243,#17244,#17245,#17246,#17247,#17248,#17249,#17250,
#17251,#17252,#17253,#17254,#17255,#17256,#17257,#17258,#17259),
 .UNSPECIFIED.,.F.,.F.,(4,2,2,2,2,2,2,2,2,2,2,2,2,2,2,2,2,4),(19.8010822666473,
19.8296971813633,19.906008297278,19.9793997719053,20.0537368961349,20.1290904646827,
20.2016554087686,20.2773962331364,20.3519041110699,20.4243981590469,20.500196098935,
20.5738737064591,20.6476431596998,20.7233186338297,20.7961510557135,20.8726600109033,
20.9473431199328,21.0023403829801),.UNSPECIFIED.);
#818=B_SPLINE_CURVE_WITH_KNOTS('',3,(#17264,#17265,#17266,#17267,#17268,
#17269,#17270,#17271,#17272,#17273,#17274,#17275,#17276,#17277,#17278,#17279,
#17280,#17281,#17282,#17283,#17284,#17285,#17286,#17287,#17288,#17289,#17290,
#17291,#17292,#17293,#17294,#17295,#17296,#17297,#17298,#17299),
 .UNSPECIFIED.,.F.,.F.,(4,2,2,2,2,2,2,2,2,2,2,2,2,2,2,2,2,4),(0.0931362008875077,
0.149790300478668,0.22456899063002,0.300876335984474,0.373791545212683,
0.449557496276257,0.523224461713842,0.596984331376484,0.67280719625716,
0.745289827435934,0.819880533368118,0.895676274953773,0.968397209774783,
1.04394319560093,1.11824450231286,1.19181633349106,1.26832090648479,1.29536360785537),
 .UNSPECIFIED.);
#819=B_SPLINE_CURVE_WITH_KNOTS('',3,(#17300,#17301,#17302,#17303,#17304,
#17305,#17306,#17307,#17308,#17309,#17310,#17311,#17312,#17313,#17314,#17315,
#17316,#17317,#17318,#17319,#17320,#17321,#17322,#17323,#17324,#17325,#17326,
#17327,#17328,#17329,#17330,#17331,#17332,#17333,#17334,#17335),
 .UNSPECIFIED.,.F.,.F.,(4,2,2,2,2,2,2,2,2,2,2,2,2,2,2,2,2,4),(21.0023403829801,
21.0197048750824,21.0954669052174,21.1693184250428,21.2426289506514,21.3185035201107,
21.3915117307964,21.4672078751245,21.5421076664978,21.6144392466584,21.6901867449512,
21.7642514729239,21.8371851198342,21.9132980208032,21.9865171840574,22.0614720493734,
22.1366219228939,22.2034453162522),.UNSPECIFIED.);
#820=B_SPLINE_CURVE_WITH_KNOTS('',3,(#17341,#17342,#17343,#17344,#17345,
#17346,#17347,#17348,#17349,#17350,#17351,#17352,#17353,#17354,#17355,#17356),
 .UNSPECIFIED.,.F.,.F.,(4,2,2,2,2,2,2,4),(22.05254318977,22.1180882873261,
22.1913966771312,22.2674423144429,22.3406104852454,22.4162117292643,22.4590238164125,
22.5016957284502),.UNSPECIFIED.);
#821=B_SPLINE_CURVE_WITH_KNOTS('',3,(#17359,#17360,#17361,#17362,#17363,
#17364,#17365,#17366,#17367,#17368,#17369,#17370),.UNSPECIFIED.,.F.,.F.,
(4,2,2,2,2,4),(9.9999999344546E-7,0.0733434466267004,0.148679158126967,
0.222930175188716,0.296371686733512,0.300253786431838),.UNSPECIFIED.);
#822=B_SPLINE_CURVE_WITH_KNOTS('',3,(#17375,#17376,#17377,#17378,#17379,
#17380,#17381,#17382,#17383,#17384,#17385,#17386,#17387,#17388,#17389,#17390,
#17391,#17392,#17393,#17394,#17395,#17396,#17397,#17398,#17399,#17400,#17401,
#17402,#17403,#17404,#17405,#17406,#17407,#17408,#17409,#17410,#17411,#17412),
 .UNSPECIFIED.,.F.,.F.,(4,2,2,2,2,2,2,2,2,2,2,2,2,2,2,2,2,2,4),(20.8492626875425,
20.8526997788034,20.92633985541,21.000728096518,21.0763435643888,21.1491317214545,
21.2250018067689,21.2996612587163,21.3722181264907,21.4481158219413,21.5219436477844,
21.5956936182336,21.6715288843462,21.7445111612003,21.82091239387,21.8957589923512,
21.968208067014,22.0440753652377,22.05254318977),.UNSPECIFIED.);
#823=B_SPLINE_CURVE_WITH_KNOTS('',3,(#17413,#17414,#17415,#17416,#17417,
#17418,#17419,#17420,#17421,#17422,#17423,#17424,#17425,#17426,#17427,#17428,
#17429,#17430,#17431,#17432,#17433,#17434,#17435,#17436,#17437,#17438,#17439,
#17440,#17441,#17442,#17443,#17444,#17445,#17446,#17447,#17448),
 .UNSPECIFIED.,.F.,.F.,(4,2,2,2,2,2,2,2,2,2,2,2,2,2,2,2,2,4),(0.300253786431838,
0.372738742718709,0.445357707142144,0.519651496018735,0.595372982506417,
0.667771570411935,0.742905776016391,0.817772805632994,0.890974369726359,
0.967070519807669,1.03994508219452,1.11399215053163,1.18970337979295,1.26200299001726,
1.33688506897023,1.4124856469306,1.48547398290461,1.50088857683023),
 .UNSPECIFIED.);
#824=B_SPLINE_CURVE_WITH_KNOTS('',3,(#17453,#17454,#17455,#17456,#17457,
#17458,#17459,#17460,#17461,#17462,#17463,#17464,#17465,#17466,#17467,#17468,
#17469,#17470,#17471,#17472,#17473,#17474,#17475,#17476,#17477,#17478,#17479,
#17480,#17481,#17482,#17483,#17484,#17485,#17486,#17487,#17488),
 .UNSPECIFIED.,.F.,.F.,(4,2,2,2,2,2,2,2,2,2,2,2,2,2,2,2,2,4),(19.645692524193,
19.6606922925129,19.7338735908416,19.8095956125189,19.8846784522713,19.9571568609594,
20.0330517465526,20.1072971763248,20.180323721384,20.2566251773908,20.3300226670146,
20.405017375142,20.4803551658045,20.5529426548938,20.6288497632478,20.703344608527,
20.7761247410544,20.8492626875425),.UNSPECIFIED.);
#825=B_SPLINE_CURVE_WITH_KNOTS('',3,(#17489,#17490,#17491,#17492,#17493,
#17494,#17495,#17496,#17497,#17498,#17499,#17500,#17501,#17502,#17503,#17504,
#17505,#17506,#17507,#17508,#17509,#17510,#17511,#17512,#17513,#17514,#17515,
#17516,#17517,#17518,#17519,#17520,#17521,#17522,#17523,#17524),
 .UNSPECIFIED.,.F.,.F.,(4,2,2,2,2,2,2,2,2,2,2,2,2,2,2,2,2,4),(1.50088857683023,
1.56132926031601,1.63457285707235,1.70840412356841,1.78412819690882,1.85644929963145,
1.93111194973725,2.00752125551993,2.08033097553257,2.15598401092867,2.22968137937417,
2.30333560484894,2.37909398462287,2.45154044534442,2.526024569367,2.60175189775299,
2.67437074343493,2.70178082223175),.UNSPECIFIED.);
#826=B_SPLINE_CURVE_WITH_KNOTS('',3,(#17529,#17530,#17531,#17532,#17533,
#17534,#17535,#17536,#17537,#17538,#17539,#17540,#17541,#17542,#17543,#17544,
#17545,#17546,#17547,#17548,#17549,#17550,#17551,#17552,#17553,#17554,#17555,
#17556,#17557,#17558,#17559,#17560,#17561,#17562,#17563,#17564),
 .UNSPECIFIED.,.F.,.F.,(4,2,2,2,2,2,2,2,2,2,2,2,2,2,2,2,2,4),(18.4419253882545,
18.4689607777214,18.5417674330568,18.6176764482914,18.692353915849,18.7649629384551,
18.8409016431339,18.9147471603291,18.9885848629576,19.064436034922,19.1374352663987,
19.21396378216,19.2888237212987,19.361314468639,19.437220454931,19.511246779585,
19.5846350260553,19.645692524193),.UNSPECIFIED.);
#827=B_SPLINE_CURVE_WITH_KNOTS('',3,(#17565,#17566,#17567,#17568,#17569,
#17570,#17571,#17572,#17573,#17574,#17575,#17576,#17577,#17578,#17579,#17580,
#17581,#17582,#17583,#17584,#17585,#17586,#17587,#17588,#17589,#17590,#17591,
#17592,#17593,#17594,#17595,#17596,#17597,#17598,#17599,#17600),
 .UNSPECIFIED.,.F.,.F.,(4,2,2,2,2,2,2,2,2,2,2,2,2,2,2,2,2,4),(2.70178082223175,
2.7498075868511,2.82416793687965,2.89763867153337,2.97403371648344,3.0467255487614,
3.12104813871485,3.19682290300267,3.26925914401864,3.34442216914417,3.41941186677616,
3.49264454688915,3.56877103926687,3.64173068239134,3.71580904480027,3.79157592600334,
3.86392532985084,3.90337860449495),.UNSPECIFIED.);
#828=B_SPLINE_CURVE_WITH_KNOTS('',3,(#17605,#17606,#17607,#17608,#17609,
#17610,#17611,#17612,#17613,#17614,#17615,#17616,#17617,#17618,#17619,#17620,
#17621,#17622,#17623,#17624,#17625,#17626,#17627,#17628,#17629,#17630,#17631,
#17632,#17633,#17634,#17635,#17636,#17637,#17638,#17639,#17640),
 .UNSPECIFIED.,.F.,.F.,(4,2,2,2,2,2,2,2,2,2,2,2,2,2,2,2,2,4),(17.2375105283243,
17.2766093876775,17.3491289223455,17.4250714160394,17.499338938451,17.5724438079126,
17.6487660648582,17.7221856134517,17.7972979623461,17.8726551407408,17.9452709356035,
18.0212231268876,18.0957374704035,18.1685829757813,18.2451763533381,18.3188362628287,
18.393327694986,18.4419253882545),.UNSPECIFIED.);
#829=B_SPLINE_CURVE_WITH_KNOTS('',3,(#17641,#17642,#17643,#17644,#17645,
#17646,#17647,#17648,#17649,#17650,#17651,#17652,#17653,#17654,#17655,#17656,
#17657,#17658,#17659,#17660,#17661,#17662,#17663,#17664,#17665,#17666,#17667,
#17668,#17669,#17670,#17671,#17672,#17673,#17674,#17675,#17676),
 .UNSPECIFIED.,.F.,.F.,(4,2,2,2,2,2,2,2,2,2,2,2,2,2,2,2,2,4),(3.90337860449495,
3.93883886724166,4.01457219092803,4.08759458450174,4.16348348884845,4.23682236672617,
4.31068828214277,4.38647020014597,4.45885236050979,4.53355002247132,4.61009741287901,
4.68294485075255,4.75863558635613,4.83243494391621,4.90612786986772,4.98194618038897,
5.05446269206163,5.10503562671789),.UNSPECIFIED.);
#830=B_SPLINE_CURVE_WITH_KNOTS('',3,(#17681,#17682,#17683,#17684,#17685,
#17686,#17687,#17688,#17689,#17690,#17691,#17692,#17693,#17694,#17695,#17696,
#17697,#17698,#17699,#17700,#17701,#17702,#17703,#17704,#17705,#17706,#17707,
#17708,#17709,#17710,#17711,#17712,#17713,#17714,#17715,#17716),
 .UNSPECIFIED.,.F.,.F.,(4,2,2,2,2,2,2,2,2,2,2,2,2,2,2,2,2,4),(16.0330840204075,
16.0841125680968,16.1568062445162,16.2328002845215,16.3066506773229,16.3806513190249,
16.4565023761763,16.529505085786,16.6054509302403,16.6803367129194,16.752880602522,
16.8288365206925,16.9028884433636,16.9763659562233,17.0524474525173,17.1256538804743,
17.2015044165735,17.2375105283243),.UNSPECIFIED.);
#831=B_SPLINE_CURVE_WITH_KNOTS('',3,(#17717,#17718,#17719,#17720,#17721,
#17722,#17723,#17724,#17725,#17726,#17727,#17728,#17729,#17730,#17731,#17732,
#17733,#17734,#17735,#17736,#17737,#17738,#17739,#17740,#17741,#17742,#17743,
#17744,#17745,#17746,#17747,#17748,#17749,#17750,#17751,#17752),
 .UNSPECIFIED.,.F.,.F.,(4,2,2,2,2,2,2,2,2,2,2,2,2,2,2,2,2,4),(5.10503562671789,
5.128986095298,5.20474754783383,5.27732785095318,5.35269704620258,5.4270671253138,
5.50047437008582,5.57680143647526,5.64947178183473,5.72372970158786,5.79946041374855,
5.87184324601293,5.94694059652358,6.02195142938892,6.09512293367728,6.17118401925371,
6.24413288664852,6.30606327815735),.UNSPECIFIED.);
#832=B_SPLINE_CURVE_WITH_KNOTS('',3,(#17757,#17758,#17759,#17760,#17761,
#17762,#17763,#17764,#17765,#17766,#17767,#17768,#17769,#17770,#17771,#17772,
#17773,#17774,#17775,#17776,#17777,#17778,#17779,#17780,#17781,#17782,#17783,
#17784,#17785,#17786,#17787,#17788,#17789,#17790,#17791,#17792),
 .UNSPECIFIED.,.F.,.F.,(4,2,2,2,2,2,2,2,2,2,2,2,2,2,2,2,2,4),(14.8292463189387,
14.8916714870627,14.9648135885411,15.0410390970424,15.1143699500454,15.1896012848457,
15.2648602033373,15.3374059196021,15.4133145735808,15.4877324338808,15.5605880748831,
15.6370785099079,15.7106441465414,15.7852253876934,15.8607555191899,15.9334919583014,
16.009429815992,16.0330840204075),.UNSPECIFIED.);
#833=B_SPLINE_CURVE_WITH_KNOTS('',3,(#17793,#17794,#17795,#17796,#17797,
#17798,#17799,#17800,#17801,#17802,#17803,#17804,#17805,#17806,#17807,#17808,
#17809,#17810,#17811,#17812,#17813,#17814,#17815,#17816,#17817,#17818,#17819,
#17820,#17821,#17822,#17823,#17824,#17825,#17826,#17827,#17828),
 .UNSPECIFIED.,.F.,.F.,(4,2,2,2,2,2,2,2,2,2,2,2,2,2,2,2,2,4),(6.30606327815735,
6.3181492331229,6.39387422239827,6.4661814102393,6.54103207285242,6.61679445258831,
6.68975868398347,6.76558555007303,6.83892225320291,6.91272954788185,6.98847154733521,
7.06082159277665,7.13545996398158,7.2111879061331,7.28395060515172,7.35954946368319,
7.43343288378257,7.50694329613649),.UNSPECIFIED.);
#834=B_SPLINE_CURVE_WITH_KNOTS('',3,(#17833,#17834,#17835,#17836,#17837,
#17838,#17839,#17840,#17841,#17842,#17843,#17844,#17845,#17846,#17847,#17848,
#17849,#17850,#17851,#17852,#17853,#17854,#17855,#17856,#17857,#17858,#17859,
#17860,#17861,#17862,#17863,#17864,#17865,#17866,#17867,#17868,#17869,#17870),
 .UNSPECIFIED.,.F.,.F.,(4,2,2,2,2,2,2,2,2,2,2,2,2,2,2,2,2,2,4),(13.6255081123504,
13.6257686237007,13.69954079358,13.7736346929468,13.8493998261943,13.9223235489263,
13.9982307610449,14.0730338438641,14.1455609916275,14.2214837444646,14.2954539153653,
14.3689905924738,14.444983558864,14.5181086459962,14.5940987389015,14.6691122320421,
14.7415896580288,14.8174940250215,14.8292463189387),.UNSPECIFIED.);
#835=B_SPLINE_CURVE_WITH_KNOTS('',3,(#17871,#17872,#17873,#17874,#17875,
#17876,#17877,#17878,#17879,#17880,#17881,#17882,#17883,#17884,#17885,#17886,
#17887,#17888,#17889,#17890,#17891,#17892,#17893,#17894,#17895,#17896,#17897,
#17898,#17899,#17900,#17901,#17902,#17903,#17904,#17905,#17906,#17907,#17908),
 .UNSPECIFIED.,.F.,.F.,(4,2,2,2,2,2,2,2,2,2,2,2,2,2,2,2,2,2,4),(7.50694329613649,
7.50704168142511,7.58359819570377,7.65609581512641,7.73056303342993,7.80629057752357,
7.87881785040344,7.95412986788821,8.02852802101149,8.10188223252519,8.17815202887751,
8.25081592351181,8.32501973957617,8.40071914005803,8.47306065592921,8.54810300239926,
8.62315419471727,8.69627520937395,8.7076043136218),.UNSPECIFIED.);
#836=B_SPLINE_CURVE_WITH_KNOTS('',3,(#17913,#17914,#17915,#17916,#17917,
#17918,#17919,#17920,#17921,#17922,#17923,#17924,#17925,#17926,#17927,#17928,
#17929,#17930,#17931,#17932,#17933,#17934,#17935,#17936,#17937,#17938,#17939,
#17940,#17941,#17942,#17943,#17944,#17945,#17946,#17947,#17948),
 .UNSPECIFIED.,.F.,.F.,(4,2,2,2,2,2,2,2,2,2,2,2,2,2,2,2,2,4),(12.4219370484953,
12.4336739434024,12.5069599844754,12.582242359428,12.6574519243816,12.7299629676721,
12.8058471386926,12.8802164895036,12.9530740102056,13.0295128346491,13.1030309691241,
13.1776505229453,13.2531289951954,13.3258184291418,13.4017291063575,13.4763611441305,
13.5490436531927,13.6255081123504),.UNSPECIFIED.);
#837=B_SPLINE_CURVE_WITH_KNOTS('',3,(#17949,#17950,#17951,#17952,#17953,
#17954,#17955,#17956,#17957,#17958,#17959,#17960,#17961,#17962,#17963,#17964,
#17965,#17966,#17967,#17968,#17969,#17970,#17971,#17972,#17973,#17974,#17975,
#17976,#17977,#17978,#17979,#17980,#17981,#17982,#17983,#17984),
 .UNSPECIFIED.,.F.,.F.,(4,2,2,2,2,2,2,2,2,2,2,2,2,2,2,2,2,4),(8.7076043136218,
8.77228185453319,8.84523584591332,8.91920100935851,8.99489701762563,9.06717503350083,
9.14197377622361,9.21778488216681,9.2907019327574,9.36647805600043,9.43982904332821,
9.51358887943921,9.58930403779362,9.66163574037612,9.73622612410351,9.81192490828735,
9.88464155555956,9.90796673370336),.UNSPECIFIED.);
#838=B_SPLINE_CURVE_WITH_KNOTS('',3,(#17989,#17990,#17991,#17992,#17993,
#17994,#17995,#17996,#17997,#17998,#17999,#18000,#18001,#18002,#18003,#18004,
#18005,#18006,#18007,#18008,#18009,#18010,#18011,#18012,#18013,#18014,#18015,
#18016,#18017,#18018,#18019,#18020,#18021,#18022,#18023,#18024),
 .UNSPECIFIED.,.F.,.F.,(4,2,2,2,2,2,2,2,2,2,2,2,2,2,2,2,2,4),(11.2186140020348,
11.2423844354747,11.3152680450516,11.3911530468487,11.4659141859847,11.5384305455132,
11.6143334741864,11.6882621514422,11.7618221629515,11.8377704143951,11.9108541811434,
11.9869038522642,12.0618712560632,12.1343266856154,12.2102089949707,12.2843410369651,
12.3574970509075,12.4219370484953),.UNSPECIFIED.);
#839=B_SPLINE_CURVE_WITH_KNOTS('',3,(#18025,#18026,#18027,#18028,#18029,
#18030,#18031,#18032,#18033,#18034,#18035,#18036,#18037,#18038,#18039,#18040,
#18041,#18042,#18043,#18044,#18045,#18046,#18047,#18048,#18049,#18050,#18051,
#18052,#18053,#18054,#18055,#18056,#18057,#18058,#18059,#18060),
 .UNSPECIFIED.,.F.,.F.,(4,2,2,2,2,2,2,2,2,2,2,2,2,2,2,2,2,4),(9.90796673370336,
9.96019092336532,10.0341032107759,10.1076661950525,10.1841727231514,10.2566639152439,
10.3310840557284,10.4067886417102,10.479272885833,10.5545369162698,10.6289792715137,
10.7022896323962,10.7785115766127,10.8511823564967,10.9253413608401,11.0010205408586,
11.0733316430189,11.1084872386129),.UNSPECIFIED.);
#840=B_SPLINE_CURVE_WITH_KNOTS('',3,(#18065,#18066,#18067,#18068,#18069,
#18070,#18071,#18072,#18073,#18074,#18075,#18076,#18077,#18078,#18079,#18080,
#18081,#18082,#18083,#18084,#18085,#18086,#18087,#18088,#18089,#18090,#18091,
#18092,#18093,#18094,#18095,#18096,#18097,#18098,#18099,#18100),
 .UNSPECIFIED.,.F.,.F.,(4,2,2,2,2,2,2,2,2,2,2,2,2,2,2,2,2,4),(10.0149003245173,
10.0510187671742,10.1268082021235,10.1999760315649,10.2760177990289,10.3494433562341,
10.4234561945758,10.499367171396,10.5718669419739,10.6467132074588,10.7226146491072,
10.7955786855985,10.8713899348627,10.9453350224554,11.0191461453506,11.0950946883506,
11.1677414366375,11.2186140020348),.UNSPECIFIED.);
#841=B_SPLINE_CURVE_WITH_KNOTS('',3,(#18101,#18102,#18103,#18104,#18105,
#18106,#18107,#18108,#18109,#18110,#18111,#18112,#18113,#18114,#18115,#18116,
#18117,#18118,#18119,#18120,#18121,#18122,#18123,#18124,#18125,#18126,#18127,
#18128,#18129,#18130,#18131,#18132,#18133,#18134,#18135,#18136),
 .UNSPECIFIED.,.F.,.F.,(4,2,2,2,2,2,2,2,2,2,2,2,2,2,2,2,2,4),(11.1084872386129,
11.1483283739535,11.2234366551377,11.2991180761832,11.3729850850114,11.4460551399792,
11.5219539304636,11.5949779932755,11.6702784418692,11.7452091132129,11.8174948284876,
11.8931711695511,11.9672655283304,12.0400035862207,12.1161545493962,12.1894019596549,
12.2640057912728,12.3085142855165),.UNSPECIFIED.);
#842=B_SPLINE_CURVE_WITH_KNOTS('',3,(#18141,#18142,#18143,#18144,#18145,
#18146,#18147,#18148,#18149,#18150,#18151,#18152,#18153,#18154,#18155,#18156,
#18157,#18158,#18159,#18160,#18161,#18162,#18163,#18164,#18165,#18166,#18167,
#18168,#18169,#18170,#18171,#18172,#18173,#18174,#18175,#18176),
 .UNSPECIFIED.,.F.,.F.,(4,2,2,2,2,2,2,2,2,2,2,2,2,2,2,2,2,4),(8.81118131706356,
8.85988219698284,8.93431829400909,9.00794050109038,9.08449514330149,9.15729385741128,
9.23177017479016,9.30767841987432,9.38025515534607,9.45557394481698,9.53062772699601,
9.60400921817289,9.6802923492869,9.75334765731488,9.82757672494492,9.90347475980174,
9.97595264247102,10.0149003245173),.UNSPECIFIED.);
#843=B_SPLINE_CURVE_WITH_KNOTS('',3,(#18177,#18178,#18179,#18180,#18181,
#18182,#18183,#18184,#18185,#18186,#18187,#18188,#18189,#18190,#18191,#18192,
#18193,#18194,#18195,#18196,#18197,#18198,#18199,#18200,#18201,#18202,#18203,
#18204,#18205,#18206,#18207,#18208,#18209,#18210,#18211,#18212),
 .UNSPECIFIED.,.F.,.F.,(4,2,2,2,2,2,2,2,2,2,2,2,2,2,2,2,2,4),(12.3085142855165,
12.339197606822,12.4116248037092,12.4873199113833,12.5616695432387,12.6341950359927,
12.7106250508666,12.7841200263037,12.8581561559303,12.9336293939092,13.0062766775809,
13.0819505646389,13.1564677944215,13.2288031792112,13.3044990905332,13.3781864966043,
13.4516243658145,13.5089129023366),.UNSPECIFIED.);
#844=B_SPLINE_CURVE_WITH_KNOTS('',3,(#18217,#18218,#18219,#18220,#18221,
#18222,#18223,#18224,#18225,#18226,#18227,#18228,#18229,#18230,#18231,#18232,
#18233,#18234,#18235,#18236,#18237,#18238,#18239,#18240,#18241,#18242,#18243,
#18244,#18245,#18246,#18247,#18248,#18249,#18250,#18251,#18252),
 .UNSPECIFIED.,.F.,.F.,(4,2,2,2,2,2,2,2,2,2,2,2,2,2,2,2,2,4),(7.60809265701202,
7.66925043325465,7.74258865796053,7.81657848823611,7.89244187032674,7.96489086528524,
8.03971391088468,8.11618116990066,8.18914360620284,8.26495689720756,8.33874274405452,
8.41255092435251,8.488446529945,8.56101160072265,8.63565128320245,8.71151763515169,
8.78428725689606,8.81118131706356),.UNSPECIFIED.);
#845=B_SPLINE_CURVE_WITH_KNOTS('',3,(#18253,#18254,#18255,#18256,#18257,
#18258,#18259,#18260,#18261,#18262,#18263,#18264,#18265,#18266,#18267,#18268,
#18269,#18270,#18271,#18272,#18273,#18274,#18275,#18276,#18277,#18278,#18279,
#18280,#18281,#18282,#18283,#18284,#18285,#18286,#18287,#18288),
 .UNSPECIFIED.,.F.,.F.,(4,2,2,2,2,2,2,2,2,2,2,2,2,2,2,2,2,4),(13.5089129023366,
13.5273209464022,13.6001655562817,13.6761527551668,13.7508680671827,13.8231229487502,
13.8987942754795,13.9726772741613,14.0456959794494,14.1216133937442,14.1946532931299,
14.2698607489188,14.3448115065662,14.4170990904062,14.4927679373319,14.5668818733047,
14.6395814079699,14.70876682955),.UNSPECIFIED.);
#846=B_SPLINE_CURVE_WITH_KNOTS('',3,(#18293,#18294,#18295,#18296,#18297,
#18298,#18299,#18300,#18301,#18302,#18303,#18304,#18305,#18306,#18307,#18308,
#18309,#18310,#18311,#18312,#18313,#18314,#18315,#18316,#18317,#18318,#18319,
#18320,#18321,#18322,#18323,#18324,#18325,#18326,#18327,#18328),
 .UNSPECIFIED.,.F.,.F.,(4,2,2,2,2,2,2,2,2,2,2,2,2,2,2,2,2,4),(6.40518341674792,
6.4784162628992,6.5511518896874,6.62561134850426,6.70147691401884,6.77402804045823,
6.84933011752558,6.9242680029148,6.99763001454459,7.07389505573071,7.14687415420526,
7.22108374957461,7.29693654400393,7.36937584557916,7.44442249461365,7.52008495994635,
7.59323021339548,7.60809265701202),.UNSPECIFIED.);
#847=B_SPLINE_CURVE_WITH_KNOTS('',3,(#18329,#18330,#18331,#18332,#18333,
#18334,#18335,#18336,#18337,#18338,#18339,#18340,#18341,#18342,#18343,#18344,
#18345,#18346,#18347,#18348,#18349,#18350,#18351,#18352,#18353,#18354,#18355,
#18356,#18357,#18358,#18359,#18360,#18361,#18362,#18363,#18364,#18365,#18366),
 .UNSPECIFIED.,.F.,.F.,(4,2,2,2,2,2,2,2,2,2,2,2,2,2,2,2,2,2,4),(14.70876682955,
14.7157544850024,14.7890208603349,14.8635448396388,14.9387594701541,15.0112023807248,
15.0868928606138,15.1612646656571,15.2337659834846,15.3102205634935,15.383736740473,
15.4577093324676,15.5332071233297,15.6058763383245,15.6815523186699,15.7560929436209,
15.8284176747741,15.9041132391376,15.9090867771917),.UNSPECIFIED.);
#848=B_SPLINE_CURVE_WITH_KNOTS('',3,(#18371,#18372,#18373,#18374,#18375,
#18376,#18377,#18378,#18379,#18380,#18381,#18382,#18383,#18384,#18385,#18386,
#18387,#18388,#18389,#18390,#18391,#18392,#18393,#18394,#18395,#18396,#18397,
#18398,#18399,#18400,#18401,#18402,#18403,#18404,#18405,#18406,#18407,#18408),
 .UNSPECIFIED.,.F.,.F.,(4,2,2,2,2,2,2,2,2,2,2,2,2,2,2,2,2,2,4),(5.20254529202766,
5.21114452011972,5.28697167508392,5.35938153580539,5.43419390254545,5.51053572229188,
5.58348377267585,5.65928384720493,5.73298406017818,5.80677715192569,5.88263419023285,
5.95514950133274,6.02977380367191,6.1056037044028,6.17835739435224,6.25393740620464,
6.32827226106894,6.40187723168649,6.40518341674792),.UNSPECIFIED.);
#849=B_SPLINE_CURVE_WITH_KNOTS('',3,(#18409,#18410,#18411,#18412,#18413,
#18414,#18415,#18416,#18417,#18418,#18419,#18420,#18421,#18422,#18423,#18424,
#18425,#18426,#18427,#18428,#18429,#18430,#18431,#18432,#18433,#18434,#18435,
#18436,#18437,#18438,#18439,#18440,#18441,#18442,#18443,#18444),
 .UNSPECIFIED.,.F.,.F.,(4,2,2,2,2,2,2,2,2,2,2,2,2,2,2,2,2,4),(15.9090867771917,
15.9778238334733,16.0512144010312,16.1269370761519,16.1998050074649,16.2757053629313,
16.3504486400594,16.4227045323351,16.4983779027584,16.572288419036,16.6452693381883,
16.7212171599794,16.7942842435471,16.8694133182641,16.9443956867004,17.0166978074018,
17.0923712727689,17.1089856849962),.UNSPECIFIED.);
#850=B_SPLINE_CURVE_WITH_KNOTS('',3,(#18449,#18450,#18451,#18452,#18453,
#18454,#18455,#18456,#18457,#18458,#18459,#18460,#18461,#18462,#18463,#18464,
#18465,#18466,#18467,#18468,#18469,#18470,#18471,#18472,#18473,#18474,#18475,
#18476,#18477,#18478,#18479,#18480,#18481,#18482,#18483,#18484),
 .UNSPECIFIED.,.F.,.F.,(4,2,2,2,2,2,2,2,2,2,2,2,2,2,2,2,2,4),(4.00022881423318,
4.02070918614415,4.09654371873197,4.16908222613698,4.24438030317169,4.31921153434457,
4.39256635461615,4.46882620393768,4.54173975558394,4.61594236312608,4.69176141251603,
4.76417452467247,4.83921434981631,4.9147582004447,4.98789307802441,5.06390455041936,
5.13716531906636,5.20254529202766),.UNSPECIFIED.);
#851=B_SPLINE_CURVE_WITH_KNOTS('',3,(#18485,#18486,#18487,#18488,#18489,
#18490,#18491,#18492,#18493,#18494,#18495,#18496,#18497,#18498,#18499,#18500,
#18501,#18502,#18503,#18504,#18505,#18506,#18507,#18508,#18509,#18510,#18511,
#18512,#18513,#18514,#18515,#18516,#18517,#18518,#18519,#18520),
 .UNSPECIFIED.,.F.,.F.,(4,2,2,2,2,2,2,2,2,2,2,2,2,2,2,2,2,4),(17.1089856849962,
17.1665161724971,17.2391906728527,17.315397504744,17.3886940669098,17.4631529044837,
17.5384017461112,17.6108726881494,17.6865706351,17.7609758822802,17.8334662647143,
17.909956936562,17.9835054396964,18.0574290155657,18.1329626682353,18.2056647279776,
18.2813547593944,18.3094927861098),.UNSPECIFIED.);
#852=B_SPLINE_CURVE_WITH_KNOTS('',3,(#18525,#18526,#18527,#18528,#18529,
#18530,#18531,#18532,#18533,#18534,#18535,#18536,#18537,#18538,#18539,#18540,
#18541,#18542,#18543,#18544,#18545,#18546,#18547,#18548,#18549,#18550,#18551,
#18552,#18553,#18554,#18555,#18556,#18557,#18558,#18559,#18560),
 .UNSPECIFIED.,.F.,.F.,(4,2,2,2,2,2,2,2,2,2,2,2,2,2,2,2,2,4),(2.79777820474308,
2.82974055501476,2.90596677502876,2.97891261559774,3.05471220698905,3.12833745896342,
3.20212780791041,3.27795807200847,3.35043537338853,3.42505679873134,3.50086219836848,
3.57361214287228,3.64918997002519,3.72343368786902,3.79703376475382,3.87357013783338,
3.94625404048576,4.00022881423318),.UNSPECIFIED.);
#853=B_SPLINE_CURVE_WITH_KNOTS('',3,(#18561,#18562,#18563,#18564,#18565,
#18566,#18567,#18568,#18569,#18570,#18571,#18572,#18573,#18574,#18575,#18576,
#18577,#18578,#18579,#18580,#18581,#18582,#18583,#18584,#18585,#18586,#18587,
#18588,#18589,#18590,#18591,#18592,#18593,#18594,#18595,#18596),
 .UNSPECIFIED.,.F.,.F.,(4,2,2,2,2,2,2,2,2,2,2,2,2,2,2,2,2,4),(18.3094927861098,
18.3559299172002,18.4282566986793,18.5039638888353,18.5777086627907,18.6510659398855,
18.7268259021107,18.7997279632351,18.8755572416397,18.950339388976,19.0226087972395,
19.0982961026059,19.1722449066968,19.245202097094,19.3211912918155,19.3942961629852,
19.4693627363339,19.5096597635899),.UNSPECIFIED.);
#854=B_SPLINE_CURVE_WITH_KNOTS('',3,(#18601,#18602,#18603,#18604,#18605,
#18606,#18607,#18608,#18609,#18610,#18611,#18612,#18613,#18614,#18615,#18616,
#18617,#18618,#18619,#18620,#18621,#18622,#18623,#18624,#18625,#18626,#18627,
#18628,#18629,#18630,#18631,#18632,#18633,#18634,#18635,#18636),
 .UNSPECIFIED.,.F.,.F.,(4,2,2,2,2,2,2,2,2,2,2,2,2,2,2,2,2,4),(1.59584813976879,
1.64030318449184,1.71503898288323,1.78839885504719,1.8646663227141,1.93752618397062,
2.01173424115385,2.08753149252248,2.1599312617715,2.23497686627159,2.31041262209493,
2.3835493496218,2.45956486633182,2.53275945264887,2.60674043699168,2.68254322671225,
2.75492629137578,2.79777820474308),.UNSPECIFIED.);
#855=B_SPLINE_CURVE_WITH_KNOTS('',3,(#18637,#18638,#18639,#18640,#18641,
#18642,#18643,#18644,#18645,#18646,#18647,#18648,#18649,#18650,#18651,#18652,
#18653,#18654,#18655,#18656,#18657,#18658,#18659,#18660,#18661,#18662,#18663,
#18664,#18665,#18666,#18667,#18668,#18669,#18670,#18671,#18672),
 .UNSPECIFIED.,.F.,.F.,(4,2,2,2,2,2,2,2,2,2,2,2,2,2,2,2,2,4),(19.5096597635899,
19.5443874072969,19.6167161417866,19.6924060411691,19.7665924754453,19.8392556153294,
19.9155069695267,19.988844146723,20.0632535067116,20.1385470836438,20.2110575105348,
20.2867746653084,20.361223770174,20.4337163429507,20.5102537253887,20.5838448538204,
20.6577345355442,20.7103833929792),.UNSPECIFIED.);
#856=B_SPLINE_CURVE_WITH_KNOTS('',3,(#18677,#18678,#18679,#18680,#18681,
#18682,#18683,#18684,#18685,#18686,#18687,#18688,#18689,#18690,#18691,#18692,
#18693,#18694,#18695,#18696,#18697,#18698,#18699,#18700,#18701,#18702,#18703,
#18704,#18705,#18706,#18707,#18708,#18709,#18710,#18711,#18712),
 .UNSPECIFIED.,.F.,.F.,(4,2,2,2,2,2,2,2,2,2,2,2,2,2,2,2,2,4),(0.393548424805639,
0.4508158900413,0.524378226173459,0.598178030137416,0.673993636458548,0.746445315016936,
0.821076220256436,0.896869346725983,0.969627610190531,1.04521583748751,
1.11938021843885,1.19298764736334,1.26953416876338,1.34217863689082,1.41664190675191,
1.49245745846437,1.56499651097925,1.59584813976879),.UNSPECIFIED.);
#857=B_SPLINE_CURVE_WITH_KNOTS('',3,(#18713,#18714,#18715,#18716,#18717,
#18718,#18719,#18720,#18721,#18722,#18723,#18724,#18725,#18726,#18727,#18728,
#18729,#18730,#18731,#18732,#18733,#18734,#18735,#18736,#18737,#18738,#18739,
#18740,#18741,#18742,#18743,#18744,#18745,#18746,#18747,#18748),
 .UNSPECIFIED.,.F.,.F.,(4,2,2,2,2,2,2,2,2,2,2,2,2,2,2,2,2,4),(20.7103833929792,
20.7333144658301,20.8060594577103,20.8817750110343,20.9563949805616,21.0287361646161,
21.1044665243677,21.1782556223629,21.2515939142169,21.3274014498813,21.4003476115493,
21.4761225443347,21.550953543773,21.6232483768027,21.6989610391312,21.7729579939401,
21.8459054932902,21.9110024905134),.UNSPECIFIED.);
#858=B_SPLINE_CURVE_WITH_KNOTS('',3,(#18754,#18755,#18756,#18757,#18758,
#18759,#18760,#18761),.UNSPECIFIED.,.F.,.F.,(4,2,2,4),(22.3024920269109,
22.3688483291561,22.4097534378368,22.450488682359),.UNSPECIFIED.);
#859=B_SPLINE_CURVE_WITH_KNOTS('',3,(#18767,#18768,#18769,#18770,#18771,
#18772,#18773,#18774,#18775,#18776,#18777,#18778,#18779,#18780,#18781,#18782,
#18783,#18784,#18785,#18786,#18787,#18788,#18789,#18790,#18791,#18792,#18793,
#18794,#18795,#18796,#18797,#18798,#18799,#18800,#18801,#18802,#18803,#18804),
 .UNSPECIFIED.,.F.,.F.,(4,2,2,2,2,2,2,2,2,2,2,2,2,2,2,2,2,2,4),(21.1027737430364,
21.1049994597819,21.1806496975336,21.2549908073923,21.327447317095,21.4038709246568,
21.477356515211,21.5512705483181,21.6267378367605,21.6993771262732,21.7750151016799,
21.8495253198282,21.9218097649896,21.9974664960608,22.0711470350727,22.1444847067024,
22.2201772479808,22.2930155883394,22.3024920269109),.UNSPECIFIED.);
#860=B_SPLINE_CURVE_WITH_KNOTS('',3,(#18805,#18806,#18807,#18808,#18809,
#18810,#18811,#18812,#18813,#18814,#18815,#18816,#18817,#18818,#18819,#18820,
#18821,#18822,#18823,#18824,#18825,#18826,#18827,#18828,#18829,#18830,#18831,
#18832,#18833,#18834,#18835,#18836,#18837,#18838,#18839,#18840),
 .UNSPECIFIED.,.F.,.F.,(4,2,2,2,2,2,2,2,2,2,2,2,2,2,2,2,2,4),(9.99999992579797E-7,
0.071600740188014,0.145227781903171,0.219826582094929,0.293153757552435,
0.369389729999796,0.442157073718064,0.516332458908302,0.592067666639851,
0.664417382066663,0.739430243920045,0.814714869378155,0.887815779298927,
0.963796320979993,1.03688481767441,1.11082953216144,1.18656756573286,1.2009375425295),
 .UNSPECIFIED.);
#861=B_SPLINE_CURVE_WITH_KNOTS('',3,(#18845,#18846,#18847,#18848,#18849,
#18850,#18851,#18852,#18853,#18854,#18855,#18856,#18857,#18858,#18859,#18860,
#18861,#18862,#18863,#18864,#18865,#18866,#18867,#18868,#18869,#18870,#18871,
#18872,#18873,#18874,#18875,#18876,#18877,#18878,#18879,#18880),
 .UNSPECIFIED.,.F.,.F.,(4,2,2,2,2,2,2,2,2,2,2,2,2,2,2,2,2,4),(19.9035199005169,
19.9175621070154,19.9931913738258,20.0670419245932,20.1400064577233,20.2158912543276,
20.2888990748213,20.3640374087997,20.4389565108213,20.5112080306681,20.586835687514,
20.6609182233636,20.7335680720135,20.8097095325252,20.8829447283432,20.9574044024021,
21.0325881211151,21.1027737430364),.UNSPECIFIED.);
#862=B_SPLINE_CURVE_WITH_KNOTS('',3,(#18881,#18882,#18883,#18884,#18885,
#18886,#18887,#18888,#18889,#18890,#18891,#18892,#18893,#18894,#18895,#18896,
#18897,#18898,#18899,#18900,#18901,#18902,#18903,#18904,#18905,#18906,#18907,
#18908,#18909,#18910,#18911,#18912,#18913,#18914,#18915,#18916),
 .UNSPECIFIED.,.F.,.F.,(4,2,2,2,2,2,2,2,2,2,2,2,2,2,2,2,2,4),(1.2009375425295,
1.25888640597054,1.33366417438652,1.40973038664347,1.48263642047109,1.5583965827547,
1.63190591222369,1.70565551039325,1.78141853327558,1.85381950408462,1.92839963526476,
2.00414029370891,2.07684901974681,2.1523858558826,2.22649613810886,2.30005340880839,
2.37654787318782,2.40222076469358),.UNSPECIFIED.);
#863=B_SPLINE_CURVE_WITH_KNOTS('',3,(#18921,#18922,#18923,#18924,#18925,
#18926,#18927,#18928,#18929,#18930,#18931,#18932,#18933,#18934,#18935,#18936,
#18937,#18938,#18939,#18940,#18941,#18942,#18943,#18944,#18945,#18946,#18947,
#18948,#18949,#18950,#18951,#18952,#18953,#18954,#18955,#18956),
 .UNSPECIFIED.,.F.,.F.,(4,2,2,2,2,2,2,2,2,2,2,2,2,2,2,2,2,4),(18.7039793906749,
18.7293029617149,18.8056980625727,18.8791586520591,18.953131415963,19.0285702841427,
19.101183913415,19.1768157473824,19.2512987633797,19.3235895776797,19.3992426079428,
19.4728962017746,19.5462765111672,19.621939128249,19.6947504523395,19.7706652930376,
19.8453478358706,19.9035199005169),.UNSPECIFIED.);
#864=B_SPLINE_CURVE_WITH_KNOTS('',3,(#18957,#18958,#18959,#18960,#18961,
#18962,#18963,#18964,#18965,#18966,#18967,#18968,#18969,#18970,#18971,#18972,
#18973,#18974,#18975,#18976,#18977,#18978,#18979,#18980,#18981,#18982,#18983,
#18984,#18985,#18986,#18987,#18988,#18989,#18990,#18991,#18992),
 .UNSPECIFIED.,.F.,.F.,(4,2,2,2,2,2,2,2,2,2,2,2,2,2,2,2,2,4),(2.40222076469358,
2.44914093359071,2.52355349120749,2.59931628116421,2.67180565378717,2.74706105662188,
2.82174169130443,2.89505148167998,2.97126698121376,3.04407469365999,3.11823210506219,
3.1939764896512,3.26632610002547,3.34132049862734,3.41670007479089,3.48978674293741,
3.56575031853941,3.60344585613563),.UNSPECIFIED.);
#865=B_SPLINE_CURVE_WITH_KNOTS('',3,(#18997,#18998,#18999,#19000,#19001,
#19002,#19003,#19004,#19005,#19006,#19007,#19008,#19009,#19010,#19011,#19012,
#19013,#19014,#19015,#19016,#19017,#19018,#19019,#19020,#19021,#19022,#19023,
#19024,#19025,#19026,#19027,#19028,#19029,#19030,#19031,#19032),
 .UNSPECIFIED.,.F.,.F.,(4,2,2,2,2,2,2,2,2,2,2,2,2,2,2,2,2,4),(17.5045386553045,
17.5418586812021,17.6177208347371,17.6907089519883,17.7659355012861,17.8408305830793,
17.9130759416574,17.9887070096763,18.0627660821069,18.1354499558134,18.2115653258401,
18.2847777274801,18.3593124155404,18.4344694246712,18.506860849091,18.5825116326314,
18.6568267189528,18.7039793906749),.UNSPECIFIED.);
#866=B_SPLINE_CURVE_WITH_KNOTS('',3,(#19033,#19034,#19035,#19036,#19037,
#19038,#19039,#19040,#19041,#19042,#19043,#19044,#19045,#19046,#19047,#19048,
#19049,#19050,#19051,#19052,#19053,#19054,#19055,#19056,#19057,#19058,#19059,
#19060,#19061,#19062,#19063,#19064,#19065,#19066,#19067,#19068),
 .UNSPECIFIED.,.F.,.F.,(4,2,2,2,2,2,2,2,2,2,2,2,2,2,2,2,2,4),(3.60344585613563,
3.63889200144254,3.71282234596637,3.78857215811946,3.86090451389972,3.93566757169027,
4.01183674496613,4.08473249054017,4.16048010314507,4.23405178231718,4.30779143621035,
4.38356860368306,4.45599465938229,4.53056481489909,4.606317231512,4.67901715347343,
4.75454308534004,4.80478993825526),.UNSPECIFIED.);
#867=B_SPLINE_CURVE_WITH_KNOTS('',3,(#19073,#19074,#19075,#19076,#19077,
#19078,#19079,#19080,#19081,#19082,#19083,#19084,#19085,#19086,#19087,#19088,
#19089,#19090,#19091,#19092,#19093,#19094,#19095,#19096,#19097,#19098,#19099,
#19100,#19101,#19102,#19103,#19104,#19105,#19106,#19107,#19108),
 .UNSPECIFIED.,.F.,.F.,(4,2,2,2,2,2,2,2,2,2,2,2,2,2,2,2,2,4),(16.3050203760452,
16.3548731718868,16.4302954221762,16.5028947557627,16.5785325996716,16.6530000240717,
16.7253099644208,16.800971419953,16.8746095269004,16.9480460530331,17.0236904467053,
17.0964860271612,17.1724973404452,17.2471596152608,17.319381368035,17.3950166419569,
17.4688472747823,17.5045386553045),.UNSPECIFIED.);
#868=B_SPLINE_CURVE_WITH_KNOTS('',3,(#19109,#19110,#19111,#19112,#19113,
#19114,#19115,#19116,#19117,#19118,#19119,#19120,#19121,#19122,#19123,#19124,
#19125,#19126,#19127,#19128,#19129,#19130,#19131,#19132,#19133,#19134,#19135,
#19136,#19137,#19138,#19139,#19140,#19141,#19142,#19143,#19144),
 .UNSPECIFIED.,.F.,.F.,(4,2,2,2,2,2,2,2,2,2,2,2,2,2,2,2,2,4),(4.80478993825526,
4.82873212967197,4.90228155462143,4.97876535710322,5.05139730211433,5.12580123479856,
5.20158249025959,5.2740707767987,5.34931707642891,5.42409257488621,5.49739681707695,
5.57360418155691,5.64646503610294,5.72061649399095,5.79638216249746,5.86874457180556,
5.94373268071591,6.00642764136115),.UNSPECIFIED.);
#869=B_SPLINE_CURVE_WITH_KNOTS('',3,(#19149,#19150,#19151,#19152,#19153,
#19154,#19155,#19156,#19157,#19158,#19159,#19160,#19161,#19162,#19163,#19164,
#19165,#19166,#19167,#19168,#19169,#19170,#19171,#19172,#19173,#19174,#19175,
#19176,#19177,#19178,#19179,#19180,#19181,#19182,#19183,#19184),
 .UNSPECIFIED.,.F.,.F.,(4,2,2,2,2,2,2,2,2,2,2,2,2,2,2,2,2,4),(15.1052499210504,
15.1675158452439,15.2423988721291,15.3146509504745,15.3902976012197,15.4643450279264,
15.5370760734893,15.6131774634138,15.6863787117015,15.761002222048,15.8361443918783,
15.9085286335628,15.9841921557106,16.0584929502958,16.1310020353728,16.2073806551034,
16.2808278140705,16.3050203760452),.UNSPECIFIED.);
#870=B_SPLINE_CURVE_WITH_KNOTS('',3,(#19185,#19186,#19187,#19188,#19189,
#19190,#19191,#19192,#19193,#19194,#19195,#19196,#19197,#19198,#19199,#19200,
#19201,#19202,#19203,#19204,#19205,#19206,#19207,#19208,#19209,#19210,#19211,
#19212,#19213,#19214,#19215,#19216,#19217,#19218,#19219,#19220),
 .UNSPECIFIED.,.F.,.F.,(4,2,2,2,2,2,2,2,2,2,2,2,2,2,2,2,2,4),(6.00642764136115,
6.01921979787647,6.09230411676459,6.16826312791688,6.24147045508006,6.31539850918389,
6.39117217319509,6.46353078683716,6.5382914339967,6.61457567378796,6.6874731272014,
6.76322069995753,6.83686681762636,6.91060870469478,6.98641213318798,7.05887567245481,
7.13344818869197,7.20797850375824),.UNSPECIFIED.);
#871=B_SPLINE_CURVE_WITH_KNOTS('',3,(#19225,#19226,#19227,#19228,#19229,
#19230,#19231,#19232,#19233,#19234,#19235,#19236,#19237,#19238,#19239,#19240,
#19241,#19242,#19243,#19244,#19245,#19246,#19247,#19248,#19249,#19250,#19251,
#19252,#19253,#19254,#19255,#19256,#19257,#19258,#19259,#19260),
 .UNSPECIFIED.,.F.,.F.,(4,2,2,2,2,2,2,2,2,2,2,2,2,2,2,2,2,4),(13.9056073328072,
13.979733684865,14.0541976690322,14.1265393105317,14.2022213563442,14.2758559700236,
14.3493613399648,14.4249998082098,14.4977914544797,14.573912278901,14.6485663529743,
14.7208084008114,14.7964618439306,14.8702844710759,14.9433557153578,15.0192074340945,
15.0921875748939,15.1052499210504),.UNSPECIFIED.);
#872=B_SPLINE_CURVE_WITH_KNOTS('',3,(#19261,#19262,#19263,#19264,#19265,
#19266,#19267,#19268,#19269,#19270,#19271,#19272,#19273,#19274,#19275,#19276,
#19277,#19278,#19279,#19280,#19281,#19282,#19283,#19284,#19285,#19286,#19287,
#19288,#19289,#19290,#19291,#19292,#19293,#19294,#19295,#19296,#19297,#19298),
 .UNSPECIFIED.,.F.,.F.,(4,2,2,2,2,2,2,2,2,2,2,2,2,2,2,2,2,2,4),(7.20797850375824,
7.20922458919542,7.28192775231267,7.3574553433693,7.43173500783957,7.50528881442058,
7.58177474025056,7.65445788369708,7.72886560966757,7.80467738626606,7.87717774144433,
7.95242751469966,8.02730916972658,8.10062009072416,8.17683211153858,8.24975800118347,
8.32391592638887,8.39971483158691,8.41018693810434),.UNSPECIFIED.);
#873=B_SPLINE_CURVE_WITH_KNOTS('',3,(#19303,#19304,#19305,#19306,#19307,
#19308,#19309,#19310,#19311,#19312,#19313,#19314,#19315,#19316,#19317,#19318,
#19319,#19320,#19321,#19322,#19323,#19324,#19325,#19326,#19327,#19328,#19329,
#19330,#19331,#19332,#19333,#19334,#19335,#19336,#19337,#19338,#19339,#19340),
 .UNSPECIFIED.,.F.,.F.,(4,2,2,2,2,2,2,2,2,2,2,2,2,2,2,2,2,2,4),(12.7053500380718,
12.715500408312,12.7911747085665,12.8652227682113,12.9380133372392,13.0141133728098,
13.0873155564923,13.1620400374673,13.2371797690825,13.3095699175679,13.3852583231407,
13.4595570740892,13.5321116326848,13.6084863643335,13.6819321581728,13.7560626688118,
13.8314806701097,13.9040775820415,13.9056073328072),.UNSPECIFIED.);
#874=B_SPLINE_CURVE_WITH_KNOTS('',3,(#19341,#19342,#19343,#19344,#19345,
#19346,#19347,#19348,#19349,#19350,#19351,#19352,#19353,#19354,#19355,#19356,
#19357,#19358,#19359,#19360,#19361,#19362,#19363,#19364,#19365,#19366,#19367,
#19368,#19369,#19370,#19371,#19372,#19373,#19374,#19375,#19376),
 .UNSPECIFIED.,.F.,.F.,(4,2,2,2,2,2,2,2,2,2,2,2,2,2,2,2,2,4),(8.41018693810434,
8.47210288948872,8.54709729504254,8.62270255411287,8.69579673625766,8.77176395924554,
8.84504825099315,8.91898641394924,8.99479579943711,9.06719302368103,9.14196382255198,
9.21837305385914,9.29128438161236,9.36704463649688,9.44077591825568,9.51453237511723,
9.59037386733617,9.61221885207275),.UNSPECIFIED.);
#875=B_SPLINE_CURVE_WITH_KNOTS('',3,(#19381,#19382,#19383,#19384,#19385,
#19386,#19387,#19388,#19389,#19390,#19391,#19392,#19393,#19394,#19395,#19396,
#19397,#19398,#19399,#19400,#19401,#19402,#19403,#19404,#19405,#19406,#19407,
#19408,#19409,#19410,#19411,#19412,#19413,#19414,#19415,#19416),
 .UNSPECIFIED.,.F.,.F.,(4,2,2,2,2,2,2,2,2,2,2,2,2,2,2,2,2,4),(11.5053094523182,
11.5268488992701,11.6025634962346,11.6762068956174,11.7497924810252,11.8254376640932,
11.8982374792771,11.9744787611083,12.0491370912012,12.1214119953902,12.1970956139134,
12.2709225306323,12.3440655074962,12.4199194393904,12.4929037111634,12.5683452713175,
12.6432286827158,12.7053500380718),.UNSPECIFIED.);
#876=B_SPLINE_CURVE_WITH_KNOTS('',3,(#19417,#19418,#19419,#19420,#19421,
#19422,#19423,#19424,#19425,#19426,#19427,#19428,#19429,#19430,#19431,#19432,
#19433,#19434,#19435,#19436,#19437,#19438,#19439,#19440,#19441,#19442,#19443,
#19444,#19445,#19446,#19447,#19448,#19449,#19450,#19451,#19452),
 .UNSPECIFIED.,.F.,.F.,(4,2,2,2,2,2,2,2,2,2,2,2,2,2,2,2,2,4),(9.61221885207275,
9.66288666337229,9.73747403439585,9.81328637680854,9.88600495943817,9.96154694365518,
10.0359273989204,10.1094979228893,10.1859989158825,10.2587446558326,10.3331687130746,
10.4090226703821,10.4815480891719,10.5568140406692,10.631811171281,10.705141054464,
10.7813706230653,10.8150631151595),.UNSPECIFIED.);
#877=B_SPLINE_CURVE_WITH_KNOTS('',3,(#19457,#19458,#19459,#19460,#19461,
#19462,#19463,#19464,#19465,#19466,#19467,#19468,#19469,#19470,#19471,#19472,
#19473,#19474,#19475,#19476,#19477,#19478,#19479,#19480,#19481,#19482,#19483,
#19484,#19485,#19486,#19487,#19488,#19489,#19490,#19491,#19492),
 .UNSPECIFIED.,.F.,.F.,(4,2,2,2,2,2,2,2,2,2,2,2,2,2,2,2,2,4),(10.3044171497523,
10.3401614858824,10.4140935645159,10.489832598554,10.5621534139354,10.6369182779871,
10.7130332981672,10.7859288776338,10.861677195313,10.9352141470178,11.0089534074536,
11.0847186438897,11.1571276956958,11.2316974123293,11.3043040355563,11.3799904932741,
11.4544634746901,11.5053094523182),.UNSPECIFIED.);
#878=B_SPLINE_CURVE_WITH_KNOTS('',3,(#19493,#19494,#19495,#19496,#19497,
#19498,#19499,#19500,#19501,#19502,#19503,#19504,#19505,#19506,#19507,#19508,
#19509,#19510,#19511,#19512,#19513,#19514,#19515,#19516,#19517,#19518,#19519,
#19520,#19521,#19522,#19523,#19524,#19525,#19526,#19527,#19528),
 .UNSPECIFIED.,.F.,.F.,(4,2,2,2,2,2,2,2,2,2,2,2,2,2,2,2,2,4),(10.8150631151595,
10.8543722558447,10.928549127917,11.0043927799348,11.0768188941975,11.1518322431134,
11.2275640823162,11.3034083276436,11.3775655232947,11.4505952542184,11.5268030118463,
11.6001136025955,11.6751704644753,11.7504138876136,11.8229261851396,11.8987786494732,
11.9731806969486,12.0177749705651),.UNSPECIFIED.);
#879=B_SPLINE_CURVE_WITH_KNOTS('',3,(#19533,#19534,#19535,#19536,#19537,
#19538,#19539,#19540,#19541,#19542,#19543,#19544,#19545,#19546,#19547,#19548,
#19549,#19550,#19551,#19552,#19553,#19554,#19555,#19556,#19557,#19558,#19559,
#19560,#19561,#19562,#19563,#19564,#19565,#19566,#19567,#19568),
 .UNSPECIFIED.,.F.,.F.,(4,2,2,2,2,2,2,2,2,2,2,2,2,2,2,2,2,4),(9.10333053600743,
9.15055193771733,9.22496917372991,9.30072377279127,9.37321466466583,9.44847498318585,
9.52311148303587,9.59642450060639,9.67264449108136,9.74542789452109,9.81958874887466,
9.89532358746586,9.96766812633393,10.0426661407919,10.1179953699147,10.1910837755611,
10.2670501800193,10.3044171497523),.UNSPECIFIED.);
#880=B_SPLINE_CURVE_WITH_KNOTS('',3,(#19569,#19570,#19571,#19572,#19573,
#19574,#19575,#19576,#19577,#19578,#19579,#19580,#19581,#19582,#19583,#19584,
#19585,#19586,#19587,#19588,#19589,#19590,#19591,#19592,#19593,#19594,#19595,
#19596,#19597,#19598,#19599,#19600,#19601,#19602,#19603,#19604),
 .UNSPECIFIED.,.F.,.F.,(4,2,2,2,2,2,2,2,2,2,2,2,2,2,2,2,2,4),(12.0177749705651,
12.0459439977539,12.1224209422467,12.1959701551707,12.2703988259824,12.3459166164042,
12.4186131843801,12.4944189632762,12.5689829374183,12.6415023536567,12.7173389558782,
12.7910721614232,12.864839149528,12.9405736130224,13.0134614850999,13.0899381426276,
13.1646814782178,13.2202175978974),.UNSPECIFIED.);
#881=B_SPLINE_CURVE_WITH_KNOTS('',3,(#19609,#19610,#19611,#19612,#19613,
#19614,#19615,#19616,#19617,#19618,#19619,#19620,#19621,#19622,#19623,#19624,
#19625,#19626,#19627,#19628,#19629,#19630,#19631,#19632,#19633,#19634,#19635,
#19636,#19637,#19638,#19639,#19640,#19641,#19642,#19643,#19644),
 .UNSPECIFIED.,.F.,.F.,(4,2,2,2,2,2,2,2,2,2,2,2,2,2,2,2,2,4),(7.90214345446006,
7.96039945586104,8.03518468932147,8.11120319187168,8.18411460885446,8.25988125009896,
8.33336199006571,8.4071168320765,8.48287370775027,8.55526368666003,8.62984909064281,
8.70558475614216,8.77829819812881,8.8538407735689,8.92791467968878,9.0014762398683,
9.07797636059719,9.10333053600743),.UNSPECIFIED.);
#882=B_SPLINE_CURVE_WITH_KNOTS('',3,(#19645,#19646,#19647,#19648,#19649,
#19650,#19651,#19652,#19653,#19654,#19655,#19656,#19657,#19658,#19659,#19660,
#19661,#19662,#19663,#19664,#19665,#19666,#19667,#19668,#19669,#19670,#19671,
#19672,#19673,#19674,#19675,#19676,#19677,#19678,#19679,#19680),
 .UNSPECIFIED.,.F.,.F.,(4,2,2,2,2,2,2,2,2,2,2,2,2,2,2,2,2,4),(13.2202175978974,
13.2370767530604,13.3128793204275,13.3867903685147,13.460104092076,13.5360416304297,
13.6091088630933,13.6847766992306,13.7597402374587,13.8321156847763,13.9079057206965,
13.982033311037,14.0549791174888,14.1311582866812,14.204439423608,14.2793744030468,
14.354590742388,14.4220042621459),.UNSPECIFIED.);
#883=B_SPLINE_CURVE_WITH_KNOTS('',3,(#19685,#19686,#19687,#19688,#19689,
#19690,#19691,#19692,#19693,#19694,#19695,#19696,#19697,#19698,#19699,#19700,
#19701,#19702,#19703,#19704,#19705,#19706,#19707,#19708,#19709,#19710,#19711,
#19712,#19713,#19714,#19715,#19716,#19717,#19718,#19719,#19720),
 .UNSPECIFIED.,.F.,.F.,(4,2,2,2,2,2,2,2,2,2,2,2,2,2,2,2,2,4),(6.70124289322726,
6.7715290879724,6.84681622467596,6.9213776981955,6.99471361200024,7.07095980223775,
7.14370921775499,7.21789363955208,7.29362513808374,7.36597592622018,7.44099806657252,
7.51623904898732,7.58934725641939,7.66533640932017,7.73840086116704,7.812352957716,
7.88808605229705,7.90214345446006),.UNSPECIFIED.);
#884=B_SPLINE_CURVE_WITH_KNOTS('',3,(#19721,#19722,#19723,#19724,#19725,
#19726,#19727,#19728,#19729,#19730,#19731,#19732,#19733,#19734,#19735,#19736,
#19737,#19738,#19739,#19740,#19741,#19742,#19743,#19744,#19745,#19746,#19747,
#19748,#19749,#19750,#19751,#19752,#19753,#19754,#19755,#19756,#19757,#19758),
 .UNSPECIFIED.,.F.,.F.,(4,2,2,2,2,2,2,2,2,2,2,2,2,2,2,2,2,2,4),(14.4220042621459,
14.4270670869734,14.502867746995,14.5772427049859,14.6499344470954,14.7263851908868,
14.7999071073808,14.8742276556564,14.9497200860508,15.0223907681477,15.0981506329107,
15.172688996992,15.2451496511092,15.320938380604,15.3946463929566,15.468320170018,
15.5440309579608,15.616894466422,15.6238544618538),.UNSPECIFIED.);
#885=B_SPLINE_CURVE_WITH_KNOTS('',3,(#19763,#19764,#19765,#19766,#19767,
#19768,#19769,#19770,#19771,#19772,#19773,#19774,#19775,#19776,#19777,#19778,
#19779,#19780,#19781,#19782,#19783,#19784,#19785,#19786,#19787,#19788,#19789,
#19790,#19791,#19792,#19793,#19794,#19795,#19796,#19797,#19798,#19799,#19800),
 .UNSPECIFIED.,.F.,.F.,(4,2,2,2,2,2,2,2,2,2,2,2,2,2,2,2,2,2,4),(5.49987666712128,
5.50936969912529,5.58230823770329,5.65810491492989,5.73154304558173,5.80532493915137,
5.8810855957766,5.95346927632274,6.02808199011211,6.10382388051154,6.17656308684462,
6.25213419297739,6.32614937751272,6.39973604327568,6.47626478262863,6.54882068220162,
6.62326404859892,6.6990181768668,6.70124289322726),.UNSPECIFIED.);
#886=B_SPLINE_CURVE_WITH_KNOTS('',3,(#19801,#19802,#19803,#19804,#19805,
#19806,#19807,#19808,#19809,#19810,#19811,#19812,#19813,#19814,#19815,#19816,
#19817,#19818,#19819,#19820,#19821,#19822,#19823,#19824,#19825,#19826,#19827,
#19828,#19829,#19830,#19831,#19832,#19833,#19834,#19835,#19836),
 .UNSPECIFIED.,.F.,.F.,(4,2,2,2,2,2,2,2,2,2,2,2,2,2,2,2,2,4),(15.6238544618538,
15.6932394001919,15.7679616847285,15.8403081894406,15.9160651326732,15.9899553136894,
16.0631834109938,16.1391016155685,16.2121483828073,16.2876906971423,16.362636948483,
16.4349759477711,16.5107227353739,16.584833013443,16.657704448787,16.7338677596132,
16.8071315434702,16.8249604142555),.UNSPECIFIED.);
#887=B_SPLINE_CURVE_WITH_KNOTS('',3,(#19841,#19842,#19843,#19844,#19845,
#19846,#19847,#19848,#19849,#19850,#19851,#19852,#19853,#19854,#19855,#19856,
#19857,#19858,#19859,#19860,#19861,#19862,#19863,#19864,#19865,#19866,#19867,
#19868,#19869,#19870,#19871,#19872,#19873,#19874,#19875,#19876),
 .UNSPECIFIED.,.F.,.F.,(4,2,2,2,2,2,2,2,2,2,2,2,2,2,2,2,2,4),(4.29888383168269,
4.31944357582395,4.39281336408965,4.46909712483566,4.54182615941889,4.61604528467895,
4.6917854903481,4.76415503769022,4.83921257243693,4.91438042167323,4.98751955350481,
5.06354298907082,5.13657441885952,5.21055783230592,5.28629707756517,5.35861581800472,
5.43343286402621,5.49987666712128),.UNSPECIFIED.);
#888=B_SPLINE_CURVE_WITH_KNOTS('',3,(#19877,#19878,#19879,#19880,#19881,
#19882,#19883,#19884,#19885,#19886,#19887,#19888,#19889,#19890,#19891,#19892,
#19893,#19894,#19895,#19896,#19897,#19898,#19899,#19900,#19901,#19902,#19903,
#19904,#19905,#19906,#19907,#19908,#19909,#19910,#19911,#19912),
 .UNSPECIFIED.,.F.,.F.,(4,2,2,2,2,2,2,2,2,2,2,2,2,2,2,2,2,4),(16.8249604142555,
16.8819522219098,16.9571540489601,17.0296070213112,17.1053670193323,17.1797272900657,
17.2523579029735,17.3287952776113,17.4023020941915,17.4765231421258,17.5520028504968,
17.6246597107687,17.7003851939233,17.7749103429322,17.8473232637256,17.9230754686744,
17.9967705304612,18.0262961697653),.UNSPECIFIED.);
#889=B_SPLINE_CURVE_WITH_KNOTS('',3,(#19917,#19918,#19919,#19920,#19921,
#19922,#19923,#19924,#19925,#19926,#19927,#19928,#19929,#19930,#19931,#19932,
#19933,#19934,#19935,#19936,#19937,#19938,#19939,#19940,#19941,#19942,#19943,
#19944,#19945,#19946,#19947,#19948,#19949,#19950,#19951,#19952),
 .UNSPECIFIED.,.F.,.F.,(4,2,2,2,2,2,2,2,2,2,2,2,2,2,2,2,2,4),(3.09726687965577,
3.1293327078715,3.20315237979801,3.27892867777479,3.35131868834466,3.42596958146837,
3.50172952178251,3.57450514884734,3.65011581516003,3.7240870698342,3.79770971006065,
3.87427831122171,3.94682778477419,4.02130828556258,4.09707395257375,4.16961694382427,
4.24494202381471,4.29888383168269),.UNSPECIFIED.);
#890=B_SPLINE_CURVE_WITH_KNOTS('',3,(#19953,#19954,#19955,#19956,#19957,
#19958,#19959,#19960,#19961,#19962,#19963,#19964,#19965,#19966,#19967,#19968,
#19969,#19970,#19971,#19972,#19973,#19974,#19975,#19976,#19977,#19978,#19979,
#19980,#19981,#19982,#19983,#19984,#19985,#19986,#19987,#19988),
 .UNSPECIFIED.,.F.,.F.,(4,2,2,2,2,2,2,2,2,2,2,2,2,2,2,2,2,4),(18.0262961697653,
18.0703605134091,18.14606029023,18.2189115217723,18.2951327104639,18.3698464948732,
18.4421559925931,18.51787876332,18.5917604656892,18.6649130484959,18.7408247221732,
18.8138632321234,18.8892887401014,18.9642303518526,19.0365453779641,19.1122604897676,
19.1863659359319,19.2269385903047),.UNSPECIFIED.);
#891=B_SPLINE_CURVE_WITH_KNOTS('',3,(#19993,#19994,#19995,#19996,#19997,
#19998,#19999,#20000,#20001,#20002,#20003,#20004,#20005,#20006,#20007,#20008,
#20009,#20010,#20011,#20012,#20013,#20014,#20015,#20016,#20017,#20018,#20019,
#20020,#20021,#20022,#20023,#20024,#20025,#20026,#20027,#20028),
 .UNSPECIFIED.,.F.,.F.,(4,2,2,2,2,2,2,2,2,2,2,2,2,2,2,2,2,4),(1.8959795055474,
1.9393592958045,2.01362339134596,2.08938397654367,2.16178410462566,2.23688741543728,
2.31199833731952,2.3851787149032,2.46124709092875,2.53425958502741,2.60828479791366,
2.6840419580893,2.75637837799298,2.83123784888653,2.90710918892568,2.98008539530125,
3.0559230158524,3.09726687965577),.UNSPECIFIED.);
#892=B_SPLINE_CURVE_WITH_KNOTS('',3,(#20029,#20030,#20031,#20032,#20033,
#20034,#20035,#20036,#20037,#20038,#20039,#20040,#20041,#20042,#20043,#20044,
#20045,#20046,#20047,#20048,#20049,#20050,#20051,#20052,#20053,#20054,#20055,
#20056,#20057,#20058,#20059,#20060,#20061,#20062,#20063,#20064),
 .UNSPECIFIED.,.F.,.F.,(4,2,2,2,2,2,2,2,2,2,2,2,2,2,2,2,2,4),(19.2269385903047,
19.2591738665856,19.3353342063483,19.4085929213386,19.4833088738998,19.558508885276,
19.6309515126468,19.7066825650131,19.7810406793351,19.853621686921,19.930058624413,
20.0035626708721,20.0776946111672,20.1531743178055,20.2258295252266,20.3015326258325,
20.3760570414271,20.4278890513381),.UNSPECIFIED.);
#893=B_SPLINE_CURVE_WITH_KNOTS('',3,(#20069,#20070,#20071,#20072,#20073,
#20074,#20075,#20076,#20077,#20078,#20079,#20080,#20081,#20082,#20083,#20084,
#20085,#20086,#20087,#20088,#20089,#20090,#20091,#20092,#20093,#20094,#20095,
#20096,#20097,#20098,#20099,#20100,#20101,#20102,#20103,#20104),
 .UNSPECIFIED.,.F.,.F.,(4,2,2,2,2,2,2,2,2,2,2,2,2,2,2,2,2,4),(0.693996851653457,
0.748401533499502,0.823100571323074,0.898889829797497,0.971711662205941,
1.04737197901952,1.12131453444175,1.19498314402497,1.27160189386835,1.34415795995857,
1.41868569673119,1.49447448163682,1.56706066862621,1.6424338957219,1.71689141144651,
1.79030520660482,1.86663698237822,1.8959795055474),.UNSPECIFIED.);
#894=B_SPLINE_CURVE_WITH_KNOTS('',3,(#20105,#20106,#20107,#20108,#20109,
#20110,#20111,#20112,#20113,#20114,#20115,#20116,#20117,#20118,#20119,#20120,
#20121,#20122,#20123,#20124,#20125,#20126,#20127,#20128,#20129,#20130,#20131,
#20132,#20133,#20134,#20135,#20136,#20137,#20138,#20139,#20140),
 .UNSPECIFIED.,.F.,.F.,(4,2,2,2,2,2,2,2,2,2,2,2,2,2,2,2,2,4),(20.4278890513381,
20.4484340912896,20.5241616208347,20.5978560559012,20.6713731521802,20.7470746205059,
20.8199257271634,20.8960333809615,20.9707512015188,21.0430361070662,21.1187366153993,
21.1926222126879,21.2657107641379,21.3416286508347,21.4146710898949,21.4899906638883,
21.5649401850703,21.6282084253952),.UNSPECIFIED.);
#895=B_SPLINE_CURVE_WITH_KNOTS('',3,(#20146,#20147,#20148,#20149,#20150,
#20151,#20152,#20153,#20154,#20155,#20156,#20157,#20158,#20159,#20160,#20161,
#20162,#20163,#20164,#20165,#20166,#20167,#20168,#20169,#20170,#20171,#20172,
#20173,#20174,#20175,#20176,#20177,#20178,#20179),.UNSPECIFIED.,.F.,.F.,
(4,2,2,2,2,2,2,2,2,2,2,2,2,2,2,2,4),(21.3998620379566,21.4010821380198,
21.4745419758515,21.5484483384161,21.6238885835661,21.6965022150209,21.7721179655765,
21.8466016752083,21.9188674724763,21.994502511453,22.0681568289235,22.1414834717519,
22.2171485887074,22.2899609285255,22.3657908963153,22.4066118716899,22.447261954037),
 .UNSPECIFIED.);
#896=B_SPLINE_CURVE_WITH_KNOTS('',3,(#20182,#20183,#20184,#20185,#20186,
#20187,#20188,#20189,#20190,#20191,#20192,#20193,#20194,#20195,#20196,#20197,
#20198,#20199,#20200,#20201,#20202,#20203,#20204,#20205,#20206,#20207,#20208,
#20209,#20210,#20211),.UNSPECIFIED.,.F.,.F.,(4,2,2,2,2,2,2,2,2,2,2,2,2,
2,4),(9.99999992557917E-7,0.0390553475424834,0.0794268420902697,0.155094300389673,
0.228753948163334,0.302420633338845,0.378175682123393,0.450609245608276,
0.525105867869494,0.600831277267472,0.673461628031261,0.748911544765981,
0.823223502985756,0.896705054014033,0.900735091737263),.UNSPECIFIED.);
#897=B_SPLINE_CURVE_WITH_KNOTS('',3,(#20216,#20217,#20218,#20219,#20220,
#20221,#20222,#20223,#20224,#20225,#20226,#20227,#20228,#20229,#20230,#20231,
#20232,#20233,#20234,#20235,#20236,#20237,#20238,#20239,#20240,#20241,#20242,
#20243,#20244,#20245,#20246,#20247,#20248,#20249,#20250,#20251),
 .UNSPECIFIED.,.F.,.F.,(4,2,2,2,2,2,2,2,2,2,2,2,2,2,2,2,2,4),(20.2007312380072,
20.2134304027239,20.286413815735,20.3615507327354,20.4364439593744,20.5086741450774,
20.5842817477222,20.6583387616512,20.7309759746707,20.8070907732301,20.8803008305636,
20.954756341213,21.0299135327095,21.1023004889085,21.1779300353889,21.2522450006783,
21.3246857908901,21.3998620379566),.UNSPECIFIED.);
#898=B_SPLINE_CURVE_WITH_KNOTS('',3,(#20252,#20253,#20254,#20255,#20256,
#20257,#20258,#20259,#20260,#20261,#20262,#20263,#20264,#20265,#20266,#20267,
#20268,#20269,#20270,#20271,#20272,#20273,#20274,#20275,#20276,#20277,#20278,
#20279,#20280,#20281,#20282,#20283,#20284,#20285,#20286,#20287),
 .UNSPECIFIED.,.F.,.F.,(4,2,2,2,2,2,2,2,2,2,2,2,2,2,2,2,2,4),(0.900735091737263,
0.973113026033783,1.0457827221505,1.12011671494025,1.19588534560907,1.26832549045455,
1.34350027467199,1.41843188079472,1.49167375924559,1.56781129900037,1.64073986869053,
1.7148276667715,1.79058665025377,1.86293090550078,1.93785412351329,2.01352224202086,
2.08655154961337,2.10211990279725),.UNSPECIFIED.);
#899=B_SPLINE_CURVE_WITH_KNOTS('',3,(#20292,#20293,#20294,#20295,#20296,
#20297,#20298,#20299,#20300,#20301,#20302,#20303,#20304,#20305,#20306,#20307,
#20308,#20309,#20310,#20311,#20312,#20313,#20314,#20315,#20316,#20317,#20318,
#20319,#20320,#20321,#20322,#20323,#20324,#20325,#20326,#20327),
 .UNSPECIFIED.,.F.,.F.,(4,2,2,2,2,2,2,2,2,2,2,2,2,2,2,2,2,4),(19.0017088956488,
19.026413597501,19.0990040972824,19.1746164405539,19.2490755302594,19.321350577979,
19.3969846493222,19.4706145700775,19.5439869692317,19.6196247612694,19.6924125917538,
19.768327665187,19.8429852098392,19.9151811574575,19.9907909406617,20.0646168007593,
20.1375714521606,20.2007312380072),.UNSPECIFIED.);
#900=B_SPLINE_CURVE_WITH_KNOTS('',3,(#20328,#20329,#20330,#20331,#20332,
#20333,#20334,#20335,#20336,#20337,#20338,#20339,#20340,#20341,#20342,#20343,
#20344,#20345,#20346,#20347,#20348,#20349,#20350,#20351,#20352,#20353,#20354,
#20355,#20356,#20357,#20358,#20359,#20360,#20361,#20362,#20363),
 .UNSPECIFIED.,.F.,.F.,(4,2,2,2,2,2,2,2,2,2,2,2,2,2,2,2,2,4),(2.10211990279725,
2.16244894936447,2.23574937496902,2.30962213376385,2.38539453398937,2.4577632128723,
2.53246781384893,2.60823013701643,2.68105622872575,2.75672375742662,2.83054621909795,
2.90421795092189,2.98002840864426,3.05254665410568,3.12704873372042,3.20280316035751,
3.27536365707667,3.30365799318677),.UNSPECIFIED.);
#901=B_SPLINE_CURVE_WITH_KNOTS('',3,(#20368,#20369,#20370,#20371,#20372,
#20373,#20374,#20375,#20376,#20377,#20378,#20379,#20380,#20381,#20382,#20383,
#20384,#20385,#20386,#20387,#20388,#20389,#20390,#20391,#20392,#20393,#20394,
#20395,#20396,#20397,#20398,#20399,#20400,#20401,#20402,#20403),
 .UNSPECIFIED.,.F.,.F.,(4,2,2,2,2,2,2,2,2,2,2,2,2,2,2,2,2,4),(17.8023401640365,
17.8389668145887,17.9111936616507,17.9868073571536,18.0608434695502,18.133517651016,
18.2096089813251,18.2827987686193,18.3573324455908,18.4324654961022,18.5048353047865,
18.5804680791381,18.6547595601668,18.7272229946283,18.8035934363314,18.8770308485898,
18.9509991493981,19.0017088956488),.UNSPECIFIED.);
#902=B_SPLINE_CURVE_WITH_KNOTS('',3,(#20404,#20405,#20406,#20407,#20408,
#20409,#20410,#20411,#20412,#20413,#20414,#20415,#20416,#20417,#20418,#20419,
#20420,#20421,#20422,#20423,#20424,#20425,#20426,#20427,#20428,#20429,#20430,
#20431,#20432,#20433,#20434,#20435,#20436,#20437,#20438,#20439),
 .UNSPECIFIED.,.F.,.F.,(4,2,2,2,2,2,2,2,2,2,2,2,2,2,2,2,2,4),(3.30365799318677,
3.35071106186011,3.42511288438873,3.49850057876448,3.57480597153522,3.64748593997752,
3.72172379123405,3.7974491155508,3.86981948936067,3.94489636093728,4.01994685668824,
4.09310036383744,4.16914150257682,4.24210737920037,4.31610544665387,4.39182652214827,
4.46412891541083,4.50446478944951),.UNSPECIFIED.);
#903=B_SPLINE_CURVE_WITH_KNOTS('',3,(#20444,#20445,#20446,#20447,#20448,
#20449,#20450,#20451,#20452,#20453,#20454,#20455,#20456,#20457,#20458,#20459,
#20460,#20461,#20462,#20463,#20464,#20465,#20466,#20467,#20468,#20469,#20470,
#20471,#20472,#20473,#20474,#20475,#20476,#20477,#20478,#20479),
 .UNSPECIFIED.,.F.,.F.,(4,2,2,2,2,2,2,2,2,2,2,2,2,2,2,2,2,4),(16.6032707324218,
16.6513817973194,16.723678768177,16.7993239524381,16.8729409992827,16.9463724810034,
17.0219947252625,17.094769384138,17.170783948967,17.2454238472081,17.3176301069999,
17.3932485807392,17.4670571110006,17.5400615604984,17.6159005169778,17.6888667744311,
17.7640950147645,17.8023401640365),.UNSPECIFIED.);
#904=B_SPLINE_CURVE_WITH_KNOTS('',3,(#20480,#20481,#20482,#20483,#20484,
#20485,#20486,#20487,#20488,#20489,#20490,#20491,#20492,#20493,#20494,#20495,
#20496,#20497,#20498,#20499,#20500,#20501,#20502,#20503,#20504,#20505,#20506,
#20507,#20508,#20509,#20510,#20511,#20512,#20513,#20514,#20515),
 .UNSPECIFIED.,.F.,.F.,(4,2,2,2,2,2,2,2,2,2,2,2,2,2,2,2,2,4),(4.50446478944951,
4.53896099017265,4.61476851462214,4.68771679150871,4.76352599294146,4.83688560323665,
4.91067692380354,4.98641636639118,5.05876849076569,5.13339070946845,5.20911462118278,
5.28186203260248,5.35744396510543,5.43135962875759,5.5049534453086,5.58149289583282,
5.65400014953507,5.70546524065298),.UNSPECIFIED.);
#905=B_SPLINE_CURVE_WITH_KNOTS('',3,(#20520,#20521,#20522,#20523,#20524,
#20525,#20526,#20527,#20528,#20529,#20530,#20531,#20532,#20533,#20534,#20535,
#20536,#20537,#20538,#20539,#20540,#20541,#20542,#20543,#20544,#20545,#20546,
#20547,#20548,#20549,#20550,#20551,#20552,#20553,#20554,#20555),
 .UNSPECIFIED.,.F.,.F.,(4,2,2,2,2,2,2,2,2,2,2,2,2,2,2,2,2,4),(15.4036127818561,
15.4629837689097,15.5357079153789,15.6117880203978,15.68496929525,15.7595946060973,
15.8347155210961,15.9070810189327,15.9827292214831,16.0570090817769,16.1295081903979,
16.2058648944736,16.2792915083073,16.3533352798644,16.4287358039088,16.501314596555,
16.5769356517096,16.6032707324218),.UNSPECIFIED.);
#906=B_SPLINE_CURVE_WITH_KNOTS('',3,(#20556,#20557,#20558,#20559,#20560,
#20561,#20562,#20563,#20564,#20565,#20566,#20567,#20568,#20569,#20570,#20571,
#20572,#20573,#20574,#20575,#20576,#20577,#20578,#20579,#20580,#20581,#20582,
#20583,#20584,#20585,#20586,#20587,#20588,#20589,#20590,#20591),
 .UNSPECIFIED.,.F.,.F.,(4,2,2,2,2,2,2,2,2,2,2,2,2,2,2,2,2,4),(5.70546524065298,
5.72845174646461,5.80417918889931,5.87669291399989,5.95198889447905,6.02642912834167,
6.099769545299,6.17602356503088,6.24870556733163,6.32289513760141,6.39859617033174,
6.47093208541315,6.54595983515997,6.62106144576296,6.69417036178633,6.77016311771506,
6.8431430391509,6.90599013816734),.UNSPECIFIED.);
#907=B_SPLINE_CURVE_WITH_KNOTS('',3,(#20596,#20597,#20598,#20599,#20600,
#20601,#20602,#20603,#20604,#20605,#20606,#20607,#20608,#20609,#20610,#20611,
#20612,#20613,#20614,#20615,#20616,#20617,#20618,#20619,#20620,#20621,#20622,
#20623,#20624,#20625,#20626,#20627,#20628,#20629,#20630,#20631),
 .UNSPECIFIED.,.F.,.F.,(4,2,2,2,2,2,2,2,2,2,2,2,2,2,2,2,2,4),(14.2043028097508,
14.2747055373133,14.3482084709696,14.4238275610328,14.4966009415762,14.5727275919946,
14.6473620165199,14.7195913711808,14.795230680713,14.8690338970156,14.9421008958382,
15.0179321830715,15.0908931142881,15.1662257781497,15.2410882395189,15.3133246655807,
15.3889566201665,15.4036127818561),.UNSPECIFIED.);
#908=B_SPLINE_CURVE_WITH_KNOTS('',3,(#20632,#20633,#20634,#20635,#20636,
#20637,#20638,#20639,#20640,#20641,#20642,#20643,#20644,#20645,#20646,#20647,
#20648,#20649,#20650,#20651,#20652,#20653,#20654,#20655,#20656,#20657,#20658,
#20659,#20660,#20661,#20662,#20663,#20664,#20665,#20666,#20667,#20668,#20669),
 .UNSPECIFIED.,.F.,.F.,(4,2,2,2,2,2,2,2,2,2,2,2,2,2,2,2,2,2,4),(6.90599013816734,
6.91709591054206,6.99279511544632,7.06507570458308,7.13986191697079,7.21572907571421,
7.28863624774249,7.36440096151241,7.43778401952338,7.51153406441721,7.58725386603195,
7.65959537324807,7.73417586888514,7.80987775822848,7.88258527044843,7.95812405247512,
8.03207835995344,8.10563264968525,8.10649808593899),.UNSPECIFIED.);
#909=B_SPLINE_CURVE_WITH_KNOTS('',3,(#20674,#20675,#20676,#20677,#20678,
#20679,#20680,#20681,#20682,#20683,#20684,#20685,#20686,#20687,#20688,#20689,
#20690,#20691,#20692,#20693,#20694,#20695,#20696,#20697,#20698,#20699,#20700,
#20701,#20702,#20703,#20704,#20705,#20706,#20707,#20708,#20709,#20710,#20711),
 .UNSPECIFIED.,.F.,.F.,(4,2,2,2,2,2,2,2,2,2,2,2,2,2,2,2,2,2,4),(13.0043185145707,
13.0131961618393,13.0863810742337,13.1611097586802,13.2362310180851,13.3086053228822,
13.3842810516299,13.4585616154906,13.5311088763717,13.6074645223847,13.6808924755368,
13.7550239419564,13.8304229984377,13.9030020346595,13.9786440351523,14.0530894710899,
14.1254208536733,14.2010892882464,14.2043028097508),.UNSPECIFIED.);
#910=B_SPLINE_CURVE_WITH_KNOTS('',3,(#20712,#20713,#20714,#20715,#20716,
#20717,#20718,#20719,#20720,#20721,#20722,#20723,#20724,#20725,#20726,#20727,
#20728,#20729,#20730,#20731,#20732,#20733,#20734,#20735,#20736,#20737,#20738,
#20739,#20740,#20741,#20742,#20743,#20744,#20745,#20746,#20747),
 .UNSPECIFIED.,.F.,.F.,(4,2,2,2,2,2,2,2,2,2,2,2,2,2,2,2,2,4),(8.10649808593899,
8.18212857782179,8.25463769233127,8.32904856291924,8.40476039560251,8.47723808436404,
8.55249249244931,8.6269871616477,8.70029010543794,8.77650284076587,8.84920045806996,
8.92335167723176,8.99903990378592,9.07135287698761,9.14634154317815,9.22151071619755,
9.29458504609435,9.30692725994904),.UNSPECIFIED.);
#911=B_SPLINE_CURVE_WITH_KNOTS('',3,(#20752,#20753,#20754,#20755,#20756,
#20757,#20758,#20759,#20760,#20761,#20762,#20763,#20764,#20765,#20766,#20767,
#20768,#20769,#20770,#20771,#20772,#20773,#20774,#20775,#20776,#20777,#20778,
#20779,#20780,#20781,#20782,#20783,#20784,#20785,#20786,#20787),
 .UNSPECIFIED.,.F.,.F.,(4,2,2,2,2,2,2,2,2,2,2,2,2,2,2,2,2,4),(11.8045357693031,
11.8246955167202,11.8974797480381,11.973728941363,12.048370394829,12.1206353038175,
12.1963073859733,12.2701176287412,12.3432587958549,12.4190951183632,12.4920628764287,
12.5675110699007,12.6423766978021,12.714635590817,12.7902978126314,12.8643283394953,
12.9371145822676,13.0043185145707),.UNSPECIFIED.);
#912=B_SPLINE_CURVE_WITH_KNOTS('',3,(#20788,#20789,#20790,#20791,#20792,
#20793,#20794,#20795,#20796,#20797,#20798,#20799,#20800,#20801,#20802,#20803,
#20804,#20805,#20806,#20807,#20808,#20809,#20810,#20811,#20812,#20813,#20814,
#20815,#20816,#20817,#20818,#20819,#20820,#20821,#20822,#20823),
 .UNSPECIFIED.,.F.,.F.,(4,2,2,2,2,2,2,2,2,2,2,2,2,2,2,2,2,4),(9.30692725994904,
9.37053973428254,9.4435477643714,9.51746559946554,9.59315452652494,9.66542543740846,
9.74017607133259,9.81611935995928,9.88899567467958,9.96472648537345,10.0381472533,
10.1118664472855,10.1875783107606,10.2599216974399,10.3344710332621,10.4101625475177,
10.4828405221781,10.507197202247),.UNSPECIFIED.);
#913=B_SPLINE_CURVE_WITH_KNOTS('',3,(#20828,#20829,#20830,#20831,#20832,
#20833,#20834,#20835,#20836,#20837,#20838,#20839,#20840,#20841,#20842,#20843,
#20844,#20845,#20846,#20847,#20848,#20849,#20850,#20851,#20852,#20853,#20854,
#20855,#20856,#20857,#20858,#20859,#20860,#20861,#20862,#20863),
 .UNSPECIFIED.,.F.,.F.,(4,2,2,2,2,2,2,2,2,2,2,2,2,2,2,2,2,4),(10.6039329181875,
10.6363651346832,10.7124501879071,10.7853405670855,10.8610838827621,10.934599898383,
11.008333799212,11.0840882660137,11.156484544635,11.2310488243127,11.3036402546897,
11.3793152266208,11.4537724131331,11.5261501395238,11.6018537056525,11.6754814591988,
11.7490669060118,11.8045357693031),.UNSPECIFIED.);
#914=B_SPLINE_CURVE_WITH_KNOTS('',3,(#20864,#20865,#20866,#20867,#20868,
#20869,#20870,#20871,#20872,#20873,#20874,#20875,#20876,#20877,#20878,#20879,
#20880,#20881,#20882,#20883,#20884,#20885,#20886,#20887,#20888,#20889,#20890,
#20891,#20892,#20893,#20894,#20895,#20896,#20897,#20898,#20899),
 .UNSPECIFIED.,.F.,.F.,(4,2,2,2,2,2,2,2,2,2,2,2,2,2,2,2,2,4),(10.507197202247,
10.5583468648772,10.6323548055098,10.7058801425724,10.7823434678229,10.8548676450864,
10.929248488786,11.004956589598,11.0774099932164,11.1526336429167,11.2271981730393,
11.3029101516168,11.3766290823305,11.4500507067516,11.5257812108603,11.5986572591126,
11.6746020373567,11.7077777116762),.UNSPECIFIED.);
#915=B_SPLINE_CURVE_WITH_KNOTS('',3,(#20904,#20905,#20906,#20907,#20908,
#20909,#20910,#20911,#20912,#20913,#20914,#20915,#20916,#20917,#20918,#20919,
#20920,#20921,#20922,#20923,#20924,#20925,#20926,#20927,#20928,#20929,#20930,
#20931,#20932,#20933,#20934,#20935,#20936,#20937,#20938,#20939),
 .UNSPECIFIED.,.F.,.F.,(4,2,2,2,2,2,2,2,2,2,2,2,2,2,2,2,2,4),(9.40314292363424,
9.44807926432923,9.52269054080882,9.59599985679214,9.67221651690302,9.74498383159651,
9.81914102601776,9.8948661844282,9.96720341425604,10.0421977895991,10.1174988854888,
10.1905829359148,10.2665452811273,10.3396376931852,10.413565359407,10.4892941509423,
10.5616047072099,10.6039329181875),.UNSPECIFIED.);
#916=B_SPLINE_CURVE_WITH_KNOTS('',3,(#20940,#20941,#20942,#20943,#20944,
#20945,#20946,#20947,#20948,#20949,#20950,#20951,#20952,#20953,#20954,#20955,
#20956,#20957,#20958,#20959,#20960,#20961,#20962,#20963,#20964,#20965,#20966,
#20967,#20968,#20969,#20970,#20971,#20972,#20973,#20974,#20975),
 .UNSPECIFIED.,.F.,.F.,(4,2,2,2,2,2,2,2,2,2,2,2,2,2,2,2,2,4),(11.7077777116762,
11.7493523337136,11.8216233292765,11.8973123329413,11.9712298364502,12.0442385684753,
12.1201928820956,12.1932668846388,12.2684374097942,12.3434256811156,12.4157385236044,
12.4914267857389,12.5655776191594,12.6382757357031,12.7144880439345,12.7877906132398,
12.8622864217306,12.9079875737808),.UNSPECIFIED.);
#917=B_SPLINE_CURVE_WITH_KNOTS('',3,(#20980,#20981,#20982,#20983,#20984,
#20985,#20986,#20987,#20988,#20989,#20990,#20991,#20992,#20993,#20994,#20995,
#20996,#20997,#20998,#20999,#21000,#21001,#21002,#21003,#21004,#21005,#21006,
#21007,#21008,#21009,#21010,#21011,#21012,#21013,#21014,#21015),
 .UNSPECIFIED.,.F.,.F.,(4,2,2,2,2,2,2,2,2,2,2,2,2,2,2,2,2,4),(8.20191590591913,
8.25960106122842,8.33306373764413,8.40681574654923,8.48256448506601,8.55494444504399,
8.62952697206071,8.70525502991575,8.77796547717747,8.85350532364393,8.92755759145257,
9.00111590817091,9.07761319994366,9.15017581215132,9.22458992342226,9.30033545956258,
9.37282202157872,9.40314292363424),.UNSPECIFIED.);
#918=B_SPLINE_CURVE_WITH_KNOTS('',3,(#21016,#21017,#21018,#21019,#21020,
#21021,#21022,#21023,#21024,#21025,#21026,#21027,#21028,#21029,#21030,#21031,
#21032,#21033,#21034,#21035,#21036,#21037,#21038,#21039,#21040,#21041,#21042,
#21043,#21044,#21045,#21046,#21047,#21048,#21049,#21050,#21051),
 .UNSPECIFIED.,.F.,.F.,(4,2,2,2,2,2,2,2,2,2,2,2,2,2,2,2,2,4),(12.9079875737808,
12.937540394313,13.0100177383184,13.0857295612112,13.1601400073282,13.2326493964309,
13.309144861033,13.3826987428871,13.4566539318281,13.5321922527912,13.6048993478474,
13.6806011226957,13.7551811771442,13.8275227529135,13.9032424787233,13.976992086904,
14.0503757757738,14.1087366371979),.UNSPECIFIED.);
#919=B_SPLINE_CURVE_WITH_KNOTS('',3,(#21056,#21057,#21058,#21059,#21060,
#21061,#21062,#21063,#21064,#21065,#21066,#21067,#21068,#21069,#21070,#21071,
#21072,#21073,#21074,#21075,#21076,#21077,#21078,#21079,#21080,#21081,#21082,
#21083,#21084,#21085,#21086,#21087,#21088,#21089,#21090,#21091),
 .UNSPECIFIED.,.F.,.F.,(4,2,2,2,2,2,2,2,2,2,2,2,2,2,2,2,2,4),(7.00118688689761,
7.07080206795146,7.14353831016436,7.21772153799166,7.29344597627649,7.36579219781796,
7.44081319493958,7.51602919589249,7.58913550527881,7.66512315080874,7.73817162506754,
7.81212180542193,7.88784728261179,7.96015319704089,8.03493652227658,8.11092813520778,
8.18383683814882,8.20191590591913),.UNSPECIFIED.);
#920=B_SPLINE_CURVE_WITH_KNOTS('',3,(#21092,#21093,#21094,#21095,#21096,
#21097,#21098,#21099,#21100,#21101,#21102,#21103,#21104,#21105,#21106,#21107,
#21108,#21109,#21110,#21111,#21112,#21113,#21114,#21115,#21116,#21117,#21118,
#21119,#21120,#21121,#21122,#21123,#21124,#21125,#21126,#21127),
 .UNSPECIFIED.,.F.,.F.,(4,2,2,2,2,2,2,2,2,2,2,2,2,2,2,2,2,4),(14.1087366371979,
14.1261400064869,14.1990467415146,14.274915133928,14.3497008369486,14.4219813121166,
14.497680404552,14.5716327746707,14.6446131737348,14.7206053824683,14.7937138040713,
14.8688165097389,14.9438436963948,15.016179289806,15.0918801703987,15.1660691885856,
15.2387514714241,15.3090799178937),.UNSPECIFIED.);
#921=B_SPLINE_CURVE_WITH_KNOTS('',3,(#21132,#21133,#21134,#21135,#21136,
#21137,#21138,#21139,#21140,#21141,#21142,#21143,#21144,#21145,#21146,#21147,
#21148,#21149,#21150,#21151,#21152,#21153,#21154,#21155,#21156,#21157,#21158,
#21159,#21160,#21161,#21162,#21163,#21164,#21165,#21166,#21167,#21168,#21169),
 .UNSPECIFIED.,.F.,.F.,(4,2,2,2,2,2,2,2,2,2,2,2,2,2,2,2,2,2,4),(5.79993999134698,
5.80524971510209,5.88100482499339,5.95338123541158,6.02799348446614,6.10373035479458,
6.17646893000621,6.2520397566395,6.32603643947841,6.39962227107694,6.4761506781555,
6.54869647616329,6.62313915849589,6.69888684027576,6.77139608977099,6.84668261898845,
6.9212220444047,6.99455668680605,7.00118688689761),.UNSPECIFIED.);
#922=B_SPLINE_CURVE_WITH_KNOTS('',3,(#21170,#21171,#21172,#21173,#21174,
#21175,#21176,#21177,#21178,#21179,#21180,#21181,#21182,#21183,#21184,#21185,
#21186,#21187,#21188,#21189,#21190,#21191,#21192,#21193,#21194,#21195,#21196,
#21197,#21198,#21199,#21200,#21201,#21202,#21203,#21204,#21205,#21206,#21207),
 .UNSPECIFIED.,.F.,.F.,(4,2,2,2,2,2,2,2,2,2,2,2,2,2,2,2,2,2,4),(15.3090799178937,
15.3150048947458,15.3883447730857,15.4627858935473,15.5380812730832,15.6105944732051,
15.6863217194936,15.7607727281917,15.8332800474004,15.9098188675437,15.983412114232,
16.0573284163402,16.1329097241255,16.2056565597743,16.2813801753304,16.3560017912743,
16.4283537881353,16.5040929719216,16.5100414867088),.UNSPECIFIED.);
#923=B_SPLINE_CURVE_WITH_KNOTS('',3,(#21212,#21213,#21214,#21215,#21216,
#21217,#21218,#21219,#21220,#21221,#21222,#21223,#21224,#21225,#21226,#21227,
#21228,#21229,#21230,#21231,#21232,#21233,#21234,#21235,#21236,#21237,#21238,
#21239,#21240,#21241,#21242,#21243,#21244,#21245,#21246,#21247),
 .UNSPECIFIED.,.F.,.F.,(4,2,2,2,2,2,2,2,2,2,2,2,2,2,2,2,2,4),(4.5990670002631,
4.61605684680242,4.69179254909771,4.76416014599027,4.83921885367157,4.91436515169427,
4.98750468221458,5.06352898580182,5.13654749103522,5.21053132121442,5.28626552208576,
5.35857948073502,5.43339698071682,5.5093103302291,5.58224849564028,5.65804517900355,
5.73146827412131,5.79993999134698),.UNSPECIFIED.);
#924=B_SPLINE_CURVE_WITH_KNOTS('',3,(#21248,#21249,#21250,#21251,#21252,
#21253,#21254,#21255,#21256,#21257,#21258,#21259,#21260,#21261,#21262,#21263,
#21264,#21265,#21266,#21267,#21268,#21269,#21270,#21271,#21272,#21273,#21274,
#21275,#21276,#21277,#21278,#21279,#21280,#21281,#21282,#21283),
 .UNSPECIFIED.,.F.,.F.,(4,2,2,2,2,2,2,2,2,2,2,2,2,2,2,2,2,4),(16.5100414867088,
16.5778836963156,16.6512437083802,16.7270522652006,16.7999999483695,16.875808436759,
16.9506398455013,17.0229419365147,17.0986627186034,17.1726601299846,17.2456262600853,
17.3216666947875,17.3948195550358,17.4698708787336,17.5449470347907,17.6173169102686,
17.6930419035619,17.7107202775431),.UNSPECIFIED.);
#925=B_SPLINE_CURVE_WITH_KNOTS('',3,(#21288,#21289,#21290,#21291,#21292,
#21293,#21294,#21295,#21296,#21297,#21298,#21299,#21300,#21301,#21302,#21303,
#21304,#21305,#21306,#21307,#21308,#21309,#21310,#21311,#21312,#21313,#21314,
#21315,#21316,#21317,#21318,#21319,#21320,#21321,#21322,#21323),
 .UNSPECIFIED.,.F.,.F.,(4,2,2,2,2,2,2,2,2,2,2,2,2,2,2,2,2,4),(3.3975365581224,
3.42602438710494,3.5017817905074,3.57455897160418,3.65017161489103,3.7241276379769,
3.79775167506893,3.87432224447071,3.94686445750292,4.02134653058967,4.09710829208354,
4.16965210409428,4.24497885654866,4.31946174601459,4.39283252180053,4.46911780612146,
4.54183662559879,4.5990670002631),.UNSPECIFIED.);
#926=B_SPLINE_CURVE_WITH_KNOTS('',3,(#21324,#21325,#21326,#21327,#21328,
#21329,#21330,#21331,#21332,#21333,#21334,#21335,#21336,#21337,#21338,#21339,
#21340,#21341,#21342,#21343,#21344,#21345,#21346,#21347,#21348,#21349,#21350,
#21351,#21352,#21353,#21354,#21355,#21356,#21357,#21358,#21359),
 .UNSPECIFIED.,.F.,.F.,(4,2,2,2,2,2,2,2,2,2,2,2,2,2,2,2,2,4),(17.7107202775431,
17.7672790518916,17.8399590864096,17.9162637298069,17.9896507365271,18.0640531875706,
18.1393998421222,18.2119596512683,18.2877137050319,18.3622150485036,18.434733158509,
18.5105432221001,18.5842142230993,18.658037094598,18.7337038356029,18.8065291945043,
18.8822910488291,18.9121502857923),.UNSPECIFIED.);
#927=B_SPLINE_CURVE_WITH_KNOTS('',3,(#21364,#21365,#21366,#21367,#21368,
#21369,#21370,#21371,#21372,#21373,#21374,#21375,#21376,#21377,#21378,#21379,
#21380,#21381,#21382,#21383,#21384,#21385,#21386,#21387,#21388,#21389,#21390,
#21391,#21392,#21393,#21394,#21395,#21396,#21397,#21398,#21399),
 .UNSPECIFIED.,.F.,.F.,(4,2,2,2,2,2,2,2,2,2,2,2,2,2,2,2,2,4),(2.19630130324308,
2.23699605736667,2.31208902084933,2.38527190148058,2.46134331220889,2.53434591982495,
2.60837368609728,2.68412827430948,2.75646249211865,2.83132457944634,2.90717605118273,
2.98015404422193,3.05599389927964,3.12939165042261,3.20321306725771,3.27898631713552,
3.3513717320634,3.3975365581224),.UNSPECIFIED.);
#928=B_SPLINE_CURVE_WITH_KNOTS('',3,(#21400,#21401,#21402,#21403,#21404,
#21405,#21406,#21407,#21408,#21409,#21410,#21411,#21412,#21413,#21414,#21415,
#21416,#21417,#21418,#21419,#21420,#21421,#21422,#21423,#21424,#21425,#21426,
#21427,#21428,#21429,#21430,#21431,#21432,#21433,#21434,#21435),
 .UNSPECIFIED.,.F.,.F.,(4,2,2,2,2,2,2,2,2,2,2,2,2,2,2,2,2,4),(18.9121502857923,
18.9569948872441,19.029363239932,19.1051352086863,19.1790072138826,19.2523078208173,
19.3282044162291,19.4012329759683,19.4769018075669,19.5518242052145,19.6241679619349,
19.6999264806165,19.774013470379,19.8469420709271,19.9230787522869,19.996319834517,
20.071252010965,20.1134543703229),.UNSPECIFIED.);
#929=B_SPLINE_CURVE_WITH_KNOTS('',3,(#21440,#21441,#21442,#21443,#21444,
#21445,#21446,#21447,#21448,#21449,#21450,#21451,#21452,#21453,#21454,#21455,
#21456,#21457,#21458,#21459,#21460,#21461,#21462,#21463,#21464,#21465,#21466,
#21467,#21468,#21469,#21470,#21471,#21472,#21473,#21474,#21475),
 .UNSPECIFIED.,.F.,.F.,(4,2,2,2,2,2,2,2,2,2,2,2,2,2,2,2,2,4),(0.994462254792754,
1.04749156011108,1.12142218453664,1.19509421741773,1.27171701403914,1.34426856529834,
1.41879991994479,1.49458721880891,1.56717647764929,1.64255344225318,1.71699577898508,
1.7904126205899,1.86674803540827,1.93946305186304,2.01373032787344,2.08948885623164,
2.16188946682002,2.19630130324308),.UNSPECIFIED.);
#930=B_SPLINE_CURVE_WITH_KNOTS('',3,(#21476,#21477,#21478,#21479,#21480,
#21481,#21482,#21483,#21484,#21485,#21486,#21487,#21488,#21489,#21490,#21491,
#21492,#21493,#21494,#21495,#21496,#21497,#21498,#21499,#21500,#21501,#21502,
#21503,#21504,#21505,#21506,#21507,#21508,#21509,#21510,#21511),
 .UNSPECIFIED.,.F.,.F.,(4,2,2,2,2,2,2,2,2,2,2,2,2,2,2,2,2,4),(20.1134543703229,
20.1464259304583,20.2188653895587,20.2946335188956,20.3689666613071,20.4416362056508,
20.51804328322,20.5915240830594,20.665836496343,20.7412856015319,20.8139151933508,
20.8896400971914,20.9641359268394,21.0365692298324,21.1123238022716,21.1859897017057,
21.2596495896079,21.3148424617523),.UNSPECIFIED.);
#931=B_SPLINE_CURVE_WITH_KNOTS('',3,(#21518,#21519,#21520,#21521,#21522,
#21523,#21524,#21525,#21526,#21527,#21528,#21529,#21530,#21531),
 .UNSPECIFIED.,.F.,.F.,(4,2,2,2,2,2,4),(9.99999998850988E-7,0.0516169518680174,
0.104845041291632,0.181709819458214,0.255107103717481,0.330970348449006,
0.40012180130331),.UNSPECIFIED.);
#932=B_SPLINE_CURVE_WITH_KNOTS('',3,(#21537,#21538,#21539,#21540,#21541,
#21542,#21543,#21544,#21545,#21546,#21547,#21548,#21549,#21550,#21551,#21552),
 .UNSPECIFIED.,.F.,.F.,(4,2,2,2,2,2,2,4),(7.19320368172551,7.22969104326796,
7.30685234317664,7.3810857236285,7.45736679269846,7.53354842516138,7.60230579027905,
7.67143903153145),.UNSPECIFIED.);
#933=B_SPLINE_CURVE_WITH_KNOTS('',3,(#21554,#21555,#21556,#21557,#21558,
#21559,#21560,#21561,#21562,#21563,#21564,#21565,#21566,#21567,#21568,#21569,
#21570,#21571,#21572,#21573,#21574,#21575,#21576,#21577,#21578,#21579,#21580,
#21581,#21582,#21583,#21584,#21585,#21586,#21587,#21588,#21589,#21590,#21591),
 .UNSPECIFIED.,.F.,.F.,(4,2,2,2,2,2,2,2,2,2,2,2,2,2,2,2,2,2,4),(0.40012180130331,
0.408263585102685,0.48223140566233,0.559093024369444,0.633749160630985,
0.7085728423697,0.785465068742682,0.858957556763468,0.934624119514201,1.0114910968397,
1.08525873800664,1.16189369275507,1.23717718819415,1.31180620569013,1.38941296914438,
1.46311419611182,1.53861020423359,1.61550600313119,1.61947369254408),
 .UNSPECIFIED.);
#934=B_SPLINE_CURVE_WITH_KNOTS('',3,(#21596,#21597,#21598,#21599,#21600,
#21601,#21602,#21603,#21604,#21605,#21606,#21607,#21608,#21609,#21610,#21611,
#21612,#21613,#21614,#21615,#21616,#21617,#21618,#21619,#21620,#21621,#21622,
#21623,#21624,#21625,#21626,#21627,#21628,#21629,#21630,#21631),
 .UNSPECIFIED.,.F.,.F.,(4,2,2,2,2,2,2,2,2,2,2,2,2,2,2,2,2,4),(5.97412374915921,
6.02336400908153,6.10006341983446,6.17388859911262,6.25076071689292,6.32648861381787,
6.39995163611774,6.47684257850208,6.55172701295907,6.62625691294416,6.70318696736095,
6.77721590254118,6.85427849813963,6.93021529133003,7.0036137704599,7.08048358099157,
7.15557375602929,7.19320368172551),.UNSPECIFIED.);
#935=B_SPLINE_CURVE_WITH_KNOTS('',3,(#21632,#21633,#21634,#21635,#21636,
#21637,#21638,#21639,#21640,#21641,#21642,#21643,#21644,#21645,#21646,#21647,
#21648,#21649,#21650,#21651,#21652,#21653,#21654,#21655,#21656,#21657,#21658,
#21659,#21660,#21661,#21662,#21663,#21664,#21665,#21666,#21667),
 .UNSPECIFIED.,.F.,.F.,(4,2,2,2,2,2,2,2,2,2,2,2,2,2,2,2,2,4),(1.61947369254408,
1.68905949729837,1.76541133090778,1.84129353055796,1.91567439290728,1.99300112987828,
2.06693716068424,2.14217746504849,2.21905840786482,2.29248563659418,2.36857555377319,
2.44518301605857,2.51934077538404,2.59641539895315,2.67070516811205,2.74571872212431,
2.82260805308708,2.83860378589876),.UNSPECIFIED.);
#936=B_SPLINE_CURVE_WITH_KNOTS('',3,(#21672,#21673,#21674,#21675,#21676,
#21677,#21678,#21679,#21680,#21681,#21682,#21683,#21684,#21685,#21686,#21687,
#21688,#21689,#21690,#21691,#21692,#21693,#21694,#21695,#21696,#21697,#21698,
#21699,#21700,#21701,#21702,#21703,#21704,#21705,#21706,#21707),
 .UNSPECIFIED.,.F.,.F.,(4,2,2,2,2,2,2,2,2,2,2,2,2,2,2,2,2,4),(4.75497373082595,
4.81676779439483,4.89291059092831,4.96634139895796,5.04320276423669,5.11849451622994,
5.19232799860222,5.26971286679952,5.34414356990701,5.41981447495191,5.49622630207658,
5.56981970532191,5.6467031993106,5.72225738249546,5.79589351190913,5.87356474205255,
5.94824936086062,5.97412374915921),.UNSPECIFIED.);
#937=B_SPLINE_CURVE_WITH_KNOTS('',3,(#21708,#21709,#21710,#21711,#21712,
#21713,#21714,#21715,#21716,#21717,#21718,#21719,#21720,#21721,#21722,#21723,
#21724,#21725,#21726,#21727,#21728,#21729,#21730,#21731,#21732,#21733,#21734,
#21735,#21736,#21737,#21738,#21739,#21740,#21741,#21742,#21743),
 .UNSPECIFIED.,.F.,.F.,(4,2,2,2,2,2,2,2,2,2,2,2,2,2,2,2,2,4),(2.83860378589876,
2.89603271526497,2.97189145574824,3.04931019004864,3.12327790223017,3.20013738661533,
3.27487393439905,3.34969805164721,3.42661722293439,3.50014925659483,3.57581635011919,
3.65270773672471,3.72647689856381,3.80311152982859,3.87849324951609,3.95312500868852,
4.03073191878357,4.05823923276311),.UNSPECIFIED.);
#938=B_SPLINE_CURVE_WITH_KNOTS('',3,(#21748,#21749,#21750,#21751,#21752,
#21753,#21754,#21755,#21756,#21757,#21758,#21759,#21760,#21761,#21762,#21763,
#21764,#21765,#21766,#21767,#21768,#21769,#21770,#21771,#21772,#21773,#21774,
#21775,#21776,#21777,#21778,#21779,#21780,#21781,#21782,#21783),
 .UNSPECIFIED.,.F.,.F.,(4,2,2,2,2,2,2,2,2,2,2,2,2,2,2,2,2,4),(3.53614671007338,
3.60978705097125,3.68629180592067,3.76172365012633,3.83623446884164,3.91108901947874,
3.98566617435956,4.06256304463242,4.13656203704878,4.21371517669569,4.289616859908,
4.36300950126705,4.43987265648916,4.51492830685511,4.58908233354689,4.6662059935342,
4.74040545873923,4.75497373082595),.UNSPECIFIED.);
#939=B_SPLINE_CURVE_WITH_KNOTS('',3,(#21784,#21785,#21786,#21787,#21788,
#21789,#21790,#21791,#21792,#21793,#21794,#21795,#21796,#21797,#21798,#21799,
#21800,#21801,#21802,#21803,#21804,#21805,#21806,#21807,#21808,#21809,#21810,
#21811,#21812,#21813,#21814,#21815,#21816,#21817,#21818,#21819),
 .UNSPECIFIED.,.F.,.F.,(4,2,2,2,2,2,2,2,2,2,2,2,2,2,2,2,2,4),(4.05823923276311,
4.10448780523323,4.17998586227126,4.25691320464737,4.33047807862384,4.40683152944232,
4.48029143252306,4.5572212291454,4.63229802958326,4.70658708030576,4.78372874807228,
4.8579491025357,4.93451870778849,5.01067645232983,5.08415139575935,5.1610751136448,
5.23638220426729,5.27807262241528),.UNSPECIFIED.);
#940=B_SPLINE_CURVE_WITH_KNOTS('',3,(#21824,#21825,#21826,#21827,#21828,
#21829,#21830,#21831,#21832,#21833,#21834,#21835,#21836,#21837,#21838,#21839,
#21840,#21841,#21842,#21843,#21844,#21845,#21846,#21847,#21848,#21849,#21850,
#21851,#21852,#21853,#21854,#21855,#21856,#21857,#21858,#21859,#21860,#21861),
 .UNSPECIFIED.,.F.,.F.,(4,2,2,2,2,2,2,2,2,2,2,2,2,2,2,2,2,2,4),(2.31659118770115,
2.32826973319217,2.40239574110813,2.47943317469564,2.55383013302291,2.62881186695812,
2.70572051605027,2.7791742554401,2.85500063903863,2.93262228782763,3.00656660516336,
3.08339822550777,3.15825784805007,3.23305942009264,3.31000255015091,3.38358499197676,
3.4592295195039,3.53611466606664,3.53614671007338),.UNSPECIFIED.);
#941=B_SPLINE_CURVE_WITH_KNOTS('',3,(#21862,#21863,#21864,#21865,#21866,
#21867,#21868,#21869,#21870,#21871,#21872,#21873,#21874,#21875,#21876,#21877,
#21878,#21879,#21880,#21881,#21882,#21883,#21884,#21885,#21886,#21887,#21888,
#21889,#21890,#21891,#21892,#21893,#21894,#21895,#21896,#21897),
 .UNSPECIFIED.,.F.,.F.,(4,2,2,2,2,2,2,2,2,2,2,2,2,2,2,2,2,4),(5.27807262241528,
5.31032878063387,5.38772603381421,5.46217259388101,5.53802804503023,5.61445048702391,
5.68806469121006,5.76500582066864,5.84057124764373,5.9142960449069,5.991975837307,
6.06667282701779,6.14194400467577,6.21865141096818,6.29248720387191,6.36940565933153,
6.44514297831244,6.49826455965138),.UNSPECIFIED.);
#942=B_SPLINE_CURVE_WITH_KNOTS('',3,(#21903,#21904,#21905,#21906,#21907,
#21908,#21909,#21910,#21911,#21912,#21913,#21914,#21915,#21916,#21917,#21918,
#21919,#21920,#21921,#21922,#21923,#21924,#21925,#21926,#21927,#21928,#21929,
#21930,#21931,#21932,#21933,#21934,#21935,#21936),.UNSPECIFIED.,.F.,.F.,
(4,2,2,2,2,2,2,2,2,2,2,2,2,2,2,2,4),(7.71789666424489,7.72653208826837,
7.80344520584536,7.87877178630723,7.95267300617573,8.030092507589,8.10455789544369,
8.18032197698524,8.25676746857915,8.33039655432369,8.40733016361098,8.48291789543391,
8.55661319786207,8.63431788624882,8.70903611278883,8.76144236640241,8.8157845358832),
 .UNSPECIFIED.);
#943=B_SPLINE_CURVE_WITH_KNOTS('',3,(#21939,#21940,#21941,#21942,#21943,
#21944,#21945,#21946,#21947,#21948,#21949,#21950,#21951,#21952,#21953,#21954,
#21955,#21956,#21957,#21958,#21959,#21960,#21961,#21962,#21963,#21964,#21965,
#21966,#21967,#21968,#21969,#21970),.UNSPECIFIED.,.F.,.F.,(4,2,2,2,2,2,
2,2,2,2,2,2,2,2,2,4),(3.04265172955979E-8,0.0696297941849091,0.137949529099503,
0.213754729172505,0.291233561600052,0.365153025689182,0.441960629532694,
0.516719666380062,0.591495500873055,0.668388103886677,0.741907722473969,
0.81752609162172,0.894388800621883,0.968111365668341,1.044695954011,1.09710239300357),
 .UNSPECIFIED.);
#944=B_SPLINE_CURVE_WITH_KNOTS('',3,(#21977,#21978,#21979,#21980,#21981,
#21982,#21983,#21984,#21985,#21986,#21987,#21988,#21989,#21990),
 .UNSPECIFIED.,.F.,.F.,(4,2,2,2,2,2,4),(0.,0.0516156037256129,0.104843298805831,
0.181708269088802,0.255105736797692,0.330969171143205,0.40012079681341),
 .UNSPECIFIED.);
#945=B_SPLINE_CURVE_WITH_KNOTS('',3,(#21996,#21997,#21998,#21999,#22000,
#22001,#22002,#22003,#22004,#22005,#22006,#22007,#22008,#22009,#22010,#22011),
 .UNSPECIFIED.,.F.,.F.,(4,2,2,2,2,2,2,4),(7.19320368173748,7.22969104328008,
7.30685234318868,7.38108572364049,7.45736679271042,7.5335484251732,7.60230579029071,
7.67143903154297),.UNSPECIFIED.);
#946=B_SPLINE_CURVE_WITH_KNOTS('',3,(#22013,#22014,#22015,#22016,#22017,
#22018,#22019,#22020,#22021,#22022,#22023,#22024,#22025,#22026,#22027,#22028,
#22029,#22030,#22031,#22032,#22033,#22034,#22035,#22036,#22037,#22038,#22039,
#22040,#22041,#22042,#22043,#22044,#22045,#22046,#22047,#22048,#22049,#22050),
 .UNSPECIFIED.,.F.,.F.,(4,2,2,2,2,2,2,2,2,2,2,2,2,2,2,2,2,2,4),(0.40012079681341,
0.408262580632944,0.482230401205284,0.559092019925671,0.63374815619767,
0.70857183794918,0.785464064334543,0.85895655236679,0.934623115130469,1.01149009246842,
1.08525773364797,1.16189268840959,1.23717618385871,1.31180520136737,1.38941196483489,
1.46311319181338,1.53860919994804,1.61550499885784,1.6194726882503),
 .UNSPECIFIED.);
#947=B_SPLINE_CURVE_WITH_KNOTS('',3,(#22055,#22056,#22057,#22058,#22059,
#22060,#22061,#22062,#22063,#22064,#22065,#22066,#22067,#22068,#22069,#22070,
#22071,#22072,#22073,#22074,#22075,#22076,#22077,#22078,#22079,#22080,#22081,
#22082,#22083,#22084,#22085,#22086,#22087,#22088,#22089,#22090),
 .UNSPECIFIED.,.F.,.F.,(4,2,2,2,2,2,2,2,2,2,2,2,2,2,2,2,2,4),(5.97412374917029,
6.02336400909286,6.10006341984595,6.17388859912431,6.25076071690477,6.32648861382979,
6.39995163612972,6.47684257851413,6.55172701297119,6.62625691295634,6.70318696737316,
6.77721590255347,6.854278498152,6.93021529134235,7.00361377047219,7.08048358100381,
7.15557375604146,7.19320368173748),.UNSPECIFIED.);
#948=B_SPLINE_CURVE_WITH_KNOTS('',3,(#22091,#22092,#22093,#22094,#22095,
#22096,#22097,#22098,#22099,#22100,#22101,#22102,#22103,#22104,#22105,#22106,
#22107,#22108,#22109,#22110,#22111,#22112,#22113,#22114,#22115,#22116,#22117,
#22118,#22119,#22120,#22121,#22122,#22123,#22124,#22125,#22126),
 .UNSPECIFIED.,.F.,.F.,(4,2,2,2,2,2,2,2,2,2,2,2,2,2,2,2,2,4),(1.6194726882503,
1.68905849303729,1.76541032665973,1.84129252631949,1.91567338868131,1.99300012566542,
2.06693615648198,2.14217646085893,2.21905740368734,2.29248463242846,2.36857454962031,
2.44518201191493,2.51933977125269,2.59641439483466,2.67070416400376,2.74571771802852,
2.82260704900321,2.83860278179673),.UNSPECIFIED.);
#949=B_SPLINE_CURVE_WITH_KNOTS('',3,(#22131,#22132,#22133,#22134,#22135,
#22136,#22137,#22138,#22139,#22140,#22141,#22142,#22143,#22144,#22145,#22146,
#22147,#22148,#22149,#22150,#22151,#22152,#22153,#22154,#22155,#22156,#22157,
#22158,#22159,#22160,#22161,#22162,#22163,#22164,#22165,#22166),
 .UNSPECIFIED.,.F.,.F.,(4,2,2,2,2,2,2,2,2,2,2,2,2,2,2,2,2,4),(4.75497373083379,
4.81676779440289,4.89291059093653,4.96634139896639,5.04320276424534,5.11849451623879,
5.19232799861128,5.26971286680881,5.34414356991651,5.41981447496161,5.49622630208646,
5.569819705332,5.6467031993209,5.72225738250597,5.79589351191985,5.87356474206349,
5.94824936087176,5.97412374917029),.UNSPECIFIED.);
#950=B_SPLINE_CURVE_WITH_KNOTS('',3,(#22167,#22168,#22169,#22170,#22171,
#22172,#22173,#22174,#22175,#22176,#22177,#22178,#22179,#22180,#22181,#22182,
#22183,#22184,#22185,#22186,#22187,#22188,#22189,#22190,#22191,#22192,#22193,
#22194,#22195,#22196,#22197,#22198,#22199,#22200,#22201,#22202),
 .UNSPECIFIED.,.F.,.F.,(4,2,2,2,2,2,2,2,2,2,2,2,2,2,2,2,2,4),(2.83860278179673,
2.89603171119237,2.97189045168826,3.04930918599773,3.12327689819132,3.2001363825891,
3.27487293038277,3.34969704764319,3.42661621894219,3.50014825261352,3.57581534615027,
3.65270673276762,3.72647589461863,3.80311052589585,3.87849224559284,3.95312400477735,
4.03073091488501,4.05823822884819),.UNSPECIFIED.);
#951=B_SPLINE_CURVE_WITH_KNOTS('',3,(#22207,#22208,#22209,#22210,#22211,
#22212,#22213,#22214,#22215,#22216,#22217,#22218,#22219,#22220,#22221,#22222,
#22223,#22224,#22225,#22226,#22227,#22228,#22229,#22230,#22231,#22232,#22233,
#22234,#22235,#22236,#22237,#22238,#22239,#22240,#22241,#22242),
 .UNSPECIFIED.,.F.,.F.,(4,2,2,2,2,2,2,2,2,2,2,2,2,2,2,2,2,4),(3.53614671007836,
3.60978705097627,3.68629180592578,3.76172365013153,3.83623446884695,3.9110890194842,
3.98566617436521,4.06256304463833,4.13656203705491,4.21371517670204,4.28961685991457,
4.36300950127383,4.43987265649615,4.51492830686231,4.58908233355429,4.66620599354184,
4.74040545874708,4.75497373083379),.UNSPECIFIED.);
#952=B_SPLINE_CURVE_WITH_KNOTS('',3,(#22243,#22244,#22245,#22246,#22247,
#22248,#22249,#22250,#22251,#22252,#22253,#22254,#22255,#22256,#22257,#22258,
#22259,#22260,#22261,#22262,#22263,#22264,#22265,#22266,#22267,#22268,#22269,
#22270,#22271,#22272,#22273,#22274,#22275,#22276,#22277,#22278),
 .UNSPECIFIED.,.F.,.F.,(4,2,2,2,2,2,2,2,2,2,2,2,2,2,2,2,2,4),(4.05823822884819,
4.1044868013451,4.17998485839536,4.25691220078312,4.33047707477126,4.40683052560212,
4.4802904286941,4.5572202253281,4.63229702577646,4.70658607651159,4.78372774428882,
4.85794809876263,4.93451770402981,5.01067544858162,5.08415039202188,5.16107410991884,
5.23638120055169,5.27807161868402),.UNSPECIFIED.);
#953=B_SPLINE_CURVE_WITH_KNOTS('',3,(#22283,#22284,#22285,#22286,#22287,
#22288,#22289,#22290,#22291,#22292,#22293,#22294,#22295,#22296,#22297,#22298,
#22299,#22300,#22301,#22302,#22303,#22304,#22305,#22306,#22307,#22308,#22309,
#22310,#22311,#22312,#22313,#22314,#22315,#22316,#22317,#22318,#22319,#22320),
 .UNSPECIFIED.,.F.,.F.,(4,2,2,2,2,2,2,2,2,2,2,2,2,2,2,2,2,2,4),(2.31659118770463,
2.32826973319563,2.40239574111168,2.47943317469931,2.55383013302671,2.62881186696204,
2.7057205160543,2.77917425544425,2.85500063904291,2.93262228783198,3.00656660516777,
3.08339822551228,3.15825784805468,3.23305942009734,3.31000255015569,3.38358499198161,
3.45922951950883,3.5361146660716,3.53614671007836),.UNSPECIFIED.);
#954=B_SPLINE_CURVE_WITH_KNOTS('',3,(#22321,#22322,#22323,#22324,#22325,
#22326,#22327,#22328,#22329,#22330,#22331,#22332,#22333,#22334,#22335,#22336,
#22337,#22338,#22339,#22340,#22341,#22342,#22343,#22344,#22345,#22346,#22347,
#22348,#22349,#22350,#22351,#22352,#22353,#22354,#22355,#22356),
 .UNSPECIFIED.,.F.,.F.,(4,2,2,2,2,2,2,2,2,2,2,2,2,2,2,2,2,4),(5.27807161868402,
5.31032777693036,5.38772503012124,5.46217159019827,5.53802704136127,5.6144494833653,
5.68806368756168,5.76500481703162,5.84057024401696,5.91429504129166,5.99197483370221,
6.06667182342315,6.14194300109424,6.21865040739694,6.29248620031064,6.36940465578137,
6.4451419747725,6.49826355609911),.UNSPECIFIED.);
#955=B_SPLINE_CURVE_WITH_KNOTS('',3,(#22362,#22363,#22364,#22365,#22366,
#22367,#22368,#22369,#22370,#22371,#22372,#22373,#22374,#22375,#22376,#22377,
#22378,#22379,#22380,#22381,#22382,#22383,#22384,#22385,#22386,#22387,#22388,
#22389,#22390,#22391,#22392,#22393,#22394,#22395),.UNSPECIFIED.,.F.,.F.,
(4,2,2,2,2,2,2,2,2,2,2,2,2,2,2,2,4),(7.71789566086823,7.72653108491538,
7.80344420250335,7.8787707829751,7.9526720028552,8.03009150427855,8.10455689214304,
8.18032097369781,8.25676646530167,8.33039555105596,8.40732916035414,8.48291689218689,
8.55661219462614,8.63431688302293,8.70903510957268,8.76144136318372,8.81578353266249),
 .UNSPECIFIED.);
#956=B_SPLINE_CURVE_WITH_KNOTS('',3,(#22398,#22399,#22400,#22401,#22402,
#22403,#22404,#22405,#22406,#22407,#22408,#22409,#22410,#22411,#22412,#22413,
#22414,#22415,#22416,#22417,#22418,#22419,#22420,#22421,#22422,#22423,#22424,
#22425,#22426,#22427,#22428,#22429),.UNSPECIFIED.,.F.,.F.,(4,2,2,2,2,2,
2,2,2,2,2,2,2,2,2,4),(3.04265128429249E-8,0.0696297941848276,0.137949529099356,
0.213754729172342,0.291233561599973,0.365153025689176,0.441960629532743,
0.516719666380159,0.591495500873206,0.668388103886912,0.741907722474293,
0.817526091622124,0.89438880062244,0.968111365669073,1.04469595401189,1.09710239300462),
 .UNSPECIFIED.);
#957=B_SPLINE_CURVE_WITH_KNOTS('',3,(#22436,#22437,#22438,#22439,#22440,
#22441,#22442,#22443,#22444,#22445,#22446,#22447,#22448,#22449),
 .UNSPECIFIED.,.F.,.F.,(4,2,2,2,2,2,4),(9.99999998850988E-7,0.0516169518680174,
0.104845041291632,0.181709819458214,0.255107103717481,0.330970348449006,
0.40012180130331),.UNSPECIFIED.);
#958=B_SPLINE_CURVE_WITH_KNOTS('',3,(#22455,#22456,#22457,#22458,#22459,
#22460,#22461,#22462,#22463,#22464,#22465,#22466,#22467,#22468,#22469,#22470),
 .UNSPECIFIED.,.F.,.F.,(4,2,2,2,2,2,2,4),(7.19320368172767,7.22969104327013,
7.30685234317884,7.38108572363072,7.4573667927007,7.53354842516364,7.60230579028133,
7.67143903153375),.UNSPECIFIED.);
#959=B_SPLINE_CURVE_WITH_KNOTS('',3,(#22472,#22473,#22474,#22475,#22476,
#22477,#22478,#22479,#22480,#22481,#22482,#22483,#22484,#22485,#22486,#22487,
#22488,#22489,#22490,#22491,#22492,#22493,#22494,#22495,#22496,#22497,#22498,
#22499,#22500,#22501,#22502,#22503,#22504,#22505,#22506,#22507,#22508,#22509),
 .UNSPECIFIED.,.F.,.F.,(4,2,2,2,2,2,2,2,2,2,2,2,2,2,2,2,2,2,4),(0.40012180130331,
0.408263585102685,0.48223140566233,0.559093024369444,0.633749160630985,
0.7085728423697,0.785465068742682,0.858957556763468,0.934624119514201,1.0114910968397,
1.08525873800664,1.16189369275507,1.23717718819415,1.31180620569013,1.38941296914438,
1.46311419611182,1.53861020423359,1.61550600313119,1.61947369254408),
 .UNSPECIFIED.);
#960=B_SPLINE_CURVE_WITH_KNOTS('',3,(#22514,#22515,#22516,#22517,#22518,
#22519,#22520,#22521,#22522,#22523,#22524,#22525,#22526,#22527,#22528,#22529,
#22530,#22531,#22532,#22533,#22534,#22535,#22536,#22537,#22538,#22539,#22540,
#22541,#22542,#22543,#22544,#22545,#22546,#22547,#22548,#22549),
 .UNSPECIFIED.,.F.,.F.,(4,2,2,2,2,2,2,2,2,2,2,2,2,2,2,2,2,4),(5.974123749161,
6.02336400908333,6.10006341983629,6.17388859911447,6.2507607168948,6.32648861381977,
6.39995163611967,6.47684257850402,6.55172701296104,6.62625691294614,6.70318696736296,
6.77721590254322,6.85427849814168,6.93021529133211,7.003613770462,7.08048358099369,
7.15557375603143,7.19320368172767),.UNSPECIFIED.);
#961=B_SPLINE_CURVE_WITH_KNOTS('',3,(#22550,#22551,#22552,#22553,#22554,
#22555,#22556,#22557,#22558,#22559,#22560,#22561,#22562,#22563,#22564,#22565,
#22566,#22567,#22568,#22569,#22570,#22571,#22572,#22573,#22574,#22575,#22576,
#22577,#22578,#22579,#22580,#22581,#22582,#22583,#22584,#22585),
 .UNSPECIFIED.,.F.,.F.,(4,2,2,2,2,2,2,2,2,2,2,2,2,2,2,2,2,4),(1.61947369254408,
1.68905949729837,1.76541133090778,1.84129353055796,1.91567439290728,1.99300112987828,
2.06693716068424,2.14217746504849,2.21905840786482,2.29248563659418,2.36857555377319,
2.44518301605857,2.51934077538404,2.59641539895315,2.67070516811205,2.74571872212431,
2.82260805308708,2.83860378589876),.UNSPECIFIED.);
#962=B_SPLINE_CURVE_WITH_KNOTS('',3,(#22590,#22591,#22592,#22593,#22594,
#22595,#22596,#22597,#22598,#22599,#22600,#22601,#22602,#22603,#22604,#22605,
#22606,#22607,#22608,#22609,#22610,#22611,#22612,#22613,#22614,#22615,#22616,
#22617,#22618,#22619,#22620,#22621,#22622,#22623,#22624,#22625),
 .UNSPECIFIED.,.F.,.F.,(4,2,2,2,2,2,2,2,2,2,2,2,2,2,2,2,2,4),(4.75497373082735,
4.81676779439626,4.89291059092976,4.96634139895943,5.04320276423819,5.11849451623147,
5.19232799860378,5.2697128668011,5.34414356990862,5.41981447495354,5.49622630207823,
5.56981970532358,5.6467031993123,5.72225738249718,5.79589351191087,5.87356474205431,
5.94824936086241,5.974123749161),.UNSPECIFIED.);
#963=B_SPLINE_CURVE_WITH_KNOTS('',3,(#22626,#22627,#22628,#22629,#22630,
#22631,#22632,#22633,#22634,#22635,#22636,#22637,#22638,#22639,#22640,#22641,
#22642,#22643,#22644,#22645,#22646,#22647,#22648,#22649,#22650,#22651,#22652,
#22653,#22654,#22655,#22656,#22657,#22658,#22659,#22660,#22661),
 .UNSPECIFIED.,.F.,.F.,(4,2,2,2,2,2,2,2,2,2,2,2,2,2,2,2,2,4),(2.83860378589876,
2.89603271526497,2.97189145574824,3.04931019004864,3.12327790223017,3.20013738661533,
3.27487393439905,3.34969805164721,3.42661722293439,3.50014925659483,3.57581635011919,
3.65270773672471,3.72647689856381,3.80311152982859,3.87849324951609,3.95312500868852,
4.03073191878357,4.05823923276311),.UNSPECIFIED.);
#964=B_SPLINE_CURVE_WITH_KNOTS('',3,(#22666,#22667,#22668,#22669,#22670,
#22671,#22672,#22673,#22674,#22675,#22676,#22677,#22678,#22679,#22680,#22681,
#22682,#22683,#22684,#22685,#22686,#22687,#22688,#22689,#22690,#22691,#22692,
#22693,#22694,#22695,#22696,#22697,#22698,#22699,#22700,#22701),
 .UNSPECIFIED.,.F.,.F.,(4,2,2,2,2,2,2,2,2,2,2,2,2,2,2,2,2,4),(3.53614671007441,
3.6097870509723,3.68629180592174,3.76172365012743,3.83623446884277,3.91108901947988,
3.98566617436073,4.06256304463361,4.13656203704999,4.21371517669692,4.28961685990926,
4.36300950126833,4.43987265649047,4.51492830685644,4.58908233354824,4.66620599353558,
4.74040545874063,4.75497373082735),.UNSPECIFIED.);
#965=B_SPLINE_CURVE_WITH_KNOTS('',3,(#22702,#22703,#22704,#22705,#22706,
#22707,#22708,#22709,#22710,#22711,#22712,#22713,#22714,#22715,#22716,#22717,
#22718,#22719,#22720,#22721,#22722,#22723,#22724,#22725,#22726,#22727,#22728,
#22729,#22730,#22731,#22732,#22733,#22734,#22735,#22736,#22737),
 .UNSPECIFIED.,.F.,.F.,(4,2,2,2,2,2,2,2,2,2,2,2,2,2,2,2,2,4),(4.05823923276311,
4.10448780523323,4.17998586227126,4.25691320464737,4.33047807862384,4.40683152944232,
4.48029143252306,4.5572212291454,4.63229802958326,4.70658708030576,4.78372874807228,
4.8579491025357,4.93451870778849,5.01067645232983,5.08415139575935,5.1610751136448,
5.23638220426729,5.27807262241528),.UNSPECIFIED.);
#966=B_SPLINE_CURVE_WITH_KNOTS('',3,(#22742,#22743,#22744,#22745,#22746,
#22747,#22748,#22749,#22750,#22751,#22752,#22753,#22754,#22755,#22756,#22757,
#22758,#22759,#22760,#22761,#22762,#22763,#22764,#22765,#22766,#22767,#22768,
#22769,#22770,#22771,#22772,#22773,#22774,#22775,#22776,#22777,#22778,#22779),
 .UNSPECIFIED.,.F.,.F.,(4,2,2,2,2,2,2,2,2,2,2,2,2,2,2,2,2,2,4),(2.31659118770178,
2.32826973319281,2.40239574110879,2.47943317469632,2.55383013302362,2.62881186695886,
2.70572051605103,2.77917425544088,2.85500063903944,2.93262228782847,3.00656660516422,
3.08339822550865,3.15825784805098,3.23305942009357,3.31000255015187,3.38358499197773,
3.45922951950491,3.53611466606766,3.53614671007441),.UNSPECIFIED.);
#967=B_SPLINE_CURVE_WITH_KNOTS('',3,(#22780,#22781,#22782,#22783,#22784,
#22785,#22786,#22787,#22788,#22789,#22790,#22791,#22792,#22793,#22794,#22795,
#22796,#22797,#22798,#22799,#22800,#22801,#22802,#22803,#22804,#22805,#22806,
#22807,#22808,#22809,#22810,#22811,#22812,#22813,#22814,#22815),
 .UNSPECIFIED.,.F.,.F.,(4,2,2,2,2,2,2,2,2,2,2,2,2,2,2,2,2,4),(5.27807262241528,
5.31032878063387,5.38772603381421,5.46217259388101,5.53802804503023,5.61445048702391,
5.68806469121006,5.76500582066864,5.84057124764373,5.9142960449069,5.991975837307,
6.06667282701779,6.14194400467577,6.21865141096818,6.29248720387191,6.36940565933153,
6.44514297831244,6.49826455965138),.UNSPECIFIED.);
#968=B_SPLINE_CURVE_WITH_KNOTS('',3,(#22821,#22822,#22823,#22824,#22825,
#22826,#22827,#22828,#22829,#22830,#22831,#22832,#22833,#22834,#22835,#22836,
#22837,#22838,#22839,#22840,#22841,#22842,#22843,#22844,#22845,#22846,#22847,
#22848,#22849,#22850,#22851,#22852,#22853,#22854),.UNSPECIFIED.,.F.,.F.,
(4,2,2,2,2,2,2,2,2,2,2,2,2,2,2,2,4),(7.71789666424489,7.72653208826837,
7.80344520584536,7.87877178630723,7.95267300617573,8.030092507589,8.10455789544369,
8.18032197698524,8.25676746857915,8.33039655432369,8.40733016361098,8.48291789543391,
8.55661319786207,8.63431788624882,8.70903611278883,8.76144236640241,8.8157845358832),
 .UNSPECIFIED.);
#969=B_SPLINE_CURVE_WITH_KNOTS('',3,(#22857,#22858,#22859,#22860,#22861,
#22862,#22863,#22864,#22865,#22866,#22867,#22868,#22869,#22870,#22871,#22872,
#22873,#22874,#22875,#22876,#22877,#22878,#22879,#22880,#22881,#22882,#22883,
#22884,#22885,#22886,#22887,#22888),.UNSPECIFIED.,.F.,.F.,(4,2,2,2,2,2,
2,2,2,2,2,2,2,2,2,4),(3.04265172991663E-8,0.0696297941849219,0.137949529099536,
0.21375472917256,0.291233561600128,0.365153025689274,0.441960629532807,
0.516719666380197,0.591495500873207,0.668388103886848,0.74190772247416,
0.817526091621932,0.894388800622119,0.968111365668598,1.04469595401127,
1.09710239300385),.UNSPECIFIED.);
#970=B_SPLINE_CURVE_WITH_KNOTS('',3,(#22895,#22896,#22897,#22898,#22899,
#22900,#22901,#22902,#22903,#22904,#22905,#22906,#22907,#22908),
 .UNSPECIFIED.,.F.,.F.,(4,2,2,2,2,2,4),(0.,0.0516156037392325,0.104843298833226,
0.181708269115714,0.255105736824021,0.330969171170157,0.400120796811339),
 .UNSPECIFIED.);
#971=B_SPLINE_CURVE_WITH_KNOTS('',3,(#22914,#22915,#22916,#22917,#22918,
#22919,#22920,#22921,#22922,#22923,#22924,#22925,#22926,#22927,#22928,#22929),
 .UNSPECIFIED.,.F.,.F.,(4,2,2,2,2,2,2,4),(7.19320368173771,7.22969111960813,
7.30685258093042,7.381086116671,7.45736734531324,7.53354913714033,7.60230617175925,
7.67143902533004),.UNSPECIFIED.);
#972=B_SPLINE_CURVE_WITH_KNOTS('',3,(#22931,#22932,#22933,#22934,#22935,
#22936,#22937,#22938,#22939,#22940,#22941,#22942,#22943,#22944,#22945,#22946,
#22947,#22948,#22949,#22950,#22951,#22952,#22953,#22954,#22955,#22956,#22957,
#22958,#22959,#22960,#22961,#22962,#22963,#22964,#22965,#22966,#22967,#22968),
 .UNSPECIFIED.,.F.,.F.,(4,2,2,2,2,2,2,2,2,2,2,2,2,2,2,2,2,2,4),(0.400120796811339,
0.408262580655585,0.482230401228364,0.559092019949293,0.633748156218688,
0.708571837970628,0.785464064355422,0.858956552386623,0.93462311515074,
1.01149009248822,1.08525773366815,1.16189268843024,1.23717618387609,1.3118052013851,
1.3894119648531,1.46311319182998,1.53860919996502,1.61550499887409,1.6194726882389),
 .UNSPECIFIED.);
#973=B_SPLINE_CURVE_WITH_KNOTS('',3,(#22973,#22974,#22975,#22976,#22977,
#22978,#22979,#22980,#22981,#22982,#22983,#22984,#22985,#22986,#22987,#22988,
#22989,#22990,#22991,#22992,#22993,#22994,#22995,#22996,#22997,#22998,#22999,
#23000,#23001,#23002,#23003,#23004,#23005,#23006,#23007,#23008),
 .UNSPECIFIED.,.F.,.F.,(4,2,2,2,2,2,2,2,2,2,2,2,2,2,2,2,2,4),(5.97412374917094,
6.02336400909344,6.1000634198465,6.17388859912484,6.25076071690528,6.32648861383027,
6.39995163613019,6.47684257851458,6.55172701297161,6.62625691295673,6.70318696737352,
6.77721590255381,6.8542784981523,6.93021529134263,7.00361377047243,7.08048358100402,
7.15557375604164,7.19320368173771),.UNSPECIFIED.);
#974=B_SPLINE_CURVE_WITH_KNOTS('',3,(#23009,#23010,#23011,#23012,#23013,
#23014,#23015,#23016,#23017,#23018,#23019,#23020,#23021,#23022,#23023,#23024,
#23025,#23026,#23027,#23028,#23029,#23030,#23031,#23032,#23033,#23034,#23035,
#23036,#23037,#23038,#23039,#23040,#23041,#23042,#23043,#23044),
 .UNSPECIFIED.,.F.,.F.,(4,2,2,2,2,2,2,2,2,2,2,2,2,2,2,2,2,4),(1.6194726882389,
1.68905849305358,1.76541032667645,1.84129252633228,1.91567338869436,1.99300012567884,
2.06693615649319,2.14217646087043,2.21905740369798,2.29248463243857,2.36857454963071,
2.4451820119209,2.5193397712588,2.596414394841,2.67070416400741,2.7457177180323,
2.82260704900607,2.83860278177238),.UNSPECIFIED.);
#975=B_SPLINE_CURVE_WITH_KNOTS('',3,(#23049,#23050,#23051,#23052,#23053,
#23054,#23055,#23056,#23057,#23058,#23059,#23060,#23061,#23062,#23063,#23064,
#23065,#23066,#23067,#23068,#23069,#23070,#23071,#23072,#23073,#23074,#23075,
#23076,#23077,#23078,#23079,#23080,#23081,#23082,#23083,#23084),
 .UNSPECIFIED.,.F.,.F.,(4,2,2,2,2,2,2,2,2,2,2,2,2,2,2,2,2,4),(4.75497373083482,
4.81676779440388,4.89291059093751,4.96634139896734,5.04320276424626,5.11849451623969,
5.19232799861215,5.26971286680966,5.34414356991732,5.41981447496239,5.4962263020872,
5.56981970533272,5.6467031993216,5.72225738250664,5.7958935119205,5.87356474206412,
5.94824936087237,5.97412374917094),.UNSPECIFIED.);
#976=B_SPLINE_CURVE_WITH_KNOTS('',3,(#23085,#23086,#23087,#23088,#23089,
#23090,#23091,#23092,#23093,#23094,#23095,#23096,#23097,#23098,#23099,#23100,
#23101,#23102,#23103,#23104,#23105,#23106,#23107,#23108,#23109,#23110,#23111,
#23112,#23113,#23114,#23115,#23116,#23117,#23118,#23119,#23120),
 .UNSPECIFIED.,.F.,.F.,(4,2,2,2,2,2,2,2,2,2,2,2,2,2,2,2,2,4),(2.83860278177238,
2.89603171119416,2.9718904516902,3.04930918599495,3.12327689818853,3.20013638258635,
3.27487293037699,3.34969704763737,3.42661621893534,3.50014825260515,3.57581534614186,
3.65270673275826,3.72647589460919,3.80311052588641,3.87849224557971,3.95312400476411,
4.03073091487175,4.05823822880769),.UNSPECIFIED.);
#977=B_SPLINE_CURVE_WITH_KNOTS('',3,(#23125,#23126,#23127,#23128,#23129,
#23130,#23131,#23132,#23133,#23134,#23135,#23136,#23137,#23138,#23139,#23140,
#23141,#23142,#23143,#23144,#23145,#23146,#23147,#23148,#23149,#23150,#23151,
#23152,#23153,#23154,#23155,#23156,#23157,#23158,#23159,#23160),
 .UNSPECIFIED.,.F.,.F.,(4,2,2,2,2,2,2,2,2,2,2,2,2,2,2,2,2,4),(3.53614671007962,
3.60978705097756,3.6862918059271,3.76172365013287,3.83623446884831,3.91108901948555,
3.98566617436653,4.06256304463961,4.13656203705616,4.21371517670325,4.28961685991574,
4.36300950127498,4.43987265649728,4.5149283068634,4.58908233355535,4.66620599354287,
4.74040545874809,4.75497373083482),.UNSPECIFIED.);
#978=B_SPLINE_CURVE_WITH_KNOTS('',3,(#23161,#23162,#23163,#23164,#23165,
#23166,#23167,#23168,#23169,#23170,#23171,#23172,#23173,#23174,#23175,#23176,
#23177,#23178,#23179,#23180,#23181,#23182,#23183,#23184,#23185,#23186,#23187,
#23188,#23189,#23190,#23191,#23192,#23193,#23194,#23195,#23196),
 .UNSPECIFIED.,.F.,.F.,(4,2,2,2,2,2,2,2,2,2,2,2,2,2,2,2,2,4),(4.05823822880769,
4.10448680132977,4.17998485837995,4.25691220076652,4.33047707475418,4.40683052558499,
4.48029042867599,4.55722022530881,4.6322970257549,4.70658607649072,4.78372774426551,
4.85794809873707,4.93451770400669,5.01067544855601,5.08415039199467,5.16107410989033,
5.23638120052075,5.2780716186238),.UNSPECIFIED.);
#979=B_SPLINE_CURVE_WITH_KNOTS('',3,(#23201,#23202,#23203,#23204,#23205,
#23206,#23207,#23208,#23209,#23210,#23211,#23212,#23213,#23214,#23215,#23216,
#23217,#23218,#23219,#23220,#23221,#23222,#23223,#23224,#23225,#23226,#23227,
#23228,#23229,#23230,#23231,#23232,#23233,#23234,#23235,#23236,#23237,#23238),
 .UNSPECIFIED.,.F.,.F.,(4,2,2,2,2,2,2,2,2,2,2,2,2,2,2,2,2,2,4),(2.31659118770536,
2.32826973319637,2.40239574111246,2.47943317470013,2.55383013302756,2.62881186696292,
2.70572051605522,2.77917425544518,2.85500063904386,2.93262228783295,3.00656660516877,
3.08339822551331,3.15825784805574,3.23305942009844,3.31000255015683,3.38358499198278,
3.45922951951005,3.53611466607286,3.53614671007962),.UNSPECIFIED.);
#980=B_SPLINE_CURVE_WITH_KNOTS('',3,(#23239,#23240,#23241,#23242,#23243,
#23244,#23245,#23246,#23247,#23248,#23249,#23250,#23251,#23252,#23253,#23254,
#23255,#23256,#23257,#23258,#23259,#23260,#23261,#23262,#23263,#23264,#23265,
#23266,#23267,#23268,#23269,#23270,#23271,#23272,#23273,#23274),
 .UNSPECIFIED.,.F.,.F.,(4,2,2,2,2,2,2,2,2,2,2,2,2,2,2,2,2,4),(5.2780716186238,
5.31032777689959,5.38772503008789,5.46217159016254,5.53802704132747,5.61444948332891,
5.68806368752308,5.76500481699161,5.84057024397439,5.91429504124862,5.99197483365645,
6.06667182337488,6.14194300104719,6.21865040734719,6.29248620025837,6.36940465572739,
6.44514197471589,6.49826355601516),.UNSPECIFIED.);
#981=B_SPLINE_CURVE_WITH_KNOTS('',3,(#23280,#23281,#23282,#23283,#23284,
#23285,#23286,#23287,#23288,#23289,#23290,#23291,#23292,#23293,#23294,#23295,
#23296,#23297,#23298,#23299,#23300,#23301,#23302,#23303,#23304,#23305,#23306,
#23307,#23308,#23309,#23310,#23311,#23312,#23313),.UNSPECIFIED.,.F.,.F.,
(4,2,2,2,2,2,2,2,2,2,2,2,2,2,2,2,4),(7.71789566075662,7.72653108483295,
7.803444202419,7.8787707828877,7.95267200276729,8.03009150418741,8.10455689204888,
8.18032097360487,8.25676646520549,8.33039555095692,8.40732916025302,8.48291689208259,
8.5566121945207,8.63431688291413,8.70903510946076,8.76144136305708,8.81578353252107),
 .UNSPECIFIED.);
#982=B_SPLINE_CURVE_WITH_KNOTS('',3,(#23316,#23317,#23318,#23319,#23320,
#23321,#23322,#23323,#23324,#23325,#23326,#23327,#23328,#23329,#23330,#23331,
#23332,#23333,#23334,#23335,#23336,#23337,#23338,#23339,#23340,#23341,#23342,
#23343,#23344,#23345,#23346,#23347),.UNSPECIFIED.,.F.,.F.,(4,2,2,2,2,2,
2,2,2,2,2,2,2,2,2,4),(3.04265160429364E-8,0.069629794184829,0.137949529099366,
0.213754729172367,0.291233561600009,0.365153025689221,0.441960629532807,
0.51671966638024,0.591495500873295,0.668388103887014,0.741907722474407,
0.817526091622261,0.8943888006226,0.96811136566926,1.0446959540121,1.09710239300487),
 .UNSPECIFIED.);
#983=B_SPLINE_CURVE_WITH_KNOTS('',3,(#23349,#23350,#23351,#23352,#23353,
#23354,#23355,#23356,#23357,#23358,#23359,#23360,#23361,#23362,#23363,#23364,
#23365,#23366,#23367,#23368,#23369,#23370,#23371,#23372,#23373,#23374,#23375,
#23376,#23377,#23378,#23379,#23380,#23381,#23382,#23383,#23384),
 .UNSPECIFIED.,.F.,.F.,(4,2,2,2,2,2,2,2,2,2,2,2,2,2,2,2,2,4),(1.09710239300487,
1.12011517711278,1.19470090123193,1.27225761508382,1.34601419186938,1.42146508618074,
1.49836987210414,1.57189808509923,1.64820345609062,1.72425249768454,1.7985949229751,
1.87587698848718,1.94989642538678,2.02509727325677,2.10199260325516,2.17542254085659,
2.25147199531572,2.31659118770536),.UNSPECIFIED.);
#984=B_SPLINE_CURVE_WITH_KNOTS('',3,(#23385,#23386,#23387,#23388,#23389,
#23390,#23391,#23392,#23393,#23394,#23395,#23396,#23397,#23398,#23399,#23400,
#23401,#23402,#23403,#23404,#23405,#23406,#23407,#23408,#23409,#23410,#23411,
#23412,#23413,#23414,#23415,#23416,#23417,#23418,#23419,#23420),
 .UNSPECIFIED.,.F.,.F.,(4,2,2,2,2,2,2,2,2,2,2,2,2,2,2,2,2,4),(6.49826355601516,
6.51867068512192,6.59561216979648,6.67050587384408,6.74516442447251,6.82210014899345,
6.89613760570075,6.97339767877051,7.04933639285787,7.12278074933092,7.1996971518762,
7.27478951608072,7.34901910305193,7.42617920383861,7.50041497326189,7.57687878673137,
7.65305660455958,7.71789566075662),.UNSPECIFIED.);
#985=B_SPLINE_CURVE_WITH_KNOTS('',3,(#23422,#23423,#23424,#23425,#23426,
#23427,#23428,#23429,#23430,#23431,#23432,#23433,#23434,#23435,#23436,#23437,
#23438,#23439,#23440,#23441,#23442,#23443,#23444,#23445,#23446,#23447,#23448,
#23449,#23450,#23451,#23452,#23453,#23454,#23455,#23456,#23457),
 .UNSPECIFIED.,.F.,.F.,(4,2,2,2,2,2,2,2,2,2,2,2,2,2,2,2,2,4),(1.09710239300385,
1.12011517711179,1.19470090123079,1.27225761508249,1.34601419186788,1.42146508617906,
1.49836987210228,1.5718980850972,1.64820345608845,1.72425249768224,1.79859492297267,
1.87587698848456,1.94989642538399,2.02509727325381,2.10199260325204,2.1754225408533,
2.25147199531227,2.31659118770178),.UNSPECIFIED.);
#986=B_SPLINE_CURVE_WITH_KNOTS('',3,(#23458,#23459,#23460,#23461,#23462,
#23463,#23464,#23465,#23466,#23467,#23468,#23469,#23470,#23471,#23472,#23473,
#23474,#23475,#23476,#23477,#23478,#23479,#23480,#23481,#23482,#23483,#23484,
#23485,#23486,#23487,#23488,#23489,#23490,#23491,#23492,#23493),
 .UNSPECIFIED.,.F.,.F.,(4,2,2,2,2,2,2,2,2,2,2,2,2,2,2,2,2,4),(6.49826455965138,
6.5186716887085,6.5956131733735,6.67050687741361,6.74516542802906,6.8221011525425,
6.89613860924244,6.97339868229584,7.04933739637596,7.12278175283993,7.19969815537587,
7.27479051957324,7.34902010653224,7.42618020731174,7.50041597672795,7.57687979018179,
7.65305760800301,7.71789666424489),.UNSPECIFIED.);
#987=B_SPLINE_CURVE_WITH_KNOTS('',3,(#23495,#23496,#23497,#23498,#23499,
#23500,#23501,#23502,#23503,#23504,#23505,#23506,#23507,#23508,#23509,#23510,
#23511,#23512,#23513,#23514,#23515,#23516,#23517,#23518,#23519,#23520,#23521,
#23522,#23523,#23524,#23525,#23526,#23527,#23528,#23529,#23530),
 .UNSPECIFIED.,.F.,.F.,(4,2,2,2,2,2,2,2,2,2,2,2,2,2,2,2,2,4),(1.09710239300462,
1.12011517711253,1.19470090123165,1.27225761508352,1.34601419186906,1.42146508618039,
1.49836987210376,1.57189808509882,1.64820345609019,1.72425249768409,1.79859492297463,
1.87587698848668,1.94989642538625,2.02509727325621,2.10199260325456,2.17542254085595,
2.25147199531503,2.31659118770463),.UNSPECIFIED.);
#988=B_SPLINE_CURVE_WITH_KNOTS('',3,(#23531,#23532,#23533,#23534,#23535,
#23536,#23537,#23538,#23539,#23540,#23541,#23542,#23543,#23544,#23545,#23546,
#23547,#23548,#23549,#23550,#23551,#23552,#23553,#23554,#23555,#23556,#23557,
#23558,#23559,#23560,#23561,#23562,#23563,#23564,#23565,#23566),
 .UNSPECIFIED.,.F.,.F.,(4,2,2,2,2,2,2,2,2,2,2,2,2,2,2,2,2,4),(6.49826355609911,
6.5186706851796,6.59561216985577,6.67050587390597,6.74516442453385,6.82210014905756,
6.89613760576745,6.973397678835,7.04933639292522,7.12278074939984,7.19969715194686,
7.27478951615419,7.34901910312529,7.42617920391494,7.500414973341,7.57687878680861,
7.65305660463983,7.71789566086823),.UNSPECIFIED.);
#989=B_SPLINE_CURVE_WITH_KNOTS('',3,(#23568,#23569,#23570,#23571,#23572,
#23573,#23574,#23575,#23576,#23577,#23578,#23579,#23580,#23581,#23582,#23583,
#23584,#23585,#23586,#23587,#23588,#23589,#23590,#23591,#23592,#23593,#23594,
#23595,#23596,#23597,#23598,#23599,#23600,#23601,#23602,#23603),
 .UNSPECIFIED.,.F.,.F.,(4,2,2,2,2,2,2,2,2,2,2,2,2,2,2,2,2,4),(1.09710239300357,
1.1201151771115,1.19470090123049,1.27225761508217,1.34601419186753,1.42146508617868,
1.49836987210188,1.57189808509679,1.64820345608801,1.72425249768178,1.79859492297218,
1.87587698848406,1.94989642538346,2.02509727325326,2.10199260325146,2.17542254085271,
2.25147199531166,2.31659118770115),.UNSPECIFIED.);
#990=B_SPLINE_CURVE_WITH_KNOTS('',3,(#23604,#23605,#23606,#23607,#23608,
#23609,#23610,#23611,#23612,#23613,#23614,#23615,#23616,#23617,#23618,#23619,
#23620,#23621,#23622,#23623,#23624,#23625,#23626,#23627,#23628,#23629,#23630,
#23631,#23632,#23633,#23634,#23635,#23636,#23637,#23638,#23639),
 .UNSPECIFIED.,.F.,.F.,(4,2,2,2,2,2,2,2,2,2,2,2,2,2,2,2,2,4),(6.49826455965138,
6.5186716887085,6.5956131733735,6.67050687741361,6.74516542802906,6.8221011525425,
6.89613860924244,6.97339868229584,7.04933739637596,7.12278175283993,7.19969815537587,
7.27479051957324,7.34902010653224,7.42618020731174,7.50041597672795,7.57687979018179,
7.65305760800301,7.71789666424489),.UNSPECIFIED.);
#991=B_SPLINE_CURVE_WITH_KNOTS('',3,(#23642,#23643,#23644,#23645,#23646,
#23647,#23648,#23649,#23650,#23651,#23652,#23653,#23654,#23655,#23656,#23657,
#23658,#23659,#23660,#23661,#23662,#23663,#23664,#23665,#23666,#23667,#23668,
#23669,#23670,#23671,#23672,#23673,#23674,#23675,#23676,#23677),
 .UNSPECIFIED.,.F.,.F.,(4,2,2,2,2,2,2,2,2,2,2,2,2,2,2,2,2,4),(21.3148424617523,
21.3353161897489,21.4081377842537,21.4844828604283,21.5591605315819,21.6314755220292,
21.7071973308415,21.7810434185569,21.8542546835973,21.9301267130465,22.0031298277028,
22.0786702152169,22.153570144142,22.2258725023802,22.301583175239,22.3756477399792,
22.417649122091,22.4598825016052),.UNSPECIFIED.);
#992=B_SPLINE_CURVE_WITH_KNOTS('',3,(#23680,#23681,#23682,#23683,#23684,
#23685,#23686,#23687,#23688,#23689,#23690,#23691,#23692,#23693,#23694,#23695,
#23696,#23697,#23698,#23699,#23700,#23701,#23702,#23703,#23704,#23705,#23706,
#23707,#23708,#23709,#23710,#23711),.UNSPECIFIED.,.F.,.F.,(4,2,2,2,2,2,
2,2,2,2,2,2,2,2,2,4),(9.9999999597469E-7,0.0410609715951109,0.0810353625720383,
0.153401243599348,0.228317275003317,0.304123825641722,0.377151035158167,
0.453043725999999,0.526430357230195,0.600301304337368,0.676103842764624,
0.748510230606864,0.823212972034187,0.899001954842751,0.971827250111653,
0.994462254792754),.UNSPECIFIED.);
#993=B_SPLINE_CURVE_WITH_KNOTS('',3,(#23714,#23715,#23716,#23717,#23718,
#23719,#23720,#23721,#23722,#23723,#23724,#23725,#23726,#23727,#23728,#23729,
#23730,#23731,#23732,#23733,#23734,#23735,#23736,#23737,#23738,#23739,#23740,
#23741),.UNSPECIFIED.,.F.,.F.,(4,2,2,2,2,2,2,2,2,2,2,2,2,4),(21.6282084253952,
21.6372441032614,21.7129394368562,21.7870523479308,21.8598087122815,21.9359787394778,
22.0092444905551,22.083867163104,22.1590778009158,22.2315231390981,22.3072372394324,
22.3816054833466,22.4274081248573,22.4730897400475),.UNSPECIFIED.);
#994=B_SPLINE_CURVE_WITH_KNOTS('',3,(#23744,#23745,#23746,#23747,#23748,
#23749,#23750,#23751,#23752,#23753,#23754,#23755,#23756,#23757,#23758,#23759,
#23760,#23761,#23762,#23763,#23764,#23765,#23766,#23767),.UNSPECIFIED.,
 .F.,.F.,(4,2,2,2,2,2,2,2,2,2,2,4),(9.9999999828754E-7,0.0409987765676221,
0.0809155863998274,0.15328123806841,0.228192677104899,0.304015356848976,
0.377038791813246,0.452927204977614,0.526322673925784,0.6001898532434,0.675993042874638,
0.693996851653457),.UNSPECIFIED.);
#995=B_SPLINE_CURVE_WITH_KNOTS('',3,(#23770,#23771,#23772,#23773,#23774,
#23775,#23776,#23777,#23778,#23779,#23780,#23781,#23782,#23783,#23784,#23785,
#23786,#23787,#23788,#23789),.UNSPECIFIED.,.F.,.F.,(4,2,2,2,2,2,2,2,2,4),
(21.9110024905134,21.9219460418809,21.9950982805857,22.0701188260611,22.1451953864536,
22.2175618280791,22.2932793240977,22.3675167787528,22.4116383044439,22.4558211302722),
 .UNSPECIFIED.);
#996=B_SPLINE_CURVE_WITH_KNOTS('',3,(#23792,#23793,#23794,#23795,#23796,
#23797,#23798,#23799,#23800,#23801,#23802,#23803,#23804,#23805,#23806,#23807),
 .UNSPECIFIED.,.F.,.F.,(4,2,2,2,2,2,2,4),(1.00000007208917E-6,0.0398646418385672,
0.0787292474270129,0.15109808491172,0.225926380077501,0.302048834068036,
0.375004296118167,0.393548424805639),.UNSPECIFIED.);
#997=B_SPLINE_CURVE_WITH_KNOTS('',3,(#23810,#23811,#23812,#23813,#23814,
#23815,#23816,#23817,#23818,#23819,#23820,#23821),.UNSPECIFIED.,.F.,.F.,
(4,2,2,2,2,4),(22.2034453162522,22.2090431050947,22.2847987209526,22.3591079335028,
22.4036884637069,22.4482924175264),.UNSPECIFIED.);
#998=B_SPLINE_CURVE_WITH_KNOTS('',3,(#23824,#23825,#23826,#23827,#23828,
#23829,#23830,#23831),.UNSPECIFIED.,.F.,.F.,(4,2,2,4),(9.99999993021828E-7,
0.0391830186935133,0.0774132307502166,0.0931362008875077),.UNSPECIFIED.);
#999=B_SPLINE_CURVE_WITH_KNOTS('',3,(#23856,#23857,#23858,#23859,#23860,
#23861,#23862,#23863,#23864,#23865,#23866,#23867,#23868,#23869,#23870,#23871,
#23872,#23873,#23874,#23875,#23876,#23877,#23878,#23879,#23880,#23881,#23882,
#23883),.UNSPECIFIED.,.F.,.F.,(4,2,2,2,2,2,2,2,2,2,2,2,2,4),(9.99999999757183E-7,
0.0731124278909269,0.166057761117533,0.286367941469741,0.41317168458484,
0.536466369898799,0.671513511979461,0.863012275266548,1.04829331747803,
1.23237898344787,1.40408133486915,1.58846641457555,1.74526991258573,1.84895017902434),
 .UNSPECIFIED.);
#1000=B_SPLINE_CURVE_WITH_KNOTS('',3,(#23885,#23886,#23887,#23888,#23889,
#23890,#23891,#23892,#23893,#23894,#23895,#23896),.UNSPECIFIED.,.F.,.F.,
(4,2,2,2,2,4),(1.00000013382259E-6,0.059650139456479,0.121379110068548,
0.202618081235281,0.282064568203206,0.362961601069192),.UNSPECIFIED.);
#1001=B_SPLINE_CURVE_WITH_KNOTS('',3,(#23899,#23900,#23901,#23902,#23903,
#23904,#23905,#23906,#23907,#23908,#23909,#23910,#23911,#23912),
 .UNSPECIFIED.,.F.,.F.,(4,2,2,2,2,2,4),(1.84895017902434,1.87439516116018,
2.01076363118188,2.16135413763144,2.34266213664141,2.4563787856096,2.57527002953519),
 .UNSPECIFIED.);
#1002=B_SPLINE_CURVE_WITH_KNOTS('',3,(#23918,#23919,#23920,#23921,#23922,
#23923,#23924,#23925,#23926,#23927,#23928,#23929,#23930,#23931,#23932,#23933,
#23934,#23935,#23936,#23937,#23938,#23939,#23940,#23941,#23942,#23943,#23944,
#23945),.UNSPECIFIED.,.F.,.F.,(4,2,2,2,2,2,2,2,2,2,2,2,2,4),(9.99999999927736E-7,
0.0731124278938116,0.166057761124268,0.286367941476178,0.413171684591601,
0.536466369905737,0.671513511989027,0.863012275271149,1.04829331747739,
1.23237898344594,1.40408133486366,1.58846641456642,1.7452699125751,1.84895017900088),
 .UNSPECIFIED.);
#1003=B_SPLINE_CURVE_WITH_KNOTS('',3,(#23947,#23948,#23949,#23950,#23951,
#23952,#23953,#23954,#23955,#23956,#23957,#23958),.UNSPECIFIED.,.F.,.F.,
(4,2,2,2,2,4),(0.,0.0596482959180104,0.121377436598889,0.202616631617369,
0.282063337473005,0.362960593220025),.UNSPECIFIED.);
#1004=B_SPLINE_CURVE_WITH_KNOTS('',3,(#23961,#23962,#23963,#23964,#23965,
#23966,#23967,#23968,#23969,#23970,#23971,#23972,#23973,#23974),
 .UNSPECIFIED.,.F.,.F.,(4,2,2,2,2,2,4),(1.84895017900088,1.87439516115146,
2.01076363117394,2.16135413764315,2.34266213672471,2.45637878572962,2.57527002969303),
 .UNSPECIFIED.);
#1005=B_SPLINE_CURVE_WITH_KNOTS('',3,(#23980,#23981,#23982,#23983,#23984,
#23985,#23986,#23987,#23988,#23989,#23990,#23991,#23992,#23993,#23994,#23995,
#23996,#23997,#23998,#23999,#24000,#24001,#24002,#24003,#24004,#24005,#24006,
#24007),.UNSPECIFIED.,.F.,.F.,(4,2,2,2,2,2,2,2,2,2,2,2,2,4),(9.99999999995091E-7,
0.0731124278961,0.166057761129691,0.286367941481508,0.413171684597363,0.536466369911867,
0.671513511997779,0.863012275276778,1.04829331747967,1.23237898344799,1.40408133486366,
1.58846641456439,1.74526991257199,1.84895017898734),.UNSPECIFIED.);
#1006=B_SPLINE_CURVE_WITH_KNOTS('',3,(#24009,#24010,#24011,#24012,#24013,
#24014,#24015,#24016,#24017,#24018,#24019,#24020),.UNSPECIFIED.,.F.,.F.,
(4,2,2,2,2,4),(1.0000001340625E-6,0.0596501394587982,0.121379110070747,
0.202618081237259,0.282064568204757,0.36296160107052),.UNSPECIFIED.);
#1007=B_SPLINE_CURVE_WITH_KNOTS('',3,(#24023,#24024,#24025,#24026,#24027,
#24028,#24029,#24030,#24031,#24032,#24033,#24034,#24035,#24036),
 .UNSPECIFIED.,.F.,.F.,(4,2,2,2,2,2,4),(1.84895017898734,1.87439516114959,
2.01076363117243,2.16135413765848,2.34266213680017,2.45637878583639,2.57527002983203),
 .UNSPECIFIED.);
#1008=B_SPLINE_CURVE_WITH_KNOTS('',3,(#24042,#24043,#24044,#24045,#24046,
#24047,#24048,#24049,#24050,#24051,#24052,#24053,#24054,#24055,#24056,#24057,
#24058,#24059,#24060,#24061,#24062,#24063,#24064,#24065,#24066,#24067,#24068,
#24069),.UNSPECIFIED.,.F.,.F.,(4,2,2,2,2,2,2,2,2,2,2,2,2,4),(9.99999999927736E-7,
0.0731124278938116,0.166057761124268,0.286367941476178,0.413171684591601,
0.536466369905737,0.671513511989027,0.863012275271149,1.04829331747739,
1.23237898344594,1.40408133486366,1.58846641456642,1.7452699125751,1.84895017900088),
 .UNSPECIFIED.);
#1009=B_SPLINE_CURVE_WITH_KNOTS('',3,(#24071,#24072,#24073,#24074,#24075,
#24076,#24077,#24078,#24079,#24080,#24081,#24082),.UNSPECIFIED.,.F.,.F.,
(4,2,2,2,2,4),(0.,0.0596482959180104,0.121377436598889,0.202616631617369,
0.282063337473005,0.362960593220025),.UNSPECIFIED.);
#1010=B_SPLINE_CURVE_WITH_KNOTS('',3,(#24085,#24086,#24087,#24088,#24089,
#24090,#24091,#24092,#24093,#24094,#24095,#24096,#24097,#24098),
 .UNSPECIFIED.,.F.,.F.,(4,2,2,2,2,2,4),(1.84895017900088,1.87439516115146,
2.01076363117394,2.16135413764315,2.34266213672471,2.45637878572962,2.57527002969303),
 .UNSPECIFIED.);
#1019=TOROIDAL_SURFACE('',#11444,1.905,1.27);
#1020=TOROIDAL_SURFACE('',#11480,1.905,1.27);
#1021=TOROIDAL_SURFACE('',#11516,1.905,1.27);
#1022=TOROIDAL_SURFACE('',#11552,1.905,1.27);
#1027=FACE_OUTER_BOUND('',#1641,.T.);
#1028=FACE_OUTER_BOUND('',#1642,.T.);
#1029=FACE_OUTER_BOUND('',#1643,.T.);
#1030=FACE_OUTER_BOUND('',#1644,.T.);
#1031=FACE_OUTER_BOUND('',#1645,.T.);
#1032=FACE_OUTER_BOUND('',#1646,.T.);
#1033=FACE_OUTER_BOUND('',#1647,.T.);
#1034=FACE_OUTER_BOUND('',#1648,.T.);
#1035=FACE_OUTER_BOUND('',#1649,.T.);
#1036=FACE_OUTER_BOUND('',#1650,.T.);
#1037=FACE_OUTER_BOUND('',#1651,.T.);
#1038=FACE_OUTER_BOUND('',#1652,.T.);
#1039=FACE_OUTER_BOUND('',#1653,.T.);
#1040=FACE_OUTER_BOUND('',#1654,.T.);
#1041=FACE_OUTER_BOUND('',#1655,.T.);
#1042=FACE_OUTER_BOUND('',#1656,.T.);
#1043=FACE_OUTER_BOUND('',#1657,.T.);
#1044=FACE_OUTER_BOUND('',#1658,.T.);
#1045=FACE_OUTER_BOUND('',#1659,.T.);
#1046=FACE_OUTER_BOUND('',#1660,.T.);
#1047=FACE_OUTER_BOUND('',#1661,.T.);
#1048=FACE_OUTER_BOUND('',#1662,.T.);
#1049=FACE_OUTER_BOUND('',#1663,.T.);
#1050=FACE_OUTER_BOUND('',#1664,.T.);
#1051=FACE_OUTER_BOUND('',#1665,.T.);
#1052=FACE_OUTER_BOUND('',#1666,.T.);
#1053=FACE_OUTER_BOUND('',#1667,.T.);
#1054=FACE_OUTER_BOUND('',#1668,.T.);
#1055=FACE_OUTER_BOUND('',#1669,.T.);
#1056=FACE_OUTER_BOUND('',#1670,.T.);
#1057=FACE_OUTER_BOUND('',#1671,.T.);
#1058=FACE_OUTER_BOUND('',#1672,.T.);
#1059=FACE_OUTER_BOUND('',#1673,.T.);
#1060=FACE_OUTER_BOUND('',#1674,.T.);
#1061=FACE_OUTER_BOUND('',#1675,.T.);
#1062=FACE_OUTER_BOUND('',#1676,.T.);
#1063=FACE_OUTER_BOUND('',#1677,.T.);
#1064=FACE_OUTER_BOUND('',#1678,.T.);
#1065=FACE_OUTER_BOUND('',#1679,.T.);
#1066=FACE_OUTER_BOUND('',#1680,.T.);
#1067=FACE_OUTER_BOUND('',#1681,.T.);
#1068=FACE_OUTER_BOUND('',#1682,.T.);
#1069=FACE_OUTER_BOUND('',#1683,.T.);
#1070=FACE_OUTER_BOUND('',#1684,.T.);
#1071=FACE_OUTER_BOUND('',#1685,.T.);
#1072=FACE_OUTER_BOUND('',#1686,.T.);
#1073=FACE_OUTER_BOUND('',#1687,.T.);
#1074=FACE_OUTER_BOUND('',#1688,.T.);
#1075=FACE_OUTER_BOUND('',#1689,.T.);
#1076=FACE_OUTER_BOUND('',#1690,.T.);
#1077=FACE_OUTER_BOUND('',#1691,.T.);
#1078=FACE_OUTER_BOUND('',#1692,.T.);
#1079=FACE_OUTER_BOUND('',#1693,.T.);
#1080=FACE_OUTER_BOUND('',#1694,.T.);
#1081=FACE_OUTER_BOUND('',#1695,.T.);
#1082=FACE_OUTER_BOUND('',#1696,.T.);
#1083=FACE_OUTER_BOUND('',#1697,.T.);
#1084=FACE_OUTER_BOUND('',#1698,.T.);
#1085=FACE_OUTER_BOUND('',#1699,.T.);
#1086=FACE_OUTER_BOUND('',#1700,.T.);
#1087=FACE_OUTER_BOUND('',#1701,.T.);
#1088=FACE_OUTER_BOUND('',#1702,.T.);
#1089=FACE_OUTER_BOUND('',#1703,.T.);
#1090=FACE_OUTER_BOUND('',#1704,.T.);
#1091=FACE_OUTER_BOUND('',#1705,.T.);
#1092=FACE_OUTER_BOUND('',#1706,.T.);
#1093=FACE_OUTER_BOUND('',#1707,.T.);
#1094=FACE_OUTER_BOUND('',#1708,.T.);
#1095=FACE_OUTER_BOUND('',#1709,.T.);
#1096=FACE_OUTER_BOUND('',#1710,.T.);
#1097=FACE_OUTER_BOUND('',#1711,.T.);
#1098=FACE_OUTER_BOUND('',#1712,.T.);
#1099=FACE_OUTER_BOUND('',#1713,.T.);
#1100=FACE_OUTER_BOUND('',#1714,.T.);
#1101=FACE_OUTER_BOUND('',#1715,.T.);
#1102=FACE_OUTER_BOUND('',#1716,.T.);
#1103=FACE_OUTER_BOUND('',#1717,.T.);
#1104=FACE_OUTER_BOUND('',#1718,.T.);
#1105=FACE_OUTER_BOUND('',#1719,.T.);
#1106=FACE_OUTER_BOUND('',#1720,.T.);
#1107=FACE_OUTER_BOUND('',#1721,.T.);
#1108=FACE_OUTER_BOUND('',#1722,.T.);
#1109=FACE_OUTER_BOUND('',#1723,.T.);
#1110=FACE_OUTER_BOUND('',#1724,.T.);
#1111=FACE_OUTER_BOUND('',#1725,.T.);
#1112=FACE_OUTER_BOUND('',#1726,.T.);
#1113=FACE_OUTER_BOUND('',#1727,.T.);
#1114=FACE_OUTER_BOUND('',#1728,.T.);
#1115=FACE_OUTER_BOUND('',#1729,.T.);
#1116=FACE_OUTER_BOUND('',#1730,.T.);
#1117=FACE_OUTER_BOUND('',#1731,.T.);
#1118=FACE_OUTER_BOUND('',#1732,.T.);
#1119=FACE_OUTER_BOUND('',#1733,.T.);
#1120=FACE_OUTER_BOUND('',#1734,.T.);
#1121=FACE_OUTER_BOUND('',#1735,.T.);
#1122=FACE_OUTER_BOUND('',#1736,.T.);
#1123=FACE_OUTER_BOUND('',#1737,.T.);
#1124=FACE_OUTER_BOUND('',#1738,.T.);
#1125=FACE_OUTER_BOUND('',#1739,.T.);
#1126=FACE_OUTER_BOUND('',#1740,.T.);
#1127=FACE_OUTER_BOUND('',#1741,.T.);
#1128=FACE_OUTER_BOUND('',#1742,.T.);
#1129=FACE_OUTER_BOUND('',#1743,.T.);
#1130=FACE_OUTER_BOUND('',#1744,.T.);
#1131=FACE_OUTER_BOUND('',#1745,.T.);
#1132=FACE_OUTER_BOUND('',#1746,.T.);
#1133=FACE_OUTER_BOUND('',#1747,.T.);
#1134=FACE_OUTER_BOUND('',#1748,.T.);
#1135=FACE_OUTER_BOUND('',#1749,.T.);
#1136=FACE_OUTER_BOUND('',#1750,.T.);
#1137=FACE_OUTER_BOUND('',#1751,.T.);
#1138=FACE_OUTER_BOUND('',#1752,.T.);
#1139=FACE_OUTER_BOUND('',#1753,.T.);
#1140=FACE_OUTER_BOUND('',#1754,.T.);
#1141=FACE_OUTER_BOUND('',#1755,.T.);
#1142=FACE_OUTER_BOUND('',#1756,.T.);
#1143=FACE_OUTER_BOUND('',#1757,.T.);
#1144=FACE_OUTER_BOUND('',#1758,.T.);
#1145=FACE_OUTER_BOUND('',#1759,.T.);
#1146=FACE_OUTER_BOUND('',#1760,.T.);
#1147=FACE_OUTER_BOUND('',#1761,.T.);
#1148=FACE_OUTER_BOUND('',#1762,.T.);
#1149=FACE_OUTER_BOUND('',#1763,.T.);
#1150=FACE_OUTER_BOUND('',#1764,.T.);
#1151=FACE_OUTER_BOUND('',#1765,.T.);
#1152=FACE_OUTER_BOUND('',#1766,.T.);
#1153=FACE_OUTER_BOUND('',#1767,.T.);
#1154=FACE_OUTER_BOUND('',#1768,.T.);
#1155=FACE_OUTER_BOUND('',#1769,.T.);
#1156=FACE_OUTER_BOUND('',#1770,.T.);
#1157=FACE_OUTER_BOUND('',#1771,.T.);
#1158=FACE_OUTER_BOUND('',#1772,.T.);
#1159=FACE_OUTER_BOUND('',#1773,.T.);
#1160=FACE_OUTER_BOUND('',#1774,.T.);
#1161=FACE_OUTER_BOUND('',#1775,.T.);
#1162=FACE_OUTER_BOUND('',#1776,.T.);
#1163=FACE_OUTER_BOUND('',#1777,.T.);
#1164=FACE_OUTER_BOUND('',#1778,.T.);
#1165=FACE_OUTER_BOUND('',#1779,.T.);
#1166=FACE_OUTER_BOUND('',#1780,.T.);
#1167=FACE_OUTER_BOUND('',#1781,.T.);
#1168=FACE_OUTER_BOUND('',#1782,.T.);
#1169=FACE_OUTER_BOUND('',#1783,.T.);
#1170=FACE_OUTER_BOUND('',#1784,.T.);
#1171=FACE_OUTER_BOUND('',#1785,.T.);
#1172=FACE_OUTER_BOUND('',#1786,.T.);
#1173=FACE_OUTER_BOUND('',#1787,.T.);
#1174=FACE_OUTER_BOUND('',#1788,.T.);
#1175=FACE_OUTER_BOUND('',#1789,.T.);
#1176=FACE_OUTER_BOUND('',#1790,.T.);
#1177=FACE_OUTER_BOUND('',#1791,.T.);
#1178=FACE_OUTER_BOUND('',#1792,.T.);
#1179=FACE_OUTER_BOUND('',#1793,.T.);
#1180=FACE_OUTER_BOUND('',#1794,.T.);
#1181=FACE_OUTER_BOUND('',#1795,.T.);
#1182=FACE_OUTER_BOUND('',#1796,.T.);
#1183=FACE_OUTER_BOUND('',#1797,.T.);
#1184=FACE_OUTER_BOUND('',#1798,.T.);
#1185=FACE_OUTER_BOUND('',#1799,.T.);
#1186=FACE_OUTER_BOUND('',#1800,.T.);
#1187=FACE_OUTER_BOUND('',#1801,.T.);
#1188=FACE_OUTER_BOUND('',#1802,.T.);
#1189=FACE_OUTER_BOUND('',#1803,.T.);
#1190=FACE_OUTER_BOUND('',#1804,.T.);
#1191=FACE_OUTER_BOUND('',#1805,.T.);
#1192=FACE_OUTER_BOUND('',#1806,.T.);
#1193=FACE_OUTER_BOUND('',#1807,.T.);
#1194=FACE_OUTER_BOUND('',#1808,.T.);
#1195=FACE_OUTER_BOUND('',#1809,.T.);
#1196=FACE_OUTER_BOUND('',#1810,.T.);
#1197=FACE_OUTER_BOUND('',#1811,.T.);
#1198=FACE_OUTER_BOUND('',#1812,.T.);
#1199=FACE_OUTER_BOUND('',#1813,.T.);
#1200=FACE_OUTER_BOUND('',#1814,.T.);
#1201=FACE_OUTER_BOUND('',#1815,.T.);
#1202=FACE_OUTER_BOUND('',#1816,.T.);
#1203=FACE_OUTER_BOUND('',#1817,.T.);
#1204=FACE_OUTER_BOUND('',#1818,.T.);
#1205=FACE_OUTER_BOUND('',#1819,.T.);
#1206=FACE_OUTER_BOUND('',#1820,.T.);
#1207=FACE_OUTER_BOUND('',#1821,.T.);
#1208=FACE_OUTER_BOUND('',#1822,.T.);
#1209=FACE_OUTER_BOUND('',#1823,.T.);
#1210=FACE_OUTER_BOUND('',#1824,.T.);
#1211=FACE_OUTER_BOUND('',#1825,.T.);
#1212=FACE_OUTER_BOUND('',#1826,.T.);
#1213=FACE_OUTER_BOUND('',#1827,.T.);
#1214=FACE_OUTER_BOUND('',#1828,.T.);
#1215=FACE_OUTER_BOUND('',#1829,.T.);
#1216=FACE_OUTER_BOUND('',#1830,.T.);
#1217=FACE_OUTER_BOUND('',#1831,.T.);
#1218=FACE_OUTER_BOUND('',#1832,.T.);
#1219=FACE_OUTER_BOUND('',#1833,.T.);
#1220=FACE_OUTER_BOUND('',#1834,.T.);
#1221=FACE_OUTER_BOUND('',#1835,.T.);
#1222=FACE_OUTER_BOUND('',#1836,.T.);
#1223=FACE_OUTER_BOUND('',#1837,.T.);
#1224=FACE_OUTER_BOUND('',#1838,.T.);
#1225=FACE_OUTER_BOUND('',#1839,.T.);
#1226=FACE_OUTER_BOUND('',#1840,.T.);
#1227=FACE_OUTER_BOUND('',#1841,.T.);
#1228=FACE_OUTER_BOUND('',#1842,.T.);
#1229=FACE_OUTER_BOUND('',#1843,.T.);
#1230=FACE_OUTER_BOUND('',#1844,.T.);
#1231=FACE_OUTER_BOUND('',#1850,.T.);
#1232=FACE_OUTER_BOUND('',#1851,.T.);
#1233=FACE_OUTER_BOUND('',#1852,.T.);
#1234=FACE_OUTER_BOUND('',#1853,.T.);
#1235=FACE_OUTER_BOUND('',#1854,.T.);
#1236=FACE_OUTER_BOUND('',#1855,.T.);
#1237=FACE_OUTER_BOUND('',#1856,.T.);
#1238=FACE_OUTER_BOUND('',#1857,.T.);
#1239=FACE_OUTER_BOUND('',#1858,.T.);
#1240=FACE_OUTER_BOUND('',#1859,.T.);
#1241=FACE_OUTER_BOUND('',#1860,.T.);
#1242=FACE_OUTER_BOUND('',#1861,.T.);
#1243=FACE_OUTER_BOUND('',#1862,.T.);
#1244=FACE_OUTER_BOUND('',#1864,.T.);
#1245=FACE_OUTER_BOUND('',#1866,.T.);
#1246=FACE_OUTER_BOUND('',#1867,.T.);
#1247=FACE_OUTER_BOUND('',#1868,.T.);
#1248=FACE_OUTER_BOUND('',#1869,.T.);
#1249=FACE_OUTER_BOUND('',#1870,.T.);
#1250=FACE_OUTER_BOUND('',#1871,.T.);
#1251=FACE_OUTER_BOUND('',#1872,.T.);
#1252=FACE_OUTER_BOUND('',#1873,.T.);
#1253=FACE_OUTER_BOUND('',#1874,.T.);
#1254=FACE_OUTER_BOUND('',#1875,.T.);
#1255=FACE_OUTER_BOUND('',#1876,.T.);
#1256=FACE_OUTER_BOUND('',#1877,.T.);
#1257=FACE_OUTER_BOUND('',#1878,.T.);
#1258=FACE_OUTER_BOUND('',#1879,.T.);
#1259=FACE_OUTER_BOUND('',#1880,.T.);
#1260=FACE_OUTER_BOUND('',#1881,.T.);
#1261=FACE_OUTER_BOUND('',#1882,.T.);
#1262=FACE_OUTER_BOUND('',#1888,.T.);
#1263=FACE_OUTER_BOUND('',#1889,.T.);
#1264=FACE_OUTER_BOUND('',#1890,.T.);
#1265=FACE_OUTER_BOUND('',#1891,.T.);
#1266=FACE_OUTER_BOUND('',#1892,.T.);
#1267=FACE_OUTER_BOUND('',#1894,.T.);
#1268=FACE_OUTER_BOUND('',#1895,.T.);
#1269=FACE_OUTER_BOUND('',#1896,.T.);
#1270=FACE_OUTER_BOUND('',#1897,.T.);
#1271=FACE_OUTER_BOUND('',#1898,.T.);
#1272=FACE_OUTER_BOUND('',#1899,.T.);
#1273=FACE_OUTER_BOUND('',#1900,.T.);
#1274=FACE_OUTER_BOUND('',#1901,.T.);
#1275=FACE_OUTER_BOUND('',#1902,.T.);
#1276=FACE_OUTER_BOUND('',#1903,.T.);
#1277=FACE_OUTER_BOUND('',#1904,.T.);
#1278=FACE_OUTER_BOUND('',#1905,.T.);
#1279=FACE_OUTER_BOUND('',#1906,.T.);
#1280=FACE_OUTER_BOUND('',#1907,.T.);
#1281=FACE_OUTER_BOUND('',#1908,.T.);
#1282=FACE_OUTER_BOUND('',#1909,.T.);
#1283=FACE_OUTER_BOUND('',#1910,.T.);
#1284=FACE_OUTER_BOUND('',#1911,.T.);
#1285=FACE_OUTER_BOUND('',#1912,.T.);
#1286=FACE_OUTER_BOUND('',#1913,.T.);
#1287=FACE_OUTER_BOUND('',#1914,.T.);
#1288=FACE_OUTER_BOUND('',#1915,.T.);
#1289=FACE_OUTER_BOUND('',#1916,.T.);
#1290=FACE_OUTER_BOUND('',#1918,.T.);
#1291=FACE_OUTER_BOUND('',#1919,.T.);
#1292=FACE_OUTER_BOUND('',#1925,.T.);
#1293=FACE_OUTER_BOUND('',#1926,.T.);
#1294=FACE_OUTER_BOUND('',#1927,.T.);
#1295=FACE_OUTER_BOUND('',#1928,.T.);
#1296=FACE_OUTER_BOUND('',#1929,.T.);
#1297=FACE_OUTER_BOUND('',#1930,.T.);
#1298=FACE_OUTER_BOUND('',#1931,.T.);
#1299=FACE_OUTER_BOUND('',#1932,.T.);
#1300=FACE_OUTER_BOUND('',#1933,.T.);
#1301=FACE_OUTER_BOUND('',#1934,.T.);
#1302=FACE_OUTER_BOUND('',#1935,.T.);
#1303=FACE_OUTER_BOUND('',#1936,.T.);
#1304=FACE_OUTER_BOUND('',#1937,.T.);
#1305=FACE_OUTER_BOUND('',#1938,.T.);
#1306=FACE_OUTER_BOUND('',#1939,.T.);
#1307=FACE_OUTER_BOUND('',#1940,.T.);
#1308=FACE_OUTER_BOUND('',#1941,.T.);
#1309=FACE_OUTER_BOUND('',#1942,.T.);
#1310=FACE_OUTER_BOUND('',#1943,.T.);
#1311=FACE_OUTER_BOUND('',#1944,.T.);
#1312=FACE_OUTER_BOUND('',#1946,.T.);
#1313=FACE_OUTER_BOUND('',#1948,.T.);
#1314=FACE_OUTER_BOUND('',#1949,.T.);
#1315=FACE_OUTER_BOUND('',#1950,.T.);
#1316=FACE_OUTER_BOUND('',#1951,.T.);
#1317=FACE_OUTER_BOUND('',#1952,.T.);
#1318=FACE_OUTER_BOUND('',#1953,.T.);
#1319=FACE_OUTER_BOUND('',#1955,.T.);
#1320=FACE_OUTER_BOUND('',#1961,.T.);
#1321=FACE_OUTER_BOUND('',#1962,.T.);
#1322=FACE_OUTER_BOUND('',#1963,.T.);
#1323=FACE_OUTER_BOUND('',#1964,.T.);
#1324=FACE_OUTER_BOUND('',#1965,.T.);
#1325=FACE_OUTER_BOUND('',#1966,.T.);
#1326=FACE_OUTER_BOUND('',#1967,.T.);
#1327=FACE_OUTER_BOUND('',#1968,.T.);
#1328=FACE_OUTER_BOUND('',#1969,.T.);
#1329=FACE_OUTER_BOUND('',#1970,.T.);
#1330=FACE_OUTER_BOUND('',#1971,.T.);
#1331=FACE_OUTER_BOUND('',#1972,.T.);
#1641=EDGE_LOOP('',(#7238,#7239,#7240,#7241,#7242));
#1642=EDGE_LOOP('',(#7243,#7244,#7245,#7246,#7247,#7248,#7249,#7250,#7251,
#7252,#7253,#7254,#7255,#7256,#7257,#7258,#7259,#7260,#7261,#7262,#7263));
#1643=EDGE_LOOP('',(#7264,#7265,#7266));
#1644=EDGE_LOOP('',(#7267,#7268,#7269));
#1645=EDGE_LOOP('',(#7270,#7271,#7272));
#1646=EDGE_LOOP('',(#7273));
#1647=EDGE_LOOP('',(#7274,#7275,#7276));
#1648=EDGE_LOOP('',(#7277,#7278,#7279,#7280,#7281));
#1649=EDGE_LOOP('',(#7282,#7283,#7284,#7285,#7286));
#1650=EDGE_LOOP('',(#7287,#7288,#7289,#7290,#7291));
#1651=EDGE_LOOP('',(#7292,#7293,#7294,#7295));
#1652=EDGE_LOOP('',(#7296,#7297,#7298,#7299,#7300));
#1653=EDGE_LOOP('',(#7301,#7302,#7303,#7304));
#1654=EDGE_LOOP('',(#7305,#7306,#7307,#7308,#7309,#7310,#7311,#7312,#7313,
#7314,#7315,#7316));
#1655=EDGE_LOOP('',(#7317,#7318,#7319,#7320));
#1656=EDGE_LOOP('',(#7321,#7322,#7323,#7324,#7325));
#1657=EDGE_LOOP('',(#7326,#7327,#7328,#7329,#7330));
#1658=EDGE_LOOP('',(#7331,#7332,#7333,#7334,#7335));
#1659=EDGE_LOOP('',(#7336,#7337,#7338,#7339,#7340));
#1660=EDGE_LOOP('',(#7341,#7342,#7343,#7344,#7345));
#1661=EDGE_LOOP('',(#7346,#7347,#7348,#7349,#7350));
#1662=EDGE_LOOP('',(#7351,#7352,#7353,#7354,#7355,#7356,#7357,#7358,#7359,
#7360,#7361,#7362,#7363,#7364,#7365,#7366,#7367,#7368,#7369,#7370,#7371));
#1663=EDGE_LOOP('',(#7372,#7373,#7374));
#1664=EDGE_LOOP('',(#7375,#7376,#7377));
#1665=EDGE_LOOP('',(#7378,#7379,#7380));
#1666=EDGE_LOOP('',(#7381));
#1667=EDGE_LOOP('',(#7382,#7383,#7384));
#1668=EDGE_LOOP('',(#7385,#7386,#7387,#7388,#7389));
#1669=EDGE_LOOP('',(#7390,#7391,#7392,#7393,#7394));
#1670=EDGE_LOOP('',(#7395,#7396,#7397,#7398,#7399));
#1671=EDGE_LOOP('',(#7400,#7401,#7402,#7403));
#1672=EDGE_LOOP('',(#7404,#7405,#7406,#7407,#7408));
#1673=EDGE_LOOP('',(#7409,#7410,#7411,#7412));
#1674=EDGE_LOOP('',(#7413,#7414,#7415,#7416,#7417,#7418,#7419,#7420,#7421,
#7422,#7423,#7424));
#1675=EDGE_LOOP('',(#7425,#7426,#7427,#7428));
#1676=EDGE_LOOP('',(#7429,#7430,#7431,#7432,#7433));
#1677=EDGE_LOOP('',(#7434,#7435,#7436,#7437,#7438));
#1678=EDGE_LOOP('',(#7439,#7440,#7441,#7442,#7443));
#1679=EDGE_LOOP('',(#7444,#7445,#7446,#7447,#7448));
#1680=EDGE_LOOP('',(#7449,#7450,#7451,#7452,#7453));
#1681=EDGE_LOOP('',(#7454,#7455,#7456,#7457,#7458));
#1682=EDGE_LOOP('',(#7459,#7460,#7461,#7462,#7463,#7464,#7465,#7466,#7467,
#7468,#7469,#7470,#7471,#7472,#7473,#7474,#7475,#7476,#7477,#7478,#7479));
#1683=EDGE_LOOP('',(#7480,#7481,#7482));
#1684=EDGE_LOOP('',(#7483,#7484,#7485));
#1685=EDGE_LOOP('',(#7486,#7487,#7488));
#1686=EDGE_LOOP('',(#7489));
#1687=EDGE_LOOP('',(#7490,#7491,#7492));
#1688=EDGE_LOOP('',(#7493,#7494,#7495,#7496,#7497));
#1689=EDGE_LOOP('',(#7498,#7499,#7500,#7501,#7502));
#1690=EDGE_LOOP('',(#7503,#7504,#7505,#7506,#7507));
#1691=EDGE_LOOP('',(#7508,#7509,#7510,#7511));
#1692=EDGE_LOOP('',(#7512,#7513,#7514,#7515,#7516));
#1693=EDGE_LOOP('',(#7517,#7518,#7519,#7520));
#1694=EDGE_LOOP('',(#7521,#7522,#7523,#7524,#7525,#7526,#7527,#7528,#7529,
#7530,#7531,#7532));
#1695=EDGE_LOOP('',(#7533,#7534,#7535,#7536));
#1696=EDGE_LOOP('',(#7537,#7538,#7539,#7540,#7541));
#1697=EDGE_LOOP('',(#7542,#7543,#7544,#7545,#7546));
#1698=EDGE_LOOP('',(#7547,#7548,#7549,#7550,#7551));
#1699=EDGE_LOOP('',(#7552,#7553,#7554,#7555,#7556));
#1700=EDGE_LOOP('',(#7557,#7558,#7559,#7560,#7561));
#1701=EDGE_LOOP('',(#7562,#7563,#7564,#7565,#7566));
#1702=EDGE_LOOP('',(#7567,#7568,#7569,#7570,#7571,#7572,#7573,#7574,#7575,
#7576,#7577,#7578,#7579,#7580,#7581,#7582,#7583,#7584,#7585,#7586,#7587));
#1703=EDGE_LOOP('',(#7588,#7589,#7590));
#1704=EDGE_LOOP('',(#7591,#7592,#7593));
#1705=EDGE_LOOP('',(#7594,#7595,#7596));
#1706=EDGE_LOOP('',(#7597));
#1707=EDGE_LOOP('',(#7598,#7599,#7600));
#1708=EDGE_LOOP('',(#7601,#7602,#7603,#7604,#7605));
#1709=EDGE_LOOP('',(#7606,#7607,#7608,#7609,#7610));
#1710=EDGE_LOOP('',(#7611,#7612,#7613,#7614,#7615));
#1711=EDGE_LOOP('',(#7616,#7617,#7618,#7619));
#1712=EDGE_LOOP('',(#7620,#7621,#7622,#7623,#7624));
#1713=EDGE_LOOP('',(#7625,#7626,#7627,#7628));
#1714=EDGE_LOOP('',(#7629,#7630,#7631,#7632,#7633,#7634,#7635,#7636,#7637,
#7638,#7639,#7640));
#1715=EDGE_LOOP('',(#7641,#7642,#7643,#7644));
#1716=EDGE_LOOP('',(#7645,#7646,#7647,#7648,#7649));
#1717=EDGE_LOOP('',(#7650,#7651,#7652,#7653,#7654));
#1718=EDGE_LOOP('',(#7655,#7656,#7657,#7658,#7659));
#1719=EDGE_LOOP('',(#7660,#7661,#7662,#7663,#7664));
#1720=EDGE_LOOP('',(#7665,#7666,#7667,#7668,#7669));
#1721=EDGE_LOOP('',(#7670,#7671,#7672,#7673));
#1722=EDGE_LOOP('',(#7674,#7675,#7676,#7677));
#1723=EDGE_LOOP('',(#7678,#7679,#7680,#7681));
#1724=EDGE_LOOP('',(#7682,#7683,#7684,#7685));
#1725=EDGE_LOOP('',(#7686,#7687,#7688,#7689));
#1726=EDGE_LOOP('',(#7690,#7691,#7692,#7693));
#1727=EDGE_LOOP('',(#7694,#7695,#7696,#7697));
#1728=EDGE_LOOP('',(#7698,#7699,#7700,#7701));
#1729=EDGE_LOOP('',(#7702,#7703,#7704,#7705));
#1730=EDGE_LOOP('',(#7706,#7707,#7708,#7709));
#1731=EDGE_LOOP('',(#7710,#7711,#7712,#7713));
#1732=EDGE_LOOP('',(#7714,#7715,#7716,#7717));
#1733=EDGE_LOOP('',(#7718,#7719,#7720,#7721));
#1734=EDGE_LOOP('',(#7722,#7723,#7724,#7725));
#1735=EDGE_LOOP('',(#7726,#7727,#7728,#7729));
#1736=EDGE_LOOP('',(#7730,#7731,#7732,#7733));
#1737=EDGE_LOOP('',(#7734,#7735,#7736,#7737));
#1738=EDGE_LOOP('',(#7738,#7739,#7740,#7741));
#1739=EDGE_LOOP('',(#7742,#7743,#7744,#7745));
#1740=EDGE_LOOP('',(#7746,#7747,#7748,#7749));
#1741=EDGE_LOOP('',(#7750,#7751,#7752,#7753));
#1742=EDGE_LOOP('',(#7754,#7755,#7756,#7757));
#1743=EDGE_LOOP('',(#7758,#7759,#7760,#7761));
#1744=EDGE_LOOP('',(#7762,#7763,#7764,#7765));
#1745=EDGE_LOOP('',(#7766,#7767,#7768,#7769));
#1746=EDGE_LOOP('',(#7770,#7771,#7772,#7773));
#1747=EDGE_LOOP('',(#7774,#7775,#7776,#7777));
#1748=EDGE_LOOP('',(#7778,#7779,#7780,#7781));
#1749=EDGE_LOOP('',(#7782,#7783,#7784,#7785));
#1750=EDGE_LOOP('',(#7786,#7787,#7788,#7789));
#1751=EDGE_LOOP('',(#7790,#7791,#7792,#7793));
#1752=EDGE_LOOP('',(#7794,#7795,#7796,#7797));
#1753=EDGE_LOOP('',(#7798,#7799,#7800,#7801));
#1754=EDGE_LOOP('',(#7802,#7803,#7804,#7805));
#1755=EDGE_LOOP('',(#7806,#7807,#7808,#7809));
#1756=EDGE_LOOP('',(#7810,#7811,#7812,#7813));
#1757=EDGE_LOOP('',(#7814,#7815,#7816,#7817));
#1758=EDGE_LOOP('',(#7818,#7819,#7820,#7821));
#1759=EDGE_LOOP('',(#7822,#7823,#7824));
#1760=EDGE_LOOP('',(#7825,#7826,#7827,#7828));
#1761=EDGE_LOOP('',(#7829,#7830,#7831,#7832));
#1762=EDGE_LOOP('',(#7833,#7834,#7835,#7836));
#1763=EDGE_LOOP('',(#7837,#7838,#7839,#7840));
#1764=EDGE_LOOP('',(#7841,#7842,#7843,#7844));
#1765=EDGE_LOOP('',(#7845,#7846,#7847,#7848));
#1766=EDGE_LOOP('',(#7849,#7850,#7851,#7852));
#1767=EDGE_LOOP('',(#7853,#7854,#7855,#7856));
#1768=EDGE_LOOP('',(#7857,#7858,#7859,#7860));
#1769=EDGE_LOOP('',(#7861,#7862,#7863,#7864));
#1770=EDGE_LOOP('',(#7865,#7866,#7867,#7868));
#1771=EDGE_LOOP('',(#7869,#7870,#7871,#7872));
#1772=EDGE_LOOP('',(#7873,#7874,#7875,#7876));
#1773=EDGE_LOOP('',(#7877,#7878,#7879,#7880));
#1774=EDGE_LOOP('',(#7881,#7882,#7883,#7884));
#1775=EDGE_LOOP('',(#7885,#7886,#7887,#7888));
#1776=EDGE_LOOP('',(#7889,#7890,#7891,#7892));
#1777=EDGE_LOOP('',(#7893,#7894,#7895,#7896));
#1778=EDGE_LOOP('',(#7897,#7898,#7899,#7900));
#1779=EDGE_LOOP('',(#7901,#7902,#7903,#7904));
#1780=EDGE_LOOP('',(#7905,#7906,#7907,#7908));
#1781=EDGE_LOOP('',(#7909,#7910,#7911,#7912));
#1782=EDGE_LOOP('',(#7913,#7914,#7915,#7916));
#1783=EDGE_LOOP('',(#7917,#7918,#7919,#7920));
#1784=EDGE_LOOP('',(#7921,#7922,#7923,#7924));
#1785=EDGE_LOOP('',(#7925,#7926,#7927,#7928));
#1786=EDGE_LOOP('',(#7929,#7930,#7931,#7932));
#1787=EDGE_LOOP('',(#7933,#7934,#7935,#7936));
#1788=EDGE_LOOP('',(#7937,#7938,#7939,#7940));
#1789=EDGE_LOOP('',(#7941,#7942,#7943,#7944));
#1790=EDGE_LOOP('',(#7945,#7946,#7947,#7948));
#1791=EDGE_LOOP('',(#7949,#7950,#7951,#7952));
#1792=EDGE_LOOP('',(#7953,#7954,#7955,#7956));
#1793=EDGE_LOOP('',(#7957,#7958,#7959,#7960));
#1794=EDGE_LOOP('',(#7961,#7962,#7963,#7964));
#1795=EDGE_LOOP('',(#7965,#7966,#7967,#7968));
#1796=EDGE_LOOP('',(#7969,#7970,#7971));
#1797=EDGE_LOOP('',(#7972,#7973,#7974,#7975,#7976));
#1798=EDGE_LOOP('',(#7977,#7978,#7979,#7980));
#1799=EDGE_LOOP('',(#7981,#7982,#7983,#7984));
#1800=EDGE_LOOP('',(#7985,#7986,#7987,#7988));
#1801=EDGE_LOOP('',(#7989,#7990,#7991,#7992));
#1802=EDGE_LOOP('',(#7993,#7994,#7995,#7996));
#1803=EDGE_LOOP('',(#7997,#7998,#7999));
#1804=EDGE_LOOP('',(#8000,#8001,#8002,#8003,#8004));
#1805=EDGE_LOOP('',(#8005,#8006,#8007,#8008));
#1806=EDGE_LOOP('',(#8009,#8010,#8011,#8012));
#1807=EDGE_LOOP('',(#8013,#8014,#8015,#8016));
#1808=EDGE_LOOP('',(#8017,#8018,#8019,#8020));
#1809=EDGE_LOOP('',(#8021,#8022,#8023,#8024));
#1810=EDGE_LOOP('',(#8025,#8026,#8027));
#1811=EDGE_LOOP('',(#8028,#8029,#8030,#8031,#8032));
#1812=EDGE_LOOP('',(#8033,#8034,#8035,#8036));
#1813=EDGE_LOOP('',(#8037,#8038,#8039,#8040));
#1814=EDGE_LOOP('',(#8041,#8042,#8043,#8044));
#1815=EDGE_LOOP('',(#8045,#8046,#8047,#8048));
#1816=EDGE_LOOP('',(#8049,#8050,#8051,#8052));
#1817=EDGE_LOOP('',(#8053,#8054,#8055));
#1818=EDGE_LOOP('',(#8056,#8057,#8058,#8059,#8060));
#1819=EDGE_LOOP('',(#8061,#8062,#8063,#8064));
#1820=EDGE_LOOP('',(#8065,#8066,#8067,#8068));
#1821=EDGE_LOOP('',(#8069,#8070,#8071,#8072));
#1822=EDGE_LOOP('',(#8073,#8074,#8075,#8076));
#1823=EDGE_LOOP('',(#8077,#8078,#8079,#8080));
#1824=EDGE_LOOP('',(#8081,#8082,#8083,#8084));
#1825=EDGE_LOOP('',(#8085,#8086,#8087,#8088));
#1826=EDGE_LOOP('',(#8089,#8090,#8091,#8092));
#1827=EDGE_LOOP('',(#8093,#8094,#8095,#8096));
#1828=EDGE_LOOP('',(#8097,#8098,#8099,#8100));
#1829=EDGE_LOOP('',(#8101,#8102,#8103,#8104));
#1830=EDGE_LOOP('',(#8105,#8106,#8107,#8108));
#1831=EDGE_LOOP('',(#8109,#8110,#8111,#8112));
#1832=EDGE_LOOP('',(#8113,#8114,#8115,#8116));
#1833=EDGE_LOOP('',(#8117,#8118,#8119,#8120));
#1834=EDGE_LOOP('',(#8121,#8122,#8123,#8124));
#1835=EDGE_LOOP('',(#8125,#8126,#8127,#8128));
#1836=EDGE_LOOP('',(#8129,#8130,#8131,#8132,#8133,#8134,#8135,#8136));
#1837=EDGE_LOOP('',(#8137,#8138,#8139,#8140,#8141,#8142,#8143,#8144));
#1838=EDGE_LOOP('',(#8145,#8146,#8147,#8148,#8149,#8150,#8151,#8152));
#1839=EDGE_LOOP('',(#8153,#8154,#8155,#8156,#8157,#8158,#8159,#8160));
#1840=EDGE_LOOP('',(#8161,#8162,#8163,#8164,#8165,#8166,#8167,#8168,#8169,
#8170,#8171,#8172,#8173,#8174,#8175,#8176,#8177,#8178,#8179,#8180,#8181,
#8182,#8183,#8184,#8185,#8186,#8187,#8188,#8189,#8190,#8191,#8192));
#1841=EDGE_LOOP('',(#8193,#8194,#8195,#8196,#8197,#8198,#8199,#8200,#8201,
#8202,#8203,#8204,#8205,#8206,#8207,#8208,#8209,#8210,#8211,#8212,#8213,
#8214,#8215,#8216,#8217,#8218,#8219,#8220,#8221,#8222));
#1842=EDGE_LOOP('',(#8223,#8224,#8225,#8226));
#1843=EDGE_LOOP('',(#8227,#8228,#8229,#8230));
#1844=EDGE_LOOP('',(#8231,#8232,#8233,#8234,#8235,#8236,#8237,#8238));
#1845=EDGE_LOOP('',(#8239));
#1846=EDGE_LOOP('',(#8240,#8241,#8242,#8243,#8244));
#1847=EDGE_LOOP('',(#8245,#8246,#8247,#8248,#8249));
#1848=EDGE_LOOP('',(#8250,#8251,#8252,#8253,#8254));
#1849=EDGE_LOOP('',(#8255,#8256,#8257,#8258,#8259));
#1850=EDGE_LOOP('',(#8260,#8261,#8262,#8263,#8264,#8265,#8266,#8267,#8268,
#8269,#8270,#8271,#8272,#8273,#8274,#8275,#8276,#8277,#8278,#8279,#8280,
#8281,#8282,#8283,#8284,#8285,#8286,#8287,#8288,#8289,#8290,#8291));
#1851=EDGE_LOOP('',(#8292,#8293,#8294,#8295,#8296,#8297,#8298,#8299,#8300,
#8301,#8302,#8303,#8304,#8305,#8306,#8307,#8308,#8309,#8310,#8311,#8312,
#8313,#8314,#8315,#8316,#8317,#8318,#8319,#8320,#8321,#8322));
#1852=EDGE_LOOP('',(#8323,#8324,#8325,#8326));
#1853=EDGE_LOOP('',(#8327,#8328,#8329,#8330));
#1854=EDGE_LOOP('',(#8331,#8332,#8333,#8334,#8335,#8336,#8337,#8338,#8339,
#8340,#8341,#8342,#8343,#8344,#8345,#8346,#8347,#8348,#8349,#8350,#8351,
#8352,#8353,#8354,#8355,#8356,#8357,#8358,#8359,#8360,#8361,#8362,#8363));
#1855=EDGE_LOOP('',(#8364,#8365,#8366,#8367,#8368,#8369,#8370,#8371,#8372,
#8373,#8374,#8375,#8376,#8377,#8378,#8379,#8380,#8381,#8382,#8383,#8384,
#8385,#8386,#8387,#8388,#8389,#8390,#8391,#8392,#8393,#8394));
#1856=EDGE_LOOP('',(#8395,#8396,#8397,#8398));
#1857=EDGE_LOOP('',(#8399,#8400,#8401,#8402));
#1858=EDGE_LOOP('',(#8403,#8404,#8405,#8406,#8407,#8408,#8409,#8410,#8411,
#8412,#8413,#8414,#8415,#8416,#8417,#8418,#8419,#8420,#8421,#8422,#8423,
#8424,#8425,#8426,#8427,#8428,#8429,#8430,#8431,#8432,#8433,#8434,#8435));
#1859=EDGE_LOOP('',(#8436,#8437,#8438,#8439,#8440,#8441,#8442,#8443,#8444,
#8445,#8446,#8447,#8448,#8449,#8450,#8451,#8452,#8453,#8454,#8455,#8456,
#8457,#8458,#8459,#8460,#8461,#8462,#8463,#8464,#8465,#8466));
#1860=EDGE_LOOP('',(#8467,#8468,#8469,#8470));
#1861=EDGE_LOOP('',(#8471,#8472,#8473,#8474));
#1862=EDGE_LOOP('',(#8475));
#1863=EDGE_LOOP('',(#8476));
#1864=EDGE_LOOP('',(#8477));
#1865=EDGE_LOOP('',(#8478));
#1866=EDGE_LOOP('',(#8479,#8480,#8481,#8482));
#1867=EDGE_LOOP('',(#8483,#8484,#8485,#8486));
#1868=EDGE_LOOP('',(#8487,#8488,#8489,#8490));
#1869=EDGE_LOOP('',(#8491,#8492,#8493,#8494));
#1870=EDGE_LOOP('',(#8495,#8496,#8497,#8498));
#1871=EDGE_LOOP('',(#8499,#8500,#8501,#8502));
#1872=EDGE_LOOP('',(#8503,#8504,#8505,#8506));
#1873=EDGE_LOOP('',(#8507,#8508,#8509,#8510));
#1874=EDGE_LOOP('',(#8511,#8512,#8513,#8514));
#1875=EDGE_LOOP('',(#8515,#8516,#8517,#8518));
#1876=EDGE_LOOP('',(#8519,#8520,#8521,#8522));
#1877=EDGE_LOOP('',(#8523,#8524,#8525,#8526));
#1878=EDGE_LOOP('',(#8527,#8528,#8529,#8530));
#1879=EDGE_LOOP('',(#8531,#8532,#8533,#8534));
#1880=EDGE_LOOP('',(#8535,#8536,#8537,#8538));
#1881=EDGE_LOOP('',(#8539,#8540,#8541,#8542));
#1882=EDGE_LOOP('',(#8543,#8544,#8545,#8546,#8547,#8548,#8549,#8550));
#1883=EDGE_LOOP('',(#8551));
#1884=EDGE_LOOP('',(#8552));
#1885=EDGE_LOOP('',(#8553));
#1886=EDGE_LOOP('',(#8554));
#1887=EDGE_LOOP('',(#8555));
#1888=EDGE_LOOP('',(#8556,#8557,#8558,#8559));
#1889=EDGE_LOOP('',(#8560,#8561,#8562,#8563));
#1890=EDGE_LOOP('',(#8564,#8565,#8566));
#1891=EDGE_LOOP('',(#8567,#8568,#8569,#8570,#8571,#8572,#8573,#8574));
#1892=EDGE_LOOP('',(#8575,#8576));
#1893=EDGE_LOOP('',(#8577));
#1894=EDGE_LOOP('',(#8578));
#1895=EDGE_LOOP('',(#8579,#8580));
#1896=EDGE_LOOP('',(#8581,#8582,#8583,#8584,#8585));
#1897=EDGE_LOOP('',(#8586,#8587,#8588,#8589));
#1898=EDGE_LOOP('',(#8590,#8591,#8592,#8593));
#1899=EDGE_LOOP('',(#8594,#8595,#8596,#8597));
#1900=EDGE_LOOP('',(#8598,#8599,#8600,#8601));
#1901=EDGE_LOOP('',(#8602,#8603,#8604,#8605));
#1902=EDGE_LOOP('',(#8606,#8607,#8608,#8609));
#1903=EDGE_LOOP('',(#8610,#8611,#8612,#8613));
#1904=EDGE_LOOP('',(#8614,#8615,#8616,#8617));
#1905=EDGE_LOOP('',(#8618,#8619,#8620,#8621));
#1906=EDGE_LOOP('',(#8622,#8623,#8624,#8625));
#1907=EDGE_LOOP('',(#8626));
#1908=EDGE_LOOP('',(#8627));
#1909=EDGE_LOOP('',(#8628));
#1910=EDGE_LOOP('',(#8629));
#1911=EDGE_LOOP('',(#8630,#8631,#8632,#8633));
#1912=EDGE_LOOP('',(#8634,#8635,#8636,#8637));
#1913=EDGE_LOOP('',(#8638,#8639,#8640,#8641));
#1914=EDGE_LOOP('',(#8642,#8643,#8644,#8645));
#1915=EDGE_LOOP('',(#8646,#8647,#8648,#8649));
#1916=EDGE_LOOP('',(#8650,#8651,#8652,#8653));
#1917=EDGE_LOOP('',(#8654,#8655,#8656,#8657));
#1918=EDGE_LOOP('',(#8658,#8659,#8660,#8661));
#1919=EDGE_LOOP('',(#8662,#8663,#8664,#8665,#8666,#8667,#8668,#8669));
#1920=EDGE_LOOP('',(#8670));
#1921=EDGE_LOOP('',(#8671));
#1922=EDGE_LOOP('',(#8672));
#1923=EDGE_LOOP('',(#8673));
#1924=EDGE_LOOP('',(#8674));
#1925=EDGE_LOOP('',(#8675,#8676,#8677,#8678));
#1926=EDGE_LOOP('',(#8679,#8680,#8681,#8682));
#1927=EDGE_LOOP('',(#8683,#8684,#8685,#8686));
#1928=EDGE_LOOP('',(#8687,#8688,#8689,#8690));
#1929=EDGE_LOOP('',(#8691,#8692,#8693,#8694));
#1930=EDGE_LOOP('',(#8695,#8696,#8697,#8698));
#1931=EDGE_LOOP('',(#8699,#8700,#8701,#8702));
#1932=EDGE_LOOP('',(#8703,#8704,#8705,#8706));
#1933=EDGE_LOOP('',(#8707,#8708,#8709,#8710));
#1934=EDGE_LOOP('',(#8711,#8712,#8713,#8714));
#1935=EDGE_LOOP('',(#8715,#8716,#8717,#8718));
#1936=EDGE_LOOP('',(#8719,#8720,#8721,#8722));
#1937=EDGE_LOOP('',(#8723,#8724,#8725,#8726));
#1938=EDGE_LOOP('',(#8727,#8728,#8729,#8730,#8731));
#1939=EDGE_LOOP('',(#8732,#8733,#8734,#8735));
#1940=EDGE_LOOP('',(#8736,#8737,#8738,#8739,#8740));
#1941=EDGE_LOOP('',(#8741,#8742,#8743,#8744,#8745,#8746,#8747,#8748));
#1942=EDGE_LOOP('',(#8749,#8750,#8751,#8752));
#1943=EDGE_LOOP('',(#8753,#8754,#8755,#8756,#8757,#8758,#8759,#8760));
#1944=EDGE_LOOP('',(#8761,#8762,#8763,#8764,#8765,#8766,#8767,#8768));
#1945=EDGE_LOOP('',(#8769));
#1946=EDGE_LOOP('',(#8770));
#1947=EDGE_LOOP('',(#8771));
#1948=EDGE_LOOP('',(#8772,#8773,#8774,#8775));
#1949=EDGE_LOOP('',(#8776,#8777,#8778,#8779));
#1950=EDGE_LOOP('',(#8780,#8781,#8782,#8783));
#1951=EDGE_LOOP('',(#8784,#8785,#8786,#8787));
#1952=EDGE_LOOP('',(#8788,#8789,#8790,#8791));
#1953=EDGE_LOOP('',(#8792,#8793,#8794,#8795,#8796,#8797,#8798,#8799));
#1954=EDGE_LOOP('',(#8800));
#1955=EDGE_LOOP('',(#8801,#8802,#8803,#8804,#8805,#8806,#8807,#8808));
#1956=EDGE_LOOP('',(#8809));
#1957=EDGE_LOOP('',(#8810));
#1958=EDGE_LOOP('',(#8811));
#1959=EDGE_LOOP('',(#8812));
#1960=EDGE_LOOP('',(#8813));
#1961=EDGE_LOOP('',(#8814,#8815,#8816,#8817));
#1962=EDGE_LOOP('',(#8818,#8819,#8820,#8821));
#1963=EDGE_LOOP('',(#8822,#8823,#8824,#8825));
#1964=EDGE_LOOP('',(#8826,#8827,#8828,#8829));
#1965=EDGE_LOOP('',(#8830,#8831,#8832,#8833));
#1966=EDGE_LOOP('',(#8834,#8835,#8836,#8837));
#1967=EDGE_LOOP('',(#8838,#8839,#8840,#8841));
#1968=EDGE_LOOP('',(#8842,#8843,#8844,#8845));
#1969=EDGE_LOOP('',(#8846));
#1970=EDGE_LOOP('',(#8847));
#1971=EDGE_LOOP('',(#8848));
#1972=EDGE_LOOP('',(#8849));
#2388=LINE('',#15387,#3334);
#2389=LINE('',#15450,#3335);
#2390=LINE('',#15451,#3336);
#2391=LINE('',#15454,#3337);
#2392=LINE('',#15455,#3338);
#2393=LINE('',#15458,#3339);
#2394=LINE('',#15459,#3340);
#2395=LINE('',#15463,#3341);
#2396=LINE('',#15464,#3342);
#2397=LINE('',#15467,#3343);
#2398=LINE('',#15469,#3344);
#2399=LINE('',#15470,#3345);
#2400=LINE('',#15473,#3346);
#2401=LINE('',#15475,#3347);
#2402=LINE('',#15476,#3348);
#2403=LINE('',#15479,#3349);
#2404=LINE('',#15481,#3350);
#2405=LINE('',#15482,#3351);
#2406=LINE('',#15484,#3352);
#2407=LINE('',#15487,#3353);
#2408=LINE('',#15489,#3354);
#2409=LINE('',#15490,#3355);
#2410=LINE('',#15492,#3356);
#2411=LINE('',#15495,#3357);
#2412=LINE('',#15497,#3358);
#2413=LINE('',#15498,#3359);
#2414=LINE('',#15500,#3360);
#2415=LINE('',#15502,#3361);
#2416=LINE('',#15503,#3362);
#2417=LINE('',#15505,#3363);
#2418=LINE('',#15506,#3364);
#2419=LINE('',#15510,#3365);
#2420=LINE('',#15512,#3366);
#2421=LINE('',#15518,#3367);
#2422=LINE('',#15581,#3368);
#2423=LINE('',#15582,#3369);
#2424=LINE('',#15585,#3370);
#2425=LINE('',#15586,#3371);
#2426=LINE('',#15589,#3372);
#2427=LINE('',#15590,#3373);
#2428=LINE('',#15594,#3374);
#2429=LINE('',#15595,#3375);
#2430=LINE('',#15598,#3376);
#2431=LINE('',#15600,#3377);
#2432=LINE('',#15601,#3378);
#2433=LINE('',#15604,#3379);
#2434=LINE('',#15606,#3380);
#2435=LINE('',#15607,#3381);
#2436=LINE('',#15610,#3382);
#2437=LINE('',#15612,#3383);
#2438=LINE('',#15613,#3384);
#2439=LINE('',#15615,#3385);
#2440=LINE('',#15618,#3386);
#2441=LINE('',#15620,#3387);
#2442=LINE('',#15621,#3388);
#2443=LINE('',#15623,#3389);
#2444=LINE('',#15626,#3390);
#2445=LINE('',#15628,#3391);
#2446=LINE('',#15629,#3392);
#2447=LINE('',#15631,#3393);
#2448=LINE('',#15633,#3394);
#2449=LINE('',#15634,#3395);
#2450=LINE('',#15636,#3396);
#2451=LINE('',#15637,#3397);
#2452=LINE('',#15641,#3398);
#2453=LINE('',#15643,#3399);
#2454=LINE('',#15649,#3400);
#2455=LINE('',#15712,#3401);
#2456=LINE('',#15713,#3402);
#2457=LINE('',#15716,#3403);
#2458=LINE('',#15717,#3404);
#2459=LINE('',#15720,#3405);
#2460=LINE('',#15721,#3406);
#2461=LINE('',#15725,#3407);
#2462=LINE('',#15726,#3408);
#2463=LINE('',#15729,#3409);
#2464=LINE('',#15731,#3410);
#2465=LINE('',#15732,#3411);
#2466=LINE('',#15735,#3412);
#2467=LINE('',#15737,#3413);
#2468=LINE('',#15738,#3414);
#2469=LINE('',#15741,#3415);
#2470=LINE('',#15743,#3416);
#2471=LINE('',#15744,#3417);
#2472=LINE('',#15746,#3418);
#2473=LINE('',#15749,#3419);
#2474=LINE('',#15751,#3420);
#2475=LINE('',#15752,#3421);
#2476=LINE('',#15754,#3422);
#2477=LINE('',#15757,#3423);
#2478=LINE('',#15759,#3424);
#2479=LINE('',#15760,#3425);
#2480=LINE('',#15762,#3426);
#2481=LINE('',#15764,#3427);
#2482=LINE('',#15765,#3428);
#2483=LINE('',#15767,#3429);
#2484=LINE('',#15768,#3430);
#2485=LINE('',#15772,#3431);
#2486=LINE('',#15774,#3432);
#2487=LINE('',#15780,#3433);
#2488=LINE('',#15843,#3434);
#2489=LINE('',#15844,#3435);
#2490=LINE('',#15847,#3436);
#2491=LINE('',#15848,#3437);
#2492=LINE('',#15851,#3438);
#2493=LINE('',#15852,#3439);
#2494=LINE('',#15856,#3440);
#2495=LINE('',#15857,#3441);
#2496=LINE('',#15860,#3442);
#2497=LINE('',#15862,#3443);
#2498=LINE('',#15863,#3444);
#2499=LINE('',#15866,#3445);
#2500=LINE('',#15868,#3446);
#2501=LINE('',#15869,#3447);
#2502=LINE('',#15872,#3448);
#2503=LINE('',#15874,#3449);
#2504=LINE('',#15875,#3450);
#2505=LINE('',#15877,#3451);
#2506=LINE('',#15880,#3452);
#2507=LINE('',#15882,#3453);
#2508=LINE('',#15883,#3454);
#2509=LINE('',#15885,#3455);
#2510=LINE('',#15888,#3456);
#2511=LINE('',#15890,#3457);
#2512=LINE('',#15891,#3458);
#2513=LINE('',#15893,#3459);
#2514=LINE('',#15895,#3460);
#2515=LINE('',#15896,#3461);
#2516=LINE('',#15898,#3462);
#2517=LINE('',#15899,#3463);
#2518=LINE('',#15903,#3464);
#2519=LINE('',#15905,#3465);
#2520=LINE('',#15910,#3466);
#2521=LINE('',#15961,#3467);
#2522=LINE('',#16039,#3468);
#2523=LINE('',#16115,#3469);
#2524=LINE('',#16191,#3470);
#2525=LINE('',#16267,#3471);
#2526=LINE('',#16343,#3472);
#2527=LINE('',#16421,#3473);
#2528=LINE('',#16499,#3474);
#2529=LINE('',#16575,#3475);
#2530=LINE('',#16651,#3476);
#2531=LINE('',#16727,#3477);
#2532=LINE('',#16803,#3478);
#2533=LINE('',#16879,#3479);
#2534=LINE('',#16957,#3480);
#2535=LINE('',#17035,#3481);
#2536=LINE('',#17111,#3482);
#2537=LINE('',#17187,#3483);
#2538=LINE('',#17263,#3484);
#2539=LINE('',#17339,#3485);
#2540=LINE('',#17374,#3486);
#2541=LINE('',#17452,#3487);
#2542=LINE('',#17528,#3488);
#2543=LINE('',#17604,#3489);
#2544=LINE('',#17680,#3490);
#2545=LINE('',#17756,#3491);
#2546=LINE('',#17832,#3492);
#2547=LINE('',#17912,#3493);
#2548=LINE('',#17988,#3494);
#2549=LINE('',#18064,#3495);
#2550=LINE('',#18140,#3496);
#2551=LINE('',#18216,#3497);
#2552=LINE('',#18292,#3498);
#2553=LINE('',#18370,#3499);
#2554=LINE('',#18448,#3500);
#2555=LINE('',#18524,#3501);
#2556=LINE('',#18600,#3502);
#2557=LINE('',#18676,#3503);
#2558=LINE('',#18752,#3504);
#2559=LINE('',#18766,#3505);
#2560=LINE('',#18844,#3506);
#2561=LINE('',#18920,#3507);
#2562=LINE('',#18996,#3508);
#2563=LINE('',#19072,#3509);
#2564=LINE('',#19148,#3510);
#2565=LINE('',#19224,#3511);
#2566=LINE('',#19302,#3512);
#2567=LINE('',#19380,#3513);
#2568=LINE('',#19456,#3514);
#2569=LINE('',#19532,#3515);
#2570=LINE('',#19608,#3516);
#2571=LINE('',#19684,#3517);
#2572=LINE('',#19762,#3518);
#2573=LINE('',#19840,#3519);
#2574=LINE('',#19916,#3520);
#2575=LINE('',#19992,#3521);
#2576=LINE('',#20068,#3522);
#2577=LINE('',#20144,#3523);
#2578=LINE('',#20215,#3524);
#2579=LINE('',#20291,#3525);
#2580=LINE('',#20367,#3526);
#2581=LINE('',#20443,#3527);
#2582=LINE('',#20519,#3528);
#2583=LINE('',#20595,#3529);
#2584=LINE('',#20673,#3530);
#2585=LINE('',#20751,#3531);
#2586=LINE('',#20827,#3532);
#2587=LINE('',#20903,#3533);
#2588=LINE('',#20979,#3534);
#2589=LINE('',#21055,#3535);
#2590=LINE('',#21131,#3536);
#2591=LINE('',#21211,#3537);
#2592=LINE('',#21287,#3538);
#2593=LINE('',#21363,#3539);
#2594=LINE('',#21439,#3540);
#2595=LINE('',#21515,#3541);
#2596=LINE('',#21535,#3542);
#2597=LINE('',#21595,#3543);
#2598=LINE('',#21671,#3544);
#2599=LINE('',#21747,#3545);
#2600=LINE('',#21823,#3546);
#2601=LINE('',#21901,#3547);
#2602=LINE('',#21938,#3548);
#2603=LINE('',#21974,#3549);
#2604=LINE('',#21994,#3550);
#2605=LINE('',#22054,#3551);
#2606=LINE('',#22130,#3552);
#2607=LINE('',#22206,#3553);
#2608=LINE('',#22282,#3554);
#2609=LINE('',#22360,#3555);
#2610=LINE('',#22397,#3556);
#2611=LINE('',#22433,#3557);
#2612=LINE('',#22453,#3558);
#2613=LINE('',#22513,#3559);
#2614=LINE('',#22589,#3560);
#2615=LINE('',#22665,#3561);
#2616=LINE('',#22741,#3562);
#2617=LINE('',#22819,#3563);
#2618=LINE('',#22856,#3564);
#2619=LINE('',#22892,#3565);
#2620=LINE('',#22912,#3566);
#2621=LINE('',#22972,#3567);
#2622=LINE('',#23048,#3568);
#2623=LINE('',#23124,#3569);
#2624=LINE('',#23200,#3570);
#2625=LINE('',#23278,#3571);
#2626=LINE('',#23315,#3572);
#2627=LINE('',#23836,#3573);
#2628=LINE('',#23842,#3574);
#2629=LINE('',#23848,#3575);
#2630=LINE('',#23852,#3576);
#2631=LINE('',#23914,#3577);
#2632=LINE('',#23976,#3578);
#2633=LINE('',#24038,#3579);
#2634=LINE('',#24100,#3580);
#2635=LINE('',#25043,#3581);
#2636=LINE('',#25684,#3582);
#2637=LINE('',#25987,#3583);
#2638=LINE('',#26633,#3584);
#2639=LINE('',#26635,#3585);
#2640=LINE('',#26637,#3586);
#2641=LINE('',#26639,#3587);
#2642=LINE('',#26641,#3588);
#2643=LINE('',#26643,#3589);
#2644=LINE('',#26645,#3590);
#2645=LINE('',#26646,#3591);
#2646=LINE('',#27593,#3592);
#2647=LINE('',#28233,#3593);
#2648=LINE('',#28536,#3594);
#2649=LINE('',#30119,#3595);
#2650=LINE('',#30759,#3596);
#2651=LINE('',#31062,#3597);
#2652=LINE('',#32645,#3598);
#2653=LINE('',#33285,#3599);
#2654=LINE('',#33588,#3600);
#2655=LINE('',#34235,#3601);
#2656=LINE('',#34237,#3602);
#2657=LINE('',#34238,#3603);
#2658=LINE('',#34241,#3604);
#2659=LINE('',#34242,#3605);
#2660=LINE('',#34247,#3606);
#2661=LINE('',#34251,#3607);
#2662=LINE('',#34252,#3608);
#2663=LINE('',#34255,#3609);
#2664=LINE('',#34256,#3610);
#2665=LINE('',#34260,#3611);
#2666=LINE('',#34263,#3612);
#2667=LINE('',#34264,#3613);
#2668=LINE('',#34268,#3614);
#2669=LINE('',#34271,#3615);
#2670=LINE('',#34272,#3616);
#2671=LINE('',#34276,#3617);
#2672=LINE('',#34279,#3618);
#2673=LINE('',#34280,#3619);
#2674=LINE('',#34284,#3620);
#2675=LINE('',#34286,#3621);
#2676=LINE('',#34290,#3622);
#2677=LINE('',#34294,#3623);
#2678=LINE('',#34296,#3624);
#2679=LINE('',#34301,#3625);
#2680=LINE('',#34319,#3626);
#2681=LINE('',#34324,#3627);
#2682=LINE('',#34326,#3628);
#2683=LINE('',#34329,#3629);
#2684=LINE('',#34333,#3630);
#2685=LINE('',#34339,#3631);
#2686=LINE('',#34345,#3632);
#2687=LINE('',#34351,#3633);
#2688=LINE('',#34357,#3634);
#2689=LINE('',#34363,#3635);
#2690=LINE('',#34368,#3636);
#2691=LINE('',#34372,#3637);
#2692=LINE('',#34376,#3638);
#2693=LINE('',#34380,#3639);
#2694=LINE('',#34385,#3640);
#2695=LINE('',#34394,#3641);
#2696=LINE('',#34396,#3642);
#2697=LINE('',#34398,#3643);
#2698=LINE('',#34399,#3644);
#2699=LINE('',#34403,#3645);
#2700=LINE('',#34404,#3646);
#2701=LINE('',#34405,#3647);
#2702=LINE('',#34408,#3648);
#2703=LINE('',#34409,#3649);
#2704=LINE('',#34412,#3650);
#2705=LINE('',#34413,#3651);
#2706=LINE('',#34415,#3652);
#2707=LINE('',#34419,#3653);
#2708=LINE('',#34421,#3654);
#2709=LINE('',#34423,#3655);
#2710=LINE('',#34424,#3656);
#2711=LINE('',#34427,#3657);
#2712=LINE('',#34429,#3658);
#2713=LINE('',#34430,#3659);
#2714=LINE('',#34434,#3660);
#2715=LINE('',#34436,#3661);
#2716=LINE('',#34438,#3662);
#2717=LINE('',#34440,#3663);
#2718=LINE('',#34442,#3664);
#2719=LINE('',#34444,#3665);
#2720=LINE('',#34446,#3666);
#2721=LINE('',#34447,#3667);
#2722=LINE('',#34453,#3668);
#2723=LINE('',#34457,#3669);
#2724=LINE('',#34461,#3670);
#2725=LINE('',#34464,#3671);
#2726=LINE('',#34466,#3672);
#2727=LINE('',#34467,#3673);
#2728=LINE('',#34471,#3674);
#2729=LINE('',#34474,#3675);
#2730=LINE('',#34475,#3676);
#2731=LINE('',#34479,#3677);
#2732=LINE('',#34482,#3678);
#2733=LINE('',#34483,#3679);
#2734=LINE('',#34487,#3680);
#2735=LINE('',#34490,#3681);
#2736=LINE('',#34491,#3682);
#2737=LINE('',#34495,#3683);
#2738=LINE('',#34498,#3684);
#2739=LINE('',#34499,#3685);
#2740=LINE('',#34502,#3686);
#2741=LINE('',#34503,#3687);
#2742=LINE('',#34508,#3688);
#2743=LINE('',#34509,#3689);
#2744=LINE('',#34512,#3690);
#2745=LINE('',#34513,#3691);
#2746=LINE('',#34516,#3692);
#2747=LINE('',#34519,#3693);
#2748=LINE('',#34520,#3694);
#2749=LINE('',#34523,#3695);
#2750=LINE('',#34524,#3696);
#2751=LINE('',#34526,#3697);
#2752=LINE('',#34533,#3698);
#2753=LINE('',#34539,#3699);
#2754=LINE('',#34545,#3700);
#2755=LINE('',#34551,#3701);
#2756=LINE('',#34557,#3702);
#2757=LINE('',#34562,#3703);
#2758=LINE('',#34564,#3704);
#2759=LINE('',#34566,#3705);
#2760=LINE('',#34568,#3706);
#2761=LINE('',#34570,#3707);
#2762=LINE('',#34572,#3708);
#2763=LINE('',#34574,#3709);
#2764=LINE('',#34575,#3710);
#2765=LINE('',#34579,#3711);
#2766=LINE('',#34581,#3712);
#2767=LINE('',#34583,#3713);
#2768=LINE('',#34585,#3714);
#2769=LINE('',#34587,#3715);
#2770=LINE('',#34589,#3716);
#2771=LINE('',#34591,#3717);
#2772=LINE('',#34592,#3718);
#2773=LINE('',#34594,#3719);
#2774=LINE('',#34595,#3720);
#2775=LINE('',#34597,#3721);
#2776=LINE('',#34599,#3722);
#2777=LINE('',#34601,#3723);
#2778=LINE('',#34602,#3724);
#2779=LINE('',#34604,#3725);
#2780=LINE('',#34605,#3726);
#3334=VECTOR('',#12445,3.175);
#3335=VECTOR('',#12480,1000.);
#3336=VECTOR('',#12481,1000.);
#3337=VECTOR('',#12484,1000.);
#3338=VECTOR('',#12485,1000.);
#3339=VECTOR('',#12488,1000.);
#3340=VECTOR('',#12489,1000.);
#3341=VECTOR('',#12494,1000.);
#3342=VECTOR('',#12495,1000.);
#3343=VECTOR('',#12498,1000.);
#3344=VECTOR('',#12499,1000.);
#3345=VECTOR('',#12500,1000.);
#3346=VECTOR('',#12503,1000.);
#3347=VECTOR('',#12504,1000.);
#3348=VECTOR('',#12505,1000.);
#3349=VECTOR('',#12508,1000.);
#3350=VECTOR('',#12509,1000.);
#3351=VECTOR('',#12510,1000.);
#3352=VECTOR('',#12513,1000.);
#3353=VECTOR('',#12516,1000.);
#3354=VECTOR('',#12517,1000.);
#3355=VECTOR('',#12518,1000.);
#3356=VECTOR('',#12521,1000.);
#3357=VECTOR('',#12524,1000.);
#3358=VECTOR('',#12525,1000.);
#3359=VECTOR('',#12526,1000.);
#3360=VECTOR('',#12527,1000.);
#3361=VECTOR('',#12528,1000.);
#3362=VECTOR('',#12529,1000.);
#3363=VECTOR('',#12532,1000.);
#3364=VECTOR('',#12533,1000.);
#3365=VECTOR('',#12540,1000.);
#3366=VECTOR('',#12543,1000.);
#3367=VECTOR('',#12550,3.175);
#3368=VECTOR('',#12585,1000.);
#3369=VECTOR('',#12586,1000.);
#3370=VECTOR('',#12589,1000.);
#3371=VECTOR('',#12590,1000.);
#3372=VECTOR('',#12593,1000.);
#3373=VECTOR('',#12594,1000.);
#3374=VECTOR('',#12599,1000.);
#3375=VECTOR('',#12600,1000.);
#3376=VECTOR('',#12603,1000.);
#3377=VECTOR('',#12604,1000.);
#3378=VECTOR('',#12605,1000.);
#3379=VECTOR('',#12608,1000.);
#3380=VECTOR('',#12609,1000.);
#3381=VECTOR('',#12610,1000.);
#3382=VECTOR('',#12613,1000.);
#3383=VECTOR('',#12614,1000.);
#3384=VECTOR('',#12615,1000.);
#3385=VECTOR('',#12618,1000.);
#3386=VECTOR('',#12621,1000.);
#3387=VECTOR('',#12622,1000.);
#3388=VECTOR('',#12623,1000.);
#3389=VECTOR('',#12626,1000.);
#3390=VECTOR('',#12629,1000.);
#3391=VECTOR('',#12630,1000.);
#3392=VECTOR('',#12631,1000.);
#3393=VECTOR('',#12632,1000.);
#3394=VECTOR('',#12633,1000.);
#3395=VECTOR('',#12634,1000.);
#3396=VECTOR('',#12637,1000.);
#3397=VECTOR('',#12638,1000.);
#3398=VECTOR('',#12645,1000.);
#3399=VECTOR('',#12648,1000.);
#3400=VECTOR('',#12655,3.175);
#3401=VECTOR('',#12690,1000.);
#3402=VECTOR('',#12691,1000.);
#3403=VECTOR('',#12694,1000.);
#3404=VECTOR('',#12695,1000.);
#3405=VECTOR('',#12698,1000.);
#3406=VECTOR('',#12699,1000.);
#3407=VECTOR('',#12704,1000.);
#3408=VECTOR('',#12705,1000.);
#3409=VECTOR('',#12708,1000.);
#3410=VECTOR('',#12709,1000.);
#3411=VECTOR('',#12710,1000.);
#3412=VECTOR('',#12713,1000.);
#3413=VECTOR('',#12714,1000.);
#3414=VECTOR('',#12715,1000.);
#3415=VECTOR('',#12718,1000.);
#3416=VECTOR('',#12719,1000.);
#3417=VECTOR('',#12720,1000.);
#3418=VECTOR('',#12723,1000.);
#3419=VECTOR('',#12726,1000.);
#3420=VECTOR('',#12727,1000.);
#3421=VECTOR('',#12728,1000.);
#3422=VECTOR('',#12731,1000.);
#3423=VECTOR('',#12734,1000.);
#3424=VECTOR('',#12735,1000.);
#3425=VECTOR('',#12736,1000.);
#3426=VECTOR('',#12737,1000.);
#3427=VECTOR('',#12738,1000.);
#3428=VECTOR('',#12739,1000.);
#3429=VECTOR('',#12742,1000.);
#3430=VECTOR('',#12743,1000.);
#3431=VECTOR('',#12750,1000.);
#3432=VECTOR('',#12753,1000.);
#3433=VECTOR('',#12760,3.175);
#3434=VECTOR('',#12795,1000.);
#3435=VECTOR('',#12796,1000.);
#3436=VECTOR('',#12799,1000.);
#3437=VECTOR('',#12800,1000.);
#3438=VECTOR('',#12803,1000.);
#3439=VECTOR('',#12804,1000.);
#3440=VECTOR('',#12809,1000.);
#3441=VECTOR('',#12810,1000.);
#3442=VECTOR('',#12813,1000.);
#3443=VECTOR('',#12814,1000.);
#3444=VECTOR('',#12815,1000.);
#3445=VECTOR('',#12818,1000.);
#3446=VECTOR('',#12819,1000.);
#3447=VECTOR('',#12820,1000.);
#3448=VECTOR('',#12823,1000.);
#3449=VECTOR('',#12824,1000.);
#3450=VECTOR('',#12825,1000.);
#3451=VECTOR('',#12828,1000.);
#3452=VECTOR('',#12831,1000.);
#3453=VECTOR('',#12832,1000.);
#3454=VECTOR('',#12833,1000.);
#3455=VECTOR('',#12836,1000.);
#3456=VECTOR('',#12839,1000.);
#3457=VECTOR('',#12840,1000.);
#3458=VECTOR('',#12841,1000.);
#3459=VECTOR('',#12842,1000.);
#3460=VECTOR('',#12843,1000.);
#3461=VECTOR('',#12844,1000.);
#3462=VECTOR('',#12847,1000.);
#3463=VECTOR('',#12848,1000.);
#3464=VECTOR('',#12855,1000.);
#3465=VECTOR('',#12858,1000.);
#3466=VECTOR('',#12863,1.905);
#3467=VECTOR('',#12868,1.905);
#3468=VECTOR('',#12871,1.905);
#3469=VECTOR('',#12874,1.905);
#3470=VECTOR('',#12877,1.905);
#3471=VECTOR('',#12880,1.905);
#3472=VECTOR('',#12883,1.905);
#3473=VECTOR('',#12886,1.905);
#3474=VECTOR('',#12889,1.905);
#3475=VECTOR('',#12892,1.905);
#3476=VECTOR('',#12895,1.905);
#3477=VECTOR('',#12898,1.905);
#3478=VECTOR('',#12901,1.905);
#3479=VECTOR('',#12904,1.905);
#3480=VECTOR('',#12907,1.905);
#3481=VECTOR('',#12910,1.905);
#3482=VECTOR('',#12913,1.905);
#3483=VECTOR('',#12916,1.905);
#3484=VECTOR('',#12919,1.905);
#3485=VECTOR('',#12922,1.905);
#3486=VECTOR('',#12927,1.905);
#3487=VECTOR('',#12930,1.905);
#3488=VECTOR('',#12933,1.905);
#3489=VECTOR('',#12936,1.905);
#3490=VECTOR('',#12939,1.905);
#3491=VECTOR('',#12942,1.905);
#3492=VECTOR('',#12945,1.905);
#3493=VECTOR('',#12948,1.905);
#3494=VECTOR('',#12951,1.905);
#3495=VECTOR('',#12954,1.905);
#3496=VECTOR('',#12957,1.905);
#3497=VECTOR('',#12960,1.905);
#3498=VECTOR('',#12963,1.905);
#3499=VECTOR('',#12966,1.905);
#3500=VECTOR('',#12969,1.905);
#3501=VECTOR('',#12972,1.905);
#3502=VECTOR('',#12975,1.905);
#3503=VECTOR('',#12978,1.905);
#3504=VECTOR('',#12981,1.905);
#3505=VECTOR('',#12986,1.905);
#3506=VECTOR('',#12989,1.905);
#3507=VECTOR('',#12992,1.905);
#3508=VECTOR('',#12995,1.905);
#3509=VECTOR('',#12998,1.905);
#3510=VECTOR('',#13001,1.905);
#3511=VECTOR('',#13004,1.905);
#3512=VECTOR('',#13007,1.905);
#3513=VECTOR('',#13010,1.905);
#3514=VECTOR('',#13013,1.905);
#3515=VECTOR('',#13016,1.905);
#3516=VECTOR('',#13019,1.905);
#3517=VECTOR('',#13022,1.905);
#3518=VECTOR('',#13025,1.905);
#3519=VECTOR('',#13028,1.905);
#3520=VECTOR('',#13031,1.905);
#3521=VECTOR('',#13034,1.905);
#3522=VECTOR('',#13037,1.905);
#3523=VECTOR('',#13040,1.905);
#3524=VECTOR('',#13045,1.905);
#3525=VECTOR('',#13048,1.905);
#3526=VECTOR('',#13051,1.905);
#3527=VECTOR('',#13054,1.905);
#3528=VECTOR('',#13057,1.905);
#3529=VECTOR('',#13060,1.905);
#3530=VECTOR('',#13063,1.905);
#3531=VECTOR('',#13066,1.905);
#3532=VECTOR('',#13069,1.905);
#3533=VECTOR('',#13072,1.905);
#3534=VECTOR('',#13075,1.905);
#3535=VECTOR('',#13078,1.905);
#3536=VECTOR('',#13081,1.905);
#3537=VECTOR('',#13084,1.905);
#3538=VECTOR('',#13087,1.905);
#3539=VECTOR('',#13090,1.905);
#3540=VECTOR('',#13093,1.905);
#3541=VECTOR('',#13096,1.93206329386826);
#3542=VECTOR('',#13101,1.93206329386826);
#3543=VECTOR('',#13106,1.93206329386826);
#3544=VECTOR('',#13109,1.93206329386826);
#3545=VECTOR('',#13112,1.93206329386826);
#3546=VECTOR('',#13115,1.93206329386826);
#3547=VECTOR('',#13118,1.93206329386826);
#3548=VECTOR('',#13119,10.);
#3549=VECTOR('',#13122,1.93206329386825);
#3550=VECTOR('',#13127,1.93206329386825);
#3551=VECTOR('',#13132,1.93206329386825);
#3552=VECTOR('',#13135,1.93206329386825);
#3553=VECTOR('',#13138,1.93206329386825);
#3554=VECTOR('',#13141,1.93206329386825);
#3555=VECTOR('',#13144,1.93206329386825);
#3556=VECTOR('',#13145,10.);
#3557=VECTOR('',#13148,1.93206329386826);
#3558=VECTOR('',#13153,1.93206329386826);
#3559=VECTOR('',#13158,1.93206329386826);
#3560=VECTOR('',#13161,1.93206329386826);
#3561=VECTOR('',#13164,1.93206329386826);
#3562=VECTOR('',#13167,1.93206329386826);
#3563=VECTOR('',#13170,1.93206329386826);
#3564=VECTOR('',#13171,10.);
#3565=VECTOR('',#13174,1.93206329386822);
#3566=VECTOR('',#13179,1.93206329386822);
#3567=VECTOR('',#13184,1.93206329386822);
#3568=VECTOR('',#13187,1.93206329386822);
#3569=VECTOR('',#13190,1.93206329386822);
#3570=VECTOR('',#13193,1.93206329386822);
#3571=VECTOR('',#13196,1.93206329386822);
#3572=VECTOR('',#13197,10.);
#3573=VECTOR('',#13226,2.62699999999999);
#3574=VECTOR('',#13233,3.76999999999999);
#3575=VECTOR('',#13240,10.985);
#3576=VECTOR('',#13245,10.985);
#3577=VECTOR('',#13252,2.155);
#3578=VECTOR('',#13259,2.155);
#3579=VECTOR('',#13266,2.155);
#3580=VECTOR('',#13273,2.155);
#3581=VECTOR('',#13278,10.);
#3582=VECTOR('',#13281,10.);
#3583=VECTOR('',#13284,10.);
#3584=VECTOR('',#13287,1000.);
#3585=VECTOR('',#13288,1000.);
#3586=VECTOR('',#13289,1000.);
#3587=VECTOR('',#13290,1000.);
#3588=VECTOR('',#13291,1000.);
#3589=VECTOR('',#13292,1000.);
#3590=VECTOR('',#13293,1000.);
#3591=VECTOR('',#13294,1000.);
#3592=VECTOR('',#13307,9.99999999999999);
#3593=VECTOR('',#13308,10.);
#3594=VECTOR('',#13311,10.);
#3595=VECTOR('',#13312,10.);
#3596=VECTOR('',#13313,10.);
#3597=VECTOR('',#13316,10.);
#3598=VECTOR('',#13317,9.99999999999999);
#3599=VECTOR('',#13318,10.);
#3600=VECTOR('',#13321,10.);
#3601=VECTOR('',#13328,1000.);
#3602=VECTOR('',#13329,1000.);
#3603=VECTOR('',#13330,1000.);
#3604=VECTOR('',#13333,1000.);
#3605=VECTOR('',#13334,1000.);
#3606=VECTOR('',#13339,1000.);
#3607=VECTOR('',#13344,1000.);
#3608=VECTOR('',#13345,1000.);
#3609=VECTOR('',#13348,1000.);
#3610=VECTOR('',#13349,1000.);
#3611=VECTOR('',#13354,1000.);
#3612=VECTOR('',#13357,1000.);
#3613=VECTOR('',#13358,1000.);
#3614=VECTOR('',#13363,1000.);
#3615=VECTOR('',#13366,1000.);
#3616=VECTOR('',#13367,1000.);
#3617=VECTOR('',#13372,1000.);
#3618=VECTOR('',#13375,1000.);
#3619=VECTOR('',#13376,1000.);
#3620=VECTOR('',#13381,1000.);
#3621=VECTOR('',#13384,1000.);
#3622=VECTOR('',#13389,1000.);
#3623=VECTOR('',#13394,1000.);
#3624=VECTOR('',#13397,1000.);
#3625=VECTOR('',#13402,1.99200000000004);
#3626=VECTOR('',#13415,0.975999999999995);
#3627=VECTOR('',#13422,2.5);
#3628=VECTOR('',#13423,1000.);
#3629=VECTOR('',#13426,1000.);
#3630=VECTOR('',#13433,1000.);
#3631=VECTOR('',#13440,5.16699999999999);
#3632=VECTOR('',#13447,3.175);
#3633=VECTOR('',#13454,3.175);
#3634=VECTOR('',#13461,3.175);
#3635=VECTOR('',#13468,3.175);
#3636=VECTOR('',#13475,3.175);
#3637=VECTOR('',#13480,3.175);
#3638=VECTOR('',#13485,3.175);
#3639=VECTOR('',#13490,3.175);
#3640=VECTOR('',#13495,2.62699999999999);
#3641=VECTOR('',#13508,1000.);
#3642=VECTOR('',#13509,1000.);
#3643=VECTOR('',#13510,1000.);
#3644=VECTOR('',#13511,1000.);
#3645=VECTOR('',#13514,1000.);
#3646=VECTOR('',#13515,1000.);
#3647=VECTOR('',#13516,1000.);
#3648=VECTOR('',#13519,1000.);
#3649=VECTOR('',#13520,1000.);
#3650=VECTOR('',#13523,1000.);
#3651=VECTOR('',#13524,1000.);
#3652=VECTOR('',#13527,1000.);
#3653=VECTOR('',#13530,1000.);
#3654=VECTOR('',#13531,1000.);
#3655=VECTOR('',#13532,1000.);
#3656=VECTOR('',#13533,1000.);
#3657=VECTOR('',#13536,1000.);
#3658=VECTOR('',#13537,1000.);
#3659=VECTOR('',#13538,1000.);
#3660=VECTOR('',#13541,1000.);
#3661=VECTOR('',#13542,1000.);
#3662=VECTOR('',#13543,1000.);
#3663=VECTOR('',#13544,1000.);
#3664=VECTOR('',#13545,1000.);
#3665=VECTOR('',#13546,1000.);
#3666=VECTOR('',#13547,1000.);
#3667=VECTOR('',#13548,1000.);
#3668=VECTOR('',#13555,1000.);
#3669=VECTOR('',#13560,1000.);
#3670=VECTOR('',#13565,1000.);
#3671=VECTOR('',#13568,1000.);
#3672=VECTOR('',#13569,1000.);
#3673=VECTOR('',#13570,1000.);
#3674=VECTOR('',#13575,1000.);
#3675=VECTOR('',#13578,1000.);
#3676=VECTOR('',#13579,1000.);
#3677=VECTOR('',#13584,1000.);
#3678=VECTOR('',#13587,1000.);
#3679=VECTOR('',#13588,1000.);
#3680=VECTOR('',#13593,1000.);
#3681=VECTOR('',#13596,1000.);
#3682=VECTOR('',#13597,1000.);
#3683=VECTOR('',#13602,1000.);
#3684=VECTOR('',#13605,1000.);
#3685=VECTOR('',#13606,1000.);
#3686=VECTOR('',#13609,1000.);
#3687=VECTOR('',#13610,1000.);
#3688=VECTOR('',#13615,1000.);
#3689=VECTOR('',#13616,1000.);
#3690=VECTOR('',#13619,1000.);
#3691=VECTOR('',#13620,1000.);
#3692=VECTOR('',#13623,1000.);
#3693=VECTOR('',#13628,1000.);
#3694=VECTOR('',#13629,1000.);
#3695=VECTOR('',#13632,1000.);
#3696=VECTOR('',#13633,1000.);
#3697=VECTOR('',#13636,1000.);
#3698=VECTOR('',#13645,2.62699999999999);
#3699=VECTOR('',#13652,1.905);
#3700=VECTOR('',#13659,1.905);
#3701=VECTOR('',#13666,1.905);
#3702=VECTOR('',#13673,1.905);
#3703=VECTOR('',#13678,1000.);
#3704=VECTOR('',#13679,1000.);
#3705=VECTOR('',#13680,1000.);
#3706=VECTOR('',#13681,1000.);
#3707=VECTOR('',#13682,1000.);
#3708=VECTOR('',#13683,1000.);
#3709=VECTOR('',#13684,1000.);
#3710=VECTOR('',#13685,1000.);
#3711=VECTOR('',#13688,1000.);
#3712=VECTOR('',#13689,1000.);
#3713=VECTOR('',#13690,1000.);
#3714=VECTOR('',#13691,1000.);
#3715=VECTOR('',#13692,1000.);
#3716=VECTOR('',#13693,1000.);
#3717=VECTOR('',#13694,1000.);
#3718=VECTOR('',#13695,1000.);
#3719=VECTOR('',#13698,1000.);
#3720=VECTOR('',#13699,1000.);
#3721=VECTOR('',#13702,1000.);
#3722=VECTOR('',#13705,1000.);
#3723=VECTOR('',#13708,1000.);
#3724=VECTOR('',#13709,1000.);
#3725=VECTOR('',#13712,1000.);
#3726=VECTOR('',#13713,1000.);
#4280=CIRCLE('',#11441,3.175);
#4281=CIRCLE('',#11442,3.175);
#4282=CIRCLE('',#11443,3.175);
#4283=CIRCLE('',#11445,1.27);
#4284=CIRCLE('',#11447,1.905);
#4285=CIRCLE('',#11450,1.905);
#4286=CIRCLE('',#11453,1.905);
#4287=CIRCLE('',#11456,1.905);
#4288=CIRCLE('',#11477,3.175);
#4289=CIRCLE('',#11478,3.175);
#4290=CIRCLE('',#11479,3.175);
#4291=CIRCLE('',#11481,1.27);
#4292=CIRCLE('',#11483,1.905);
#4293=CIRCLE('',#11486,1.905);
#4294=CIRCLE('',#11489,1.905);
#4295=CIRCLE('',#11492,1.905);
#4296=CIRCLE('',#11513,3.175);
#4297=CIRCLE('',#11514,3.175);
#4298=CIRCLE('',#11515,3.175);
#4299=CIRCLE('',#11517,1.27);
#4300=CIRCLE('',#11519,1.905);
#4301=CIRCLE('',#11522,1.905);
#4302=CIRCLE('',#11525,1.905);
#4303=CIRCLE('',#11528,1.905);
#4304=CIRCLE('',#11549,3.175);
#4305=CIRCLE('',#11550,3.175);
#4306=CIRCLE('',#11551,3.175);
#4307=CIRCLE('',#11553,1.27);
#4308=CIRCLE('',#11555,1.905);
#4309=CIRCLE('',#11558,1.905);
#4310=CIRCLE('',#11561,1.905);
#4311=CIRCLE('',#11564,1.905);
#4312=CIRCLE('',#11585,1.905);
#4313=CIRCLE('',#11605,1.905);
#4314=CIRCLE('',#11625,1.905);
#4315=CIRCLE('',#11645,1.905);
#4316=CIRCLE('',#11664,1.93206329386826);
#4317=CIRCLE('',#11666,1.93206329386826);
#4318=CIRCLE('',#11673,1.93206329386825);
#4319=CIRCLE('',#11675,1.93206329386825);
#4320=CIRCLE('',#11682,1.93206329386826);
#4321=CIRCLE('',#11684,1.93206329386826);
#4322=CIRCLE('',#11691,1.93206329386822);
#4323=CIRCLE('',#11693,1.93206329386822);
#4324=CIRCLE('',#11704,1.905);
#4325=CIRCLE('',#11706,1.905);
#4326=CIRCLE('',#11708,1.905);
#4327=CIRCLE('',#11710,1.905);
#4328=CIRCLE('',#11712,2.62699999999999);
#4329=CIRCLE('',#11713,2.62699999999999);
#4330=CIRCLE('',#11715,3.76999999999999);
#4331=CIRCLE('',#11716,3.76999999999999);
#4332=CIRCLE('',#11718,11.493);
#4333=CIRCLE('',#11719,10.985);
#4334=CIRCLE('',#11721,10.985);
#4335=CIRCLE('',#11723,1.58024047358085);
#4336=CIRCLE('',#11724,2.155);
#4337=CIRCLE('',#11726,1.58024047358083);
#4338=CIRCLE('',#11727,2.155);
#4339=CIRCLE('',#11729,1.58024047358085);
#4340=CIRCLE('',#11730,2.155);
#4341=CIRCLE('',#11732,1.58024047358083);
#4342=CIRCLE('',#11733,2.155);
#4343=CIRCLE('',#11734,1.86136507718219);
#4344=CIRCLE('',#11735,1.90494743284919);
#4345=CIRCLE('',#11738,1.86136507718315);
#4346=CIRCLE('',#11739,1.9049474328492);
#4347=CIRCLE('',#11740,1.86136507718391);
#4348=CIRCLE('',#11741,1.90494743284917);
#4349=CIRCLE('',#11742,1.86136507718316);
#4350=CIRCLE('',#11743,1.90494743284856);
#4351=CIRCLE('',#11775,2.5);
#4352=CIRCLE('',#11776,1.99200000000004);
#4353=CIRCLE('',#11778,1.99200000000004);
#4354=CIRCLE('',#11779,2.5);
#4355=CIRCLE('',#11781,0.975999999999995);
#4356=CIRCLE('',#11783,2.5);
#4357=CIRCLE('',#11784,2.5);
#4358=CIRCLE('',#11790,5.16699999999999);
#4359=CIRCLE('',#11791,5.16699999999999);
#4360=CIRCLE('',#11793,3.175);
#4361=CIRCLE('',#11794,3.429);
#4362=CIRCLE('',#11796,3.175);
#4363=CIRCLE('',#11797,3.429);
#4364=CIRCLE('',#11799,3.175);
#4365=CIRCLE('',#11800,3.429);
#4366=CIRCLE('',#11802,3.175);
#4367=CIRCLE('',#11803,3.429);
#4368=CIRCLE('',#11805,3.175);
#4369=CIRCLE('',#11807,3.175);
#4370=CIRCLE('',#11809,3.175);
#4371=CIRCLE('',#11811,3.175);
#4372=CIRCLE('',#11813,2.62699999999999);
#4373=CIRCLE('',#11814,2.62699999999999);
#4374=CIRCLE('',#11849,0.761999999999999);
#4375=CIRCLE('',#11852,0.761999999999999);
#4376=CIRCLE('',#11859,2.62699999999999);
#4377=CIRCLE('',#11860,2.62699999999999);
#4378=CIRCLE('',#11862,1.905);
#4379=CIRCLE('',#11863,1.905);
#4380=CIRCLE('',#11865,1.905);
#4381=CIRCLE('',#11866,1.905);
#4382=CIRCLE('',#11868,1.905);
#4383=CIRCLE('',#11869,1.905);
#4384=CIRCLE('',#11871,1.905);
#4385=CIRCLE('',#11872,1.905);
#4593=VERTEX_POINT('',#15384);
#4594=VERTEX_POINT('',#15386);
#4595=VERTEX_POINT('',#15388);
#4596=VERTEX_POINT('',#15392);
#4597=VERTEX_POINT('',#15393);
#4598=VERTEX_POINT('',#15399);
#4599=VERTEX_POINT('',#15404);
#4600=VERTEX_POINT('',#15406);
#4601=VERTEX_POINT('',#15408);
#4602=VERTEX_POINT('',#15410);
#4603=VERTEX_POINT('',#15417);
#4604=VERTEX_POINT('',#15419);
#4605=VERTEX_POINT('',#15421);
#4606=VERTEX_POINT('',#15423);
#4607=VERTEX_POINT('',#15430);
#4608=VERTEX_POINT('',#15432);
#4609=VERTEX_POINT('',#15434);
#4610=VERTEX_POINT('',#15436);
#4611=VERTEX_POINT('',#15443);
#4612=VERTEX_POINT('',#15445);
#4613=VERTEX_POINT('',#15449);
#4614=VERTEX_POINT('',#15453);
#4615=VERTEX_POINT('',#15457);
#4616=VERTEX_POINT('',#15462);
#4617=VERTEX_POINT('',#15466);
#4618=VERTEX_POINT('',#15468);
#4619=VERTEX_POINT('',#15472);
#4620=VERTEX_POINT('',#15474);
#4621=VERTEX_POINT('',#15478);
#4622=VERTEX_POINT('',#15480);
#4623=VERTEX_POINT('',#15486);
#4624=VERTEX_POINT('',#15488);
#4625=VERTEX_POINT('',#15494);
#4626=VERTEX_POINT('',#15496);
#4627=VERTEX_POINT('',#15499);
#4628=VERTEX_POINT('',#15501);
#4629=VERTEX_POINT('',#15515);
#4630=VERTEX_POINT('',#15517);
#4631=VERTEX_POINT('',#15519);
#4632=VERTEX_POINT('',#15523);
#4633=VERTEX_POINT('',#15524);
#4634=VERTEX_POINT('',#15530);
#4635=VERTEX_POINT('',#15535);
#4636=VERTEX_POINT('',#15537);
#4637=VERTEX_POINT('',#15539);
#4638=VERTEX_POINT('',#15541);
#4639=VERTEX_POINT('',#15548);
#4640=VERTEX_POINT('',#15550);
#4641=VERTEX_POINT('',#15552);
#4642=VERTEX_POINT('',#15554);
#4643=VERTEX_POINT('',#15561);
#4644=VERTEX_POINT('',#15563);
#4645=VERTEX_POINT('',#15565);
#4646=VERTEX_POINT('',#15567);
#4647=VERTEX_POINT('',#15574);
#4648=VERTEX_POINT('',#15576);
#4649=VERTEX_POINT('',#15580);
#4650=VERTEX_POINT('',#15584);
#4651=VERTEX_POINT('',#15588);
#4652=VERTEX_POINT('',#15593);
#4653=VERTEX_POINT('',#15597);
#4654=VERTEX_POINT('',#15599);
#4655=VERTEX_POINT('',#15603);
#4656=VERTEX_POINT('',#15605);
#4657=VERTEX_POINT('',#15609);
#4658=VERTEX_POINT('',#15611);
#4659=VERTEX_POINT('',#15617);
#4660=VERTEX_POINT('',#15619);
#4661=VERTEX_POINT('',#15625);
#4662=VERTEX_POINT('',#15627);
#4663=VERTEX_POINT('',#15630);
#4664=VERTEX_POINT('',#15632);
#4665=VERTEX_POINT('',#15646);
#4666=VERTEX_POINT('',#15648);
#4667=VERTEX_POINT('',#15650);
#4668=VERTEX_POINT('',#15654);
#4669=VERTEX_POINT('',#15655);
#4670=VERTEX_POINT('',#15661);
#4671=VERTEX_POINT('',#15666);
#4672=VERTEX_POINT('',#15668);
#4673=VERTEX_POINT('',#15670);
#4674=VERTEX_POINT('',#15672);
#4675=VERTEX_POINT('',#15679);
#4676=VERTEX_POINT('',#15681);
#4677=VERTEX_POINT('',#15683);
#4678=VERTEX_POINT('',#15685);
#4679=VERTEX_POINT('',#15692);
#4680=VERTEX_POINT('',#15694);
#4681=VERTEX_POINT('',#15696);
#4682=VERTEX_POINT('',#15698);
#4683=VERTEX_POINT('',#15705);
#4684=VERTEX_POINT('',#15707);
#4685=VERTEX_POINT('',#15711);
#4686=VERTEX_POINT('',#15715);
#4687=VERTEX_POINT('',#15719);
#4688=VERTEX_POINT('',#15724);
#4689=VERTEX_POINT('',#15728);
#4690=VERTEX_POINT('',#15730);
#4691=VERTEX_POINT('',#15734);
#4692=VERTEX_POINT('',#15736);
#4693=VERTEX_POINT('',#15740);
#4694=VERTEX_POINT('',#15742);
#4695=VERTEX_POINT('',#15748);
#4696=VERTEX_POINT('',#15750);
#4697=VERTEX_POINT('',#15756);
#4698=VERTEX_POINT('',#15758);
#4699=VERTEX_POINT('',#15761);
#4700=VERTEX_POINT('',#15763);
#4701=VERTEX_POINT('',#15777);
#4702=VERTEX_POINT('',#15779);
#4703=VERTEX_POINT('',#15781);
#4704=VERTEX_POINT('',#15785);
#4705=VERTEX_POINT('',#15786);
#4706=VERTEX_POINT('',#15792);
#4707=VERTEX_POINT('',#15797);
#4708=VERTEX_POINT('',#15799);
#4709=VERTEX_POINT('',#15801);
#4710=VERTEX_POINT('',#15803);
#4711=VERTEX_POINT('',#15810);
#4712=VERTEX_POINT('',#15812);
#4713=VERTEX_POINT('',#15814);
#4714=VERTEX_POINT('',#15816);
#4715=VERTEX_POINT('',#15823);
#4716=VERTEX_POINT('',#15825);
#4717=VERTEX_POINT('',#15827);
#4718=VERTEX_POINT('',#15829);
#4719=VERTEX_POINT('',#15836);
#4720=VERTEX_POINT('',#15838);
#4721=VERTEX_POINT('',#15842);
#4722=VERTEX_POINT('',#15846);
#4723=VERTEX_POINT('',#15850);
#4724=VERTEX_POINT('',#15855);
#4725=VERTEX_POINT('',#15859);
#4726=VERTEX_POINT('',#15861);
#4727=VERTEX_POINT('',#15865);
#4728=VERTEX_POINT('',#15867);
#4729=VERTEX_POINT('',#15871);
#4730=VERTEX_POINT('',#15873);
#4731=VERTEX_POINT('',#15879);
#4732=VERTEX_POINT('',#15881);
#4733=VERTEX_POINT('',#15887);
#4734=VERTEX_POINT('',#15889);
#4735=VERTEX_POINT('',#15892);
#4736=VERTEX_POINT('',#15894);
#4737=VERTEX_POINT('',#15908);
#4738=VERTEX_POINT('',#15909);
#4739=VERTEX_POINT('',#15911);
#4740=VERTEX_POINT('',#15936);
#4741=VERTEX_POINT('',#15959);
#4742=VERTEX_POINT('',#15960);
#4743=VERTEX_POINT('',#16037);
#4744=VERTEX_POINT('',#16038);
#4745=VERTEX_POINT('',#16113);
#4746=VERTEX_POINT('',#16114);
#4747=VERTEX_POINT('',#16189);
#4748=VERTEX_POINT('',#16190);
#4749=VERTEX_POINT('',#16265);
#4750=VERTEX_POINT('',#16266);
#4751=VERTEX_POINT('',#16341);
#4752=VERTEX_POINT('',#16342);
#4753=VERTEX_POINT('',#16419);
#4754=VERTEX_POINT('',#16420);
#4755=VERTEX_POINT('',#16497);
#4756=VERTEX_POINT('',#16498);
#4757=VERTEX_POINT('',#16573);
#4758=VERTEX_POINT('',#16574);
#4759=VERTEX_POINT('',#16649);
#4760=VERTEX_POINT('',#16650);
#4761=VERTEX_POINT('',#16725);
#4762=VERTEX_POINT('',#16726);
#4763=VERTEX_POINT('',#16801);
#4764=VERTEX_POINT('',#16802);
#4765=VERTEX_POINT('',#16877);
#4766=VERTEX_POINT('',#16878);
#4767=VERTEX_POINT('',#16955);
#4768=VERTEX_POINT('',#16956);
#4769=VERTEX_POINT('',#17033);
#4770=VERTEX_POINT('',#17034);
#4771=VERTEX_POINT('',#17109);
#4772=VERTEX_POINT('',#17110);
#4773=VERTEX_POINT('',#17185);
#4774=VERTEX_POINT('',#17186);
#4775=VERTEX_POINT('',#17261);
#4776=VERTEX_POINT('',#17262);
#4777=VERTEX_POINT('',#17337);
#4778=VERTEX_POINT('',#17338);
#4779=VERTEX_POINT('',#17340);
#4780=VERTEX_POINT('',#17357);
#4781=VERTEX_POINT('',#17372);
#4782=VERTEX_POINT('',#17373);
#4783=VERTEX_POINT('',#17450);
#4784=VERTEX_POINT('',#17451);
#4785=VERTEX_POINT('',#17526);
#4786=VERTEX_POINT('',#17527);
#4787=VERTEX_POINT('',#17602);
#4788=VERTEX_POINT('',#17603);
#4789=VERTEX_POINT('',#17678);
#4790=VERTEX_POINT('',#17679);
#4791=VERTEX_POINT('',#17754);
#4792=VERTEX_POINT('',#17755);
#4793=VERTEX_POINT('',#17830);
#4794=VERTEX_POINT('',#17831);
#4795=VERTEX_POINT('',#17910);
#4796=VERTEX_POINT('',#17911);
#4797=VERTEX_POINT('',#17986);
#4798=VERTEX_POINT('',#17987);
#4799=VERTEX_POINT('',#18062);
#4800=VERTEX_POINT('',#18063);
#4801=VERTEX_POINT('',#18138);
#4802=VERTEX_POINT('',#18139);
#4803=VERTEX_POINT('',#18214);
#4804=VERTEX_POINT('',#18215);
#4805=VERTEX_POINT('',#18290);
#4806=VERTEX_POINT('',#18291);
#4807=VERTEX_POINT('',#18368);
#4808=VERTEX_POINT('',#18369);
#4809=VERTEX_POINT('',#18446);
#4810=VERTEX_POINT('',#18447);
#4811=VERTEX_POINT('',#18522);
#4812=VERTEX_POINT('',#18523);
#4813=VERTEX_POINT('',#18598);
#4814=VERTEX_POINT('',#18599);
#4815=VERTEX_POINT('',#18674);
#4816=VERTEX_POINT('',#18675);
#4817=VERTEX_POINT('',#18750);
#4818=VERTEX_POINT('',#18751);
#4819=VERTEX_POINT('',#18753);
#4820=VERTEX_POINT('',#18764);
#4821=VERTEX_POINT('',#18765);
#4822=VERTEX_POINT('',#18842);
#4823=VERTEX_POINT('',#18843);
#4824=VERTEX_POINT('',#18918);
#4825=VERTEX_POINT('',#18919);
#4826=VERTEX_POINT('',#18994);
#4827=VERTEX_POINT('',#18995);
#4828=VERTEX_POINT('',#19070);
#4829=VERTEX_POINT('',#19071);
#4830=VERTEX_POINT('',#19146);
#4831=VERTEX_POINT('',#19147);
#4832=VERTEX_POINT('',#19222);
#4833=VERTEX_POINT('',#19223);
#4834=VERTEX_POINT('',#19300);
#4835=VERTEX_POINT('',#19301);
#4836=VERTEX_POINT('',#19378);
#4837=VERTEX_POINT('',#19379);
#4838=VERTEX_POINT('',#19454);
#4839=VERTEX_POINT('',#19455);
#4840=VERTEX_POINT('',#19530);
#4841=VERTEX_POINT('',#19531);
#4842=VERTEX_POINT('',#19606);
#4843=VERTEX_POINT('',#19607);
#4844=VERTEX_POINT('',#19682);
#4845=VERTEX_POINT('',#19683);
#4846=VERTEX_POINT('',#19760);
#4847=VERTEX_POINT('',#19761);
#4848=VERTEX_POINT('',#19838);
#4849=VERTEX_POINT('',#19839);
#4850=VERTEX_POINT('',#19914);
#4851=VERTEX_POINT('',#19915);
#4852=VERTEX_POINT('',#19990);
#4853=VERTEX_POINT('',#19991);
#4854=VERTEX_POINT('',#20066);
#4855=VERTEX_POINT('',#20067);
#4856=VERTEX_POINT('',#20142);
#4857=VERTEX_POINT('',#20143);
#4858=VERTEX_POINT('',#20145);
#4859=VERTEX_POINT('',#20180);
#4860=VERTEX_POINT('',#20213);
#4861=VERTEX_POINT('',#20214);
#4862=VERTEX_POINT('',#20289);
#4863=VERTEX_POINT('',#20290);
#4864=VERTEX_POINT('',#20365);
#4865=VERTEX_POINT('',#20366);
#4866=VERTEX_POINT('',#20441);
#4867=VERTEX_POINT('',#20442);
#4868=VERTEX_POINT('',#20517);
#4869=VERTEX_POINT('',#20518);
#4870=VERTEX_POINT('',#20593);
#4871=VERTEX_POINT('',#20594);
#4872=VERTEX_POINT('',#20671);
#4873=VERTEX_POINT('',#20672);
#4874=VERTEX_POINT('',#20749);
#4875=VERTEX_POINT('',#20750);
#4876=VERTEX_POINT('',#20825);
#4877=VERTEX_POINT('',#20826);
#4878=VERTEX_POINT('',#20901);
#4879=VERTEX_POINT('',#20902);
#4880=VERTEX_POINT('',#20977);
#4881=VERTEX_POINT('',#20978);
#4882=VERTEX_POINT('',#21053);
#4883=VERTEX_POINT('',#21054);
#4884=VERTEX_POINT('',#21129);
#4885=VERTEX_POINT('',#21130);
#4886=VERTEX_POINT('',#21209);
#4887=VERTEX_POINT('',#21210);
#4888=VERTEX_POINT('',#21285);
#4889=VERTEX_POINT('',#21286);
#4890=VERTEX_POINT('',#21361);
#4891=VERTEX_POINT('',#21362);
#4892=VERTEX_POINT('',#21437);
#4893=VERTEX_POINT('',#21438);
#4894=VERTEX_POINT('',#21513);
#4895=VERTEX_POINT('',#21514);
#4896=VERTEX_POINT('',#21516);
#4897=VERTEX_POINT('',#21533);
#4898=VERTEX_POINT('',#21534);
#4899=VERTEX_POINT('',#21536);
#4900=VERTEX_POINT('',#21593);
#4901=VERTEX_POINT('',#21594);
#4902=VERTEX_POINT('',#21669);
#4903=VERTEX_POINT('',#21670);
#4904=VERTEX_POINT('',#21745);
#4905=VERTEX_POINT('',#21746);
#4906=VERTEX_POINT('',#21821);
#4907=VERTEX_POINT('',#21822);
#4908=VERTEX_POINT('',#21899);
#4909=VERTEX_POINT('',#21900);
#4910=VERTEX_POINT('',#21902);
#4911=VERTEX_POINT('',#21937);
#4912=VERTEX_POINT('',#21972);
#4913=VERTEX_POINT('',#21973);
#4914=VERTEX_POINT('',#21975);
#4915=VERTEX_POINT('',#21992);
#4916=VERTEX_POINT('',#21993);
#4917=VERTEX_POINT('',#21995);
#4918=VERTEX_POINT('',#22052);
#4919=VERTEX_POINT('',#22053);
#4920=VERTEX_POINT('',#22128);
#4921=VERTEX_POINT('',#22129);
#4922=VERTEX_POINT('',#22204);
#4923=VERTEX_POINT('',#22205);
#4924=VERTEX_POINT('',#22280);
#4925=VERTEX_POINT('',#22281);
#4926=VERTEX_POINT('',#22358);
#4927=VERTEX_POINT('',#22359);
#4928=VERTEX_POINT('',#22361);
#4929=VERTEX_POINT('',#22396);
#4930=VERTEX_POINT('',#22431);
#4931=VERTEX_POINT('',#22432);
#4932=VERTEX_POINT('',#22434);
#4933=VERTEX_POINT('',#22451);
#4934=VERTEX_POINT('',#22452);
#4935=VERTEX_POINT('',#22454);
#4936=VERTEX_POINT('',#22511);
#4937=VERTEX_POINT('',#22512);
#4938=VERTEX_POINT('',#22587);
#4939=VERTEX_POINT('',#22588);
#4940=VERTEX_POINT('',#22663);
#4941=VERTEX_POINT('',#22664);
#4942=VERTEX_POINT('',#22739);
#4943=VERTEX_POINT('',#22740);
#4944=VERTEX_POINT('',#22817);
#4945=VERTEX_POINT('',#22818);
#4946=VERTEX_POINT('',#22820);
#4947=VERTEX_POINT('',#22855);
#4948=VERTEX_POINT('',#22890);
#4949=VERTEX_POINT('',#22891);
#4950=VERTEX_POINT('',#22893);
#4951=VERTEX_POINT('',#22910);
#4952=VERTEX_POINT('',#22911);
#4953=VERTEX_POINT('',#22913);
#4954=VERTEX_POINT('',#22970);
#4955=VERTEX_POINT('',#22971);
#4956=VERTEX_POINT('',#23046);
#4957=VERTEX_POINT('',#23047);
#4958=VERTEX_POINT('',#23122);
#4959=VERTEX_POINT('',#23123);
#4960=VERTEX_POINT('',#23198);
#4961=VERTEX_POINT('',#23199);
#4962=VERTEX_POINT('',#23276);
#4963=VERTEX_POINT('',#23277);
#4964=VERTEX_POINT('',#23279);
#4965=VERTEX_POINT('',#23314);
#4966=VERTEX_POINT('',#23641);
#4967=VERTEX_POINT('',#23678);
#4968=VERTEX_POINT('',#23713);
#4969=VERTEX_POINT('',#23742);
#4970=VERTEX_POINT('',#23769);
#4971=VERTEX_POINT('',#23790);
#4972=VERTEX_POINT('',#23809);
#4973=VERTEX_POINT('',#23822);
#4974=VERTEX_POINT('',#23833);
#4975=VERTEX_POINT('',#23835);
#4976=VERTEX_POINT('',#23839);
#4977=VERTEX_POINT('',#23841);
#4978=VERTEX_POINT('',#23845);
#4979=VERTEX_POINT('',#23847);
#4980=VERTEX_POINT('',#23851);
#4981=VERTEX_POINT('',#23855);
#4982=VERTEX_POINT('',#23884);
#4983=VERTEX_POINT('',#23897);
#4984=VERTEX_POINT('',#23913);
#4985=VERTEX_POINT('',#23917);
#4986=VERTEX_POINT('',#23946);
#4987=VERTEX_POINT('',#23959);
#4988=VERTEX_POINT('',#23975);
#4989=VERTEX_POINT('',#23979);
#4990=VERTEX_POINT('',#24008);
#4991=VERTEX_POINT('',#24021);
#4992=VERTEX_POINT('',#24037);
#4993=VERTEX_POINT('',#24041);
#4994=VERTEX_POINT('',#24070);
#4995=VERTEX_POINT('',#24083);
#4996=VERTEX_POINT('',#24099);
#4997=VERTEX_POINT('',#24741);
#4998=VERTEX_POINT('',#25683);
#4999=VERTEX_POINT('',#26631);
#5000=VERTEX_POINT('',#26632);
#5001=VERTEX_POINT('',#26634);
#5002=VERTEX_POINT('',#26636);
#5003=VERTEX_POINT('',#26638);
#5004=VERTEX_POINT('',#26640);
#5005=VERTEX_POINT('',#26642);
#5006=VERTEX_POINT('',#26644);
#5007=VERTEX_POINT('',#27291);
#5008=VERTEX_POINT('',#28232);
#5009=VERTEX_POINT('',#29817);
#5010=VERTEX_POINT('',#30758);
#5011=VERTEX_POINT('',#32343);
#5012=VERTEX_POINT('',#33284);
#5013=VERTEX_POINT('',#34234);
#5014=VERTEX_POINT('',#34236);
#5015=VERTEX_POINT('',#34240);
#5016=VERTEX_POINT('',#34244);
#5017=VERTEX_POINT('',#34246);
#5018=VERTEX_POINT('',#34250);
#5019=VERTEX_POINT('',#34254);
#5020=VERTEX_POINT('',#34258);
#5021=VERTEX_POINT('',#34262);
#5022=VERTEX_POINT('',#34266);
#5023=VERTEX_POINT('',#34270);
#5024=VERTEX_POINT('',#34274);
#5025=VERTEX_POINT('',#34278);
#5026=VERTEX_POINT('',#34282);
#5027=VERTEX_POINT('',#34288);
#5028=VERTEX_POINT('',#34292);
#5029=VERTEX_POINT('',#34299);
#5030=VERTEX_POINT('',#34300);
#5031=VERTEX_POINT('',#34302);
#5032=VERTEX_POINT('',#34304);
#5033=VERTEX_POINT('',#34311);
#5034=VERTEX_POINT('',#34317);
#5035=VERTEX_POINT('',#34318);
#5036=VERTEX_POINT('',#34322);
#5037=VERTEX_POINT('',#34325);
#5038=VERTEX_POINT('',#34327);
#5039=VERTEX_POINT('',#34336);
#5040=VERTEX_POINT('',#34338);
#5041=VERTEX_POINT('',#34342);
#5042=VERTEX_POINT('',#34344);
#5043=VERTEX_POINT('',#34348);
#5044=VERTEX_POINT('',#34350);
#5045=VERTEX_POINT('',#34354);
#5046=VERTEX_POINT('',#34356);
#5047=VERTEX_POINT('',#34360);
#5048=VERTEX_POINT('',#34362);
#5049=VERTEX_POINT('',#34366);
#5050=VERTEX_POINT('',#34370);
#5051=VERTEX_POINT('',#34374);
#5052=VERTEX_POINT('',#34378);
#5053=VERTEX_POINT('',#34382);
#5054=VERTEX_POINT('',#34384);
#5055=VERTEX_POINT('',#34392);
#5056=VERTEX_POINT('',#34393);
#5057=VERTEX_POINT('',#34395);
#5058=VERTEX_POINT('',#34397);
#5059=VERTEX_POINT('',#34401);
#5060=VERTEX_POINT('',#34402);
#5061=VERTEX_POINT('',#34407);
#5062=VERTEX_POINT('',#34411);
#5063=VERTEX_POINT('',#34417);
#5064=VERTEX_POINT('',#34418);
#5065=VERTEX_POINT('',#34420);
#5066=VERTEX_POINT('',#34422);
#5067=VERTEX_POINT('',#34426);
#5068=VERTEX_POINT('',#34428);
#5069=VERTEX_POINT('',#34432);
#5070=VERTEX_POINT('',#34433);
#5071=VERTEX_POINT('',#34435);
#5072=VERTEX_POINT('',#34437);
#5073=VERTEX_POINT('',#34439);
#5074=VERTEX_POINT('',#34441);
#5075=VERTEX_POINT('',#34443);
#5076=VERTEX_POINT('',#34445);
#5077=VERTEX_POINT('',#34449);
#5078=VERTEX_POINT('',#34451);
#5079=VERTEX_POINT('',#34455);
#5080=VERTEX_POINT('',#34459);
#5081=VERTEX_POINT('',#34463);
#5082=VERTEX_POINT('',#34465);
#5083=VERTEX_POINT('',#34469);
#5084=VERTEX_POINT('',#34473);
#5085=VERTEX_POINT('',#34477);
#5086=VERTEX_POINT('',#34481);
#5087=VERTEX_POINT('',#34485);
#5088=VERTEX_POINT('',#34489);
#5089=VERTEX_POINT('',#34493);
#5090=VERTEX_POINT('',#34497);
#5091=VERTEX_POINT('',#34501);
#5092=VERTEX_POINT('',#34505);
#5093=VERTEX_POINT('',#34507);
#5094=VERTEX_POINT('',#34511);
#5095=VERTEX_POINT('',#34515);
#5096=VERTEX_POINT('',#34522);
#5097=VERTEX_POINT('',#34530);
#5098=VERTEX_POINT('',#34532);
#5099=VERTEX_POINT('',#34536);
#5100=VERTEX_POINT('',#34538);
#5101=VERTEX_POINT('',#34542);
#5102=VERTEX_POINT('',#34544);
#5103=VERTEX_POINT('',#34548);
#5104=VERTEX_POINT('',#34550);
#5105=VERTEX_POINT('',#34554);
#5106=VERTEX_POINT('',#34556);
#5107=VERTEX_POINT('',#34560);
#5108=VERTEX_POINT('',#34561);
#5109=VERTEX_POINT('',#34563);
#5110=VERTEX_POINT('',#34565);
#5111=VERTEX_POINT('',#34567);
#5112=VERTEX_POINT('',#34569);
#5113=VERTEX_POINT('',#34571);
#5114=VERTEX_POINT('',#34573);
#5115=VERTEX_POINT('',#34577);
#5116=VERTEX_POINT('',#34578);
#5117=VERTEX_POINT('',#34580);
#5118=VERTEX_POINT('',#34582);
#5119=VERTEX_POINT('',#34584);
#5120=VERTEX_POINT('',#34586);
#5121=VERTEX_POINT('',#34588);
#5122=VERTEX_POINT('',#34590);
#5650=EDGE_CURVE('',#4593,#4593,#4280,.T.);
#5651=EDGE_CURVE('',#4593,#4594,#2388,.T.);
#5652=EDGE_CURVE('',#4594,#4595,#4281,.T.);
#5653=EDGE_CURVE('',#4595,#4594,#4282,.T.);
#5654=EDGE_CURVE('',#4596,#4597,#762,.F.);
#5655=EDGE_CURVE('',#4597,#4595,#4283,.T.);
#5656=EDGE_CURVE('',#4597,#4598,#763,.F.);
#5657=EDGE_CURVE('',#4598,#4599,#714,.T.);
#5658=EDGE_CURVE('',#4600,#4599,#4284,.T.);
#5659=EDGE_CURVE('',#4601,#4600,#715,.T.);
#5660=EDGE_CURVE('',#4601,#4602,#764,.T.);
#5661=EDGE_CURVE('',#4602,#4603,#716,.T.);
#5662=EDGE_CURVE('',#4604,#4603,#4285,.T.);
#5663=EDGE_CURVE('',#4604,#4605,#717,.T.);
#5664=EDGE_CURVE('',#4605,#4606,#765,.F.);
#5665=EDGE_CURVE('',#4607,#4606,#718,.T.);
#5666=EDGE_CURVE('',#4608,#4607,#4286,.T.);
#5667=EDGE_CURVE('',#4608,#4609,#719,.T.);
#5668=EDGE_CURVE('',#4609,#4610,#766,.T.);
#5669=EDGE_CURVE('',#4611,#4610,#720,.T.);
#5670=EDGE_CURVE('',#4612,#4611,#4287,.T.);
#5671=EDGE_CURVE('',#4596,#4612,#721,.T.);
#5672=EDGE_CURVE('',#4603,#4613,#2389,.T.);
#5673=EDGE_CURVE('',#4613,#4604,#2390,.T.);
#5674=EDGE_CURVE('',#4614,#4607,#2391,.T.);
#5675=EDGE_CURVE('',#4614,#4608,#2392,.T.);
#5676=EDGE_CURVE('',#4615,#4611,#2393,.T.);
#5677=EDGE_CURVE('',#4612,#4615,#2394,.T.);
#5678=EDGE_CURVE('',#4600,#4616,#2395,.T.);
#5679=EDGE_CURVE('',#4599,#4616,#2396,.T.);
#5680=EDGE_CURVE('',#4617,#4616,#2397,.T.);
#5681=EDGE_CURVE('',#4618,#4617,#2398,.T.);
#5682=EDGE_CURVE('',#4618,#4601,#2399,.T.);
#5683=EDGE_CURVE('',#4619,#4602,#2400,.T.);
#5684=EDGE_CURVE('',#4619,#4620,#2401,.T.);
#5685=EDGE_CURVE('',#4620,#4613,#2402,.T.);
#5686=EDGE_CURVE('',#4621,#4610,#2403,.T.);
#5687=EDGE_CURVE('',#4622,#4621,#2404,.T.);
#5688=EDGE_CURVE('',#4622,#4615,#2405,.T.);
#5689=EDGE_CURVE('',#4618,#4619,#2406,.T.);
#5690=EDGE_CURVE('',#4623,#4614,#2407,.T.);
#5691=EDGE_CURVE('',#4623,#4624,#2408,.T.);
#5692=EDGE_CURVE('',#4624,#4609,#2409,.T.);
#5693=EDGE_CURVE('',#4624,#4621,#2410,.T.);
#5694=EDGE_CURVE('',#4623,#4625,#2411,.T.);
#5695=EDGE_CURVE('',#4626,#4625,#2412,.T.);
#5696=EDGE_CURVE('',#4620,#4626,#2413,.T.);
#5697=EDGE_CURVE('',#4627,#4617,#2414,.T.);
#5698=EDGE_CURVE('',#4628,#4627,#2415,.T.);
#5699=EDGE_CURVE('',#4628,#4622,#2416,.T.);
#5700=EDGE_CURVE('',#4626,#4605,#2417,.T.);
#5701=EDGE_CURVE('',#4625,#4606,#2418,.T.);
#5702=EDGE_CURVE('',#4628,#4596,#2419,.T.);
#5703=EDGE_CURVE('',#4627,#4598,#2420,.T.);
#5704=EDGE_CURVE('',#4629,#4629,#4288,.T.);
#5705=EDGE_CURVE('',#4629,#4630,#2421,.T.);
#5706=EDGE_CURVE('',#4630,#4631,#4289,.T.);
#5707=EDGE_CURVE('',#4631,#4630,#4290,.T.);
#5708=EDGE_CURVE('',#4632,#4633,#767,.F.);
#5709=EDGE_CURVE('',#4633,#4631,#4291,.T.);
#5710=EDGE_CURVE('',#4633,#4634,#768,.F.);
#5711=EDGE_CURVE('',#4634,#4635,#722,.T.);
#5712=EDGE_CURVE('',#4636,#4635,#4292,.T.);
#5713=EDGE_CURVE('',#4637,#4636,#723,.T.);
#5714=EDGE_CURVE('',#4637,#4638,#769,.T.);
#5715=EDGE_CURVE('',#4638,#4639,#724,.T.);
#5716=EDGE_CURVE('',#4640,#4639,#4293,.T.);
#5717=EDGE_CURVE('',#4640,#4641,#725,.T.);
#5718=EDGE_CURVE('',#4641,#4642,#770,.F.);
#5719=EDGE_CURVE('',#4643,#4642,#726,.T.);
#5720=EDGE_CURVE('',#4644,#4643,#4294,.T.);
#5721=EDGE_CURVE('',#4644,#4645,#727,.T.);
#5722=EDGE_CURVE('',#4645,#4646,#771,.T.);
#5723=EDGE_CURVE('',#4647,#4646,#728,.T.);
#5724=EDGE_CURVE('',#4648,#4647,#4295,.T.);
#5725=EDGE_CURVE('',#4632,#4648,#729,.T.);
#5726=EDGE_CURVE('',#4639,#4649,#2422,.T.);
#5727=EDGE_CURVE('',#4649,#4640,#2423,.T.);
#5728=EDGE_CURVE('',#4650,#4643,#2424,.T.);
#5729=EDGE_CURVE('',#4650,#4644,#2425,.T.);
#5730=EDGE_CURVE('',#4651,#4647,#2426,.T.);
#5731=EDGE_CURVE('',#4648,#4651,#2427,.T.);
#5732=EDGE_CURVE('',#4636,#4652,#2428,.T.);
#5733=EDGE_CURVE('',#4635,#4652,#2429,.T.);
#5734=EDGE_CURVE('',#4653,#4652,#2430,.T.);
#5735=EDGE_CURVE('',#4654,#4653,#2431,.T.);
#5736=EDGE_CURVE('',#4654,#4637,#2432,.T.);
#5737=EDGE_CURVE('',#4655,#4638,#2433,.T.);
#5738=EDGE_CURVE('',#4655,#4656,#2434,.T.);
#5739=EDGE_CURVE('',#4656,#4649,#2435,.T.);
#5740=EDGE_CURVE('',#4657,#4646,#2436,.T.);
#5741=EDGE_CURVE('',#4658,#4657,#2437,.T.);
#5742=EDGE_CURVE('',#4658,#4651,#2438,.T.);
#5743=EDGE_CURVE('',#4654,#4655,#2439,.T.);
#5744=EDGE_CURVE('',#4659,#4650,#2440,.T.);
#5745=EDGE_CURVE('',#4659,#4660,#2441,.T.);
#5746=EDGE_CURVE('',#4660,#4645,#2442,.T.);
#5747=EDGE_CURVE('',#4660,#4657,#2443,.T.);
#5748=EDGE_CURVE('',#4659,#4661,#2444,.T.);
#5749=EDGE_CURVE('',#4662,#4661,#2445,.T.);
#5750=EDGE_CURVE('',#4656,#4662,#2446,.T.);
#5751=EDGE_CURVE('',#4663,#4653,#2447,.T.);
#5752=EDGE_CURVE('',#4664,#4663,#2448,.T.);
#5753=EDGE_CURVE('',#4664,#4658,#2449,.T.);
#5754=EDGE_CURVE('',#4662,#4641,#2450,.T.);
#5755=EDGE_CURVE('',#4661,#4642,#2451,.T.);
#5756=EDGE_CURVE('',#4664,#4632,#2452,.T.);
#5757=EDGE_CURVE('',#4663,#4634,#2453,.T.);
#5758=EDGE_CURVE('',#4665,#4665,#4296,.T.);
#5759=EDGE_CURVE('',#4665,#4666,#2454,.T.);
#5760=EDGE_CURVE('',#4666,#4667,#4297,.T.);
#5761=EDGE_CURVE('',#4667,#4666,#4298,.T.);
#5762=EDGE_CURVE('',#4668,#4669,#772,.F.);
#5763=EDGE_CURVE('',#4669,#4667,#4299,.T.);
#5764=EDGE_CURVE('',#4669,#4670,#773,.F.);
#5765=EDGE_CURVE('',#4670,#4671,#730,.T.);
#5766=EDGE_CURVE('',#4672,#4671,#4300,.T.);
#5767=EDGE_CURVE('',#4673,#4672,#731,.T.);
#5768=EDGE_CURVE('',#4673,#4674,#774,.T.);
#5769=EDGE_CURVE('',#4674,#4675,#732,.T.);
#5770=EDGE_CURVE('',#4676,#4675,#4301,.T.);
#5771=EDGE_CURVE('',#4676,#4677,#733,.T.);
#5772=EDGE_CURVE('',#4677,#4678,#775,.F.);
#5773=EDGE_CURVE('',#4679,#4678,#734,.T.);
#5774=EDGE_CURVE('',#4680,#4679,#4302,.T.);
#5775=EDGE_CURVE('',#4680,#4681,#735,.T.);
#5776=EDGE_CURVE('',#4681,#4682,#776,.T.);
#5777=EDGE_CURVE('',#4683,#4682,#736,.T.);
#5778=EDGE_CURVE('',#4684,#4683,#4303,.T.);
#5779=EDGE_CURVE('',#4668,#4684,#737,.T.);
#5780=EDGE_CURVE('',#4675,#4685,#2455,.T.);
#5781=EDGE_CURVE('',#4685,#4676,#2456,.T.);
#5782=EDGE_CURVE('',#4686,#4679,#2457,.T.);
#5783=EDGE_CURVE('',#4686,#4680,#2458,.T.);
#5784=EDGE_CURVE('',#4687,#4683,#2459,.T.);
#5785=EDGE_CURVE('',#4684,#4687,#2460,.T.);
#5786=EDGE_CURVE('',#4672,#4688,#2461,.T.);
#5787=EDGE_CURVE('',#4671,#4688,#2462,.T.);
#5788=EDGE_CURVE('',#4689,#4688,#2463,.T.);
#5789=EDGE_CURVE('',#4690,#4689,#2464,.T.);
#5790=EDGE_CURVE('',#4690,#4673,#2465,.T.);
#5791=EDGE_CURVE('',#4691,#4674,#2466,.T.);
#5792=EDGE_CURVE('',#4691,#4692,#2467,.T.);
#5793=EDGE_CURVE('',#4692,#4685,#2468,.T.);
#5794=EDGE_CURVE('',#4693,#4682,#2469,.T.);
#5795=EDGE_CURVE('',#4694,#4693,#2470,.T.);
#5796=EDGE_CURVE('',#4694,#4687,#2471,.T.);
#5797=EDGE_CURVE('',#4690,#4691,#2472,.T.);
#5798=EDGE_CURVE('',#4695,#4686,#2473,.T.);
#5799=EDGE_CURVE('',#4695,#4696,#2474,.T.);
#5800=EDGE_CURVE('',#4696,#4681,#2475,.T.);
#5801=EDGE_CURVE('',#4696,#4693,#2476,.T.);
#5802=EDGE_CURVE('',#4695,#4697,#2477,.T.);
#5803=EDGE_CURVE('',#4698,#4697,#2478,.T.);
#5804=EDGE_CURVE('',#4692,#4698,#2479,.T.);
#5805=EDGE_CURVE('',#4699,#4689,#2480,.T.);
#5806=EDGE_CURVE('',#4700,#4699,#2481,.T.);
#5807=EDGE_CURVE('',#4700,#4694,#2482,.T.);
#5808=EDGE_CURVE('',#4698,#4677,#2483,.T.);
#5809=EDGE_CURVE('',#4697,#4678,#2484,.T.);
#5810=EDGE_CURVE('',#4700,#4668,#2485,.T.);
#5811=EDGE_CURVE('',#4699,#4670,#2486,.T.);
#5812=EDGE_CURVE('',#4701,#4701,#4304,.T.);
#5813=EDGE_CURVE('',#4701,#4702,#2487,.T.);
#5814=EDGE_CURVE('',#4702,#4703,#4305,.T.);
#5815=EDGE_CURVE('',#4703,#4702,#4306,.T.);
#5816=EDGE_CURVE('',#4704,#4705,#777,.F.);
#5817=EDGE_CURVE('',#4705,#4703,#4307,.T.);
#5818=EDGE_CURVE('',#4705,#4706,#778,.F.);
#5819=EDGE_CURVE('',#4706,#4707,#738,.T.);
#5820=EDGE_CURVE('',#4708,#4707,#4308,.T.);
#5821=EDGE_CURVE('',#4709,#4708,#739,.T.);
#5822=EDGE_CURVE('',#4709,#4710,#779,.T.);
#5823=EDGE_CURVE('',#4710,#4711,#740,.T.);
#5824=EDGE_CURVE('',#4712,#4711,#4309,.T.);
#5825=EDGE_CURVE('',#4712,#4713,#741,.T.);
#5826=EDGE_CURVE('',#4713,#4714,#780,.F.);
#5827=EDGE_CURVE('',#4715,#4714,#742,.T.);
#5828=EDGE_CURVE('',#4716,#4715,#4310,.T.);
#5829=EDGE_CURVE('',#4716,#4717,#743,.T.);
#5830=EDGE_CURVE('',#4717,#4718,#781,.T.);
#5831=EDGE_CURVE('',#4719,#4718,#744,.T.);
#5832=EDGE_CURVE('',#4720,#4719,#4311,.T.);
#5833=EDGE_CURVE('',#4704,#4720,#745,.T.);
#5834=EDGE_CURVE('',#4711,#4721,#2488,.T.);
#5835=EDGE_CURVE('',#4721,#4712,#2489,.T.);
#5836=EDGE_CURVE('',#4722,#4715,#2490,.T.);
#5837=EDGE_CURVE('',#4722,#4716,#2491,.T.);
#5838=EDGE_CURVE('',#4723,#4719,#2492,.T.);
#5839=EDGE_CURVE('',#4720,#4723,#2493,.T.);
#5840=EDGE_CURVE('',#4708,#4724,#2494,.T.);
#5841=EDGE_CURVE('',#4707,#4724,#2495,.T.);
#5842=EDGE_CURVE('',#4725,#4724,#2496,.T.);
#5843=EDGE_CURVE('',#4726,#4725,#2497,.T.);
#5844=EDGE_CURVE('',#4726,#4709,#2498,.T.);
#5845=EDGE_CURVE('',#4727,#4710,#2499,.T.);
#5846=EDGE_CURVE('',#4727,#4728,#2500,.T.);
#5847=EDGE_CURVE('',#4728,#4721,#2501,.T.);
#5848=EDGE_CURVE('',#4729,#4718,#2502,.T.);
#5849=EDGE_CURVE('',#4730,#4729,#2503,.T.);
#5850=EDGE_CURVE('',#4730,#4723,#2504,.T.);
#5851=EDGE_CURVE('',#4726,#4727,#2505,.T.);
#5852=EDGE_CURVE('',#4731,#4722,#2506,.T.);
#5853=EDGE_CURVE('',#4731,#4732,#2507,.T.);
#5854=EDGE_CURVE('',#4732,#4717,#2508,.T.);
#5855=EDGE_CURVE('',#4732,#4729,#2509,.T.);
#5856=EDGE_CURVE('',#4731,#4733,#2510,.T.);
#5857=EDGE_CURVE('',#4734,#4733,#2511,.T.);
#5858=EDGE_CURVE('',#4728,#4734,#2512,.T.);
#5859=EDGE_CURVE('',#4735,#4725,#2513,.T.);
#5860=EDGE_CURVE('',#4736,#4735,#2514,.T.);
#5861=EDGE_CURVE('',#4736,#4730,#2515,.T.);
#5862=EDGE_CURVE('',#4734,#4713,#2516,.T.);
#5863=EDGE_CURVE('',#4733,#4714,#2517,.T.);
#5864=EDGE_CURVE('',#4736,#4704,#2518,.T.);
#5865=EDGE_CURVE('',#4735,#4706,#2519,.T.);
#5866=EDGE_CURVE('',#4737,#4738,#2520,.T.);
#5867=EDGE_CURVE('',#4737,#4739,#782,.T.);
#5868=EDGE_CURVE('',#4739,#4740,#4312,.T.);
#5869=EDGE_CURVE('',#4740,#4738,#783,.T.);
#5870=EDGE_CURVE('',#4741,#4742,#2521,.T.);
#5871=EDGE_CURVE('',#4741,#4737,#784,.T.);
#5872=EDGE_CURVE('',#4738,#4742,#785,.T.);
#5873=EDGE_CURVE('',#4743,#4744,#2522,.T.);
#5874=EDGE_CURVE('',#4743,#4741,#786,.T.);
#5875=EDGE_CURVE('',#4742,#4744,#787,.T.);
#5876=EDGE_CURVE('',#4745,#4746,#2523,.T.);
#5877=EDGE_CURVE('',#4745,#4743,#788,.T.);
#5878=EDGE_CURVE('',#4744,#4746,#789,.T.);
#5879=EDGE_CURVE('',#4747,#4748,#2524,.T.);
#5880=EDGE_CURVE('',#4747,#4745,#790,.T.);
#5881=EDGE_CURVE('',#4746,#4748,#791,.T.);
#5882=EDGE_CURVE('',#4749,#4750,#2525,.T.);
#5883=EDGE_CURVE('',#4749,#4747,#792,.T.);
#5884=EDGE_CURVE('',#4748,#4750,#793,.T.);
#5885=EDGE_CURVE('',#4751,#4752,#2526,.T.);
#5886=EDGE_CURVE('',#4751,#4749,#794,.T.);
#5887=EDGE_CURVE('',#4750,#4752,#795,.T.);
#5888=EDGE_CURVE('',#4753,#4754,#2527,.T.);
#5889=EDGE_CURVE('',#4753,#4751,#796,.T.);
#5890=EDGE_CURVE('',#4752,#4754,#797,.T.);
#5891=EDGE_CURVE('',#4755,#4756,#2528,.T.);
#5892=EDGE_CURVE('',#4755,#4753,#798,.T.);
#5893=EDGE_CURVE('',#4754,#4756,#799,.T.);
#5894=EDGE_CURVE('',#4757,#4758,#2529,.T.);
#5895=EDGE_CURVE('',#4757,#4755,#800,.T.);
#5896=EDGE_CURVE('',#4756,#4758,#801,.T.);
#5897=EDGE_CURVE('',#4759,#4760,#2530,.T.);
#5898=EDGE_CURVE('',#4759,#4757,#802,.T.);
#5899=EDGE_CURVE('',#4758,#4760,#803,.T.);
#5900=EDGE_CURVE('',#4761,#4762,#2531,.T.);
#5901=EDGE_CURVE('',#4761,#4759,#804,.T.);
#5902=EDGE_CURVE('',#4760,#4762,#805,.T.);
#5903=EDGE_CURVE('',#4763,#4764,#2532,.T.);
#5904=EDGE_CURVE('',#4763,#4761,#806,.T.);
#5905=EDGE_CURVE('',#4762,#4764,#807,.T.);
#5906=EDGE_CURVE('',#4765,#4766,#2533,.T.);
#5907=EDGE_CURVE('',#4765,#4763,#808,.T.);
#5908=EDGE_CURVE('',#4764,#4766,#809,.T.);
#5909=EDGE_CURVE('',#4767,#4768,#2534,.T.);
#5910=EDGE_CURVE('',#4767,#4765,#810,.T.);
#5911=EDGE_CURVE('',#4766,#4768,#811,.T.);
#5912=EDGE_CURVE('',#4769,#4770,#2535,.T.);
#5913=EDGE_CURVE('',#4769,#4767,#812,.T.);
#5914=EDGE_CURVE('',#4768,#4770,#813,.T.);
#5915=EDGE_CURVE('',#4771,#4772,#2536,.T.);
#5916=EDGE_CURVE('',#4771,#4769,#814,.T.);
#5917=EDGE_CURVE('',#4770,#4772,#815,.T.);
#5918=EDGE_CURVE('',#4773,#4774,#2537,.T.);
#5919=EDGE_CURVE('',#4773,#4771,#816,.T.);
#5920=EDGE_CURVE('',#4772,#4774,#817,.T.);
#5921=EDGE_CURVE('',#4775,#4776,#2538,.T.);
#5922=EDGE_CURVE('',#4775,#4773,#818,.T.);
#5923=EDGE_CURVE('',#4774,#4776,#819,.T.);
#5924=EDGE_CURVE('',#4777,#4778,#2539,.T.);
#5925=EDGE_CURVE('',#4777,#4779,#820,.T.);
#5926=EDGE_CURVE('',#4779,#4780,#4313,.T.);
#5927=EDGE_CURVE('',#4780,#4778,#821,.T.);
#5928=EDGE_CURVE('',#4781,#4782,#2540,.T.);
#5929=EDGE_CURVE('',#4781,#4777,#822,.T.);
#5930=EDGE_CURVE('',#4778,#4782,#823,.T.);
#5931=EDGE_CURVE('',#4783,#4784,#2541,.T.);
#5932=EDGE_CURVE('',#4783,#4781,#824,.T.);
#5933=EDGE_CURVE('',#4782,#4784,#825,.T.);
#5934=EDGE_CURVE('',#4785,#4786,#2542,.T.);
#5935=EDGE_CURVE('',#4785,#4783,#826,.T.);
#5936=EDGE_CURVE('',#4784,#4786,#827,.T.);
#5937=EDGE_CURVE('',#4787,#4788,#2543,.T.);
#5938=EDGE_CURVE('',#4787,#4785,#828,.T.);
#5939=EDGE_CURVE('',#4786,#4788,#829,.T.);
#5940=EDGE_CURVE('',#4789,#4790,#2544,.T.);
#5941=EDGE_CURVE('',#4789,#4787,#830,.T.);
#5942=EDGE_CURVE('',#4788,#4790,#831,.T.);
#5943=EDGE_CURVE('',#4791,#4792,#2545,.T.);
#5944=EDGE_CURVE('',#4791,#4789,#832,.T.);
#5945=EDGE_CURVE('',#4790,#4792,#833,.T.);
#5946=EDGE_CURVE('',#4793,#4794,#2546,.T.);
#5947=EDGE_CURVE('',#4793,#4791,#834,.T.);
#5948=EDGE_CURVE('',#4792,#4794,#835,.T.);
#5949=EDGE_CURVE('',#4795,#4796,#2547,.T.);
#5950=EDGE_CURVE('',#4795,#4793,#836,.T.);
#5951=EDGE_CURVE('',#4794,#4796,#837,.T.);
#5952=EDGE_CURVE('',#4797,#4798,#2548,.T.);
#5953=EDGE_CURVE('',#4797,#4795,#838,.T.);
#5954=EDGE_CURVE('',#4796,#4798,#839,.T.);
#5955=EDGE_CURVE('',#4799,#4800,#2549,.T.);
#5956=EDGE_CURVE('',#4799,#4797,#840,.T.);
#5957=EDGE_CURVE('',#4798,#4800,#841,.T.);
#5958=EDGE_CURVE('',#4801,#4802,#2550,.T.);
#5959=EDGE_CURVE('',#4801,#4799,#842,.T.);
#5960=EDGE_CURVE('',#4800,#4802,#843,.T.);
#5961=EDGE_CURVE('',#4803,#4804,#2551,.T.);
#5962=EDGE_CURVE('',#4803,#4801,#844,.T.);
#5963=EDGE_CURVE('',#4802,#4804,#845,.T.);
#5964=EDGE_CURVE('',#4805,#4806,#2552,.T.);
#5965=EDGE_CURVE('',#4805,#4803,#846,.T.);
#5966=EDGE_CURVE('',#4804,#4806,#847,.T.);
#5967=EDGE_CURVE('',#4807,#4808,#2553,.T.);
#5968=EDGE_CURVE('',#4807,#4805,#848,.T.);
#5969=EDGE_CURVE('',#4806,#4808,#849,.T.);
#5970=EDGE_CURVE('',#4809,#4810,#2554,.T.);
#5971=EDGE_CURVE('',#4809,#4807,#850,.T.);
#5972=EDGE_CURVE('',#4808,#4810,#851,.T.);
#5973=EDGE_CURVE('',#4811,#4812,#2555,.T.);
#5974=EDGE_CURVE('',#4811,#4809,#852,.T.);
#5975=EDGE_CURVE('',#4810,#4812,#853,.T.);
#5976=EDGE_CURVE('',#4813,#4814,#2556,.T.);
#5977=EDGE_CURVE('',#4813,#4811,#854,.T.);
#5978=EDGE_CURVE('',#4812,#4814,#855,.T.);
#5979=EDGE_CURVE('',#4815,#4816,#2557,.T.);
#5980=EDGE_CURVE('',#4815,#4813,#856,.T.);
#5981=EDGE_CURVE('',#4814,#4816,#857,.T.);
#5982=EDGE_CURVE('',#4817,#4818,#2558,.T.);
#5983=EDGE_CURVE('',#4817,#4819,#858,.T.);
#5984=EDGE_CURVE('',#4819,#4818,#4314,.T.);
#5985=EDGE_CURVE('',#4820,#4821,#2559,.T.);
#5986=EDGE_CURVE('',#4820,#4817,#859,.T.);
#5987=EDGE_CURVE('',#4818,#4821,#860,.T.);
#5988=EDGE_CURVE('',#4822,#4823,#2560,.T.);
#5989=EDGE_CURVE('',#4822,#4820,#861,.T.);
#5990=EDGE_CURVE('',#4821,#4823,#862,.T.);
#5991=EDGE_CURVE('',#4824,#4825,#2561,.T.);
#5992=EDGE_CURVE('',#4824,#4822,#863,.T.);
#5993=EDGE_CURVE('',#4823,#4825,#864,.T.);
#5994=EDGE_CURVE('',#4826,#4827,#2562,.T.);
#5995=EDGE_CURVE('',#4826,#4824,#865,.T.);
#5996=EDGE_CURVE('',#4825,#4827,#866,.T.);
#5997=EDGE_CURVE('',#4828,#4829,#2563,.T.);
#5998=EDGE_CURVE('',#4828,#4826,#867,.T.);
#5999=EDGE_CURVE('',#4827,#4829,#868,.T.);
#6000=EDGE_CURVE('',#4830,#4831,#2564,.T.);
#6001=EDGE_CURVE('',#4830,#4828,#869,.T.);
#6002=EDGE_CURVE('',#4829,#4831,#870,.T.);
#6003=EDGE_CURVE('',#4832,#4833,#2565,.T.);
#6004=EDGE_CURVE('',#4832,#4830,#871,.T.);
#6005=EDGE_CURVE('',#4831,#4833,#872,.T.);
#6006=EDGE_CURVE('',#4834,#4835,#2566,.T.);
#6007=EDGE_CURVE('',#4834,#4832,#873,.T.);
#6008=EDGE_CURVE('',#4833,#4835,#874,.T.);
#6009=EDGE_CURVE('',#4836,#4837,#2567,.T.);
#6010=EDGE_CURVE('',#4836,#4834,#875,.T.);
#6011=EDGE_CURVE('',#4835,#4837,#876,.T.);
#6012=EDGE_CURVE('',#4838,#4839,#2568,.T.);
#6013=EDGE_CURVE('',#4838,#4836,#877,.T.);
#6014=EDGE_CURVE('',#4837,#4839,#878,.T.);
#6015=EDGE_CURVE('',#4840,#4841,#2569,.T.);
#6016=EDGE_CURVE('',#4840,#4838,#879,.T.);
#6017=EDGE_CURVE('',#4839,#4841,#880,.T.);
#6018=EDGE_CURVE('',#4842,#4843,#2570,.T.);
#6019=EDGE_CURVE('',#4842,#4840,#881,.T.);
#6020=EDGE_CURVE('',#4841,#4843,#882,.T.);
#6021=EDGE_CURVE('',#4844,#4845,#2571,.T.);
#6022=EDGE_CURVE('',#4844,#4842,#883,.T.);
#6023=EDGE_CURVE('',#4843,#4845,#884,.T.);
#6024=EDGE_CURVE('',#4846,#4847,#2572,.T.);
#6025=EDGE_CURVE('',#4846,#4844,#885,.T.);
#6026=EDGE_CURVE('',#4845,#4847,#886,.T.);
#6027=EDGE_CURVE('',#4848,#4849,#2573,.T.);
#6028=EDGE_CURVE('',#4848,#4846,#887,.T.);
#6029=EDGE_CURVE('',#4847,#4849,#888,.T.);
#6030=EDGE_CURVE('',#4850,#4851,#2574,.T.);
#6031=EDGE_CURVE('',#4850,#4848,#889,.T.);
#6032=EDGE_CURVE('',#4849,#4851,#890,.T.);
#6033=EDGE_CURVE('',#4852,#4853,#2575,.T.);
#6034=EDGE_CURVE('',#4852,#4850,#891,.T.);
#6035=EDGE_CURVE('',#4851,#4853,#892,.T.);
#6036=EDGE_CURVE('',#4854,#4855,#2576,.T.);
#6037=EDGE_CURVE('',#4854,#4852,#893,.T.);
#6038=EDGE_CURVE('',#4853,#4855,#894,.T.);
#6039=EDGE_CURVE('',#4856,#4857,#2577,.T.);
#6040=EDGE_CURVE('',#4856,#4858,#895,.T.);
#6041=EDGE_CURVE('',#4858,#4859,#4315,.T.);
#6042=EDGE_CURVE('',#4859,#4857,#896,.T.);
#6043=EDGE_CURVE('',#4860,#4861,#2578,.T.);
#6044=EDGE_CURVE('',#4860,#4856,#897,.T.);
#6045=EDGE_CURVE('',#4857,#4861,#898,.T.);
#6046=EDGE_CURVE('',#4862,#4863,#2579,.T.);
#6047=EDGE_CURVE('',#4862,#4860,#899,.T.);
#6048=EDGE_CURVE('',#4861,#4863,#900,.T.);
#6049=EDGE_CURVE('',#4864,#4865,#2580,.T.);
#6050=EDGE_CURVE('',#4864,#4862,#901,.T.);
#6051=EDGE_CURVE('',#4863,#4865,#902,.T.);
#6052=EDGE_CURVE('',#4866,#4867,#2581,.T.);
#6053=EDGE_CURVE('',#4866,#4864,#903,.T.);
#6054=EDGE_CURVE('',#4865,#4867,#904,.T.);
#6055=EDGE_CURVE('',#4868,#4869,#2582,.T.);
#6056=EDGE_CURVE('',#4868,#4866,#905,.T.);
#6057=EDGE_CURVE('',#4867,#4869,#906,.T.);
#6058=EDGE_CURVE('',#4870,#4871,#2583,.T.);
#6059=EDGE_CURVE('',#4870,#4868,#907,.T.);
#6060=EDGE_CURVE('',#4869,#4871,#908,.T.);
#6061=EDGE_CURVE('',#4872,#4873,#2584,.T.);
#6062=EDGE_CURVE('',#4872,#4870,#909,.T.);
#6063=EDGE_CURVE('',#4871,#4873,#910,.T.);
#6064=EDGE_CURVE('',#4874,#4875,#2585,.T.);
#6065=EDGE_CURVE('',#4874,#4872,#911,.T.);
#6066=EDGE_CURVE('',#4873,#4875,#912,.T.);
#6067=EDGE_CURVE('',#4876,#4877,#2586,.T.);
#6068=EDGE_CURVE('',#4876,#4874,#913,.T.);
#6069=EDGE_CURVE('',#4875,#4877,#914,.T.);
#6070=EDGE_CURVE('',#4878,#4879,#2587,.T.);
#6071=EDGE_CURVE('',#4878,#4876,#915,.T.);
#6072=EDGE_CURVE('',#4877,#4879,#916,.T.);
#6073=EDGE_CURVE('',#4880,#4881,#2588,.T.);
#6074=EDGE_CURVE('',#4880,#4878,#917,.T.);
#6075=EDGE_CURVE('',#4879,#4881,#918,.T.);
#6076=EDGE_CURVE('',#4882,#4883,#2589,.T.);
#6077=EDGE_CURVE('',#4882,#4880,#919,.T.);
#6078=EDGE_CURVE('',#4881,#4883,#920,.T.);
#6079=EDGE_CURVE('',#4884,#4885,#2590,.T.);
#6080=EDGE_CURVE('',#4884,#4882,#921,.T.);
#6081=EDGE_CURVE('',#4883,#4885,#922,.T.);
#6082=EDGE_CURVE('',#4886,#4887,#2591,.T.);
#6083=EDGE_CURVE('',#4886,#4884,#923,.T.);
#6084=EDGE_CURVE('',#4885,#4887,#924,.T.);
#6085=EDGE_CURVE('',#4888,#4889,#2592,.T.);
#6086=EDGE_CURVE('',#4888,#4886,#925,.T.);
#6087=EDGE_CURVE('',#4887,#4889,#926,.T.);
#6088=EDGE_CURVE('',#4890,#4891,#2593,.T.);
#6089=EDGE_CURVE('',#4890,#4888,#927,.T.);
#6090=EDGE_CURVE('',#4889,#4891,#928,.T.);
#6091=EDGE_CURVE('',#4892,#4893,#2594,.T.);
#6092=EDGE_CURVE('',#4892,#4890,#929,.T.);
#6093=EDGE_CURVE('',#4891,#4893,#930,.T.);
#6094=EDGE_CURVE('',#4894,#4895,#2595,.T.);
#6095=EDGE_CURVE('',#4896,#4895,#4316,.T.);
#6096=EDGE_CURVE('',#4896,#4894,#931,.T.);
#6097=EDGE_CURVE('',#4897,#4898,#2596,.T.);
#6098=EDGE_CURVE('',#4899,#4898,#932,.F.);
#6099=EDGE_CURVE('',#4895,#4899,#4317,.T.);
#6100=EDGE_CURVE('',#4894,#4897,#933,.T.);
#6101=EDGE_CURVE('',#4900,#4901,#2597,.T.);
#6102=EDGE_CURVE('',#4898,#4901,#934,.F.);
#6103=EDGE_CURVE('',#4897,#4900,#935,.T.);
#6104=EDGE_CURVE('',#4902,#4903,#2598,.T.);
#6105=EDGE_CURVE('',#4901,#4903,#936,.F.);
#6106=EDGE_CURVE('',#4900,#4902,#937,.T.);
#6107=EDGE_CURVE('',#4904,#4905,#2599,.T.);
#6108=EDGE_CURVE('',#4903,#4905,#938,.F.);
#6109=EDGE_CURVE('',#4902,#4904,#939,.T.);
#6110=EDGE_CURVE('',#4906,#4907,#2600,.T.);
#6111=EDGE_CURVE('',#4905,#4907,#940,.F.);
#6112=EDGE_CURVE('',#4904,#4906,#941,.T.);
#6113=EDGE_CURVE('',#4908,#4909,#2601,.T.);
#6114=EDGE_CURVE('',#4908,#4910,#942,.T.);
#6115=EDGE_CURVE('',#4911,#4910,#2602,.T.);
#6116=EDGE_CURVE('',#4909,#4911,#943,.F.);
#6117=EDGE_CURVE('',#4912,#4913,#2603,.T.);
#6118=EDGE_CURVE('',#4914,#4913,#4318,.T.);
#6119=EDGE_CURVE('',#4914,#4912,#944,.T.);
#6120=EDGE_CURVE('',#4915,#4916,#2604,.T.);
#6121=EDGE_CURVE('',#4917,#4916,#945,.F.);
#6122=EDGE_CURVE('',#4913,#4917,#4319,.T.);
#6123=EDGE_CURVE('',#4912,#4915,#946,.T.);
#6124=EDGE_CURVE('',#4918,#4919,#2605,.T.);
#6125=EDGE_CURVE('',#4916,#4919,#947,.F.);
#6126=EDGE_CURVE('',#4915,#4918,#948,.T.);
#6127=EDGE_CURVE('',#4920,#4921,#2606,.T.);
#6128=EDGE_CURVE('',#4919,#4921,#949,.F.);
#6129=EDGE_CURVE('',#4918,#4920,#950,.T.);
#6130=EDGE_CURVE('',#4922,#4923,#2607,.T.);
#6131=EDGE_CURVE('',#4921,#4923,#951,.F.);
#6132=EDGE_CURVE('',#4920,#4922,#952,.T.);
#6133=EDGE_CURVE('',#4924,#4925,#2608,.T.);
#6134=EDGE_CURVE('',#4923,#4925,#953,.F.);
#6135=EDGE_CURVE('',#4922,#4924,#954,.T.);
#6136=EDGE_CURVE('',#4926,#4927,#2609,.T.);
#6137=EDGE_CURVE('',#4926,#4928,#955,.T.);
#6138=EDGE_CURVE('',#4929,#4928,#2610,.T.);
#6139=EDGE_CURVE('',#4927,#4929,#956,.F.);
#6140=EDGE_CURVE('',#4930,#4931,#2611,.T.);
#6141=EDGE_CURVE('',#4932,#4931,#4320,.T.);
#6142=EDGE_CURVE('',#4932,#4930,#957,.T.);
#6143=EDGE_CURVE('',#4933,#4934,#2612,.T.);
#6144=EDGE_CURVE('',#4935,#4934,#958,.F.);
#6145=EDGE_CURVE('',#4931,#4935,#4321,.T.);
#6146=EDGE_CURVE('',#4930,#4933,#959,.T.);
#6147=EDGE_CURVE('',#4936,#4937,#2613,.T.);
#6148=EDGE_CURVE('',#4934,#4937,#960,.F.);
#6149=EDGE_CURVE('',#4933,#4936,#961,.T.);
#6150=EDGE_CURVE('',#4938,#4939,#2614,.T.);
#6151=EDGE_CURVE('',#4937,#4939,#962,.F.);
#6152=EDGE_CURVE('',#4936,#4938,#963,.T.);
#6153=EDGE_CURVE('',#4940,#4941,#2615,.T.);
#6154=EDGE_CURVE('',#4939,#4941,#964,.F.);
#6155=EDGE_CURVE('',#4938,#4940,#965,.T.);
#6156=EDGE_CURVE('',#4942,#4943,#2616,.T.);
#6157=EDGE_CURVE('',#4941,#4943,#966,.F.);
#6158=EDGE_CURVE('',#4940,#4942,#967,.T.);
#6159=EDGE_CURVE('',#4944,#4945,#2617,.T.);
#6160=EDGE_CURVE('',#4944,#4946,#968,.T.);
#6161=EDGE_CURVE('',#4947,#4946,#2618,.T.);
#6162=EDGE_CURVE('',#4945,#4947,#969,.F.);
#6163=EDGE_CURVE('',#4948,#4949,#2619,.T.);
#6164=EDGE_CURVE('',#4950,#4949,#4322,.T.);
#6165=EDGE_CURVE('',#4950,#4948,#970,.T.);
#6166=EDGE_CURVE('',#4951,#4952,#2620,.T.);
#6167=EDGE_CURVE('',#4953,#4952,#971,.F.);
#6168=EDGE_CURVE('',#4949,#4953,#4323,.T.);
#6169=EDGE_CURVE('',#4948,#4951,#972,.T.);
#6170=EDGE_CURVE('',#4954,#4955,#2621,.T.);
#6171=EDGE_CURVE('',#4952,#4955,#973,.F.);
#6172=EDGE_CURVE('',#4951,#4954,#974,.T.);
#6173=EDGE_CURVE('',#4956,#4957,#2622,.T.);
#6174=EDGE_CURVE('',#4955,#4957,#975,.F.);
#6175=EDGE_CURVE('',#4954,#4956,#976,.T.);
#6176=EDGE_CURVE('',#4958,#4959,#2623,.T.);
#6177=EDGE_CURVE('',#4957,#4959,#977,.F.);
#6178=EDGE_CURVE('',#4956,#4958,#978,.T.);
#6179=EDGE_CURVE('',#4960,#4961,#2624,.T.);
#6180=EDGE_CURVE('',#4959,#4961,#979,.F.);
#6181=EDGE_CURVE('',#4958,#4960,#980,.T.);
#6182=EDGE_CURVE('',#4962,#4963,#2625,.T.);
#6183=EDGE_CURVE('',#4962,#4964,#981,.T.);
#6184=EDGE_CURVE('',#4965,#4964,#2626,.T.);
#6185=EDGE_CURVE('',#4963,#4965,#982,.F.);
#6186=EDGE_CURVE('',#4961,#4963,#983,.F.);
#6187=EDGE_CURVE('',#4960,#4962,#984,.T.);
#6188=EDGE_CURVE('',#4943,#4945,#985,.F.);
#6189=EDGE_CURVE('',#4942,#4944,#986,.T.);
#6190=EDGE_CURVE('',#4925,#4927,#987,.F.);
#6191=EDGE_CURVE('',#4924,#4926,#988,.T.);
#6192=EDGE_CURVE('',#4907,#4909,#989,.F.);
#6193=EDGE_CURVE('',#4906,#4908,#990,.T.);
#6194=EDGE_CURVE('',#4893,#4966,#991,.T.);
#6195=EDGE_CURVE('',#4967,#4966,#4324,.T.);
#6196=EDGE_CURVE('',#4967,#4892,#992,.T.);
#6197=EDGE_CURVE('',#4855,#4968,#993,.T.);
#6198=EDGE_CURVE('',#4969,#4968,#4325,.T.);
#6199=EDGE_CURVE('',#4969,#4854,#994,.T.);
#6200=EDGE_CURVE('',#4816,#4970,#995,.T.);
#6201=EDGE_CURVE('',#4971,#4970,#4326,.T.);
#6202=EDGE_CURVE('',#4971,#4815,#996,.T.);
#6203=EDGE_CURVE('',#4776,#4972,#997,.T.);
#6204=EDGE_CURVE('',#4973,#4972,#4327,.T.);
#6205=EDGE_CURVE('',#4973,#4775,#998,.T.);
#6206=EDGE_CURVE('',#4974,#4974,#4328,.T.);
#6207=EDGE_CURVE('',#4974,#4975,#2627,.T.);
#6208=EDGE_CURVE('',#4975,#4975,#4329,.T.);
#6209=EDGE_CURVE('',#4976,#4976,#4330,.T.);
#6210=EDGE_CURVE('',#4976,#4977,#2628,.T.);
#6211=EDGE_CURVE('',#4977,#4977,#4331,.T.);
#6212=EDGE_CURVE('',#4978,#4978,#4332,.T.);
#6213=EDGE_CURVE('',#4978,#4979,#2629,.T.);
#6214=EDGE_CURVE('',#4979,#4979,#4333,.T.);
#6215=EDGE_CURVE('',#4979,#4980,#2630,.T.);
#6216=EDGE_CURVE('',#4980,#4980,#4334,.T.);
#6217=EDGE_CURVE('',#4740,#4981,#999,.T.);
#6218=EDGE_CURVE('',#4982,#4739,#1000,.T.);
#6219=EDGE_CURVE('',#4983,#4982,#4335,.T.);
#6220=EDGE_CURVE('',#4981,#4983,#1001,.T.);
#6221=EDGE_CURVE('',#4981,#4984,#2631,.T.);
#6222=EDGE_CURVE('',#4984,#4984,#4336,.T.);
#6223=EDGE_CURVE('',#4780,#4985,#1002,.T.);
#6224=EDGE_CURVE('',#4986,#4779,#1003,.T.);
#6225=EDGE_CURVE('',#4987,#4986,#4337,.T.);
#6226=EDGE_CURVE('',#4985,#4987,#1004,.T.);
#6227=EDGE_CURVE('',#4985,#4988,#2632,.T.);
#6228=EDGE_CURVE('',#4988,#4988,#4338,.T.);
#6229=EDGE_CURVE('',#4818,#4989,#1005,.T.);
#6230=EDGE_CURVE('',#4990,#4819,#1006,.T.);
#6231=EDGE_CURVE('',#4991,#4990,#4339,.T.);
#6232=EDGE_CURVE('',#4989,#4991,#1007,.T.);
#6233=EDGE_CURVE('',#4989,#4992,#2633,.T.);
#6234=EDGE_CURVE('',#4992,#4992,#4340,.T.);
#6235=EDGE_CURVE('',#4859,#4993,#1008,.T.);
#6236=EDGE_CURVE('',#4994,#4858,#1009,.T.);
#6237=EDGE_CURVE('',#4995,#4994,#4341,.T.);
#6238=EDGE_CURVE('',#4993,#4995,#1010,.T.);
#6239=EDGE_CURVE('',#4993,#4996,#2634,.T.);
#6240=EDGE_CURVE('',#4996,#4996,#4342,.T.);
#6241=EDGE_CURVE('',#4966,#4896,#4343,.T.);
#6242=EDGE_CURVE('',#4995,#4997,#265,.T.);
#6243=EDGE_CURVE('',#4910,#4997,#2635,.T.);
#6244=EDGE_CURVE('',#4899,#4967,#4344,.T.);
#6245=EDGE_CURVE('',#4998,#4911,#2636,.T.);
#6246=EDGE_CURVE('',#4994,#4998,#266,.T.);
#6247=EDGE_CURVE('',#4997,#4998,#2637,.T.);
#6248=EDGE_CURVE('',#4999,#5000,#2638,.T.);
#6249=EDGE_CURVE('',#5001,#4999,#2639,.T.);
#6250=EDGE_CURVE('',#5002,#5001,#2640,.T.);
#6251=EDGE_CURVE('',#5003,#5002,#2641,.T.);
#6252=EDGE_CURVE('',#5003,#5004,#2642,.T.);
#6253=EDGE_CURVE('',#5005,#5004,#2643,.T.);
#6254=EDGE_CURVE('',#5006,#5005,#2644,.T.);
#6255=EDGE_CURVE('',#5000,#5006,#2645,.T.);
#6256=EDGE_CURVE('',#4972,#4950,#4345,.T.);
#6257=EDGE_CURVE('',#4953,#4973,#4346,.T.);
#6258=EDGE_CURVE('',#4970,#4932,#4347,.T.);
#6259=EDGE_CURVE('',#4935,#4971,#4348,.T.);
#6260=EDGE_CURVE('',#4968,#4914,#4349,.T.);
#6261=EDGE_CURVE('',#4917,#4969,#4350,.T.);
#6262=EDGE_CURVE('',#4991,#5007,#267,.T.);
#6263=EDGE_CURVE('',#4928,#5007,#2646,.T.);
#6264=EDGE_CURVE('',#5008,#4929,#2647,.T.);
#6265=EDGE_CURVE('',#4990,#5008,#268,.T.);
#6266=EDGE_CURVE('',#5007,#5008,#2648,.T.);
#6267=EDGE_CURVE('',#4987,#5009,#269,.T.);
#6268=EDGE_CURVE('',#4946,#5009,#2649,.T.);
#6269=EDGE_CURVE('',#5010,#4947,#2650,.T.);
#6270=EDGE_CURVE('',#4986,#5010,#270,.T.);
#6271=EDGE_CURVE('',#5009,#5010,#2651,.T.);
#6272=EDGE_CURVE('',#4983,#5011,#271,.T.);
#6273=EDGE_CURVE('',#4964,#5011,#2652,.T.);
#6274=EDGE_CURVE('',#5012,#4965,#2653,.T.);
#6275=EDGE_CURVE('',#4982,#5012,#272,.T.);
#6276=EDGE_CURVE('',#5011,#5012,#2654,.T.);
#6277=EDGE_CURVE('',#5013,#5006,#2655,.T.);
#6278=EDGE_CURVE('',#5013,#5014,#2656,.T.);
#6279=EDGE_CURVE('',#5014,#5000,#2657,.T.);
#6280=EDGE_CURVE('',#5015,#5005,#2658,.T.);
#6281=EDGE_CURVE('',#5015,#5013,#2659,.T.);
#6282=EDGE_CURVE('',#5013,#5016,#746,.T.);
#6283=EDGE_CURVE('',#5017,#5016,#2660,.T.);
#6284=EDGE_CURVE('',#5014,#5017,#747,.T.);
#6285=EDGE_CURVE('',#5014,#5018,#2661,.T.);
#6286=EDGE_CURVE('',#5018,#4999,#2662,.T.);
#6287=EDGE_CURVE('',#5019,#5004,#2663,.T.);
#6288=EDGE_CURVE('',#5019,#5015,#2664,.T.);
#6289=EDGE_CURVE('',#5015,#5020,#748,.T.);
#6290=EDGE_CURVE('',#5016,#5020,#2665,.T.);
#6291=EDGE_CURVE('',#5021,#5003,#2666,.T.);
#6292=EDGE_CURVE('',#5021,#5019,#2667,.T.);
#6293=EDGE_CURVE('',#5022,#5019,#749,.T.);
#6294=EDGE_CURVE('',#5020,#5022,#2668,.T.);
#6295=EDGE_CURVE('',#5023,#5002,#2669,.T.);
#6296=EDGE_CURVE('',#5023,#5021,#2670,.T.);
#6297=EDGE_CURVE('',#5024,#5021,#750,.T.);
#6298=EDGE_CURVE('',#5022,#5024,#2671,.T.);
#6299=EDGE_CURVE('',#5025,#5001,#2672,.T.);
#6300=EDGE_CURVE('',#5025,#5023,#2673,.T.);
#6301=EDGE_CURVE('',#5026,#5023,#751,.T.);
#6302=EDGE_CURVE('',#5024,#5026,#2674,.T.);
#6303=EDGE_CURVE('',#5018,#5025,#2675,.T.);
#6304=EDGE_CURVE('',#5027,#5025,#752,.T.);
#6305=EDGE_CURVE('',#5026,#5027,#2676,.T.);
#6306=EDGE_CURVE('',#5018,#5028,#753,.T.);
#6307=EDGE_CURVE('',#5027,#5028,#2677,.T.);
#6308=EDGE_CURVE('',#5028,#5017,#2678,.T.);
#6309=EDGE_CURVE('',#5029,#5030,#2679,.T.);
#6310=EDGE_CURVE('',#5031,#5029,#4351,.T.);
#6311=EDGE_CURVE('',#5032,#5031,#273,.T.);
#6312=EDGE_CURVE('',#5030,#5032,#4352,.T.);
#6313=EDGE_CURVE('',#5032,#5030,#4353,.T.);
#6314=EDGE_CURVE('',#5033,#5032,#274,.T.);
#6315=EDGE_CURVE('',#5029,#5033,#4354,.T.);
#6316=EDGE_CURVE('',#5034,#5035,#2680,.T.);
#6317=EDGE_CURVE('',#5035,#5035,#4355,.T.);
#6318=EDGE_CURVE('',#5036,#5036,#4356,.T.);
#6319=EDGE_CURVE('',#5036,#5029,#2681,.T.);
#6320=EDGE_CURVE('',#5033,#5037,#2682,.T.);
#6321=EDGE_CURVE('',#5037,#5038,#4357,.T.);
#6322=EDGE_CURVE('',#5038,#5031,#2683,.T.);
#6323=EDGE_CURVE('',#5037,#5038,#2684,.T.);
#6324=EDGE_CURVE('',#5039,#5039,#4358,.T.);
#6325=EDGE_CURVE('',#5039,#5040,#2685,.T.);
#6326=EDGE_CURVE('',#5040,#5040,#4359,.T.);
#6327=EDGE_CURVE('',#5041,#5041,#4360,.T.);
#6328=EDGE_CURVE('',#5041,#5042,#2686,.T.);
#6329=EDGE_CURVE('',#5042,#5042,#4361,.T.);
#6330=EDGE_CURVE('',#5043,#5043,#4362,.T.);
#6331=EDGE_CURVE('',#5043,#5044,#2687,.T.);
#6332=EDGE_CURVE('',#5044,#5044,#4363,.T.);
#6333=EDGE_CURVE('',#5045,#5045,#4364,.T.);
#6334=EDGE_CURVE('',#5045,#5046,#2688,.T.);
#6335=EDGE_CURVE('',#5046,#5046,#4365,.T.);
#6336=EDGE_CURVE('',#5047,#5047,#4366,.T.);
#6337=EDGE_CURVE('',#5047,#5048,#2689,.T.);
#6338=EDGE_CURVE('',#5048,#5048,#4367,.T.);
#6339=EDGE_CURVE('',#5049,#5049,#4368,.T.);
#6340=EDGE_CURVE('',#5049,#5041,#2690,.T.);
#6341=EDGE_CURVE('',#5050,#5050,#4369,.T.);
#6342=EDGE_CURVE('',#5050,#5043,#2691,.T.);
#6343=EDGE_CURVE('',#5051,#5051,#4370,.T.);
#6344=EDGE_CURVE('',#5051,#5045,#2692,.T.);
#6345=EDGE_CURVE('',#5052,#5052,#4371,.T.);
#6346=EDGE_CURVE('',#5052,#5047,#2693,.T.);
#6347=EDGE_CURVE('',#5053,#5053,#4372,.T.);
#6348=EDGE_CURVE('',#5053,#5054,#2694,.T.);
#6349=EDGE_CURVE('',#5054,#5054,#4373,.T.);
#6350=EDGE_CURVE('',#5055,#5056,#2695,.T.);
#6351=EDGE_CURVE('',#5056,#5057,#2696,.T.);
#6352=EDGE_CURVE('',#5057,#5058,#2697,.T.);
#6353=EDGE_CURVE('',#5058,#5055,#2698,.T.);
#6354=EDGE_CURVE('',#5059,#5060,#2699,.T.);
#6355=EDGE_CURVE('',#5058,#5060,#2700,.T.);
#6356=EDGE_CURVE('',#5057,#5059,#2701,.T.);
#6357=EDGE_CURVE('',#5060,#5061,#2702,.T.);
#6358=EDGE_CURVE('',#5055,#5061,#2703,.T.);
#6359=EDGE_CURVE('',#5061,#5062,#2704,.T.);
#6360=EDGE_CURVE('',#5056,#5062,#2705,.T.);
#6361=EDGE_CURVE('',#5062,#5059,#2706,.T.);
#6362=EDGE_CURVE('',#5063,#5064,#2707,.T.);
#6363=EDGE_CURVE('',#5064,#5065,#2708,.T.);
#6364=EDGE_CURVE('',#5065,#5066,#2709,.T.);
#6365=EDGE_CURVE('',#5066,#5063,#2710,.T.);
#6366=EDGE_CURVE('',#5064,#5067,#2711,.T.);
#6367=EDGE_CURVE('',#5067,#5068,#2712,.T.);
#6368=EDGE_CURVE('',#5065,#5068,#2713,.T.);
#6369=EDGE_CURVE('',#5069,#5070,#2714,.T.);
#6370=EDGE_CURVE('',#5070,#5071,#2715,.T.);
#6371=EDGE_CURVE('',#5071,#5072,#2716,.T.);
#6372=EDGE_CURVE('',#5072,#5073,#2717,.T.);
#6373=EDGE_CURVE('',#5073,#5074,#2718,.T.);
#6374=EDGE_CURVE('',#5074,#5075,#2719,.T.);
#6375=EDGE_CURVE('',#5075,#5076,#2720,.T.);
#6376=EDGE_CURVE('',#5076,#5069,#2721,.T.);
#6377=EDGE_CURVE('',#5077,#5073,#754,.T.);
#6378=EDGE_CURVE('',#5078,#5072,#755,.T.);
#6379=EDGE_CURVE('',#5077,#5078,#2722,.T.);
#6380=EDGE_CURVE('',#5079,#5071,#756,.T.);
#6381=EDGE_CURVE('',#5078,#5079,#2723,.T.);
#6382=EDGE_CURVE('',#5070,#5080,#757,.T.);
#6383=EDGE_CURVE('',#5079,#5080,#2724,.T.);
#6384=EDGE_CURVE('',#5081,#5078,#2725,.T.);
#6385=EDGE_CURVE('',#5082,#5079,#2726,.T.);
#6386=EDGE_CURVE('',#5081,#5082,#2727,.T.);
#6387=EDGE_CURVE('',#5069,#5083,#758,.T.);
#6388=EDGE_CURVE('',#5080,#5083,#2728,.T.);
#6389=EDGE_CURVE('',#5084,#5080,#2729,.T.);
#6390=EDGE_CURVE('',#5082,#5084,#2730,.T.);
#6391=EDGE_CURVE('',#5076,#5085,#759,.T.);
#6392=EDGE_CURVE('',#5083,#5085,#2731,.T.);
#6393=EDGE_CURVE('',#5086,#5083,#2732,.T.);
#6394=EDGE_CURVE('',#5086,#5084,#2733,.T.);
#6395=EDGE_CURVE('',#5075,#5087,#760,.T.);
#6396=EDGE_CURVE('',#5085,#5087,#2734,.T.);
#6397=EDGE_CURVE('',#5088,#5085,#2735,.T.);
#6398=EDGE_CURVE('',#5086,#5088,#2736,.T.);
#6399=EDGE_CURVE('',#5089,#5074,#761,.T.);
#6400=EDGE_CURVE('',#5087,#5089,#2737,.T.);
#6401=EDGE_CURVE('',#5090,#5087,#2738,.T.);
#6402=EDGE_CURVE('',#5088,#5090,#2739,.T.);
#6403=EDGE_CURVE('',#5091,#5077,#2740,.T.);
#6404=EDGE_CURVE('',#5091,#5081,#2741,.T.);
#6405=EDGE_CURVE('',#5068,#5092,#4374,.T.);
#6406=EDGE_CURVE('',#5092,#5093,#2742,.T.);
#6407=EDGE_CURVE('',#5066,#5093,#2743,.T.);
#6408=EDGE_CURVE('',#5093,#5094,#2744,.T.);
#6409=EDGE_CURVE('',#5063,#5094,#2745,.T.);
#6410=EDGE_CURVE('',#5094,#5095,#2746,.T.);
#6411=EDGE_CURVE('',#5095,#5067,#4375,.T.);
#6412=EDGE_CURVE('',#5092,#5077,#2747,.T.);
#6413=EDGE_CURVE('',#5089,#5095,#2748,.T.);
#6414=EDGE_CURVE('',#5096,#5089,#2749,.T.);
#6415=EDGE_CURVE('',#5090,#5096,#2750,.T.);
#6416=EDGE_CURVE('',#5096,#5091,#2751,.T.);
#6417=EDGE_CURVE('',#5097,#5097,#4376,.T.);
#6418=EDGE_CURVE('',#5097,#5098,#2752,.T.);
#6419=EDGE_CURVE('',#5098,#5098,#4377,.T.);
#6420=EDGE_CURVE('',#5099,#5099,#4378,.T.);
#6421=EDGE_CURVE('',#5099,#5100,#2753,.T.);
#6422=EDGE_CURVE('',#5100,#5100,#4379,.T.);
#6423=EDGE_CURVE('',#5101,#5101,#4380,.T.);
#6424=EDGE_CURVE('',#5101,#5102,#2754,.T.);
#6425=EDGE_CURVE('',#5102,#5102,#4381,.T.);
#6426=EDGE_CURVE('',#5103,#5103,#4382,.T.);
#6427=EDGE_CURVE('',#5103,#5104,#2755,.T.);
#6428=EDGE_CURVE('',#5104,#5104,#4383,.T.);
#6429=EDGE_CURVE('',#5105,#5105,#4384,.T.);
#6430=EDGE_CURVE('',#5105,#5106,#2756,.T.);
#6431=EDGE_CURVE('',#5106,#5106,#4385,.T.);
#6432=EDGE_CURVE('',#5107,#5108,#2757,.T.);
#6433=EDGE_CURVE('',#5108,#5109,#2758,.T.);
#6434=EDGE_CURVE('',#5110,#5109,#2759,.T.);
#6435=EDGE_CURVE('',#5111,#5110,#2760,.T.);
#6436=EDGE_CURVE('',#5112,#5111,#2761,.T.);
#6437=EDGE_CURVE('',#5112,#5113,#2762,.T.);
#6438=EDGE_CURVE('',#5113,#5114,#2763,.T.);
#6439=EDGE_CURVE('',#5114,#5107,#2764,.T.);
#6440=EDGE_CURVE('',#5115,#5116,#2765,.T.);
#6441=EDGE_CURVE('',#5117,#5115,#2766,.T.);
#6442=EDGE_CURVE('',#5118,#5117,#2767,.T.);
#6443=EDGE_CURVE('',#5119,#5118,#2768,.T.);
#6444=EDGE_CURVE('',#5119,#5120,#2769,.T.);
#6445=EDGE_CURVE('',#5120,#5121,#2770,.T.);
#6446=EDGE_CURVE('',#5121,#5122,#2771,.T.);
#6447=EDGE_CURVE('',#5116,#5122,#2772,.T.);
#6448=EDGE_CURVE('',#5107,#5115,#2773,.T.);
#6449=EDGE_CURVE('',#5114,#5117,#2774,.T.);
#6450=EDGE_CURVE('',#5108,#5116,#2775,.T.);
#6451=EDGE_CURVE('',#5113,#5118,#2776,.T.);
#6452=EDGE_CURVE('',#5110,#5121,#2777,.T.);
#6453=EDGE_CURVE('',#5109,#5122,#2778,.T.);
#6454=EDGE_CURVE('',#5112,#5119,#2779,.T.);
#6455=EDGE_CURVE('',#5111,#5120,#2780,.T.);
#7238=ORIENTED_EDGE('',*,*,#5650,.T.);
#7239=ORIENTED_EDGE('',*,*,#5651,.T.);
#7240=ORIENTED_EDGE('',*,*,#5652,.T.);
#7241=ORIENTED_EDGE('',*,*,#5653,.T.);
#7242=ORIENTED_EDGE('',*,*,#5651,.F.);
#7243=ORIENTED_EDGE('',*,*,#5654,.T.);
#7244=ORIENTED_EDGE('',*,*,#5655,.T.);
#7245=ORIENTED_EDGE('',*,*,#5652,.F.);
#7246=ORIENTED_EDGE('',*,*,#5653,.F.);
#7247=ORIENTED_EDGE('',*,*,#5655,.F.);
#7248=ORIENTED_EDGE('',*,*,#5656,.T.);
#7249=ORIENTED_EDGE('',*,*,#5657,.T.);
#7250=ORIENTED_EDGE('',*,*,#5658,.F.);
#7251=ORIENTED_EDGE('',*,*,#5659,.F.);
#7252=ORIENTED_EDGE('',*,*,#5660,.T.);
#7253=ORIENTED_EDGE('',*,*,#5661,.T.);
#7254=ORIENTED_EDGE('',*,*,#5662,.F.);
#7255=ORIENTED_EDGE('',*,*,#5663,.T.);
#7256=ORIENTED_EDGE('',*,*,#5664,.T.);
#7257=ORIENTED_EDGE('',*,*,#5665,.F.);
#7258=ORIENTED_EDGE('',*,*,#5666,.F.);
#7259=ORIENTED_EDGE('',*,*,#5667,.T.);
#7260=ORIENTED_EDGE('',*,*,#5668,.T.);
#7261=ORIENTED_EDGE('',*,*,#5669,.F.);
#7262=ORIENTED_EDGE('',*,*,#5670,.F.);
#7263=ORIENTED_EDGE('',*,*,#5671,.F.);
#7264=ORIENTED_EDGE('',*,*,#5662,.T.);
#7265=ORIENTED_EDGE('',*,*,#5672,.T.);
#7266=ORIENTED_EDGE('',*,*,#5673,.T.);
#7267=ORIENTED_EDGE('',*,*,#5674,.F.);
#7268=ORIENTED_EDGE('',*,*,#5675,.T.);
#7269=ORIENTED_EDGE('',*,*,#5666,.T.);
#7270=ORIENTED_EDGE('',*,*,#5676,.F.);
#7271=ORIENTED_EDGE('',*,*,#5677,.F.);
#7272=ORIENTED_EDGE('',*,*,#5670,.T.);
#7273=ORIENTED_EDGE('',*,*,#5650,.F.);
#7274=ORIENTED_EDGE('',*,*,#5678,.F.);
#7275=ORIENTED_EDGE('',*,*,#5658,.T.);
#7276=ORIENTED_EDGE('',*,*,#5679,.T.);
#7277=ORIENTED_EDGE('',*,*,#5659,.T.);
#7278=ORIENTED_EDGE('',*,*,#5678,.T.);
#7279=ORIENTED_EDGE('',*,*,#5680,.F.);
#7280=ORIENTED_EDGE('',*,*,#5681,.F.);
#7281=ORIENTED_EDGE('',*,*,#5682,.T.);
#7282=ORIENTED_EDGE('',*,*,#5683,.F.);
#7283=ORIENTED_EDGE('',*,*,#5684,.T.);
#7284=ORIENTED_EDGE('',*,*,#5685,.T.);
#7285=ORIENTED_EDGE('',*,*,#5672,.F.);
#7286=ORIENTED_EDGE('',*,*,#5661,.F.);
#7287=ORIENTED_EDGE('',*,*,#5669,.T.);
#7288=ORIENTED_EDGE('',*,*,#5686,.F.);
#7289=ORIENTED_EDGE('',*,*,#5687,.F.);
#7290=ORIENTED_EDGE('',*,*,#5688,.T.);
#7291=ORIENTED_EDGE('',*,*,#5676,.T.);
#7292=ORIENTED_EDGE('',*,*,#5682,.F.);
#7293=ORIENTED_EDGE('',*,*,#5689,.T.);
#7294=ORIENTED_EDGE('',*,*,#5683,.T.);
#7295=ORIENTED_EDGE('',*,*,#5660,.F.);
#7296=ORIENTED_EDGE('',*,*,#5675,.F.);
#7297=ORIENTED_EDGE('',*,*,#5690,.F.);
#7298=ORIENTED_EDGE('',*,*,#5691,.T.);
#7299=ORIENTED_EDGE('',*,*,#5692,.T.);
#7300=ORIENTED_EDGE('',*,*,#5667,.F.);
#7301=ORIENTED_EDGE('',*,*,#5692,.F.);
#7302=ORIENTED_EDGE('',*,*,#5693,.T.);
#7303=ORIENTED_EDGE('',*,*,#5686,.T.);
#7304=ORIENTED_EDGE('',*,*,#5668,.F.);
#7305=ORIENTED_EDGE('',*,*,#5687,.T.);
#7306=ORIENTED_EDGE('',*,*,#5693,.F.);
#7307=ORIENTED_EDGE('',*,*,#5691,.F.);
#7308=ORIENTED_EDGE('',*,*,#5694,.T.);
#7309=ORIENTED_EDGE('',*,*,#5695,.F.);
#7310=ORIENTED_EDGE('',*,*,#5696,.F.);
#7311=ORIENTED_EDGE('',*,*,#5684,.F.);
#7312=ORIENTED_EDGE('',*,*,#5689,.F.);
#7313=ORIENTED_EDGE('',*,*,#5681,.T.);
#7314=ORIENTED_EDGE('',*,*,#5697,.F.);
#7315=ORIENTED_EDGE('',*,*,#5698,.F.);
#7316=ORIENTED_EDGE('',*,*,#5699,.T.);
#7317=ORIENTED_EDGE('',*,*,#5700,.F.);
#7318=ORIENTED_EDGE('',*,*,#5695,.T.);
#7319=ORIENTED_EDGE('',*,*,#5701,.T.);
#7320=ORIENTED_EDGE('',*,*,#5664,.F.);
#7321=ORIENTED_EDGE('',*,*,#5673,.F.);
#7322=ORIENTED_EDGE('',*,*,#5685,.F.);
#7323=ORIENTED_EDGE('',*,*,#5696,.T.);
#7324=ORIENTED_EDGE('',*,*,#5700,.T.);
#7325=ORIENTED_EDGE('',*,*,#5663,.F.);
#7326=ORIENTED_EDGE('',*,*,#5665,.T.);
#7327=ORIENTED_EDGE('',*,*,#5701,.F.);
#7328=ORIENTED_EDGE('',*,*,#5694,.F.);
#7329=ORIENTED_EDGE('',*,*,#5690,.T.);
#7330=ORIENTED_EDGE('',*,*,#5674,.T.);
#7331=ORIENTED_EDGE('',*,*,#5671,.T.);
#7332=ORIENTED_EDGE('',*,*,#5677,.T.);
#7333=ORIENTED_EDGE('',*,*,#5688,.F.);
#7334=ORIENTED_EDGE('',*,*,#5699,.F.);
#7335=ORIENTED_EDGE('',*,*,#5702,.T.);
#7336=ORIENTED_EDGE('',*,*,#5702,.F.);
#7337=ORIENTED_EDGE('',*,*,#5698,.T.);
#7338=ORIENTED_EDGE('',*,*,#5703,.T.);
#7339=ORIENTED_EDGE('',*,*,#5656,.F.);
#7340=ORIENTED_EDGE('',*,*,#5654,.F.);
#7341=ORIENTED_EDGE('',*,*,#5703,.F.);
#7342=ORIENTED_EDGE('',*,*,#5697,.T.);
#7343=ORIENTED_EDGE('',*,*,#5680,.T.);
#7344=ORIENTED_EDGE('',*,*,#5679,.F.);
#7345=ORIENTED_EDGE('',*,*,#5657,.F.);
#7346=ORIENTED_EDGE('',*,*,#5704,.T.);
#7347=ORIENTED_EDGE('',*,*,#5705,.T.);
#7348=ORIENTED_EDGE('',*,*,#5706,.T.);
#7349=ORIENTED_EDGE('',*,*,#5707,.T.);
#7350=ORIENTED_EDGE('',*,*,#5705,.F.);
#7351=ORIENTED_EDGE('',*,*,#5708,.T.);
#7352=ORIENTED_EDGE('',*,*,#5709,.T.);
#7353=ORIENTED_EDGE('',*,*,#5706,.F.);
#7354=ORIENTED_EDGE('',*,*,#5707,.F.);
#7355=ORIENTED_EDGE('',*,*,#5709,.F.);
#7356=ORIENTED_EDGE('',*,*,#5710,.T.);
#7357=ORIENTED_EDGE('',*,*,#5711,.T.);
#7358=ORIENTED_EDGE('',*,*,#5712,.F.);
#7359=ORIENTED_EDGE('',*,*,#5713,.F.);
#7360=ORIENTED_EDGE('',*,*,#5714,.T.);
#7361=ORIENTED_EDGE('',*,*,#5715,.T.);
#7362=ORIENTED_EDGE('',*,*,#5716,.F.);
#7363=ORIENTED_EDGE('',*,*,#5717,.T.);
#7364=ORIENTED_EDGE('',*,*,#5718,.T.);
#7365=ORIENTED_EDGE('',*,*,#5719,.F.);
#7366=ORIENTED_EDGE('',*,*,#5720,.F.);
#7367=ORIENTED_EDGE('',*,*,#5721,.T.);
#7368=ORIENTED_EDGE('',*,*,#5722,.T.);
#7369=ORIENTED_EDGE('',*,*,#5723,.F.);
#7370=ORIENTED_EDGE('',*,*,#5724,.F.);
#7371=ORIENTED_EDGE('',*,*,#5725,.F.);
#7372=ORIENTED_EDGE('',*,*,#5716,.T.);
#7373=ORIENTED_EDGE('',*,*,#5726,.T.);
#7374=ORIENTED_EDGE('',*,*,#5727,.T.);
#7375=ORIENTED_EDGE('',*,*,#5728,.F.);
#7376=ORIENTED_EDGE('',*,*,#5729,.T.);
#7377=ORIENTED_EDGE('',*,*,#5720,.T.);
#7378=ORIENTED_EDGE('',*,*,#5730,.F.);
#7379=ORIENTED_EDGE('',*,*,#5731,.F.);
#7380=ORIENTED_EDGE('',*,*,#5724,.T.);
#7381=ORIENTED_EDGE('',*,*,#5704,.F.);
#7382=ORIENTED_EDGE('',*,*,#5732,.F.);
#7383=ORIENTED_EDGE('',*,*,#5712,.T.);
#7384=ORIENTED_EDGE('',*,*,#5733,.T.);
#7385=ORIENTED_EDGE('',*,*,#5713,.T.);
#7386=ORIENTED_EDGE('',*,*,#5732,.T.);
#7387=ORIENTED_EDGE('',*,*,#5734,.F.);
#7388=ORIENTED_EDGE('',*,*,#5735,.F.);
#7389=ORIENTED_EDGE('',*,*,#5736,.T.);
#7390=ORIENTED_EDGE('',*,*,#5737,.F.);
#7391=ORIENTED_EDGE('',*,*,#5738,.T.);
#7392=ORIENTED_EDGE('',*,*,#5739,.T.);
#7393=ORIENTED_EDGE('',*,*,#5726,.F.);
#7394=ORIENTED_EDGE('',*,*,#5715,.F.);
#7395=ORIENTED_EDGE('',*,*,#5723,.T.);
#7396=ORIENTED_EDGE('',*,*,#5740,.F.);
#7397=ORIENTED_EDGE('',*,*,#5741,.F.);
#7398=ORIENTED_EDGE('',*,*,#5742,.T.);
#7399=ORIENTED_EDGE('',*,*,#5730,.T.);
#7400=ORIENTED_EDGE('',*,*,#5736,.F.);
#7401=ORIENTED_EDGE('',*,*,#5743,.T.);
#7402=ORIENTED_EDGE('',*,*,#5737,.T.);
#7403=ORIENTED_EDGE('',*,*,#5714,.F.);
#7404=ORIENTED_EDGE('',*,*,#5729,.F.);
#7405=ORIENTED_EDGE('',*,*,#5744,.F.);
#7406=ORIENTED_EDGE('',*,*,#5745,.T.);
#7407=ORIENTED_EDGE('',*,*,#5746,.T.);
#7408=ORIENTED_EDGE('',*,*,#5721,.F.);
#7409=ORIENTED_EDGE('',*,*,#5746,.F.);
#7410=ORIENTED_EDGE('',*,*,#5747,.T.);
#7411=ORIENTED_EDGE('',*,*,#5740,.T.);
#7412=ORIENTED_EDGE('',*,*,#5722,.F.);
#7413=ORIENTED_EDGE('',*,*,#5741,.T.);
#7414=ORIENTED_EDGE('',*,*,#5747,.F.);
#7415=ORIENTED_EDGE('',*,*,#5745,.F.);
#7416=ORIENTED_EDGE('',*,*,#5748,.T.);
#7417=ORIENTED_EDGE('',*,*,#5749,.F.);
#7418=ORIENTED_EDGE('',*,*,#5750,.F.);
#7419=ORIENTED_EDGE('',*,*,#5738,.F.);
#7420=ORIENTED_EDGE('',*,*,#5743,.F.);
#7421=ORIENTED_EDGE('',*,*,#5735,.T.);
#7422=ORIENTED_EDGE('',*,*,#5751,.F.);
#7423=ORIENTED_EDGE('',*,*,#5752,.F.);
#7424=ORIENTED_EDGE('',*,*,#5753,.T.);
#7425=ORIENTED_EDGE('',*,*,#5754,.F.);
#7426=ORIENTED_EDGE('',*,*,#5749,.T.);
#7427=ORIENTED_EDGE('',*,*,#5755,.T.);
#7428=ORIENTED_EDGE('',*,*,#5718,.F.);
#7429=ORIENTED_EDGE('',*,*,#5727,.F.);
#7430=ORIENTED_EDGE('',*,*,#5739,.F.);
#7431=ORIENTED_EDGE('',*,*,#5750,.T.);
#7432=ORIENTED_EDGE('',*,*,#5754,.T.);
#7433=ORIENTED_EDGE('',*,*,#5717,.F.);
#7434=ORIENTED_EDGE('',*,*,#5719,.T.);
#7435=ORIENTED_EDGE('',*,*,#5755,.F.);
#7436=ORIENTED_EDGE('',*,*,#5748,.F.);
#7437=ORIENTED_EDGE('',*,*,#5744,.T.);
#7438=ORIENTED_EDGE('',*,*,#5728,.T.);
#7439=ORIENTED_EDGE('',*,*,#5725,.T.);
#7440=ORIENTED_EDGE('',*,*,#5731,.T.);
#7441=ORIENTED_EDGE('',*,*,#5742,.F.);
#7442=ORIENTED_EDGE('',*,*,#5753,.F.);
#7443=ORIENTED_EDGE('',*,*,#5756,.T.);
#7444=ORIENTED_EDGE('',*,*,#5756,.F.);
#7445=ORIENTED_EDGE('',*,*,#5752,.T.);
#7446=ORIENTED_EDGE('',*,*,#5757,.T.);
#7447=ORIENTED_EDGE('',*,*,#5710,.F.);
#7448=ORIENTED_EDGE('',*,*,#5708,.F.);
#7449=ORIENTED_EDGE('',*,*,#5757,.F.);
#7450=ORIENTED_EDGE('',*,*,#5751,.T.);
#7451=ORIENTED_EDGE('',*,*,#5734,.T.);
#7452=ORIENTED_EDGE('',*,*,#5733,.F.);
#7453=ORIENTED_EDGE('',*,*,#5711,.F.);
#7454=ORIENTED_EDGE('',*,*,#5758,.T.);
#7455=ORIENTED_EDGE('',*,*,#5759,.T.);
#7456=ORIENTED_EDGE('',*,*,#5760,.T.);
#7457=ORIENTED_EDGE('',*,*,#5761,.T.);
#7458=ORIENTED_EDGE('',*,*,#5759,.F.);
#7459=ORIENTED_EDGE('',*,*,#5762,.T.);
#7460=ORIENTED_EDGE('',*,*,#5763,.T.);
#7461=ORIENTED_EDGE('',*,*,#5760,.F.);
#7462=ORIENTED_EDGE('',*,*,#5761,.F.);
#7463=ORIENTED_EDGE('',*,*,#5763,.F.);
#7464=ORIENTED_EDGE('',*,*,#5764,.T.);
#7465=ORIENTED_EDGE('',*,*,#5765,.T.);
#7466=ORIENTED_EDGE('',*,*,#5766,.F.);
#7467=ORIENTED_EDGE('',*,*,#5767,.F.);
#7468=ORIENTED_EDGE('',*,*,#5768,.T.);
#7469=ORIENTED_EDGE('',*,*,#5769,.T.);
#7470=ORIENTED_EDGE('',*,*,#5770,.F.);
#7471=ORIENTED_EDGE('',*,*,#5771,.T.);
#7472=ORIENTED_EDGE('',*,*,#5772,.T.);
#7473=ORIENTED_EDGE('',*,*,#5773,.F.);
#7474=ORIENTED_EDGE('',*,*,#5774,.F.);
#7475=ORIENTED_EDGE('',*,*,#5775,.T.);
#7476=ORIENTED_EDGE('',*,*,#5776,.T.);
#7477=ORIENTED_EDGE('',*,*,#5777,.F.);
#7478=ORIENTED_EDGE('',*,*,#5778,.F.);
#7479=ORIENTED_EDGE('',*,*,#5779,.F.);
#7480=ORIENTED_EDGE('',*,*,#5770,.T.);
#7481=ORIENTED_EDGE('',*,*,#5780,.T.);
#7482=ORIENTED_EDGE('',*,*,#5781,.T.);
#7483=ORIENTED_EDGE('',*,*,#5782,.F.);
#7484=ORIENTED_EDGE('',*,*,#5783,.T.);
#7485=ORIENTED_EDGE('',*,*,#5774,.T.);
#7486=ORIENTED_EDGE('',*,*,#5784,.F.);
#7487=ORIENTED_EDGE('',*,*,#5785,.F.);
#7488=ORIENTED_EDGE('',*,*,#5778,.T.);
#7489=ORIENTED_EDGE('',*,*,#5758,.F.);
#7490=ORIENTED_EDGE('',*,*,#5786,.F.);
#7491=ORIENTED_EDGE('',*,*,#5766,.T.);
#7492=ORIENTED_EDGE('',*,*,#5787,.T.);
#7493=ORIENTED_EDGE('',*,*,#5767,.T.);
#7494=ORIENTED_EDGE('',*,*,#5786,.T.);
#7495=ORIENTED_EDGE('',*,*,#5788,.F.);
#7496=ORIENTED_EDGE('',*,*,#5789,.F.);
#7497=ORIENTED_EDGE('',*,*,#5790,.T.);
#7498=ORIENTED_EDGE('',*,*,#5791,.F.);
#7499=ORIENTED_EDGE('',*,*,#5792,.T.);
#7500=ORIENTED_EDGE('',*,*,#5793,.T.);
#7501=ORIENTED_EDGE('',*,*,#5780,.F.);
#7502=ORIENTED_EDGE('',*,*,#5769,.F.);
#7503=ORIENTED_EDGE('',*,*,#5777,.T.);
#7504=ORIENTED_EDGE('',*,*,#5794,.F.);
#7505=ORIENTED_EDGE('',*,*,#5795,.F.);
#7506=ORIENTED_EDGE('',*,*,#5796,.T.);
#7507=ORIENTED_EDGE('',*,*,#5784,.T.);
#7508=ORIENTED_EDGE('',*,*,#5790,.F.);
#7509=ORIENTED_EDGE('',*,*,#5797,.T.);
#7510=ORIENTED_EDGE('',*,*,#5791,.T.);
#7511=ORIENTED_EDGE('',*,*,#5768,.F.);
#7512=ORIENTED_EDGE('',*,*,#5783,.F.);
#7513=ORIENTED_EDGE('',*,*,#5798,.F.);
#7514=ORIENTED_EDGE('',*,*,#5799,.T.);
#7515=ORIENTED_EDGE('',*,*,#5800,.T.);
#7516=ORIENTED_EDGE('',*,*,#5775,.F.);
#7517=ORIENTED_EDGE('',*,*,#5800,.F.);
#7518=ORIENTED_EDGE('',*,*,#5801,.T.);
#7519=ORIENTED_EDGE('',*,*,#5794,.T.);
#7520=ORIENTED_EDGE('',*,*,#5776,.F.);
#7521=ORIENTED_EDGE('',*,*,#5795,.T.);
#7522=ORIENTED_EDGE('',*,*,#5801,.F.);
#7523=ORIENTED_EDGE('',*,*,#5799,.F.);
#7524=ORIENTED_EDGE('',*,*,#5802,.T.);
#7525=ORIENTED_EDGE('',*,*,#5803,.F.);
#7526=ORIENTED_EDGE('',*,*,#5804,.F.);
#7527=ORIENTED_EDGE('',*,*,#5792,.F.);
#7528=ORIENTED_EDGE('',*,*,#5797,.F.);
#7529=ORIENTED_EDGE('',*,*,#5789,.T.);
#7530=ORIENTED_EDGE('',*,*,#5805,.F.);
#7531=ORIENTED_EDGE('',*,*,#5806,.F.);
#7532=ORIENTED_EDGE('',*,*,#5807,.T.);
#7533=ORIENTED_EDGE('',*,*,#5808,.F.);
#7534=ORIENTED_EDGE('',*,*,#5803,.T.);
#7535=ORIENTED_EDGE('',*,*,#5809,.T.);
#7536=ORIENTED_EDGE('',*,*,#5772,.F.);
#7537=ORIENTED_EDGE('',*,*,#5781,.F.);
#7538=ORIENTED_EDGE('',*,*,#5793,.F.);
#7539=ORIENTED_EDGE('',*,*,#5804,.T.);
#7540=ORIENTED_EDGE('',*,*,#5808,.T.);
#7541=ORIENTED_EDGE('',*,*,#5771,.F.);
#7542=ORIENTED_EDGE('',*,*,#5773,.T.);
#7543=ORIENTED_EDGE('',*,*,#5809,.F.);
#7544=ORIENTED_EDGE('',*,*,#5802,.F.);
#7545=ORIENTED_EDGE('',*,*,#5798,.T.);
#7546=ORIENTED_EDGE('',*,*,#5782,.T.);
#7547=ORIENTED_EDGE('',*,*,#5779,.T.);
#7548=ORIENTED_EDGE('',*,*,#5785,.T.);
#7549=ORIENTED_EDGE('',*,*,#5796,.F.);
#7550=ORIENTED_EDGE('',*,*,#5807,.F.);
#7551=ORIENTED_EDGE('',*,*,#5810,.T.);
#7552=ORIENTED_EDGE('',*,*,#5810,.F.);
#7553=ORIENTED_EDGE('',*,*,#5806,.T.);
#7554=ORIENTED_EDGE('',*,*,#5811,.T.);
#7555=ORIENTED_EDGE('',*,*,#5764,.F.);
#7556=ORIENTED_EDGE('',*,*,#5762,.F.);
#7557=ORIENTED_EDGE('',*,*,#5811,.F.);
#7558=ORIENTED_EDGE('',*,*,#5805,.T.);
#7559=ORIENTED_EDGE('',*,*,#5788,.T.);
#7560=ORIENTED_EDGE('',*,*,#5787,.F.);
#7561=ORIENTED_EDGE('',*,*,#5765,.F.);
#7562=ORIENTED_EDGE('',*,*,#5812,.T.);
#7563=ORIENTED_EDGE('',*,*,#5813,.T.);
#7564=ORIENTED_EDGE('',*,*,#5814,.T.);
#7565=ORIENTED_EDGE('',*,*,#5815,.T.);
#7566=ORIENTED_EDGE('',*,*,#5813,.F.);
#7567=ORIENTED_EDGE('',*,*,#5816,.T.);
#7568=ORIENTED_EDGE('',*,*,#5817,.T.);
#7569=ORIENTED_EDGE('',*,*,#5814,.F.);
#7570=ORIENTED_EDGE('',*,*,#5815,.F.);
#7571=ORIENTED_EDGE('',*,*,#5817,.F.);
#7572=ORIENTED_EDGE('',*,*,#5818,.T.);
#7573=ORIENTED_EDGE('',*,*,#5819,.T.);
#7574=ORIENTED_EDGE('',*,*,#5820,.F.);
#7575=ORIENTED_EDGE('',*,*,#5821,.F.);
#7576=ORIENTED_EDGE('',*,*,#5822,.T.);
#7577=ORIENTED_EDGE('',*,*,#5823,.T.);
#7578=ORIENTED_EDGE('',*,*,#5824,.F.);
#7579=ORIENTED_EDGE('',*,*,#5825,.T.);
#7580=ORIENTED_EDGE('',*,*,#5826,.T.);
#7581=ORIENTED_EDGE('',*,*,#5827,.F.);
#7582=ORIENTED_EDGE('',*,*,#5828,.F.);
#7583=ORIENTED_EDGE('',*,*,#5829,.T.);
#7584=ORIENTED_EDGE('',*,*,#5830,.T.);
#7585=ORIENTED_EDGE('',*,*,#5831,.F.);
#7586=ORIENTED_EDGE('',*,*,#5832,.F.);
#7587=ORIENTED_EDGE('',*,*,#5833,.F.);
#7588=ORIENTED_EDGE('',*,*,#5824,.T.);
#7589=ORIENTED_EDGE('',*,*,#5834,.T.);
#7590=ORIENTED_EDGE('',*,*,#5835,.T.);
#7591=ORIENTED_EDGE('',*,*,#5836,.F.);
#7592=ORIENTED_EDGE('',*,*,#5837,.T.);
#7593=ORIENTED_EDGE('',*,*,#5828,.T.);
#7594=ORIENTED_EDGE('',*,*,#5838,.F.);
#7595=ORIENTED_EDGE('',*,*,#5839,.F.);
#7596=ORIENTED_EDGE('',*,*,#5832,.T.);
#7597=ORIENTED_EDGE('',*,*,#5812,.F.);
#7598=ORIENTED_EDGE('',*,*,#5840,.F.);
#7599=ORIENTED_EDGE('',*,*,#5820,.T.);
#7600=ORIENTED_EDGE('',*,*,#5841,.T.);
#7601=ORIENTED_EDGE('',*,*,#5821,.T.);
#7602=ORIENTED_EDGE('',*,*,#5840,.T.);
#7603=ORIENTED_EDGE('',*,*,#5842,.F.);
#7604=ORIENTED_EDGE('',*,*,#5843,.F.);
#7605=ORIENTED_EDGE('',*,*,#5844,.T.);
#7606=ORIENTED_EDGE('',*,*,#5845,.F.);
#7607=ORIENTED_EDGE('',*,*,#5846,.T.);
#7608=ORIENTED_EDGE('',*,*,#5847,.T.);
#7609=ORIENTED_EDGE('',*,*,#5834,.F.);
#7610=ORIENTED_EDGE('',*,*,#5823,.F.);
#7611=ORIENTED_EDGE('',*,*,#5831,.T.);
#7612=ORIENTED_EDGE('',*,*,#5848,.F.);
#7613=ORIENTED_EDGE('',*,*,#5849,.F.);
#7614=ORIENTED_EDGE('',*,*,#5850,.T.);
#7615=ORIENTED_EDGE('',*,*,#5838,.T.);
#7616=ORIENTED_EDGE('',*,*,#5844,.F.);
#7617=ORIENTED_EDGE('',*,*,#5851,.T.);
#7618=ORIENTED_EDGE('',*,*,#5845,.T.);
#7619=ORIENTED_EDGE('',*,*,#5822,.F.);
#7620=ORIENTED_EDGE('',*,*,#5837,.F.);
#7621=ORIENTED_EDGE('',*,*,#5852,.F.);
#7622=ORIENTED_EDGE('',*,*,#5853,.T.);
#7623=ORIENTED_EDGE('',*,*,#5854,.T.);
#7624=ORIENTED_EDGE('',*,*,#5829,.F.);
#7625=ORIENTED_EDGE('',*,*,#5854,.F.);
#7626=ORIENTED_EDGE('',*,*,#5855,.T.);
#7627=ORIENTED_EDGE('',*,*,#5848,.T.);
#7628=ORIENTED_EDGE('',*,*,#5830,.F.);
#7629=ORIENTED_EDGE('',*,*,#5849,.T.);
#7630=ORIENTED_EDGE('',*,*,#5855,.F.);
#7631=ORIENTED_EDGE('',*,*,#5853,.F.);
#7632=ORIENTED_EDGE('',*,*,#5856,.T.);
#7633=ORIENTED_EDGE('',*,*,#5857,.F.);
#7634=ORIENTED_EDGE('',*,*,#5858,.F.);
#7635=ORIENTED_EDGE('',*,*,#5846,.F.);
#7636=ORIENTED_EDGE('',*,*,#5851,.F.);
#7637=ORIENTED_EDGE('',*,*,#5843,.T.);
#7638=ORIENTED_EDGE('',*,*,#5859,.F.);
#7639=ORIENTED_EDGE('',*,*,#5860,.F.);
#7640=ORIENTED_EDGE('',*,*,#5861,.T.);
#7641=ORIENTED_EDGE('',*,*,#5862,.F.);
#7642=ORIENTED_EDGE('',*,*,#5857,.T.);
#7643=ORIENTED_EDGE('',*,*,#5863,.T.);
#7644=ORIENTED_EDGE('',*,*,#5826,.F.);
#7645=ORIENTED_EDGE('',*,*,#5835,.F.);
#7646=ORIENTED_EDGE('',*,*,#5847,.F.);
#7647=ORIENTED_EDGE('',*,*,#5858,.T.);
#7648=ORIENTED_EDGE('',*,*,#5862,.T.);
#7649=ORIENTED_EDGE('',*,*,#5825,.F.);
#7650=ORIENTED_EDGE('',*,*,#5827,.T.);
#7651=ORIENTED_EDGE('',*,*,#5863,.F.);
#7652=ORIENTED_EDGE('',*,*,#5856,.F.);
#7653=ORIENTED_EDGE('',*,*,#5852,.T.);
#7654=ORIENTED_EDGE('',*,*,#5836,.T.);
#7655=ORIENTED_EDGE('',*,*,#5833,.T.);
#7656=ORIENTED_EDGE('',*,*,#5839,.T.);
#7657=ORIENTED_EDGE('',*,*,#5850,.F.);
#7658=ORIENTED_EDGE('',*,*,#5861,.F.);
#7659=ORIENTED_EDGE('',*,*,#5864,.T.);
#7660=ORIENTED_EDGE('',*,*,#5864,.F.);
#7661=ORIENTED_EDGE('',*,*,#5860,.T.);
#7662=ORIENTED_EDGE('',*,*,#5865,.T.);
#7663=ORIENTED_EDGE('',*,*,#5818,.F.);
#7664=ORIENTED_EDGE('',*,*,#5816,.F.);
#7665=ORIENTED_EDGE('',*,*,#5865,.F.);
#7666=ORIENTED_EDGE('',*,*,#5859,.T.);
#7667=ORIENTED_EDGE('',*,*,#5842,.T.);
#7668=ORIENTED_EDGE('',*,*,#5841,.F.);
#7669=ORIENTED_EDGE('',*,*,#5819,.F.);
#7670=ORIENTED_EDGE('',*,*,#5866,.F.);
#7671=ORIENTED_EDGE('',*,*,#5867,.T.);
#7672=ORIENTED_EDGE('',*,*,#5868,.T.);
#7673=ORIENTED_EDGE('',*,*,#5869,.T.);
#7674=ORIENTED_EDGE('',*,*,#5870,.F.);
#7675=ORIENTED_EDGE('',*,*,#5871,.T.);
#7676=ORIENTED_EDGE('',*,*,#5866,.T.);
#7677=ORIENTED_EDGE('',*,*,#5872,.T.);
#7678=ORIENTED_EDGE('',*,*,#5873,.F.);
#7679=ORIENTED_EDGE('',*,*,#5874,.T.);
#7680=ORIENTED_EDGE('',*,*,#5870,.T.);
#7681=ORIENTED_EDGE('',*,*,#5875,.T.);
#7682=ORIENTED_EDGE('',*,*,#5876,.F.);
#7683=ORIENTED_EDGE('',*,*,#5877,.T.);
#7684=ORIENTED_EDGE('',*,*,#5873,.T.);
#7685=ORIENTED_EDGE('',*,*,#5878,.T.);
#7686=ORIENTED_EDGE('',*,*,#5879,.F.);
#7687=ORIENTED_EDGE('',*,*,#5880,.T.);
#7688=ORIENTED_EDGE('',*,*,#5876,.T.);
#7689=ORIENTED_EDGE('',*,*,#5881,.T.);
#7690=ORIENTED_EDGE('',*,*,#5882,.F.);
#7691=ORIENTED_EDGE('',*,*,#5883,.T.);
#7692=ORIENTED_EDGE('',*,*,#5879,.T.);
#7693=ORIENTED_EDGE('',*,*,#5884,.T.);
#7694=ORIENTED_EDGE('',*,*,#5885,.F.);
#7695=ORIENTED_EDGE('',*,*,#5886,.T.);
#7696=ORIENTED_EDGE('',*,*,#5882,.T.);
#7697=ORIENTED_EDGE('',*,*,#5887,.T.);
#7698=ORIENTED_EDGE('',*,*,#5888,.F.);
#7699=ORIENTED_EDGE('',*,*,#5889,.T.);
#7700=ORIENTED_EDGE('',*,*,#5885,.T.);
#7701=ORIENTED_EDGE('',*,*,#5890,.T.);
#7702=ORIENTED_EDGE('',*,*,#5891,.F.);
#7703=ORIENTED_EDGE('',*,*,#5892,.T.);
#7704=ORIENTED_EDGE('',*,*,#5888,.T.);
#7705=ORIENTED_EDGE('',*,*,#5893,.T.);
#7706=ORIENTED_EDGE('',*,*,#5894,.F.);
#7707=ORIENTED_EDGE('',*,*,#5895,.T.);
#7708=ORIENTED_EDGE('',*,*,#5891,.T.);
#7709=ORIENTED_EDGE('',*,*,#5896,.T.);
#7710=ORIENTED_EDGE('',*,*,#5897,.F.);
#7711=ORIENTED_EDGE('',*,*,#5898,.T.);
#7712=ORIENTED_EDGE('',*,*,#5894,.T.);
#7713=ORIENTED_EDGE('',*,*,#5899,.T.);
#7714=ORIENTED_EDGE('',*,*,#5900,.F.);
#7715=ORIENTED_EDGE('',*,*,#5901,.T.);
#7716=ORIENTED_EDGE('',*,*,#5897,.T.);
#7717=ORIENTED_EDGE('',*,*,#5902,.T.);
#7718=ORIENTED_EDGE('',*,*,#5903,.F.);
#7719=ORIENTED_EDGE('',*,*,#5904,.T.);
#7720=ORIENTED_EDGE('',*,*,#5900,.T.);
#7721=ORIENTED_EDGE('',*,*,#5905,.T.);
#7722=ORIENTED_EDGE('',*,*,#5906,.F.);
#7723=ORIENTED_EDGE('',*,*,#5907,.T.);
#7724=ORIENTED_EDGE('',*,*,#5903,.T.);
#7725=ORIENTED_EDGE('',*,*,#5908,.T.);
#7726=ORIENTED_EDGE('',*,*,#5909,.F.);
#7727=ORIENTED_EDGE('',*,*,#5910,.T.);
#7728=ORIENTED_EDGE('',*,*,#5906,.T.);
#7729=ORIENTED_EDGE('',*,*,#5911,.T.);
#7730=ORIENTED_EDGE('',*,*,#5912,.F.);
#7731=ORIENTED_EDGE('',*,*,#5913,.T.);
#7732=ORIENTED_EDGE('',*,*,#5909,.T.);
#7733=ORIENTED_EDGE('',*,*,#5914,.T.);
#7734=ORIENTED_EDGE('',*,*,#5915,.F.);
#7735=ORIENTED_EDGE('',*,*,#5916,.T.);
#7736=ORIENTED_EDGE('',*,*,#5912,.T.);
#7737=ORIENTED_EDGE('',*,*,#5917,.T.);
#7738=ORIENTED_EDGE('',*,*,#5918,.F.);
#7739=ORIENTED_EDGE('',*,*,#5919,.T.);
#7740=ORIENTED_EDGE('',*,*,#5915,.T.);
#7741=ORIENTED_EDGE('',*,*,#5920,.T.);
#7742=ORIENTED_EDGE('',*,*,#5921,.F.);
#7743=ORIENTED_EDGE('',*,*,#5922,.T.);
#7744=ORIENTED_EDGE('',*,*,#5918,.T.);
#7745=ORIENTED_EDGE('',*,*,#5923,.T.);
#7746=ORIENTED_EDGE('',*,*,#5924,.F.);
#7747=ORIENTED_EDGE('',*,*,#5925,.T.);
#7748=ORIENTED_EDGE('',*,*,#5926,.T.);
#7749=ORIENTED_EDGE('',*,*,#5927,.T.);
#7750=ORIENTED_EDGE('',*,*,#5928,.F.);
#7751=ORIENTED_EDGE('',*,*,#5929,.T.);
#7752=ORIENTED_EDGE('',*,*,#5924,.T.);
#7753=ORIENTED_EDGE('',*,*,#5930,.T.);
#7754=ORIENTED_EDGE('',*,*,#5931,.F.);
#7755=ORIENTED_EDGE('',*,*,#5932,.T.);
#7756=ORIENTED_EDGE('',*,*,#5928,.T.);
#7757=ORIENTED_EDGE('',*,*,#5933,.T.);
#7758=ORIENTED_EDGE('',*,*,#5934,.F.);
#7759=ORIENTED_EDGE('',*,*,#5935,.T.);
#7760=ORIENTED_EDGE('',*,*,#5931,.T.);
#7761=ORIENTED_EDGE('',*,*,#5936,.T.);
#7762=ORIENTED_EDGE('',*,*,#5937,.F.);
#7763=ORIENTED_EDGE('',*,*,#5938,.T.);
#7764=ORIENTED_EDGE('',*,*,#5934,.T.);
#7765=ORIENTED_EDGE('',*,*,#5939,.T.);
#7766=ORIENTED_EDGE('',*,*,#5940,.F.);
#7767=ORIENTED_EDGE('',*,*,#5941,.T.);
#7768=ORIENTED_EDGE('',*,*,#5937,.T.);
#7769=ORIENTED_EDGE('',*,*,#5942,.T.);
#7770=ORIENTED_EDGE('',*,*,#5943,.F.);
#7771=ORIENTED_EDGE('',*,*,#5944,.T.);
#7772=ORIENTED_EDGE('',*,*,#5940,.T.);
#7773=ORIENTED_EDGE('',*,*,#5945,.T.);
#7774=ORIENTED_EDGE('',*,*,#5946,.F.);
#7775=ORIENTED_EDGE('',*,*,#5947,.T.);
#7776=ORIENTED_EDGE('',*,*,#5943,.T.);
#7777=ORIENTED_EDGE('',*,*,#5948,.T.);
#7778=ORIENTED_EDGE('',*,*,#5949,.F.);
#7779=ORIENTED_EDGE('',*,*,#5950,.T.);
#7780=ORIENTED_EDGE('',*,*,#5946,.T.);
#7781=ORIENTED_EDGE('',*,*,#5951,.T.);
#7782=ORIENTED_EDGE('',*,*,#5952,.F.);
#7783=ORIENTED_EDGE('',*,*,#5953,.T.);
#7784=ORIENTED_EDGE('',*,*,#5949,.T.);
#7785=ORIENTED_EDGE('',*,*,#5954,.T.);
#7786=ORIENTED_EDGE('',*,*,#5955,.F.);
#7787=ORIENTED_EDGE('',*,*,#5956,.T.);
#7788=ORIENTED_EDGE('',*,*,#5952,.T.);
#7789=ORIENTED_EDGE('',*,*,#5957,.T.);
#7790=ORIENTED_EDGE('',*,*,#5958,.F.);
#7791=ORIENTED_EDGE('',*,*,#5959,.T.);
#7792=ORIENTED_EDGE('',*,*,#5955,.T.);
#7793=ORIENTED_EDGE('',*,*,#5960,.T.);
#7794=ORIENTED_EDGE('',*,*,#5961,.F.);
#7795=ORIENTED_EDGE('',*,*,#5962,.T.);
#7796=ORIENTED_EDGE('',*,*,#5958,.T.);
#7797=ORIENTED_EDGE('',*,*,#5963,.T.);
#7798=ORIENTED_EDGE('',*,*,#5964,.F.);
#7799=ORIENTED_EDGE('',*,*,#5965,.T.);
#7800=ORIENTED_EDGE('',*,*,#5961,.T.);
#7801=ORIENTED_EDGE('',*,*,#5966,.T.);
#7802=ORIENTED_EDGE('',*,*,#5967,.F.);
#7803=ORIENTED_EDGE('',*,*,#5968,.T.);
#7804=ORIENTED_EDGE('',*,*,#5964,.T.);
#7805=ORIENTED_EDGE('',*,*,#5969,.T.);
#7806=ORIENTED_EDGE('',*,*,#5970,.F.);
#7807=ORIENTED_EDGE('',*,*,#5971,.T.);
#7808=ORIENTED_EDGE('',*,*,#5967,.T.);
#7809=ORIENTED_EDGE('',*,*,#5972,.T.);
#7810=ORIENTED_EDGE('',*,*,#5973,.F.);
#7811=ORIENTED_EDGE('',*,*,#5974,.T.);
#7812=ORIENTED_EDGE('',*,*,#5970,.T.);
#7813=ORIENTED_EDGE('',*,*,#5975,.T.);
#7814=ORIENTED_EDGE('',*,*,#5976,.F.);
#7815=ORIENTED_EDGE('',*,*,#5977,.T.);
#7816=ORIENTED_EDGE('',*,*,#5973,.T.);
#7817=ORIENTED_EDGE('',*,*,#5978,.T.);
#7818=ORIENTED_EDGE('',*,*,#5979,.F.);
#7819=ORIENTED_EDGE('',*,*,#5980,.T.);
#7820=ORIENTED_EDGE('',*,*,#5976,.T.);
#7821=ORIENTED_EDGE('',*,*,#5981,.T.);
#7822=ORIENTED_EDGE('',*,*,#5982,.F.);
#7823=ORIENTED_EDGE('',*,*,#5983,.T.);
#7824=ORIENTED_EDGE('',*,*,#5984,.T.);
#7825=ORIENTED_EDGE('',*,*,#5985,.F.);
#7826=ORIENTED_EDGE('',*,*,#5986,.T.);
#7827=ORIENTED_EDGE('',*,*,#5982,.T.);
#7828=ORIENTED_EDGE('',*,*,#5987,.T.);
#7829=ORIENTED_EDGE('',*,*,#5988,.F.);
#7830=ORIENTED_EDGE('',*,*,#5989,.T.);
#7831=ORIENTED_EDGE('',*,*,#5985,.T.);
#7832=ORIENTED_EDGE('',*,*,#5990,.T.);
#7833=ORIENTED_EDGE('',*,*,#5991,.F.);
#7834=ORIENTED_EDGE('',*,*,#5992,.T.);
#7835=ORIENTED_EDGE('',*,*,#5988,.T.);
#7836=ORIENTED_EDGE('',*,*,#5993,.T.);
#7837=ORIENTED_EDGE('',*,*,#5994,.F.);
#7838=ORIENTED_EDGE('',*,*,#5995,.T.);
#7839=ORIENTED_EDGE('',*,*,#5991,.T.);
#7840=ORIENTED_EDGE('',*,*,#5996,.T.);
#7841=ORIENTED_EDGE('',*,*,#5997,.F.);
#7842=ORIENTED_EDGE('',*,*,#5998,.T.);
#7843=ORIENTED_EDGE('',*,*,#5994,.T.);
#7844=ORIENTED_EDGE('',*,*,#5999,.T.);
#7845=ORIENTED_EDGE('',*,*,#6000,.F.);
#7846=ORIENTED_EDGE('',*,*,#6001,.T.);
#7847=ORIENTED_EDGE('',*,*,#5997,.T.);
#7848=ORIENTED_EDGE('',*,*,#6002,.T.);
#7849=ORIENTED_EDGE('',*,*,#6003,.F.);
#7850=ORIENTED_EDGE('',*,*,#6004,.T.);
#7851=ORIENTED_EDGE('',*,*,#6000,.T.);
#7852=ORIENTED_EDGE('',*,*,#6005,.T.);
#7853=ORIENTED_EDGE('',*,*,#6006,.F.);
#7854=ORIENTED_EDGE('',*,*,#6007,.T.);
#7855=ORIENTED_EDGE('',*,*,#6003,.T.);
#7856=ORIENTED_EDGE('',*,*,#6008,.T.);
#7857=ORIENTED_EDGE('',*,*,#6009,.F.);
#7858=ORIENTED_EDGE('',*,*,#6010,.T.);
#7859=ORIENTED_EDGE('',*,*,#6006,.T.);
#7860=ORIENTED_EDGE('',*,*,#6011,.T.);
#7861=ORIENTED_EDGE('',*,*,#6012,.F.);
#7862=ORIENTED_EDGE('',*,*,#6013,.T.);
#7863=ORIENTED_EDGE('',*,*,#6009,.T.);
#7864=ORIENTED_EDGE('',*,*,#6014,.T.);
#7865=ORIENTED_EDGE('',*,*,#6015,.F.);
#7866=ORIENTED_EDGE('',*,*,#6016,.T.);
#7867=ORIENTED_EDGE('',*,*,#6012,.T.);
#7868=ORIENTED_EDGE('',*,*,#6017,.T.);
#7869=ORIENTED_EDGE('',*,*,#6018,.F.);
#7870=ORIENTED_EDGE('',*,*,#6019,.T.);
#7871=ORIENTED_EDGE('',*,*,#6015,.T.);
#7872=ORIENTED_EDGE('',*,*,#6020,.T.);
#7873=ORIENTED_EDGE('',*,*,#6021,.F.);
#7874=ORIENTED_EDGE('',*,*,#6022,.T.);
#7875=ORIENTED_EDGE('',*,*,#6018,.T.);
#7876=ORIENTED_EDGE('',*,*,#6023,.T.);
#7877=ORIENTED_EDGE('',*,*,#6024,.F.);
#7878=ORIENTED_EDGE('',*,*,#6025,.T.);
#7879=ORIENTED_EDGE('',*,*,#6021,.T.);
#7880=ORIENTED_EDGE('',*,*,#6026,.T.);
#7881=ORIENTED_EDGE('',*,*,#6027,.F.);
#7882=ORIENTED_EDGE('',*,*,#6028,.T.);
#7883=ORIENTED_EDGE('',*,*,#6024,.T.);
#7884=ORIENTED_EDGE('',*,*,#6029,.T.);
#7885=ORIENTED_EDGE('',*,*,#6030,.F.);
#7886=ORIENTED_EDGE('',*,*,#6031,.T.);
#7887=ORIENTED_EDGE('',*,*,#6027,.T.);
#7888=ORIENTED_EDGE('',*,*,#6032,.T.);
#7889=ORIENTED_EDGE('',*,*,#6033,.F.);
#7890=ORIENTED_EDGE('',*,*,#6034,.T.);
#7891=ORIENTED_EDGE('',*,*,#6030,.T.);
#7892=ORIENTED_EDGE('',*,*,#6035,.T.);
#7893=ORIENTED_EDGE('',*,*,#6036,.F.);
#7894=ORIENTED_EDGE('',*,*,#6037,.T.);
#7895=ORIENTED_EDGE('',*,*,#6033,.T.);
#7896=ORIENTED_EDGE('',*,*,#6038,.T.);
#7897=ORIENTED_EDGE('',*,*,#6039,.F.);
#7898=ORIENTED_EDGE('',*,*,#6040,.T.);
#7899=ORIENTED_EDGE('',*,*,#6041,.T.);
#7900=ORIENTED_EDGE('',*,*,#6042,.T.);
#7901=ORIENTED_EDGE('',*,*,#6043,.F.);
#7902=ORIENTED_EDGE('',*,*,#6044,.T.);
#7903=ORIENTED_EDGE('',*,*,#6039,.T.);
#7904=ORIENTED_EDGE('',*,*,#6045,.T.);
#7905=ORIENTED_EDGE('',*,*,#6046,.F.);
#7906=ORIENTED_EDGE('',*,*,#6047,.T.);
#7907=ORIENTED_EDGE('',*,*,#6043,.T.);
#7908=ORIENTED_EDGE('',*,*,#6048,.T.);
#7909=ORIENTED_EDGE('',*,*,#6049,.F.);
#7910=ORIENTED_EDGE('',*,*,#6050,.T.);
#7911=ORIENTED_EDGE('',*,*,#6046,.T.);
#7912=ORIENTED_EDGE('',*,*,#6051,.T.);
#7913=ORIENTED_EDGE('',*,*,#6052,.F.);
#7914=ORIENTED_EDGE('',*,*,#6053,.T.);
#7915=ORIENTED_EDGE('',*,*,#6049,.T.);
#7916=ORIENTED_EDGE('',*,*,#6054,.T.);
#7917=ORIENTED_EDGE('',*,*,#6055,.F.);
#7918=ORIENTED_EDGE('',*,*,#6056,.T.);
#7919=ORIENTED_EDGE('',*,*,#6052,.T.);
#7920=ORIENTED_EDGE('',*,*,#6057,.T.);
#7921=ORIENTED_EDGE('',*,*,#6058,.F.);
#7922=ORIENTED_EDGE('',*,*,#6059,.T.);
#7923=ORIENTED_EDGE('',*,*,#6055,.T.);
#7924=ORIENTED_EDGE('',*,*,#6060,.T.);
#7925=ORIENTED_EDGE('',*,*,#6061,.F.);
#7926=ORIENTED_EDGE('',*,*,#6062,.T.);
#7927=ORIENTED_EDGE('',*,*,#6058,.T.);
#7928=ORIENTED_EDGE('',*,*,#6063,.T.);
#7929=ORIENTED_EDGE('',*,*,#6064,.F.);
#7930=ORIENTED_EDGE('',*,*,#6065,.T.);
#7931=ORIENTED_EDGE('',*,*,#6061,.T.);
#7932=ORIENTED_EDGE('',*,*,#6066,.T.);
#7933=ORIENTED_EDGE('',*,*,#6067,.F.);
#7934=ORIENTED_EDGE('',*,*,#6068,.T.);
#7935=ORIENTED_EDGE('',*,*,#6064,.T.);
#7936=ORIENTED_EDGE('',*,*,#6069,.T.);
#7937=ORIENTED_EDGE('',*,*,#6070,.F.);
#7938=ORIENTED_EDGE('',*,*,#6071,.T.);
#7939=ORIENTED_EDGE('',*,*,#6067,.T.);
#7940=ORIENTED_EDGE('',*,*,#6072,.T.);
#7941=ORIENTED_EDGE('',*,*,#6073,.F.);
#7942=ORIENTED_EDGE('',*,*,#6074,.T.);
#7943=ORIENTED_EDGE('',*,*,#6070,.T.);
#7944=ORIENTED_EDGE('',*,*,#6075,.T.);
#7945=ORIENTED_EDGE('',*,*,#6076,.F.);
#7946=ORIENTED_EDGE('',*,*,#6077,.T.);
#7947=ORIENTED_EDGE('',*,*,#6073,.T.);
#7948=ORIENTED_EDGE('',*,*,#6078,.T.);
#7949=ORIENTED_EDGE('',*,*,#6079,.F.);
#7950=ORIENTED_EDGE('',*,*,#6080,.T.);
#7951=ORIENTED_EDGE('',*,*,#6076,.T.);
#7952=ORIENTED_EDGE('',*,*,#6081,.T.);
#7953=ORIENTED_EDGE('',*,*,#6082,.F.);
#7954=ORIENTED_EDGE('',*,*,#6083,.T.);
#7955=ORIENTED_EDGE('',*,*,#6079,.T.);
#7956=ORIENTED_EDGE('',*,*,#6084,.T.);
#7957=ORIENTED_EDGE('',*,*,#6085,.F.);
#7958=ORIENTED_EDGE('',*,*,#6086,.T.);
#7959=ORIENTED_EDGE('',*,*,#6082,.T.);
#7960=ORIENTED_EDGE('',*,*,#6087,.T.);
#7961=ORIENTED_EDGE('',*,*,#6088,.F.);
#7962=ORIENTED_EDGE('',*,*,#6089,.T.);
#7963=ORIENTED_EDGE('',*,*,#6085,.T.);
#7964=ORIENTED_EDGE('',*,*,#6090,.T.);
#7965=ORIENTED_EDGE('',*,*,#6091,.F.);
#7966=ORIENTED_EDGE('',*,*,#6092,.T.);
#7967=ORIENTED_EDGE('',*,*,#6088,.T.);
#7968=ORIENTED_EDGE('',*,*,#6093,.T.);
#7969=ORIENTED_EDGE('',*,*,#6094,.T.);
#7970=ORIENTED_EDGE('',*,*,#6095,.F.);
#7971=ORIENTED_EDGE('',*,*,#6096,.T.);
#7972=ORIENTED_EDGE('',*,*,#6097,.T.);
#7973=ORIENTED_EDGE('',*,*,#6098,.F.);
#7974=ORIENTED_EDGE('',*,*,#6099,.F.);
#7975=ORIENTED_EDGE('',*,*,#6094,.F.);
#7976=ORIENTED_EDGE('',*,*,#6100,.T.);
#7977=ORIENTED_EDGE('',*,*,#6101,.T.);
#7978=ORIENTED_EDGE('',*,*,#6102,.F.);
#7979=ORIENTED_EDGE('',*,*,#6097,.F.);
#7980=ORIENTED_EDGE('',*,*,#6103,.T.);
#7981=ORIENTED_EDGE('',*,*,#6104,.T.);
#7982=ORIENTED_EDGE('',*,*,#6105,.F.);
#7983=ORIENTED_EDGE('',*,*,#6101,.F.);
#7984=ORIENTED_EDGE('',*,*,#6106,.T.);
#7985=ORIENTED_EDGE('',*,*,#6107,.T.);
#7986=ORIENTED_EDGE('',*,*,#6108,.F.);
#7987=ORIENTED_EDGE('',*,*,#6104,.F.);
#7988=ORIENTED_EDGE('',*,*,#6109,.T.);
#7989=ORIENTED_EDGE('',*,*,#6110,.T.);
#7990=ORIENTED_EDGE('',*,*,#6111,.F.);
#7991=ORIENTED_EDGE('',*,*,#6107,.F.);
#7992=ORIENTED_EDGE('',*,*,#6112,.T.);
#7993=ORIENTED_EDGE('',*,*,#6113,.F.);
#7994=ORIENTED_EDGE('',*,*,#6114,.T.);
#7995=ORIENTED_EDGE('',*,*,#6115,.F.);
#7996=ORIENTED_EDGE('',*,*,#6116,.F.);
#7997=ORIENTED_EDGE('',*,*,#6117,.T.);
#7998=ORIENTED_EDGE('',*,*,#6118,.F.);
#7999=ORIENTED_EDGE('',*,*,#6119,.T.);
#8000=ORIENTED_EDGE('',*,*,#6120,.T.);
#8001=ORIENTED_EDGE('',*,*,#6121,.F.);
#8002=ORIENTED_EDGE('',*,*,#6122,.F.);
#8003=ORIENTED_EDGE('',*,*,#6117,.F.);
#8004=ORIENTED_EDGE('',*,*,#6123,.T.);
#8005=ORIENTED_EDGE('',*,*,#6124,.T.);
#8006=ORIENTED_EDGE('',*,*,#6125,.F.);
#8007=ORIENTED_EDGE('',*,*,#6120,.F.);
#8008=ORIENTED_EDGE('',*,*,#6126,.T.);
#8009=ORIENTED_EDGE('',*,*,#6127,.T.);
#8010=ORIENTED_EDGE('',*,*,#6128,.F.);
#8011=ORIENTED_EDGE('',*,*,#6124,.F.);
#8012=ORIENTED_EDGE('',*,*,#6129,.T.);
#8013=ORIENTED_EDGE('',*,*,#6130,.T.);
#8014=ORIENTED_EDGE('',*,*,#6131,.F.);
#8015=ORIENTED_EDGE('',*,*,#6127,.F.);
#8016=ORIENTED_EDGE('',*,*,#6132,.T.);
#8017=ORIENTED_EDGE('',*,*,#6133,.T.);
#8018=ORIENTED_EDGE('',*,*,#6134,.F.);
#8019=ORIENTED_EDGE('',*,*,#6130,.F.);
#8020=ORIENTED_EDGE('',*,*,#6135,.T.);
#8021=ORIENTED_EDGE('',*,*,#6136,.F.);
#8022=ORIENTED_EDGE('',*,*,#6137,.T.);
#8023=ORIENTED_EDGE('',*,*,#6138,.F.);
#8024=ORIENTED_EDGE('',*,*,#6139,.F.);
#8025=ORIENTED_EDGE('',*,*,#6140,.T.);
#8026=ORIENTED_EDGE('',*,*,#6141,.F.);
#8027=ORIENTED_EDGE('',*,*,#6142,.T.);
#8028=ORIENTED_EDGE('',*,*,#6143,.T.);
#8029=ORIENTED_EDGE('',*,*,#6144,.F.);
#8030=ORIENTED_EDGE('',*,*,#6145,.F.);
#8031=ORIENTED_EDGE('',*,*,#6140,.F.);
#8032=ORIENTED_EDGE('',*,*,#6146,.T.);
#8033=ORIENTED_EDGE('',*,*,#6147,.T.);
#8034=ORIENTED_EDGE('',*,*,#6148,.F.);
#8035=ORIENTED_EDGE('',*,*,#6143,.F.);
#8036=ORIENTED_EDGE('',*,*,#6149,.T.);
#8037=ORIENTED_EDGE('',*,*,#6150,.T.);
#8038=ORIENTED_EDGE('',*,*,#6151,.F.);
#8039=ORIENTED_EDGE('',*,*,#6147,.F.);
#8040=ORIENTED_EDGE('',*,*,#6152,.T.);
#8041=ORIENTED_EDGE('',*,*,#6153,.T.);
#8042=ORIENTED_EDGE('',*,*,#6154,.F.);
#8043=ORIENTED_EDGE('',*,*,#6150,.F.);
#8044=ORIENTED_EDGE('',*,*,#6155,.T.);
#8045=ORIENTED_EDGE('',*,*,#6156,.T.);
#8046=ORIENTED_EDGE('',*,*,#6157,.F.);
#8047=ORIENTED_EDGE('',*,*,#6153,.F.);
#8048=ORIENTED_EDGE('',*,*,#6158,.T.);
#8049=ORIENTED_EDGE('',*,*,#6159,.F.);
#8050=ORIENTED_EDGE('',*,*,#6160,.T.);
#8051=ORIENTED_EDGE('',*,*,#6161,.F.);
#8052=ORIENTED_EDGE('',*,*,#6162,.F.);
#8053=ORIENTED_EDGE('',*,*,#6163,.T.);
#8054=ORIENTED_EDGE('',*,*,#6164,.F.);
#8055=ORIENTED_EDGE('',*,*,#6165,.T.);
#8056=ORIENTED_EDGE('',*,*,#6166,.T.);
#8057=ORIENTED_EDGE('',*,*,#6167,.F.);
#8058=ORIENTED_EDGE('',*,*,#6168,.F.);
#8059=ORIENTED_EDGE('',*,*,#6163,.F.);
#8060=ORIENTED_EDGE('',*,*,#6169,.T.);
#8061=ORIENTED_EDGE('',*,*,#6170,.T.);
#8062=ORIENTED_EDGE('',*,*,#6171,.F.);
#8063=ORIENTED_EDGE('',*,*,#6166,.F.);
#8064=ORIENTED_EDGE('',*,*,#6172,.T.);
#8065=ORIENTED_EDGE('',*,*,#6173,.T.);
#8066=ORIENTED_EDGE('',*,*,#6174,.F.);
#8067=ORIENTED_EDGE('',*,*,#6170,.F.);
#8068=ORIENTED_EDGE('',*,*,#6175,.T.);
#8069=ORIENTED_EDGE('',*,*,#6176,.T.);
#8070=ORIENTED_EDGE('',*,*,#6177,.F.);
#8071=ORIENTED_EDGE('',*,*,#6173,.F.);
#8072=ORIENTED_EDGE('',*,*,#6178,.T.);
#8073=ORIENTED_EDGE('',*,*,#6179,.T.);
#8074=ORIENTED_EDGE('',*,*,#6180,.F.);
#8075=ORIENTED_EDGE('',*,*,#6176,.F.);
#8076=ORIENTED_EDGE('',*,*,#6181,.T.);
#8077=ORIENTED_EDGE('',*,*,#6182,.F.);
#8078=ORIENTED_EDGE('',*,*,#6183,.T.);
#8079=ORIENTED_EDGE('',*,*,#6184,.F.);
#8080=ORIENTED_EDGE('',*,*,#6185,.F.);
#8081=ORIENTED_EDGE('',*,*,#6182,.T.);
#8082=ORIENTED_EDGE('',*,*,#6186,.F.);
#8083=ORIENTED_EDGE('',*,*,#6179,.F.);
#8084=ORIENTED_EDGE('',*,*,#6187,.T.);
#8085=ORIENTED_EDGE('',*,*,#6159,.T.);
#8086=ORIENTED_EDGE('',*,*,#6188,.F.);
#8087=ORIENTED_EDGE('',*,*,#6156,.F.);
#8088=ORIENTED_EDGE('',*,*,#6189,.T.);
#8089=ORIENTED_EDGE('',*,*,#6136,.T.);
#8090=ORIENTED_EDGE('',*,*,#6190,.F.);
#8091=ORIENTED_EDGE('',*,*,#6133,.F.);
#8092=ORIENTED_EDGE('',*,*,#6191,.T.);
#8093=ORIENTED_EDGE('',*,*,#6113,.T.);
#8094=ORIENTED_EDGE('',*,*,#6192,.F.);
#8095=ORIENTED_EDGE('',*,*,#6110,.F.);
#8096=ORIENTED_EDGE('',*,*,#6193,.T.);
#8097=ORIENTED_EDGE('',*,*,#6091,.T.);
#8098=ORIENTED_EDGE('',*,*,#6194,.T.);
#8099=ORIENTED_EDGE('',*,*,#6195,.F.);
#8100=ORIENTED_EDGE('',*,*,#6196,.T.);
#8101=ORIENTED_EDGE('',*,*,#6036,.T.);
#8102=ORIENTED_EDGE('',*,*,#6197,.T.);
#8103=ORIENTED_EDGE('',*,*,#6198,.F.);
#8104=ORIENTED_EDGE('',*,*,#6199,.T.);
#8105=ORIENTED_EDGE('',*,*,#5979,.T.);
#8106=ORIENTED_EDGE('',*,*,#6200,.T.);
#8107=ORIENTED_EDGE('',*,*,#6201,.F.);
#8108=ORIENTED_EDGE('',*,*,#6202,.T.);
#8109=ORIENTED_EDGE('',*,*,#5921,.T.);
#8110=ORIENTED_EDGE('',*,*,#6203,.T.);
#8111=ORIENTED_EDGE('',*,*,#6204,.F.);
#8112=ORIENTED_EDGE('',*,*,#6205,.T.);
#8113=ORIENTED_EDGE('',*,*,#6206,.F.);
#8114=ORIENTED_EDGE('',*,*,#6207,.T.);
#8115=ORIENTED_EDGE('',*,*,#6208,.F.);
#8116=ORIENTED_EDGE('',*,*,#6207,.F.);
#8117=ORIENTED_EDGE('',*,*,#6209,.F.);
#8118=ORIENTED_EDGE('',*,*,#6210,.T.);
#8119=ORIENTED_EDGE('',*,*,#6211,.T.);
#8120=ORIENTED_EDGE('',*,*,#6210,.F.);
#8121=ORIENTED_EDGE('',*,*,#6212,.F.);
#8122=ORIENTED_EDGE('',*,*,#6213,.T.);
#8123=ORIENTED_EDGE('',*,*,#6214,.F.);
#8124=ORIENTED_EDGE('',*,*,#6213,.F.);
#8125=ORIENTED_EDGE('',*,*,#6214,.T.);
#8126=ORIENTED_EDGE('',*,*,#6215,.T.);
#8127=ORIENTED_EDGE('',*,*,#6216,.F.);
#8128=ORIENTED_EDGE('',*,*,#6215,.F.);
#8129=ORIENTED_EDGE('',*,*,#6217,.F.);
#8130=ORIENTED_EDGE('',*,*,#5868,.F.);
#8131=ORIENTED_EDGE('',*,*,#6218,.F.);
#8132=ORIENTED_EDGE('',*,*,#6219,.F.);
#8133=ORIENTED_EDGE('',*,*,#6220,.F.);
#8134=ORIENTED_EDGE('',*,*,#6221,.T.);
#8135=ORIENTED_EDGE('',*,*,#6222,.F.);
#8136=ORIENTED_EDGE('',*,*,#6221,.F.);
#8137=ORIENTED_EDGE('',*,*,#6223,.F.);
#8138=ORIENTED_EDGE('',*,*,#5926,.F.);
#8139=ORIENTED_EDGE('',*,*,#6224,.F.);
#8140=ORIENTED_EDGE('',*,*,#6225,.F.);
#8141=ORIENTED_EDGE('',*,*,#6226,.F.);
#8142=ORIENTED_EDGE('',*,*,#6227,.T.);
#8143=ORIENTED_EDGE('',*,*,#6228,.F.);
#8144=ORIENTED_EDGE('',*,*,#6227,.F.);
#8145=ORIENTED_EDGE('',*,*,#6229,.F.);
#8146=ORIENTED_EDGE('',*,*,#5984,.F.);
#8147=ORIENTED_EDGE('',*,*,#6230,.F.);
#8148=ORIENTED_EDGE('',*,*,#6231,.F.);
#8149=ORIENTED_EDGE('',*,*,#6232,.F.);
#8150=ORIENTED_EDGE('',*,*,#6233,.T.);
#8151=ORIENTED_EDGE('',*,*,#6234,.F.);
#8152=ORIENTED_EDGE('',*,*,#6233,.F.);
#8153=ORIENTED_EDGE('',*,*,#6235,.F.);
#8154=ORIENTED_EDGE('',*,*,#6041,.F.);
#8155=ORIENTED_EDGE('',*,*,#6236,.F.);
#8156=ORIENTED_EDGE('',*,*,#6237,.F.);
#8157=ORIENTED_EDGE('',*,*,#6238,.F.);
#8158=ORIENTED_EDGE('',*,*,#6239,.T.);
#8159=ORIENTED_EDGE('',*,*,#6240,.F.);
#8160=ORIENTED_EDGE('',*,*,#6239,.F.);
#8161=ORIENTED_EDGE('',*,*,#6241,.F.);
#8162=ORIENTED_EDGE('',*,*,#6194,.F.);
#8163=ORIENTED_EDGE('',*,*,#6093,.F.);
#8164=ORIENTED_EDGE('',*,*,#6090,.F.);
#8165=ORIENTED_EDGE('',*,*,#6087,.F.);
#8166=ORIENTED_EDGE('',*,*,#6084,.F.);
#8167=ORIENTED_EDGE('',*,*,#6081,.F.);
#8168=ORIENTED_EDGE('',*,*,#6078,.F.);
#8169=ORIENTED_EDGE('',*,*,#6075,.F.);
#8170=ORIENTED_EDGE('',*,*,#6072,.F.);
#8171=ORIENTED_EDGE('',*,*,#6069,.F.);
#8172=ORIENTED_EDGE('',*,*,#6066,.F.);
#8173=ORIENTED_EDGE('',*,*,#6063,.F.);
#8174=ORIENTED_EDGE('',*,*,#6060,.F.);
#8175=ORIENTED_EDGE('',*,*,#6057,.F.);
#8176=ORIENTED_EDGE('',*,*,#6054,.F.);
#8177=ORIENTED_EDGE('',*,*,#6051,.F.);
#8178=ORIENTED_EDGE('',*,*,#6048,.F.);
#8179=ORIENTED_EDGE('',*,*,#6045,.F.);
#8180=ORIENTED_EDGE('',*,*,#6042,.F.);
#8181=ORIENTED_EDGE('',*,*,#6235,.T.);
#8182=ORIENTED_EDGE('',*,*,#6238,.T.);
#8183=ORIENTED_EDGE('',*,*,#6242,.T.);
#8184=ORIENTED_EDGE('',*,*,#6243,.F.);
#8185=ORIENTED_EDGE('',*,*,#6114,.F.);
#8186=ORIENTED_EDGE('',*,*,#6193,.F.);
#8187=ORIENTED_EDGE('',*,*,#6112,.F.);
#8188=ORIENTED_EDGE('',*,*,#6109,.F.);
#8189=ORIENTED_EDGE('',*,*,#6106,.F.);
#8190=ORIENTED_EDGE('',*,*,#6103,.F.);
#8191=ORIENTED_EDGE('',*,*,#6100,.F.);
#8192=ORIENTED_EDGE('',*,*,#6096,.F.);
#8193=ORIENTED_EDGE('',*,*,#6244,.F.);
#8194=ORIENTED_EDGE('',*,*,#6098,.T.);
#8195=ORIENTED_EDGE('',*,*,#6102,.T.);
#8196=ORIENTED_EDGE('',*,*,#6105,.T.);
#8197=ORIENTED_EDGE('',*,*,#6108,.T.);
#8198=ORIENTED_EDGE('',*,*,#6111,.T.);
#8199=ORIENTED_EDGE('',*,*,#6192,.T.);
#8200=ORIENTED_EDGE('',*,*,#6116,.T.);
#8201=ORIENTED_EDGE('',*,*,#6245,.F.);
#8202=ORIENTED_EDGE('',*,*,#6246,.F.);
#8203=ORIENTED_EDGE('',*,*,#6236,.T.);
#8204=ORIENTED_EDGE('',*,*,#6040,.F.);
#8205=ORIENTED_EDGE('',*,*,#6044,.F.);
#8206=ORIENTED_EDGE('',*,*,#6047,.F.);
#8207=ORIENTED_EDGE('',*,*,#6050,.F.);
#8208=ORIENTED_EDGE('',*,*,#6053,.F.);
#8209=ORIENTED_EDGE('',*,*,#6056,.F.);
#8210=ORIENTED_EDGE('',*,*,#6059,.F.);
#8211=ORIENTED_EDGE('',*,*,#6062,.F.);
#8212=ORIENTED_EDGE('',*,*,#6065,.F.);
#8213=ORIENTED_EDGE('',*,*,#6068,.F.);
#8214=ORIENTED_EDGE('',*,*,#6071,.F.);
#8215=ORIENTED_EDGE('',*,*,#6074,.F.);
#8216=ORIENTED_EDGE('',*,*,#6077,.F.);
#8217=ORIENTED_EDGE('',*,*,#6080,.F.);
#8218=ORIENTED_EDGE('',*,*,#6083,.F.);
#8219=ORIENTED_EDGE('',*,*,#6086,.F.);
#8220=ORIENTED_EDGE('',*,*,#6089,.F.);
#8221=ORIENTED_EDGE('',*,*,#6092,.F.);
#8222=ORIENTED_EDGE('',*,*,#6196,.F.);
#8223=ORIENTED_EDGE('',*,*,#6243,.T.);
#8224=ORIENTED_EDGE('',*,*,#6247,.T.);
#8225=ORIENTED_EDGE('',*,*,#6245,.T.);
#8226=ORIENTED_EDGE('',*,*,#6115,.T.);
#8227=ORIENTED_EDGE('',*,*,#6242,.F.);
#8228=ORIENTED_EDGE('',*,*,#6237,.T.);
#8229=ORIENTED_EDGE('',*,*,#6246,.T.);
#8230=ORIENTED_EDGE('',*,*,#6247,.F.);
#8231=ORIENTED_EDGE('',*,*,#6248,.F.);
#8232=ORIENTED_EDGE('',*,*,#6249,.F.);
#8233=ORIENTED_EDGE('',*,*,#6250,.F.);
#8234=ORIENTED_EDGE('',*,*,#6251,.F.);
#8235=ORIENTED_EDGE('',*,*,#6252,.T.);
#8236=ORIENTED_EDGE('',*,*,#6253,.F.);
#8237=ORIENTED_EDGE('',*,*,#6254,.F.);
#8238=ORIENTED_EDGE('',*,*,#6255,.F.);
#8239=ORIENTED_EDGE('',*,*,#6206,.T.);
#8240=ORIENTED_EDGE('',*,*,#6204,.T.);
#8241=ORIENTED_EDGE('',*,*,#6256,.T.);
#8242=ORIENTED_EDGE('',*,*,#6164,.T.);
#8243=ORIENTED_EDGE('',*,*,#6168,.T.);
#8244=ORIENTED_EDGE('',*,*,#6257,.T.);
#8245=ORIENTED_EDGE('',*,*,#6201,.T.);
#8246=ORIENTED_EDGE('',*,*,#6258,.T.);
#8247=ORIENTED_EDGE('',*,*,#6141,.T.);
#8248=ORIENTED_EDGE('',*,*,#6145,.T.);
#8249=ORIENTED_EDGE('',*,*,#6259,.T.);
#8250=ORIENTED_EDGE('',*,*,#6198,.T.);
#8251=ORIENTED_EDGE('',*,*,#6260,.T.);
#8252=ORIENTED_EDGE('',*,*,#6118,.T.);
#8253=ORIENTED_EDGE('',*,*,#6122,.T.);
#8254=ORIENTED_EDGE('',*,*,#6261,.T.);
#8255=ORIENTED_EDGE('',*,*,#6195,.T.);
#8256=ORIENTED_EDGE('',*,*,#6241,.T.);
#8257=ORIENTED_EDGE('',*,*,#6095,.T.);
#8258=ORIENTED_EDGE('',*,*,#6099,.T.);
#8259=ORIENTED_EDGE('',*,*,#6244,.T.);
#8260=ORIENTED_EDGE('',*,*,#6260,.F.);
#8261=ORIENTED_EDGE('',*,*,#6197,.F.);
#8262=ORIENTED_EDGE('',*,*,#6038,.F.);
#8263=ORIENTED_EDGE('',*,*,#6035,.F.);
#8264=ORIENTED_EDGE('',*,*,#6032,.F.);
#8265=ORIENTED_EDGE('',*,*,#6029,.F.);
#8266=ORIENTED_EDGE('',*,*,#6026,.F.);
#8267=ORIENTED_EDGE('',*,*,#6023,.F.);
#8268=ORIENTED_EDGE('',*,*,#6020,.F.);
#8269=ORIENTED_EDGE('',*,*,#6017,.F.);
#8270=ORIENTED_EDGE('',*,*,#6014,.F.);
#8271=ORIENTED_EDGE('',*,*,#6011,.F.);
#8272=ORIENTED_EDGE('',*,*,#6008,.F.);
#8273=ORIENTED_EDGE('',*,*,#6005,.F.);
#8274=ORIENTED_EDGE('',*,*,#6002,.F.);
#8275=ORIENTED_EDGE('',*,*,#5999,.F.);
#8276=ORIENTED_EDGE('',*,*,#5996,.F.);
#8277=ORIENTED_EDGE('',*,*,#5993,.F.);
#8278=ORIENTED_EDGE('',*,*,#5990,.F.);
#8279=ORIENTED_EDGE('',*,*,#5987,.F.);
#8280=ORIENTED_EDGE('',*,*,#6229,.T.);
#8281=ORIENTED_EDGE('',*,*,#6232,.T.);
#8282=ORIENTED_EDGE('',*,*,#6262,.T.);
#8283=ORIENTED_EDGE('',*,*,#6263,.F.);
#8284=ORIENTED_EDGE('',*,*,#6137,.F.);
#8285=ORIENTED_EDGE('',*,*,#6191,.F.);
#8286=ORIENTED_EDGE('',*,*,#6135,.F.);
#8287=ORIENTED_EDGE('',*,*,#6132,.F.);
#8288=ORIENTED_EDGE('',*,*,#6129,.F.);
#8289=ORIENTED_EDGE('',*,*,#6126,.F.);
#8290=ORIENTED_EDGE('',*,*,#6123,.F.);
#8291=ORIENTED_EDGE('',*,*,#6119,.F.);
#8292=ORIENTED_EDGE('',*,*,#6261,.F.);
#8293=ORIENTED_EDGE('',*,*,#6121,.T.);
#8294=ORIENTED_EDGE('',*,*,#6125,.T.);
#8295=ORIENTED_EDGE('',*,*,#6128,.T.);
#8296=ORIENTED_EDGE('',*,*,#6131,.T.);
#8297=ORIENTED_EDGE('',*,*,#6134,.T.);
#8298=ORIENTED_EDGE('',*,*,#6190,.T.);
#8299=ORIENTED_EDGE('',*,*,#6139,.T.);
#8300=ORIENTED_EDGE('',*,*,#6264,.F.);
#8301=ORIENTED_EDGE('',*,*,#6265,.F.);
#8302=ORIENTED_EDGE('',*,*,#6230,.T.);
#8303=ORIENTED_EDGE('',*,*,#5983,.F.);
#8304=ORIENTED_EDGE('',*,*,#5986,.F.);
#8305=ORIENTED_EDGE('',*,*,#5989,.F.);
#8306=ORIENTED_EDGE('',*,*,#5992,.F.);
#8307=ORIENTED_EDGE('',*,*,#5995,.F.);
#8308=ORIENTED_EDGE('',*,*,#5998,.F.);
#8309=ORIENTED_EDGE('',*,*,#6001,.F.);
#8310=ORIENTED_EDGE('',*,*,#6004,.F.);
#8311=ORIENTED_EDGE('',*,*,#6007,.F.);
#8312=ORIENTED_EDGE('',*,*,#6010,.F.);
#8313=ORIENTED_EDGE('',*,*,#6013,.F.);
#8314=ORIENTED_EDGE('',*,*,#6016,.F.);
#8315=ORIENTED_EDGE('',*,*,#6019,.F.);
#8316=ORIENTED_EDGE('',*,*,#6022,.F.);
#8317=ORIENTED_EDGE('',*,*,#6025,.F.);
#8318=ORIENTED_EDGE('',*,*,#6028,.F.);
#8319=ORIENTED_EDGE('',*,*,#6031,.F.);
#8320=ORIENTED_EDGE('',*,*,#6034,.F.);
#8321=ORIENTED_EDGE('',*,*,#6037,.F.);
#8322=ORIENTED_EDGE('',*,*,#6199,.F.);
#8323=ORIENTED_EDGE('',*,*,#6263,.T.);
#8324=ORIENTED_EDGE('',*,*,#6266,.T.);
#8325=ORIENTED_EDGE('',*,*,#6264,.T.);
#8326=ORIENTED_EDGE('',*,*,#6138,.T.);
#8327=ORIENTED_EDGE('',*,*,#6262,.F.);
#8328=ORIENTED_EDGE('',*,*,#6231,.T.);
#8329=ORIENTED_EDGE('',*,*,#6265,.T.);
#8330=ORIENTED_EDGE('',*,*,#6266,.F.);
#8331=ORIENTED_EDGE('',*,*,#6258,.F.);
#8332=ORIENTED_EDGE('',*,*,#6200,.F.);
#8333=ORIENTED_EDGE('',*,*,#5981,.F.);
#8334=ORIENTED_EDGE('',*,*,#5978,.F.);
#8335=ORIENTED_EDGE('',*,*,#5975,.F.);
#8336=ORIENTED_EDGE('',*,*,#5972,.F.);
#8337=ORIENTED_EDGE('',*,*,#5969,.F.);
#8338=ORIENTED_EDGE('',*,*,#5966,.F.);
#8339=ORIENTED_EDGE('',*,*,#5963,.F.);
#8340=ORIENTED_EDGE('',*,*,#5960,.F.);
#8341=ORIENTED_EDGE('',*,*,#5957,.F.);
#8342=ORIENTED_EDGE('',*,*,#5954,.F.);
#8343=ORIENTED_EDGE('',*,*,#5951,.F.);
#8344=ORIENTED_EDGE('',*,*,#5948,.F.);
#8345=ORIENTED_EDGE('',*,*,#5945,.F.);
#8346=ORIENTED_EDGE('',*,*,#5942,.F.);
#8347=ORIENTED_EDGE('',*,*,#5939,.F.);
#8348=ORIENTED_EDGE('',*,*,#5936,.F.);
#8349=ORIENTED_EDGE('',*,*,#5933,.F.);
#8350=ORIENTED_EDGE('',*,*,#5930,.F.);
#8351=ORIENTED_EDGE('',*,*,#5927,.F.);
#8352=ORIENTED_EDGE('',*,*,#6223,.T.);
#8353=ORIENTED_EDGE('',*,*,#6226,.T.);
#8354=ORIENTED_EDGE('',*,*,#6267,.T.);
#8355=ORIENTED_EDGE('',*,*,#6268,.F.);
#8356=ORIENTED_EDGE('',*,*,#6160,.F.);
#8357=ORIENTED_EDGE('',*,*,#6189,.F.);
#8358=ORIENTED_EDGE('',*,*,#6158,.F.);
#8359=ORIENTED_EDGE('',*,*,#6155,.F.);
#8360=ORIENTED_EDGE('',*,*,#6152,.F.);
#8361=ORIENTED_EDGE('',*,*,#6149,.F.);
#8362=ORIENTED_EDGE('',*,*,#6146,.F.);
#8363=ORIENTED_EDGE('',*,*,#6142,.F.);
#8364=ORIENTED_EDGE('',*,*,#6259,.F.);
#8365=ORIENTED_EDGE('',*,*,#6144,.T.);
#8366=ORIENTED_EDGE('',*,*,#6148,.T.);
#8367=ORIENTED_EDGE('',*,*,#6151,.T.);
#8368=ORIENTED_EDGE('',*,*,#6154,.T.);
#8369=ORIENTED_EDGE('',*,*,#6157,.T.);
#8370=ORIENTED_EDGE('',*,*,#6188,.T.);
#8371=ORIENTED_EDGE('',*,*,#6162,.T.);
#8372=ORIENTED_EDGE('',*,*,#6269,.F.);
#8373=ORIENTED_EDGE('',*,*,#6270,.F.);
#8374=ORIENTED_EDGE('',*,*,#6224,.T.);
#8375=ORIENTED_EDGE('',*,*,#5925,.F.);
#8376=ORIENTED_EDGE('',*,*,#5929,.F.);
#8377=ORIENTED_EDGE('',*,*,#5932,.F.);
#8378=ORIENTED_EDGE('',*,*,#5935,.F.);
#8379=ORIENTED_EDGE('',*,*,#5938,.F.);
#8380=ORIENTED_EDGE('',*,*,#5941,.F.);
#8381=ORIENTED_EDGE('',*,*,#5944,.F.);
#8382=ORIENTED_EDGE('',*,*,#5947,.F.);
#8383=ORIENTED_EDGE('',*,*,#5950,.F.);
#8384=ORIENTED_EDGE('',*,*,#5953,.F.);
#8385=ORIENTED_EDGE('',*,*,#5956,.F.);
#8386=ORIENTED_EDGE('',*,*,#5959,.F.);
#8387=ORIENTED_EDGE('',*,*,#5962,.F.);
#8388=ORIENTED_EDGE('',*,*,#5965,.F.);
#8389=ORIENTED_EDGE('',*,*,#5968,.F.);
#8390=ORIENTED_EDGE('',*,*,#5971,.F.);
#8391=ORIENTED_EDGE('',*,*,#5974,.F.);
#8392=ORIENTED_EDGE('',*,*,#5977,.F.);
#8393=ORIENTED_EDGE('',*,*,#5980,.F.);
#8394=ORIENTED_EDGE('',*,*,#6202,.F.);
#8395=ORIENTED_EDGE('',*,*,#6268,.T.);
#8396=ORIENTED_EDGE('',*,*,#6271,.T.);
#8397=ORIENTED_EDGE('',*,*,#6269,.T.);
#8398=ORIENTED_EDGE('',*,*,#6161,.T.);
#8399=ORIENTED_EDGE('',*,*,#6267,.F.);
#8400=ORIENTED_EDGE('',*,*,#6225,.T.);
#8401=ORIENTED_EDGE('',*,*,#6270,.T.);
#8402=ORIENTED_EDGE('',*,*,#6271,.F.);
#8403=ORIENTED_EDGE('',*,*,#5869,.F.);
#8404=ORIENTED_EDGE('',*,*,#6217,.T.);
#8405=ORIENTED_EDGE('',*,*,#6220,.T.);
#8406=ORIENTED_EDGE('',*,*,#6272,.T.);
#8407=ORIENTED_EDGE('',*,*,#6273,.F.);
#8408=ORIENTED_EDGE('',*,*,#6183,.F.);
#8409=ORIENTED_EDGE('',*,*,#6187,.F.);
#8410=ORIENTED_EDGE('',*,*,#6181,.F.);
#8411=ORIENTED_EDGE('',*,*,#6178,.F.);
#8412=ORIENTED_EDGE('',*,*,#6175,.F.);
#8413=ORIENTED_EDGE('',*,*,#6172,.F.);
#8414=ORIENTED_EDGE('',*,*,#6169,.F.);
#8415=ORIENTED_EDGE('',*,*,#6165,.F.);
#8416=ORIENTED_EDGE('',*,*,#6256,.F.);
#8417=ORIENTED_EDGE('',*,*,#6203,.F.);
#8418=ORIENTED_EDGE('',*,*,#5923,.F.);
#8419=ORIENTED_EDGE('',*,*,#5920,.F.);
#8420=ORIENTED_EDGE('',*,*,#5917,.F.);
#8421=ORIENTED_EDGE('',*,*,#5914,.F.);
#8422=ORIENTED_EDGE('',*,*,#5911,.F.);
#8423=ORIENTED_EDGE('',*,*,#5908,.F.);
#8424=ORIENTED_EDGE('',*,*,#5905,.F.);
#8425=ORIENTED_EDGE('',*,*,#5902,.F.);
#8426=ORIENTED_EDGE('',*,*,#5899,.F.);
#8427=ORIENTED_EDGE('',*,*,#5896,.F.);
#8428=ORIENTED_EDGE('',*,*,#5893,.F.);
#8429=ORIENTED_EDGE('',*,*,#5890,.F.);
#8430=ORIENTED_EDGE('',*,*,#5887,.F.);
#8431=ORIENTED_EDGE('',*,*,#5884,.F.);
#8432=ORIENTED_EDGE('',*,*,#5881,.F.);
#8433=ORIENTED_EDGE('',*,*,#5878,.F.);
#8434=ORIENTED_EDGE('',*,*,#5875,.F.);
#8435=ORIENTED_EDGE('',*,*,#5872,.F.);
#8436=ORIENTED_EDGE('',*,*,#6205,.F.);
#8437=ORIENTED_EDGE('',*,*,#6257,.F.);
#8438=ORIENTED_EDGE('',*,*,#6167,.T.);
#8439=ORIENTED_EDGE('',*,*,#6171,.T.);
#8440=ORIENTED_EDGE('',*,*,#6174,.T.);
#8441=ORIENTED_EDGE('',*,*,#6177,.T.);
#8442=ORIENTED_EDGE('',*,*,#6180,.T.);
#8443=ORIENTED_EDGE('',*,*,#6186,.T.);
#8444=ORIENTED_EDGE('',*,*,#6185,.T.);
#8445=ORIENTED_EDGE('',*,*,#6274,.F.);
#8446=ORIENTED_EDGE('',*,*,#6275,.F.);
#8447=ORIENTED_EDGE('',*,*,#6218,.T.);
#8448=ORIENTED_EDGE('',*,*,#5867,.F.);
#8449=ORIENTED_EDGE('',*,*,#5871,.F.);
#8450=ORIENTED_EDGE('',*,*,#5874,.F.);
#8451=ORIENTED_EDGE('',*,*,#5877,.F.);
#8452=ORIENTED_EDGE('',*,*,#5880,.F.);
#8453=ORIENTED_EDGE('',*,*,#5883,.F.);
#8454=ORIENTED_EDGE('',*,*,#5886,.F.);
#8455=ORIENTED_EDGE('',*,*,#5889,.F.);
#8456=ORIENTED_EDGE('',*,*,#5892,.F.);
#8457=ORIENTED_EDGE('',*,*,#5895,.F.);
#8458=ORIENTED_EDGE('',*,*,#5898,.F.);
#8459=ORIENTED_EDGE('',*,*,#5901,.F.);
#8460=ORIENTED_EDGE('',*,*,#5904,.F.);
#8461=ORIENTED_EDGE('',*,*,#5907,.F.);
#8462=ORIENTED_EDGE('',*,*,#5910,.F.);
#8463=ORIENTED_EDGE('',*,*,#5913,.F.);
#8464=ORIENTED_EDGE('',*,*,#5916,.F.);
#8465=ORIENTED_EDGE('',*,*,#5919,.F.);
#8466=ORIENTED_EDGE('',*,*,#5922,.F.);
#8467=ORIENTED_EDGE('',*,*,#6273,.T.);
#8468=ORIENTED_EDGE('',*,*,#6276,.T.);
#8469=ORIENTED_EDGE('',*,*,#6274,.T.);
#8470=ORIENTED_EDGE('',*,*,#6184,.T.);
#8471=ORIENTED_EDGE('',*,*,#6272,.F.);
#8472=ORIENTED_EDGE('',*,*,#6219,.T.);
#8473=ORIENTED_EDGE('',*,*,#6275,.T.);
#8474=ORIENTED_EDGE('',*,*,#6276,.F.);
#8475=ORIENTED_EDGE('',*,*,#6209,.T.);
#8476=ORIENTED_EDGE('',*,*,#6208,.T.);
#8477=ORIENTED_EDGE('',*,*,#6216,.T.);
#8478=ORIENTED_EDGE('',*,*,#6211,.F.);
#8479=ORIENTED_EDGE('',*,*,#6277,.F.);
#8480=ORIENTED_EDGE('',*,*,#6278,.T.);
#8481=ORIENTED_EDGE('',*,*,#6279,.T.);
#8482=ORIENTED_EDGE('',*,*,#6255,.T.);
#8483=ORIENTED_EDGE('',*,*,#6280,.F.);
#8484=ORIENTED_EDGE('',*,*,#6281,.T.);
#8485=ORIENTED_EDGE('',*,*,#6277,.T.);
#8486=ORIENTED_EDGE('',*,*,#6254,.T.);
#8487=ORIENTED_EDGE('',*,*,#6282,.T.);
#8488=ORIENTED_EDGE('',*,*,#6283,.F.);
#8489=ORIENTED_EDGE('',*,*,#6284,.F.);
#8490=ORIENTED_EDGE('',*,*,#6278,.F.);
#8491=ORIENTED_EDGE('',*,*,#6279,.F.);
#8492=ORIENTED_EDGE('',*,*,#6285,.T.);
#8493=ORIENTED_EDGE('',*,*,#6286,.T.);
#8494=ORIENTED_EDGE('',*,*,#6248,.T.);
#8495=ORIENTED_EDGE('',*,*,#6287,.F.);
#8496=ORIENTED_EDGE('',*,*,#6288,.T.);
#8497=ORIENTED_EDGE('',*,*,#6280,.T.);
#8498=ORIENTED_EDGE('',*,*,#6253,.T.);
#8499=ORIENTED_EDGE('',*,*,#6289,.T.);
#8500=ORIENTED_EDGE('',*,*,#6290,.F.);
#8501=ORIENTED_EDGE('',*,*,#6282,.F.);
#8502=ORIENTED_EDGE('',*,*,#6281,.F.);
#8503=ORIENTED_EDGE('',*,*,#6291,.F.);
#8504=ORIENTED_EDGE('',*,*,#6292,.T.);
#8505=ORIENTED_EDGE('',*,*,#6287,.T.);
#8506=ORIENTED_EDGE('',*,*,#6252,.F.);
#8507=ORIENTED_EDGE('',*,*,#6289,.F.);
#8508=ORIENTED_EDGE('',*,*,#6288,.F.);
#8509=ORIENTED_EDGE('',*,*,#6293,.F.);
#8510=ORIENTED_EDGE('',*,*,#6294,.F.);
#8511=ORIENTED_EDGE('',*,*,#6295,.F.);
#8512=ORIENTED_EDGE('',*,*,#6296,.T.);
#8513=ORIENTED_EDGE('',*,*,#6291,.T.);
#8514=ORIENTED_EDGE('',*,*,#6251,.T.);
#8515=ORIENTED_EDGE('',*,*,#6293,.T.);
#8516=ORIENTED_EDGE('',*,*,#6292,.F.);
#8517=ORIENTED_EDGE('',*,*,#6297,.F.);
#8518=ORIENTED_EDGE('',*,*,#6298,.F.);
#8519=ORIENTED_EDGE('',*,*,#6299,.F.);
#8520=ORIENTED_EDGE('',*,*,#6300,.T.);
#8521=ORIENTED_EDGE('',*,*,#6295,.T.);
#8522=ORIENTED_EDGE('',*,*,#6250,.T.);
#8523=ORIENTED_EDGE('',*,*,#6297,.T.);
#8524=ORIENTED_EDGE('',*,*,#6296,.F.);
#8525=ORIENTED_EDGE('',*,*,#6301,.F.);
#8526=ORIENTED_EDGE('',*,*,#6302,.F.);
#8527=ORIENTED_EDGE('',*,*,#6286,.F.);
#8528=ORIENTED_EDGE('',*,*,#6303,.T.);
#8529=ORIENTED_EDGE('',*,*,#6299,.T.);
#8530=ORIENTED_EDGE('',*,*,#6249,.T.);
#8531=ORIENTED_EDGE('',*,*,#6301,.T.);
#8532=ORIENTED_EDGE('',*,*,#6300,.F.);
#8533=ORIENTED_EDGE('',*,*,#6304,.F.);
#8534=ORIENTED_EDGE('',*,*,#6305,.F.);
#8535=ORIENTED_EDGE('',*,*,#6304,.T.);
#8536=ORIENTED_EDGE('',*,*,#6303,.F.);
#8537=ORIENTED_EDGE('',*,*,#6306,.T.);
#8538=ORIENTED_EDGE('',*,*,#6307,.F.);
#8539=ORIENTED_EDGE('',*,*,#6284,.T.);
#8540=ORIENTED_EDGE('',*,*,#6308,.F.);
#8541=ORIENTED_EDGE('',*,*,#6306,.F.);
#8542=ORIENTED_EDGE('',*,*,#6285,.F.);
#8543=ORIENTED_EDGE('',*,*,#6307,.T.);
#8544=ORIENTED_EDGE('',*,*,#6308,.T.);
#8545=ORIENTED_EDGE('',*,*,#6283,.T.);
#8546=ORIENTED_EDGE('',*,*,#6290,.T.);
#8547=ORIENTED_EDGE('',*,*,#6294,.T.);
#8548=ORIENTED_EDGE('',*,*,#6298,.T.);
#8549=ORIENTED_EDGE('',*,*,#6302,.T.);
#8550=ORIENTED_EDGE('',*,*,#6305,.T.);
#8551=ORIENTED_EDGE('',*,*,#6228,.T.);
#8552=ORIENTED_EDGE('',*,*,#6222,.T.);
#8553=ORIENTED_EDGE('',*,*,#6234,.T.);
#8554=ORIENTED_EDGE('',*,*,#6240,.T.);
#8555=ORIENTED_EDGE('',*,*,#6212,.T.);
#8556=ORIENTED_EDGE('',*,*,#6309,.F.);
#8557=ORIENTED_EDGE('',*,*,#6310,.F.);
#8558=ORIENTED_EDGE('',*,*,#6311,.F.);
#8559=ORIENTED_EDGE('',*,*,#6312,.F.);
#8560=ORIENTED_EDGE('',*,*,#6309,.T.);
#8561=ORIENTED_EDGE('',*,*,#6313,.F.);
#8562=ORIENTED_EDGE('',*,*,#6314,.F.);
#8563=ORIENTED_EDGE('',*,*,#6315,.F.);
#8564=ORIENTED_EDGE('',*,*,#6316,.T.);
#8565=ORIENTED_EDGE('',*,*,#6317,.T.);
#8566=ORIENTED_EDGE('',*,*,#6316,.F.);
#8567=ORIENTED_EDGE('',*,*,#6318,.T.);
#8568=ORIENTED_EDGE('',*,*,#6319,.T.);
#8569=ORIENTED_EDGE('',*,*,#6315,.T.);
#8570=ORIENTED_EDGE('',*,*,#6320,.T.);
#8571=ORIENTED_EDGE('',*,*,#6321,.T.);
#8572=ORIENTED_EDGE('',*,*,#6322,.T.);
#8573=ORIENTED_EDGE('',*,*,#6310,.T.);
#8574=ORIENTED_EDGE('',*,*,#6319,.F.);
#8575=ORIENTED_EDGE('',*,*,#6313,.T.);
#8576=ORIENTED_EDGE('',*,*,#6312,.T.);
#8577=ORIENTED_EDGE('',*,*,#6317,.F.);
#8578=ORIENTED_EDGE('',*,*,#6318,.F.);
#8579=ORIENTED_EDGE('',*,*,#6323,.T.);
#8580=ORIENTED_EDGE('',*,*,#6321,.F.);
#8581=ORIENTED_EDGE('',*,*,#6314,.T.);
#8582=ORIENTED_EDGE('',*,*,#6311,.T.);
#8583=ORIENTED_EDGE('',*,*,#6322,.F.);
#8584=ORIENTED_EDGE('',*,*,#6323,.F.);
#8585=ORIENTED_EDGE('',*,*,#6320,.F.);
#8586=ORIENTED_EDGE('',*,*,#6324,.F.);
#8587=ORIENTED_EDGE('',*,*,#6325,.T.);
#8588=ORIENTED_EDGE('',*,*,#6326,.T.);
#8589=ORIENTED_EDGE('',*,*,#6325,.F.);
#8590=ORIENTED_EDGE('',*,*,#6327,.F.);
#8591=ORIENTED_EDGE('',*,*,#6328,.T.);
#8592=ORIENTED_EDGE('',*,*,#6329,.F.);
#8593=ORIENTED_EDGE('',*,*,#6328,.F.);
#8594=ORIENTED_EDGE('',*,*,#6330,.F.);
#8595=ORIENTED_EDGE('',*,*,#6331,.T.);
#8596=ORIENTED_EDGE('',*,*,#6332,.F.);
#8597=ORIENTED_EDGE('',*,*,#6331,.F.);
#8598=ORIENTED_EDGE('',*,*,#6333,.F.);
#8599=ORIENTED_EDGE('',*,*,#6334,.T.);
#8600=ORIENTED_EDGE('',*,*,#6335,.F.);
#8601=ORIENTED_EDGE('',*,*,#6334,.F.);
#8602=ORIENTED_EDGE('',*,*,#6336,.F.);
#8603=ORIENTED_EDGE('',*,*,#6337,.T.);
#8604=ORIENTED_EDGE('',*,*,#6338,.F.);
#8605=ORIENTED_EDGE('',*,*,#6337,.F.);
#8606=ORIENTED_EDGE('',*,*,#6339,.F.);
#8607=ORIENTED_EDGE('',*,*,#6340,.T.);
#8608=ORIENTED_EDGE('',*,*,#6327,.T.);
#8609=ORIENTED_EDGE('',*,*,#6340,.F.);
#8610=ORIENTED_EDGE('',*,*,#6341,.F.);
#8611=ORIENTED_EDGE('',*,*,#6342,.T.);
#8612=ORIENTED_EDGE('',*,*,#6330,.T.);
#8613=ORIENTED_EDGE('',*,*,#6342,.F.);
#8614=ORIENTED_EDGE('',*,*,#6343,.F.);
#8615=ORIENTED_EDGE('',*,*,#6344,.T.);
#8616=ORIENTED_EDGE('',*,*,#6333,.T.);
#8617=ORIENTED_EDGE('',*,*,#6344,.F.);
#8618=ORIENTED_EDGE('',*,*,#6345,.F.);
#8619=ORIENTED_EDGE('',*,*,#6346,.T.);
#8620=ORIENTED_EDGE('',*,*,#6336,.T.);
#8621=ORIENTED_EDGE('',*,*,#6346,.F.);
#8622=ORIENTED_EDGE('',*,*,#6347,.F.);
#8623=ORIENTED_EDGE('',*,*,#6348,.T.);
#8624=ORIENTED_EDGE('',*,*,#6349,.F.);
#8625=ORIENTED_EDGE('',*,*,#6348,.F.);
#8626=ORIENTED_EDGE('',*,*,#6345,.T.);
#8627=ORIENTED_EDGE('',*,*,#6343,.T.);
#8628=ORIENTED_EDGE('',*,*,#6341,.T.);
#8629=ORIENTED_EDGE('',*,*,#6339,.T.);
#8630=ORIENTED_EDGE('',*,*,#6350,.T.);
#8631=ORIENTED_EDGE('',*,*,#6351,.T.);
#8632=ORIENTED_EDGE('',*,*,#6352,.T.);
#8633=ORIENTED_EDGE('',*,*,#6353,.T.);
#8634=ORIENTED_EDGE('',*,*,#6354,.T.);
#8635=ORIENTED_EDGE('',*,*,#6355,.F.);
#8636=ORIENTED_EDGE('',*,*,#6352,.F.);
#8637=ORIENTED_EDGE('',*,*,#6356,.T.);
#8638=ORIENTED_EDGE('',*,*,#6357,.T.);
#8639=ORIENTED_EDGE('',*,*,#6358,.F.);
#8640=ORIENTED_EDGE('',*,*,#6353,.F.);
#8641=ORIENTED_EDGE('',*,*,#6355,.T.);
#8642=ORIENTED_EDGE('',*,*,#6359,.T.);
#8643=ORIENTED_EDGE('',*,*,#6360,.F.);
#8644=ORIENTED_EDGE('',*,*,#6350,.F.);
#8645=ORIENTED_EDGE('',*,*,#6358,.T.);
#8646=ORIENTED_EDGE('',*,*,#6361,.T.);
#8647=ORIENTED_EDGE('',*,*,#6356,.F.);
#8648=ORIENTED_EDGE('',*,*,#6351,.F.);
#8649=ORIENTED_EDGE('',*,*,#6360,.T.);
#8650=ORIENTED_EDGE('',*,*,#6362,.T.);
#8651=ORIENTED_EDGE('',*,*,#6363,.T.);
#8652=ORIENTED_EDGE('',*,*,#6364,.T.);
#8653=ORIENTED_EDGE('',*,*,#6365,.T.);
#8654=ORIENTED_EDGE('',*,*,#6361,.F.);
#8655=ORIENTED_EDGE('',*,*,#6359,.F.);
#8656=ORIENTED_EDGE('',*,*,#6357,.F.);
#8657=ORIENTED_EDGE('',*,*,#6354,.F.);
#8658=ORIENTED_EDGE('',*,*,#6366,.T.);
#8659=ORIENTED_EDGE('',*,*,#6367,.T.);
#8660=ORIENTED_EDGE('',*,*,#6368,.F.);
#8661=ORIENTED_EDGE('',*,*,#6363,.F.);
#8662=ORIENTED_EDGE('',*,*,#6369,.T.);
#8663=ORIENTED_EDGE('',*,*,#6370,.T.);
#8664=ORIENTED_EDGE('',*,*,#6371,.T.);
#8665=ORIENTED_EDGE('',*,*,#6372,.T.);
#8666=ORIENTED_EDGE('',*,*,#6373,.T.);
#8667=ORIENTED_EDGE('',*,*,#6374,.T.);
#8668=ORIENTED_EDGE('',*,*,#6375,.T.);
#8669=ORIENTED_EDGE('',*,*,#6376,.T.);
#8670=ORIENTED_EDGE('',*,*,#6329,.T.);
#8671=ORIENTED_EDGE('',*,*,#6332,.T.);
#8672=ORIENTED_EDGE('',*,*,#6335,.T.);
#8673=ORIENTED_EDGE('',*,*,#6338,.T.);
#8674=ORIENTED_EDGE('',*,*,#6326,.F.);
#8675=ORIENTED_EDGE('',*,*,#6377,.T.);
#8676=ORIENTED_EDGE('',*,*,#6372,.F.);
#8677=ORIENTED_EDGE('',*,*,#6378,.F.);
#8678=ORIENTED_EDGE('',*,*,#6379,.F.);
#8679=ORIENTED_EDGE('',*,*,#6378,.T.);
#8680=ORIENTED_EDGE('',*,*,#6371,.F.);
#8681=ORIENTED_EDGE('',*,*,#6380,.F.);
#8682=ORIENTED_EDGE('',*,*,#6381,.F.);
#8683=ORIENTED_EDGE('',*,*,#6380,.T.);
#8684=ORIENTED_EDGE('',*,*,#6370,.F.);
#8685=ORIENTED_EDGE('',*,*,#6382,.T.);
#8686=ORIENTED_EDGE('',*,*,#6383,.F.);
#8687=ORIENTED_EDGE('',*,*,#6384,.T.);
#8688=ORIENTED_EDGE('',*,*,#6381,.T.);
#8689=ORIENTED_EDGE('',*,*,#6385,.F.);
#8690=ORIENTED_EDGE('',*,*,#6386,.F.);
#8691=ORIENTED_EDGE('',*,*,#6387,.T.);
#8692=ORIENTED_EDGE('',*,*,#6388,.F.);
#8693=ORIENTED_EDGE('',*,*,#6382,.F.);
#8694=ORIENTED_EDGE('',*,*,#6369,.F.);
#8695=ORIENTED_EDGE('',*,*,#6385,.T.);
#8696=ORIENTED_EDGE('',*,*,#6383,.T.);
#8697=ORIENTED_EDGE('',*,*,#6389,.F.);
#8698=ORIENTED_EDGE('',*,*,#6390,.F.);
#8699=ORIENTED_EDGE('',*,*,#6391,.T.);
#8700=ORIENTED_EDGE('',*,*,#6392,.F.);
#8701=ORIENTED_EDGE('',*,*,#6387,.F.);
#8702=ORIENTED_EDGE('',*,*,#6376,.F.);
#8703=ORIENTED_EDGE('',*,*,#6389,.T.);
#8704=ORIENTED_EDGE('',*,*,#6388,.T.);
#8705=ORIENTED_EDGE('',*,*,#6393,.F.);
#8706=ORIENTED_EDGE('',*,*,#6394,.T.);
#8707=ORIENTED_EDGE('',*,*,#6395,.T.);
#8708=ORIENTED_EDGE('',*,*,#6396,.F.);
#8709=ORIENTED_EDGE('',*,*,#6391,.F.);
#8710=ORIENTED_EDGE('',*,*,#6375,.F.);
#8711=ORIENTED_EDGE('',*,*,#6393,.T.);
#8712=ORIENTED_EDGE('',*,*,#6392,.T.);
#8713=ORIENTED_EDGE('',*,*,#6397,.F.);
#8714=ORIENTED_EDGE('',*,*,#6398,.F.);
#8715=ORIENTED_EDGE('',*,*,#6395,.F.);
#8716=ORIENTED_EDGE('',*,*,#6374,.F.);
#8717=ORIENTED_EDGE('',*,*,#6399,.F.);
#8718=ORIENTED_EDGE('',*,*,#6400,.F.);
#8719=ORIENTED_EDGE('',*,*,#6397,.T.);
#8720=ORIENTED_EDGE('',*,*,#6396,.T.);
#8721=ORIENTED_EDGE('',*,*,#6401,.F.);
#8722=ORIENTED_EDGE('',*,*,#6402,.F.);
#8723=ORIENTED_EDGE('',*,*,#6403,.T.);
#8724=ORIENTED_EDGE('',*,*,#6379,.T.);
#8725=ORIENTED_EDGE('',*,*,#6384,.F.);
#8726=ORIENTED_EDGE('',*,*,#6404,.F.);
#8727=ORIENTED_EDGE('',*,*,#6368,.T.);
#8728=ORIENTED_EDGE('',*,*,#6405,.T.);
#8729=ORIENTED_EDGE('',*,*,#6406,.T.);
#8730=ORIENTED_EDGE('',*,*,#6407,.F.);
#8731=ORIENTED_EDGE('',*,*,#6364,.F.);
#8732=ORIENTED_EDGE('',*,*,#6408,.T.);
#8733=ORIENTED_EDGE('',*,*,#6409,.F.);
#8734=ORIENTED_EDGE('',*,*,#6365,.F.);
#8735=ORIENTED_EDGE('',*,*,#6407,.T.);
#8736=ORIENTED_EDGE('',*,*,#6410,.T.);
#8737=ORIENTED_EDGE('',*,*,#6411,.T.);
#8738=ORIENTED_EDGE('',*,*,#6366,.F.);
#8739=ORIENTED_EDGE('',*,*,#6362,.F.);
#8740=ORIENTED_EDGE('',*,*,#6409,.T.);
#8741=ORIENTED_EDGE('',*,*,#6399,.T.);
#8742=ORIENTED_EDGE('',*,*,#6373,.F.);
#8743=ORIENTED_EDGE('',*,*,#6377,.F.);
#8744=ORIENTED_EDGE('',*,*,#6412,.F.);
#8745=ORIENTED_EDGE('',*,*,#6405,.F.);
#8746=ORIENTED_EDGE('',*,*,#6367,.F.);
#8747=ORIENTED_EDGE('',*,*,#6411,.F.);
#8748=ORIENTED_EDGE('',*,*,#6413,.F.);
#8749=ORIENTED_EDGE('',*,*,#6401,.T.);
#8750=ORIENTED_EDGE('',*,*,#6400,.T.);
#8751=ORIENTED_EDGE('',*,*,#6414,.F.);
#8752=ORIENTED_EDGE('',*,*,#6415,.F.);
#8753=ORIENTED_EDGE('',*,*,#6414,.T.);
#8754=ORIENTED_EDGE('',*,*,#6413,.T.);
#8755=ORIENTED_EDGE('',*,*,#6410,.F.);
#8756=ORIENTED_EDGE('',*,*,#6408,.F.);
#8757=ORIENTED_EDGE('',*,*,#6406,.F.);
#8758=ORIENTED_EDGE('',*,*,#6412,.T.);
#8759=ORIENTED_EDGE('',*,*,#6403,.F.);
#8760=ORIENTED_EDGE('',*,*,#6416,.F.);
#8761=ORIENTED_EDGE('',*,*,#6404,.T.);
#8762=ORIENTED_EDGE('',*,*,#6386,.T.);
#8763=ORIENTED_EDGE('',*,*,#6390,.T.);
#8764=ORIENTED_EDGE('',*,*,#6394,.F.);
#8765=ORIENTED_EDGE('',*,*,#6398,.T.);
#8766=ORIENTED_EDGE('',*,*,#6402,.T.);
#8767=ORIENTED_EDGE('',*,*,#6415,.T.);
#8768=ORIENTED_EDGE('',*,*,#6416,.T.);
#8769=ORIENTED_EDGE('',*,*,#6349,.T.);
#8770=ORIENTED_EDGE('',*,*,#6324,.T.);
#8771=ORIENTED_EDGE('',*,*,#6347,.T.);
#8772=ORIENTED_EDGE('',*,*,#6417,.T.);
#8773=ORIENTED_EDGE('',*,*,#6418,.T.);
#8774=ORIENTED_EDGE('',*,*,#6419,.T.);
#8775=ORIENTED_EDGE('',*,*,#6418,.F.);
#8776=ORIENTED_EDGE('',*,*,#6420,.F.);
#8777=ORIENTED_EDGE('',*,*,#6421,.T.);
#8778=ORIENTED_EDGE('',*,*,#6422,.T.);
#8779=ORIENTED_EDGE('',*,*,#6421,.F.);
#8780=ORIENTED_EDGE('',*,*,#6423,.F.);
#8781=ORIENTED_EDGE('',*,*,#6424,.T.);
#8782=ORIENTED_EDGE('',*,*,#6425,.T.);
#8783=ORIENTED_EDGE('',*,*,#6424,.F.);
#8784=ORIENTED_EDGE('',*,*,#6426,.F.);
#8785=ORIENTED_EDGE('',*,*,#6427,.T.);
#8786=ORIENTED_EDGE('',*,*,#6428,.T.);
#8787=ORIENTED_EDGE('',*,*,#6427,.F.);
#8788=ORIENTED_EDGE('',*,*,#6429,.F.);
#8789=ORIENTED_EDGE('',*,*,#6430,.T.);
#8790=ORIENTED_EDGE('',*,*,#6431,.T.);
#8791=ORIENTED_EDGE('',*,*,#6430,.F.);
#8792=ORIENTED_EDGE('',*,*,#6432,.T.);
#8793=ORIENTED_EDGE('',*,*,#6433,.T.);
#8794=ORIENTED_EDGE('',*,*,#6434,.F.);
#8795=ORIENTED_EDGE('',*,*,#6435,.F.);
#8796=ORIENTED_EDGE('',*,*,#6436,.F.);
#8797=ORIENTED_EDGE('',*,*,#6437,.T.);
#8798=ORIENTED_EDGE('',*,*,#6438,.T.);
#8799=ORIENTED_EDGE('',*,*,#6439,.T.);
#8800=ORIENTED_EDGE('',*,*,#6417,.F.);
#8801=ORIENTED_EDGE('',*,*,#6440,.F.);
#8802=ORIENTED_EDGE('',*,*,#6441,.F.);
#8803=ORIENTED_EDGE('',*,*,#6442,.F.);
#8804=ORIENTED_EDGE('',*,*,#6443,.F.);
#8805=ORIENTED_EDGE('',*,*,#6444,.T.);
#8806=ORIENTED_EDGE('',*,*,#6445,.T.);
#8807=ORIENTED_EDGE('',*,*,#6446,.T.);
#8808=ORIENTED_EDGE('',*,*,#6447,.F.);
#8809=ORIENTED_EDGE('',*,*,#6425,.F.);
#8810=ORIENTED_EDGE('',*,*,#6431,.F.);
#8811=ORIENTED_EDGE('',*,*,#6428,.F.);
#8812=ORIENTED_EDGE('',*,*,#6422,.F.);
#8813=ORIENTED_EDGE('',*,*,#6419,.F.);
#8814=ORIENTED_EDGE('',*,*,#6441,.T.);
#8815=ORIENTED_EDGE('',*,*,#6448,.F.);
#8816=ORIENTED_EDGE('',*,*,#6439,.F.);
#8817=ORIENTED_EDGE('',*,*,#6449,.T.);
#8818=ORIENTED_EDGE('',*,*,#6440,.T.);
#8819=ORIENTED_EDGE('',*,*,#6450,.F.);
#8820=ORIENTED_EDGE('',*,*,#6432,.F.);
#8821=ORIENTED_EDGE('',*,*,#6448,.T.);
#8822=ORIENTED_EDGE('',*,*,#6442,.T.);
#8823=ORIENTED_EDGE('',*,*,#6449,.F.);
#8824=ORIENTED_EDGE('',*,*,#6438,.F.);
#8825=ORIENTED_EDGE('',*,*,#6451,.T.);
#8826=ORIENTED_EDGE('',*,*,#6446,.F.);
#8827=ORIENTED_EDGE('',*,*,#6452,.F.);
#8828=ORIENTED_EDGE('',*,*,#6434,.T.);
#8829=ORIENTED_EDGE('',*,*,#6453,.T.);
#8830=ORIENTED_EDGE('',*,*,#6444,.F.);
#8831=ORIENTED_EDGE('',*,*,#6454,.F.);
#8832=ORIENTED_EDGE('',*,*,#6436,.T.);
#8833=ORIENTED_EDGE('',*,*,#6455,.T.);
#8834=ORIENTED_EDGE('',*,*,#6443,.T.);
#8835=ORIENTED_EDGE('',*,*,#6451,.F.);
#8836=ORIENTED_EDGE('',*,*,#6437,.F.);
#8837=ORIENTED_EDGE('',*,*,#6454,.T.);
#8838=ORIENTED_EDGE('',*,*,#6445,.F.);
#8839=ORIENTED_EDGE('',*,*,#6455,.F.);
#8840=ORIENTED_EDGE('',*,*,#6435,.T.);
#8841=ORIENTED_EDGE('',*,*,#6452,.T.);
#8842=ORIENTED_EDGE('',*,*,#6447,.T.);
#8843=ORIENTED_EDGE('',*,*,#6453,.F.);
#8844=ORIENTED_EDGE('',*,*,#6433,.F.);
#8845=ORIENTED_EDGE('',*,*,#6450,.T.);
#8846=ORIENTED_EDGE('',*,*,#6420,.T.);
#8847=ORIENTED_EDGE('',*,*,#6423,.T.);
#8848=ORIENTED_EDGE('',*,*,#6426,.T.);
#8849=ORIENTED_EDGE('',*,*,#6429,.T.);
#10414=CYLINDRICAL_SURFACE('',#11440,3.175);
#10415=CYLINDRICAL_SURFACE('',#11476,3.175);
#10416=CYLINDRICAL_SURFACE('',#11512,3.175);
#10417=CYLINDRICAL_SURFACE('',#11548,3.175);
#10418=CYLINDRICAL_SURFACE('',#11584,1.905);
#10419=CYLINDRICAL_SURFACE('',#11586,1.905);
#10420=CYLINDRICAL_SURFACE('',#11587,1.905);
#10421=CYLINDRICAL_SURFACE('',#11588,1.905);
#10422=CYLINDRICAL_SURFACE('',#11589,1.905);
#10423=CYLINDRICAL_SURFACE('',#11590,1.905);
#10424=CYLINDRICAL_SURFACE('',#11591,1.905);
#10425=CYLINDRICAL_SURFACE('',#11592,1.905);
#10426=CYLINDRICAL_SURFACE('',#11593,1.905);
#10427=CYLINDRICAL_SURFACE('',#11594,1.905);
#10428=CYLINDRICAL_SURFACE('',#11595,1.905);
#10429=CYLINDRICAL_SURFACE('',#11596,1.905);
#10430=CYLINDRICAL_SURFACE('',#11597,1.905);
#10431=CYLINDRICAL_SURFACE('',#11598,1.905);
#10432=CYLINDRICAL_SURFACE('',#11599,1.905);
#10433=CYLINDRICAL_SURFACE('',#11600,1.905);
#10434=CYLINDRICAL_SURFACE('',#11601,1.905);
#10435=CYLINDRICAL_SURFACE('',#11602,1.905);
#10436=CYLINDRICAL_SURFACE('',#11603,1.905);
#10437=CYLINDRICAL_SURFACE('',#11604,1.905);
#10438=CYLINDRICAL_SURFACE('',#11606,1.905);
#10439=CYLINDRICAL_SURFACE('',#11607,1.905);
#10440=CYLINDRICAL_SURFACE('',#11608,1.905);
#10441=CYLINDRICAL_SURFACE('',#11609,1.905);
#10442=CYLINDRICAL_SURFACE('',#11610,1.905);
#10443=CYLINDRICAL_SURFACE('',#11611,1.905);
#10444=CYLINDRICAL_SURFACE('',#11612,1.905);
#10445=CYLINDRICAL_SURFACE('',#11613,1.905);
#10446=CYLINDRICAL_SURFACE('',#11614,1.905);
#10447=CYLINDRICAL_SURFACE('',#11615,1.905);
#10448=CYLINDRICAL_SURFACE('',#11616,1.905);
#10449=CYLINDRICAL_SURFACE('',#11617,1.905);
#10450=CYLINDRICAL_SURFACE('',#11618,1.905);
#10451=CYLINDRICAL_SURFACE('',#11619,1.905);
#10452=CYLINDRICAL_SURFACE('',#11620,1.905);
#10453=CYLINDRICAL_SURFACE('',#11621,1.905);
#10454=CYLINDRICAL_SURFACE('',#11622,1.905);
#10455=CYLINDRICAL_SURFACE('',#11623,1.905);
#10456=CYLINDRICAL_SURFACE('',#11624,1.905);
#10457=CYLINDRICAL_SURFACE('',#11626,1.905);
#10458=CYLINDRICAL_SURFACE('',#11627,1.905);
#10459=CYLINDRICAL_SURFACE('',#11628,1.905);
#10460=CYLINDRICAL_SURFACE('',#11629,1.905);
#10461=CYLINDRICAL_SURFACE('',#11630,1.905);
#10462=CYLINDRICAL_SURFACE('',#11631,1.905);
#10463=CYLINDRICAL_SURFACE('',#11632,1.905);
#10464=CYLINDRICAL_SURFACE('',#11633,1.905);
#10465=CYLINDRICAL_SURFACE('',#11634,1.905);
#10466=CYLINDRICAL_SURFACE('',#11635,1.905);
#10467=CYLINDRICAL_SURFACE('',#11636,1.905);
#10468=CYLINDRICAL_SURFACE('',#11637,1.905);
#10469=CYLINDRICAL_SURFACE('',#11638,1.905);
#10470=CYLINDRICAL_SURFACE('',#11639,1.905);
#10471=CYLINDRICAL_SURFACE('',#11640,1.905);
#10472=CYLINDRICAL_SURFACE('',#11641,1.905);
#10473=CYLINDRICAL_SURFACE('',#11642,1.905);
#10474=CYLINDRICAL_SURFACE('',#11643,1.905);
#10475=CYLINDRICAL_SURFACE('',#11644,1.905);
#10476=CYLINDRICAL_SURFACE('',#11646,1.905);
#10477=CYLINDRICAL_SURFACE('',#11647,1.905);
#10478=CYLINDRICAL_SURFACE('',#11648,1.905);
#10479=CYLINDRICAL_SURFACE('',#11649,1.905);
#10480=CYLINDRICAL_SURFACE('',#11650,1.905);
#10481=CYLINDRICAL_SURFACE('',#11651,1.905);
#10482=CYLINDRICAL_SURFACE('',#11652,1.905);
#10483=CYLINDRICAL_SURFACE('',#11653,1.905);
#10484=CYLINDRICAL_SURFACE('',#11654,1.905);
#10485=CYLINDRICAL_SURFACE('',#11655,1.905);
#10486=CYLINDRICAL_SURFACE('',#11656,1.905);
#10487=CYLINDRICAL_SURFACE('',#11657,1.905);
#10488=CYLINDRICAL_SURFACE('',#11658,1.905);
#10489=CYLINDRICAL_SURFACE('',#11659,1.905);
#10490=CYLINDRICAL_SURFACE('',#11660,1.905);
#10491=CYLINDRICAL_SURFACE('',#11661,1.905);
#10492=CYLINDRICAL_SURFACE('',#11662,1.905);
#10493=CYLINDRICAL_SURFACE('',#11663,1.93206329386826);
#10494=CYLINDRICAL_SURFACE('',#11665,1.93206329386826);
#10495=CYLINDRICAL_SURFACE('',#11667,1.93206329386826);
#10496=CYLINDRICAL_SURFACE('',#11668,1.93206329386826);
#10497=CYLINDRICAL_SURFACE('',#11669,1.93206329386826);
#10498=CYLINDRICAL_SURFACE('',#11670,1.93206329386826);
#10499=CYLINDRICAL_SURFACE('',#11671,1.93206329386826);
#10500=CYLINDRICAL_SURFACE('',#11672,1.93206329386825);
#10501=CYLINDRICAL_SURFACE('',#11674,1.93206329386825);
#10502=CYLINDRICAL_SURFACE('',#11676,1.93206329386825);
#10503=CYLINDRICAL_SURFACE('',#11677,1.93206329386825);
#10504=CYLINDRICAL_SURFACE('',#11678,1.93206329386825);
#10505=CYLINDRICAL_SURFACE('',#11679,1.93206329386825);
#10506=CYLINDRICAL_SURFACE('',#11680,1.93206329386825);
#10507=CYLINDRICAL_SURFACE('',#11681,1.93206329386826);
#10508=CYLINDRICAL_SURFACE('',#11683,1.93206329386826);
#10509=CYLINDRICAL_SURFACE('',#11685,1.93206329386826);
#10510=CYLINDRICAL_SURFACE('',#11686,1.93206329386826);
#10511=CYLINDRICAL_SURFACE('',#11687,1.93206329386826);
#10512=CYLINDRICAL_SURFACE('',#11688,1.93206329386826);
#10513=CYLINDRICAL_SURFACE('',#11689,1.93206329386826);
#10514=CYLINDRICAL_SURFACE('',#11690,1.93206329386822);
#10515=CYLINDRICAL_SURFACE('',#11692,1.93206329386822);
#10516=CYLINDRICAL_SURFACE('',#11694,1.93206329386822);
#10517=CYLINDRICAL_SURFACE('',#11695,1.93206329386822);
#10518=CYLINDRICAL_SURFACE('',#11696,1.93206329386822);
#10519=CYLINDRICAL_SURFACE('',#11697,1.93206329386822);
#10520=CYLINDRICAL_SURFACE('',#11698,1.93206329386822);
#10521=CYLINDRICAL_SURFACE('',#11699,1.93206329386822);
#10522=CYLINDRICAL_SURFACE('',#11700,1.93206329386826);
#10523=CYLINDRICAL_SURFACE('',#11701,1.93206329386825);
#10524=CYLINDRICAL_SURFACE('',#11702,1.93206329386826);
#10525=CYLINDRICAL_SURFACE('',#11703,1.905);
#10526=CYLINDRICAL_SURFACE('',#11705,1.905);
#10527=CYLINDRICAL_SURFACE('',#11707,1.905);
#10528=CYLINDRICAL_SURFACE('',#11709,1.905);
#10529=CYLINDRICAL_SURFACE('',#11711,2.62699999999999);
#10530=CYLINDRICAL_SURFACE('',#11714,3.76999999999999);
#10531=CYLINDRICAL_SURFACE('',#11720,10.985);
#10532=CYLINDRICAL_SURFACE('',#11751,0.762);
#10533=CYLINDRICAL_SURFACE('',#11756,0.761999999999999);
#10534=CYLINDRICAL_SURFACE('',#11759,0.762);
#10535=CYLINDRICAL_SURFACE('',#11762,0.761999999999999);
#10536=CYLINDRICAL_SURFACE('',#11765,0.762);
#10537=CYLINDRICAL_SURFACE('',#11768,0.762000000000001);
#10538=CYLINDRICAL_SURFACE('',#11770,0.762);
#10539=CYLINDRICAL_SURFACE('',#11772,0.762000000000001);
#10540=CYLINDRICAL_SURFACE('',#11782,2.5);
#10541=CYLINDRICAL_SURFACE('',#11789,5.16699999999999);
#10542=CYLINDRICAL_SURFACE('',#11804,3.175);
#10543=CYLINDRICAL_SURFACE('',#11806,3.175);
#10544=CYLINDRICAL_SURFACE('',#11808,3.175);
#10545=CYLINDRICAL_SURFACE('',#11810,3.175);
#10546=CYLINDRICAL_SURFACE('',#11812,2.62699999999999);
#10547=CYLINDRICAL_SURFACE('',#11827,0.762);
#10548=CYLINDRICAL_SURFACE('',#11830,0.761999999999999);
#10549=CYLINDRICAL_SURFACE('',#11832,0.762);
#10550=CYLINDRICAL_SURFACE('',#11835,0.761999999999999);
#10551=CYLINDRICAL_SURFACE('',#11838,0.762);
#10552=CYLINDRICAL_SURFACE('',#11841,0.761999999999999);
#10553=CYLINDRICAL_SURFACE('',#11844,0.762);
#10554=CYLINDRICAL_SURFACE('',#11853,0.761999999999999);
#10555=CYLINDRICAL_SURFACE('',#11858,2.62699999999999);
#10556=CYLINDRICAL_SURFACE('',#11861,1.905);
#10557=CYLINDRICAL_SURFACE('',#11864,1.905);
#10558=CYLINDRICAL_SURFACE('',#11867,1.905);
#10559=CYLINDRICAL_SURFACE('',#11870,1.905);
#10648=ADVANCED_FACE('',(#1027),#10414,.T.);
#10649=ADVANCED_FACE('',(#1028),#1019,.T.);
#10650=ADVANCED_FACE('',(#1029),#390,.T.);
#10651=ADVANCED_FACE('',(#1030),#391,.T.);
#10652=ADVANCED_FACE('',(#1031),#392,.T.);
#10653=ADVANCED_FACE('',(#1032),#393,.F.);
#10654=ADVANCED_FACE('',(#1033),#394,.T.);
#10655=ADVANCED_FACE('',(#1034),#395,.F.);
#10656=ADVANCED_FACE('',(#1035),#396,.T.);
#10657=ADVANCED_FACE('',(#1036),#397,.F.);
#10658=ADVANCED_FACE('',(#1037),#398,.T.);
#10659=ADVANCED_FACE('',(#1038),#399,.T.);
#10660=ADVANCED_FACE('',(#1039),#400,.T.);
#10661=ADVANCED_FACE('',(#1040),#401,.T.);
#10662=ADVANCED_FACE('',(#1041),#402,.T.);
#10663=ADVANCED_FACE('',(#1042),#403,.T.);
#10664=ADVANCED_FACE('',(#1043),#404,.F.);
#10665=ADVANCED_FACE('',(#1044),#405,.F.);
#10666=ADVANCED_FACE('',(#1045),#406,.T.);
#10667=ADVANCED_FACE('',(#1046),#407,.T.);
#10668=ADVANCED_FACE('',(#1047),#10415,.T.);
#10669=ADVANCED_FACE('',(#1048),#1020,.T.);
#10670=ADVANCED_FACE('',(#1049),#408,.T.);
#10671=ADVANCED_FACE('',(#1050),#409,.T.);
#10672=ADVANCED_FACE('',(#1051),#410,.T.);
#10673=ADVANCED_FACE('',(#1052),#411,.F.);
#10674=ADVANCED_FACE('',(#1053),#412,.T.);
#10675=ADVANCED_FACE('',(#1054),#413,.F.);
#10676=ADVANCED_FACE('',(#1055),#414,.T.);
#10677=ADVANCED_FACE('',(#1056),#415,.F.);
#10678=ADVANCED_FACE('',(#1057),#416,.T.);
#10679=ADVANCED_FACE('',(#1058),#417,.T.);
#10680=ADVANCED_FACE('',(#1059),#418,.T.);
#10681=ADVANCED_FACE('',(#1060),#419,.T.);
#10682=ADVANCED_FACE('',(#1061),#420,.T.);
#10683=ADVANCED_FACE('',(#1062),#421,.T.);
#10684=ADVANCED_FACE('',(#1063),#422,.F.);
#10685=ADVANCED_FACE('',(#1064),#423,.F.);
#10686=ADVANCED_FACE('',(#1065),#424,.T.);
#10687=ADVANCED_FACE('',(#1066),#425,.T.);
#10688=ADVANCED_FACE('',(#1067),#10416,.T.);
#10689=ADVANCED_FACE('',(#1068),#1021,.T.);
#10690=ADVANCED_FACE('',(#1069),#426,.T.);
#10691=ADVANCED_FACE('',(#1070),#427,.T.);
#10692=ADVANCED_FACE('',(#1071),#428,.T.);
#10693=ADVANCED_FACE('',(#1072),#429,.F.);
#10694=ADVANCED_FACE('',(#1073),#430,.T.);
#10695=ADVANCED_FACE('',(#1074),#431,.F.);
#10696=ADVANCED_FACE('',(#1075),#432,.T.);
#10697=ADVANCED_FACE('',(#1076),#433,.F.);
#10698=ADVANCED_FACE('',(#1077),#434,.T.);
#10699=ADVANCED_FACE('',(#1078),#435,.T.);
#10700=ADVANCED_FACE('',(#1079),#436,.T.);
#10701=ADVANCED_FACE('',(#1080),#437,.T.);
#10702=ADVANCED_FACE('',(#1081),#438,.T.);
#10703=ADVANCED_FACE('',(#1082),#439,.T.);
#10704=ADVANCED_FACE('',(#1083),#440,.F.);
#10705=ADVANCED_FACE('',(#1084),#441,.F.);
#10706=ADVANCED_FACE('',(#1085),#442,.T.);
#10707=ADVANCED_FACE('',(#1086),#443,.T.);
#10708=ADVANCED_FACE('',(#1087),#10417,.T.);
#10709=ADVANCED_FACE('',(#1088),#1022,.T.);
#10710=ADVANCED_FACE('',(#1089),#444,.T.);
#10711=ADVANCED_FACE('',(#1090),#445,.T.);
#10712=ADVANCED_FACE('',(#1091),#446,.T.);
#10713=ADVANCED_FACE('',(#1092),#447,.F.);
#10714=ADVANCED_FACE('',(#1093),#448,.T.);
#10715=ADVANCED_FACE('',(#1094),#449,.F.);
#10716=ADVANCED_FACE('',(#1095),#450,.T.);
#10717=ADVANCED_FACE('',(#1096),#451,.F.);
#10718=ADVANCED_FACE('',(#1097),#452,.T.);
#10719=ADVANCED_FACE('',(#1098),#453,.T.);
#10720=ADVANCED_FACE('',(#1099),#454,.T.);
#10721=ADVANCED_FACE('',(#1100),#455,.T.);
#10722=ADVANCED_FACE('',(#1101),#456,.T.);
#10723=ADVANCED_FACE('',(#1102),#457,.T.);
#10724=ADVANCED_FACE('',(#1103),#458,.F.);
#10725=ADVANCED_FACE('',(#1104),#459,.F.);
#10726=ADVANCED_FACE('',(#1105),#460,.T.);
#10727=ADVANCED_FACE('',(#1106),#461,.T.);
#10728=ADVANCED_FACE('',(#1107),#10418,.F.);
#10729=ADVANCED_FACE('',(#1108),#10419,.F.);
#10730=ADVANCED_FACE('',(#1109),#10420,.F.);
#10731=ADVANCED_FACE('',(#1110),#10421,.F.);
#10732=ADVANCED_FACE('',(#1111),#10422,.F.);
#10733=ADVANCED_FACE('',(#1112),#10423,.F.);
#10734=ADVANCED_FACE('',(#1113),#10424,.F.);
#10735=ADVANCED_FACE('',(#1114),#10425,.F.);
#10736=ADVANCED_FACE('',(#1115),#10426,.F.);
#10737=ADVANCED_FACE('',(#1116),#10427,.F.);
#10738=ADVANCED_FACE('',(#1117),#10428,.F.);
#10739=ADVANCED_FACE('',(#1118),#10429,.F.);
#10740=ADVANCED_FACE('',(#1119),#10430,.F.);
#10741=ADVANCED_FACE('',(#1120),#10431,.F.);
#10742=ADVANCED_FACE('',(#1121),#10432,.F.);
#10743=ADVANCED_FACE('',(#1122),#10433,.F.);
#10744=ADVANCED_FACE('',(#1123),#10434,.F.);
#10745=ADVANCED_FACE('',(#1124),#10435,.F.);
#10746=ADVANCED_FACE('',(#1125),#10436,.F.);
#10747=ADVANCED_FACE('',(#1126),#10437,.F.);
#10748=ADVANCED_FACE('',(#1127),#10438,.F.);
#10749=ADVANCED_FACE('',(#1128),#10439,.F.);
#10750=ADVANCED_FACE('',(#1129),#10440,.F.);
#10751=ADVANCED_FACE('',(#1130),#10441,.F.);
#10752=ADVANCED_FACE('',(#1131),#10442,.F.);
#10753=ADVANCED_FACE('',(#1132),#10443,.F.);
#10754=ADVANCED_FACE('',(#1133),#10444,.F.);
#10755=ADVANCED_FACE('',(#1134),#10445,.F.);
#10756=ADVANCED_FACE('',(#1135),#10446,.F.);
#10757=ADVANCED_FACE('',(#1136),#10447,.F.);
#10758=ADVANCED_FACE('',(#1137),#10448,.F.);
#10759=ADVANCED_FACE('',(#1138),#10449,.F.);
#10760=ADVANCED_FACE('',(#1139),#10450,.F.);
#10761=ADVANCED_FACE('',(#1140),#10451,.F.);
#10762=ADVANCED_FACE('',(#1141),#10452,.F.);
#10763=ADVANCED_FACE('',(#1142),#10453,.F.);
#10764=ADVANCED_FACE('',(#1143),#10454,.F.);
#10765=ADVANCED_FACE('',(#1144),#10455,.F.);
#10766=ADVANCED_FACE('',(#1145),#10456,.F.);
#10767=ADVANCED_FACE('',(#1146),#10457,.F.);
#10768=ADVANCED_FACE('',(#1147),#10458,.F.);
#10769=ADVANCED_FACE('',(#1148),#10459,.F.);
#10770=ADVANCED_FACE('',(#1149),#10460,.F.);
#10771=ADVANCED_FACE('',(#1150),#10461,.F.);
#10772=ADVANCED_FACE('',(#1151),#10462,.F.);
#10773=ADVANCED_FACE('',(#1152),#10463,.F.);
#10774=ADVANCED_FACE('',(#1153),#10464,.F.);
#10775=ADVANCED_FACE('',(#1154),#10465,.F.);
#10776=ADVANCED_FACE('',(#1155),#10466,.F.);
#10777=ADVANCED_FACE('',(#1156),#10467,.F.);
#10778=ADVANCED_FACE('',(#1157),#10468,.F.);
#10779=ADVANCED_FACE('',(#1158),#10469,.F.);
#10780=ADVANCED_FACE('',(#1159),#10470,.F.);
#10781=ADVANCED_FACE('',(#1160),#10471,.F.);
#10782=ADVANCED_FACE('',(#1161),#10472,.F.);
#10783=ADVANCED_FACE('',(#1162),#10473,.F.);
#10784=ADVANCED_FACE('',(#1163),#10474,.F.);
#10785=ADVANCED_FACE('',(#1164),#10475,.F.);
#10786=ADVANCED_FACE('',(#1165),#10476,.F.);
#10787=ADVANCED_FACE('',(#1166),#10477,.F.);
#10788=ADVANCED_FACE('',(#1167),#10478,.F.);
#10789=ADVANCED_FACE('',(#1168),#10479,.F.);
#10790=ADVANCED_FACE('',(#1169),#10480,.F.);
#10791=ADVANCED_FACE('',(#1170),#10481,.F.);
#10792=ADVANCED_FACE('',(#1171),#10482,.F.);
#10793=ADVANCED_FACE('',(#1172),#10483,.F.);
#10794=ADVANCED_FACE('',(#1173),#10484,.F.);
#10795=ADVANCED_FACE('',(#1174),#10485,.F.);
#10796=ADVANCED_FACE('',(#1175),#10486,.F.);
#10797=ADVANCED_FACE('',(#1176),#10487,.F.);
#10798=ADVANCED_FACE('',(#1177),#10488,.F.);
#10799=ADVANCED_FACE('',(#1178),#10489,.F.);
#10800=ADVANCED_FACE('',(#1179),#10490,.F.);
#10801=ADVANCED_FACE('',(#1180),#10491,.F.);
#10802=ADVANCED_FACE('',(#1181),#10492,.F.);
#10803=ADVANCED_FACE('',(#1182),#10493,.T.);
#10804=ADVANCED_FACE('',(#1183),#10494,.T.);
#10805=ADVANCED_FACE('',(#1184),#10495,.T.);
#10806=ADVANCED_FACE('',(#1185),#10496,.T.);
#10807=ADVANCED_FACE('',(#1186),#10497,.T.);
#10808=ADVANCED_FACE('',(#1187),#10498,.T.);
#10809=ADVANCED_FACE('',(#1188),#10499,.T.);
#10810=ADVANCED_FACE('',(#1189),#10500,.T.);
#10811=ADVANCED_FACE('',(#1190),#10501,.T.);
#10812=ADVANCED_FACE('',(#1191),#10502,.T.);
#10813=ADVANCED_FACE('',(#1192),#10503,.T.);
#10814=ADVANCED_FACE('',(#1193),#10504,.T.);
#10815=ADVANCED_FACE('',(#1194),#10505,.T.);
#10816=ADVANCED_FACE('',(#1195),#10506,.T.);
#10817=ADVANCED_FACE('',(#1196),#10507,.T.);
#10818=ADVANCED_FACE('',(#1197),#10508,.T.);
#10819=ADVANCED_FACE('',(#1198),#10509,.T.);
#10820=ADVANCED_FACE('',(#1199),#10510,.T.);
#10821=ADVANCED_FACE('',(#1200),#10511,.T.);
#10822=ADVANCED_FACE('',(#1201),#10512,.T.);
#10823=ADVANCED_FACE('',(#1202),#10513,.T.);
#10824=ADVANCED_FACE('',(#1203),#10514,.T.);
#10825=ADVANCED_FACE('',(#1204),#10515,.T.);
#10826=ADVANCED_FACE('',(#1205),#10516,.T.);
#10827=ADVANCED_FACE('',(#1206),#10517,.T.);
#10828=ADVANCED_FACE('',(#1207),#10518,.T.);
#10829=ADVANCED_FACE('',(#1208),#10519,.T.);
#10830=ADVANCED_FACE('',(#1209),#10520,.T.);
#10831=ADVANCED_FACE('',(#1210),#10521,.T.);
#10832=ADVANCED_FACE('',(#1211),#10522,.T.);
#10833=ADVANCED_FACE('',(#1212),#10523,.T.);
#10834=ADVANCED_FACE('',(#1213),#10524,.T.);
#10835=ADVANCED_FACE('',(#1214),#10525,.F.);
#10836=ADVANCED_FACE('',(#1215),#10526,.F.);
#10837=ADVANCED_FACE('',(#1216),#10527,.F.);
#10838=ADVANCED_FACE('',(#1217),#10528,.F.);
#10839=ADVANCED_FACE('',(#1218),#10529,.F.);
#10840=ADVANCED_FACE('',(#1219),#10530,.F.);
#10841=ADVANCED_FACE('',(#1220),#301,.T.);
#10842=ADVANCED_FACE('',(#1221),#10531,.T.);
#10843=ADVANCED_FACE('',(#1222),#302,.F.);
#10844=ADVANCED_FACE('',(#1223),#303,.F.);
#10845=ADVANCED_FACE('',(#1224),#304,.F.);
#10846=ADVANCED_FACE('',(#1225),#305,.F.);
#10847=ADVANCED_FACE('',(#1226),#289,.F.);
#10848=ADVANCED_FACE('',(#1227),#290,.F.);
#10849=ADVANCED_FACE('',(#1228),#462,.F.);
#10850=ADVANCED_FACE('',(#1229),#291,.F.);
#10851=ADVANCED_FACE('',(#1230,#132,#133,#134,#135,#136),#463,.F.);
#10852=ADVANCED_FACE('',(#1231),#292,.F.);
#10853=ADVANCED_FACE('',(#1232),#293,.F.);
#10854=ADVANCED_FACE('',(#1233),#464,.F.);
#10855=ADVANCED_FACE('',(#1234),#294,.F.);
#10856=ADVANCED_FACE('',(#1235),#295,.F.);
#10857=ADVANCED_FACE('',(#1236),#296,.F.);
#10858=ADVANCED_FACE('',(#1237),#465,.F.);
#10859=ADVANCED_FACE('',(#1238),#297,.F.);
#10860=ADVANCED_FACE('',(#1239),#298,.F.);
#10861=ADVANCED_FACE('',(#1240),#299,.F.);
#10862=ADVANCED_FACE('',(#1241),#466,.F.);
#10863=ADVANCED_FACE('',(#1242),#300,.F.);
#10864=ADVANCED_FACE('',(#1243,#137),#467,.T.);
#10865=ADVANCED_FACE('',(#1244,#138),#468,.T.);
#10866=ADVANCED_FACE('',(#1245),#469,.F.);
#10867=ADVANCED_FACE('',(#1246),#470,.F.);
#10868=ADVANCED_FACE('',(#1247),#10532,.T.);
#10869=ADVANCED_FACE('',(#1248),#471,.F.);
#10870=ADVANCED_FACE('',(#1249),#472,.F.);
#10871=ADVANCED_FACE('',(#1250),#10533,.T.);
#10872=ADVANCED_FACE('',(#1251),#473,.F.);
#10873=ADVANCED_FACE('',(#1252),#10534,.T.);
#10874=ADVANCED_FACE('',(#1253),#474,.F.);
#10875=ADVANCED_FACE('',(#1254),#10535,.T.);
#10876=ADVANCED_FACE('',(#1255),#475,.F.);
#10877=ADVANCED_FACE('',(#1256),#10536,.T.);
#10878=ADVANCED_FACE('',(#1257),#476,.F.);
#10879=ADVANCED_FACE('',(#1258),#10537,.T.);
#10880=ADVANCED_FACE('',(#1259),#10538,.T.);
#10881=ADVANCED_FACE('',(#1260),#10539,.T.);
#10882=ADVANCED_FACE('',(#1261,#139,#140,#141,#142,#143),#477,.F.);
#10883=ADVANCED_FACE('',(#1262),#306,.T.);
#10884=ADVANCED_FACE('',(#1263),#307,.T.);
#10885=ADVANCED_FACE('',(#1264),#308,.F.);
#10886=ADVANCED_FACE('',(#1265),#10540,.T.);
#10887=ADVANCED_FACE('',(#1266,#144),#478,.T.);
#10888=ADVANCED_FACE('',(#1267),#479,.T.);
#10889=ADVANCED_FACE('',(#1268),#480,.F.);
#10890=ADVANCED_FACE('',(#1269),#481,.F.);
#10891=ADVANCED_FACE('',(#1270),#10541,.F.);
#10892=ADVANCED_FACE('',(#1271),#309,.F.);
#10893=ADVANCED_FACE('',(#1272),#310,.F.);
#10894=ADVANCED_FACE('',(#1273),#311,.F.);
#10895=ADVANCED_FACE('',(#1274),#312,.F.);
#10896=ADVANCED_FACE('',(#1275),#10542,.F.);
#10897=ADVANCED_FACE('',(#1276),#10543,.F.);
#10898=ADVANCED_FACE('',(#1277),#10544,.F.);
#10899=ADVANCED_FACE('',(#1278),#10545,.F.);
#10900=ADVANCED_FACE('',(#1279),#10546,.F.);
#10901=ADVANCED_FACE('',(#1280),#482,.T.);
#10902=ADVANCED_FACE('',(#1281),#483,.T.);
#10903=ADVANCED_FACE('',(#1282),#484,.T.);
#10904=ADVANCED_FACE('',(#1283),#485,.T.);
#10905=ADVANCED_FACE('',(#1284),#486,.T.);
#10906=ADVANCED_FACE('',(#1285),#487,.F.);
#10907=ADVANCED_FACE('',(#1286),#488,.F.);
#10908=ADVANCED_FACE('',(#1287),#489,.F.);
#10909=ADVANCED_FACE('',(#1288),#490,.F.);
#10910=ADVANCED_FACE('',(#1289,#145),#491,.F.);
#10911=ADVANCED_FACE('',(#1290),#492,.F.);
#10912=ADVANCED_FACE('',(#1291,#146,#147,#148,#149,#150),#493,.T.);
#10913=ADVANCED_FACE('',(#1292),#10547,.T.);
#10914=ADVANCED_FACE('',(#1293),#10548,.T.);
#10915=ADVANCED_FACE('',(#1294),#10549,.T.);
#10916=ADVANCED_FACE('',(#1295),#494,.F.);
#10917=ADVANCED_FACE('',(#1296),#10550,.T.);
#10918=ADVANCED_FACE('',(#1297),#495,.F.);
#10919=ADVANCED_FACE('',(#1298),#10551,.T.);
#10920=ADVANCED_FACE('',(#1299),#496,.F.);
#10921=ADVANCED_FACE('',(#1300),#10552,.T.);
#10922=ADVANCED_FACE('',(#1301),#497,.F.);
#10923=ADVANCED_FACE('',(#1302),#10553,.T.);
#10924=ADVANCED_FACE('',(#1303),#498,.F.);
#10925=ADVANCED_FACE('',(#1304),#499,.F.);
#10926=ADVANCED_FACE('',(#1305),#500,.F.);
#10927=ADVANCED_FACE('',(#1306),#501,.F.);
#10928=ADVANCED_FACE('',(#1307),#502,.F.);
#10929=ADVANCED_FACE('',(#1308),#10554,.T.);
#10930=ADVANCED_FACE('',(#1309),#503,.F.);
#10931=ADVANCED_FACE('',(#1310),#504,.F.);
#10932=ADVANCED_FACE('',(#1311,#151),#505,.T.);
#10933=ADVANCED_FACE('',(#1312,#152),#506,.T.);
#10934=ADVANCED_FACE('',(#1313),#10555,.F.);
#10935=ADVANCED_FACE('',(#1314),#10556,.F.);
#10936=ADVANCED_FACE('',(#1315),#10557,.F.);
#10937=ADVANCED_FACE('',(#1316),#10558,.F.);
#10938=ADVANCED_FACE('',(#1317),#10559,.F.);
#10939=ADVANCED_FACE('',(#1318,#153),#507,.F.);
#10940=ADVANCED_FACE('',(#1319,#154,#155,#156,#157,#158),#508,.F.);
#10941=ADVANCED_FACE('',(#1320),#509,.F.);
#10942=ADVANCED_FACE('',(#1321),#510,.F.);
#10943=ADVANCED_FACE('',(#1322),#511,.F.);
#10944=ADVANCED_FACE('',(#1323),#512,.T.);
#10945=ADVANCED_FACE('',(#1324),#513,.T.);
#10946=ADVANCED_FACE('',(#1325),#514,.F.);
#10947=ADVANCED_FACE('',(#1326),#515,.T.);
#10948=ADVANCED_FACE('',(#1327),#516,.F.);
#10949=ADVANCED_FACE('',(#1328),#517,.T.);
#10950=ADVANCED_FACE('',(#1329),#518,.T.);
#10951=ADVANCED_FACE('',(#1330),#519,.T.);
#10952=ADVANCED_FACE('',(#1331),#520,.T.);
#11262=CLOSED_SHELL('',(#10648,#10649,#10650,#10651,#10652,#10653,#10654,
#10655,#10656,#10657,#10658,#10659,#10660,#10661,#10662,#10663,#10664,#10665,
#10666,#10667));
#11263=CLOSED_SHELL('',(#10668,#10669,#10670,#10671,#10672,#10673,#10674,
#10675,#10676,#10677,#10678,#10679,#10680,#10681,#10682,#10683,#10684,#10685,
#10686,#10687));
#11264=CLOSED_SHELL('',(#10688,#10689,#10690,#10691,#10692,#10693,#10694,
#10695,#10696,#10697,#10698,#10699,#10700,#10701,#10702,#10703,#10704,#10705,
#10706,#10707));
#11265=CLOSED_SHELL('',(#10708,#10709,#10710,#10711,#10712,#10713,#10714,
#10715,#10716,#10717,#10718,#10719,#10720,#10721,#10722,#10723,#10724,#10725,
#10726,#10727));
#11266=CLOSED_SHELL('',(#10728,#10729,#10730,#10731,#10732,#10733,#10734,
#10735,#10736,#10737,#10738,#10739,#10740,#10741,#10742,#10743,#10744,#10745,
#10746,#10747,#10748,#10749,#10750,#10751,#10752,#10753,#10754,#10755,#10756,
#10757,#10758,#10759,#10760,#10761,#10762,#10763,#10764,#10765,#10766,#10767,
#10768,#10769,#10770,#10771,#10772,#10773,#10774,#10775,#10776,#10777,#10778,
#10779,#10780,#10781,#10782,#10783,#10784,#10785,#10786,#10787,#10788,#10789,
#10790,#10791,#10792,#10793,#10794,#10795,#10796,#10797,#10798,#10799,#10800,
#10801,#10802,#10803,#10804,#10805,#10806,#10807,#10808,#10809,#10810,#10811,
#10812,#10813,#10814,#10815,#10816,#10817,#10818,#10819,#10820,#10821,#10822,
#10823,#10824,#10825,#10826,#10827,#10828,#10829,#10830,#10831,#10832,#10833,
#10834,#10835,#10836,#10837,#10838,#10839,#10840,#10841,#10842,#10843,#10844,
#10845,#10846,#10847,#10848,#10849,#10850,#10851,#10852,#10853,#10854,#10855,
#10856,#10857,#10858,#10859,#10860,#10861,#10862,#10863,#10864,#10865,#10866,
#10867,#10868,#10869,#10870,#10871,#10872,#10873,#10874,#10875,#10876,#10877,
#10878,#10879,#10880,#10881,#10882));
#11267=CLOSED_SHELL('',(#10883,#10884,#10885,#10886,#10887,#10888,#10889,
#10890));
#11268=CLOSED_SHELL('',(#10891,#10892,#10893,#10894,#10895,#10896,#10897,
#10898,#10899,#10900,#10901,#10902,#10903,#10904,#10905,#10906,#10907,#10908,
#10909,#10910,#10911,#10912,#10913,#10914,#10915,#10916,#10917,#10918,#10919,
#10920,#10921,#10922,#10923,#10924,#10925,#10926,#10927,#10928,#10929,#10930,
#10931,#10932,#10933));
#11269=CLOSED_SHELL('',(#10934,#10935,#10936,#10937,#10938,#10939,#10940,
#10941,#10942,#10943,#10944,#10945,#10946,#10947,#10948,#10949,#10950,#10951,
#10952));
#11439=AXIS2_PLACEMENT_3D('',#15382,#12439,#12440);
#11440=AXIS2_PLACEMENT_3D('',#15383,#12441,#12442);
#11441=AXIS2_PLACEMENT_3D('',#15385,#12443,#12444);
#11442=AXIS2_PLACEMENT_3D('',#15389,#12446,#12447);
#11443=AXIS2_PLACEMENT_3D('',#15390,#12448,#12449);
#11444=AXIS2_PLACEMENT_3D('',#15391,#12450,#12451);
#11445=AXIS2_PLACEMENT_3D('',#15398,#12452,#12453);
#11446=AXIS2_PLACEMENT_3D('',#15405,#12454,#12455);
#11447=AXIS2_PLACEMENT_3D('',#15407,#12456,#12457);
#11448=AXIS2_PLACEMENT_3D('',#15409,#12458,#12459);
#11449=AXIS2_PLACEMENT_3D('',#15418,#12460,#12461);
#11450=AXIS2_PLACEMENT_3D('',#15420,#12462,#12463);
#11451=AXIS2_PLACEMENT_3D('',#15422,#12464,#12465);
#11452=AXIS2_PLACEMENT_3D('',#15431,#12466,#12467);
#11453=AXIS2_PLACEMENT_3D('',#15433,#12468,#12469);
#11454=AXIS2_PLACEMENT_3D('',#15435,#12470,#12471);
#11455=AXIS2_PLACEMENT_3D('',#15444,#12472,#12473);
#11456=AXIS2_PLACEMENT_3D('',#15446,#12474,#12475);
#11457=AXIS2_PLACEMENT_3D('',#15447,#12476,#12477);
#11458=AXIS2_PLACEMENT_3D('',#15448,#12478,#12479);
#11459=AXIS2_PLACEMENT_3D('',#15452,#12482,#12483);
#11460=AXIS2_PLACEMENT_3D('',#15456,#12486,#12487);
#11461=AXIS2_PLACEMENT_3D('',#15460,#12490,#12491);
#11462=AXIS2_PLACEMENT_3D('',#15461,#12492,#12493);
#11463=AXIS2_PLACEMENT_3D('',#15465,#12496,#12497);
#11464=AXIS2_PLACEMENT_3D('',#15471,#12501,#12502);
#11465=AXIS2_PLACEMENT_3D('',#15477,#12506,#12507);
#11466=AXIS2_PLACEMENT_3D('',#15483,#12511,#12512);
#11467=AXIS2_PLACEMENT_3D('',#15485,#12514,#12515);
#11468=AXIS2_PLACEMENT_3D('',#15491,#12519,#12520);
#11469=AXIS2_PLACEMENT_3D('',#15493,#12522,#12523);
#11470=AXIS2_PLACEMENT_3D('',#15504,#12530,#12531);
#11471=AXIS2_PLACEMENT_3D('',#15507,#12534,#12535);
#11472=AXIS2_PLACEMENT_3D('',#15508,#12536,#12537);
#11473=AXIS2_PLACEMENT_3D('',#15509,#12538,#12539);
#11474=AXIS2_PLACEMENT_3D('',#15511,#12541,#12542);
#11475=AXIS2_PLACEMENT_3D('',#15513,#12544,#12545);
#11476=AXIS2_PLACEMENT_3D('',#15514,#12546,#12547);
#11477=AXIS2_PLACEMENT_3D('',#15516,#12548,#12549);
#11478=AXIS2_PLACEMENT_3D('',#15520,#12551,#12552);
#11479=AXIS2_PLACEMENT_3D('',#15521,#12553,#12554);
#11480=AXIS2_PLACEMENT_3D('',#15522,#12555,#12556);
#11481=AXIS2_PLACEMENT_3D('',#15529,#12557,#12558);
#11482=AXIS2_PLACEMENT_3D('',#15536,#12559,#12560);
#11483=AXIS2_PLACEMENT_3D('',#15538,#12561,#12562);
#11484=AXIS2_PLACEMENT_3D('',#15540,#12563,#12564);
#11485=AXIS2_PLACEMENT_3D('',#15549,#12565,#12566);
#11486=AXIS2_PLACEMENT_3D('',#15551,#12567,#12568);
#11487=AXIS2_PLACEMENT_3D('',#15553,#12569,#12570);
#11488=AXIS2_PLACEMENT_3D('',#15562,#12571,#12572);
#11489=AXIS2_PLACEMENT_3D('',#15564,#12573,#12574);
#11490=AXIS2_PLACEMENT_3D('',#15566,#12575,#12576);
#11491=AXIS2_PLACEMENT_3D('',#15575,#12577,#12578);
#11492=AXIS2_PLACEMENT_3D('',#15577,#12579,#12580);
#11493=AXIS2_PLACEMENT_3D('',#15578,#12581,#12582);
#11494=AXIS2_PLACEMENT_3D('',#15579,#12583,#12584);
#11495=AXIS2_PLACEMENT_3D('',#15583,#12587,#12588);
#11496=AXIS2_PLACEMENT_3D('',#15587,#12591,#12592);
#11497=AXIS2_PLACEMENT_3D('',#15591,#12595,#12596);
#11498=AXIS2_PLACEMENT_3D('',#15592,#12597,#12598);
#11499=AXIS2_PLACEMENT_3D('',#15596,#12601,#12602);
#11500=AXIS2_PLACEMENT_3D('',#15602,#12606,#12607);
#11501=AXIS2_PLACEMENT_3D('',#15608,#12611,#12612);
#11502=AXIS2_PLACEMENT_3D('',#15614,#12616,#12617);
#11503=AXIS2_PLACEMENT_3D('',#15616,#12619,#12620);
#11504=AXIS2_PLACEMENT_3D('',#15622,#12624,#12625);
#11505=AXIS2_PLACEMENT_3D('',#15624,#12627,#12628);
#11506=AXIS2_PLACEMENT_3D('',#15635,#12635,#12636);
#11507=AXIS2_PLACEMENT_3D('',#15638,#12639,#12640);
#11508=AXIS2_PLACEMENT_3D('',#15639,#12641,#12642);
#11509=AXIS2_PLACEMENT_3D('',#15640,#12643,#12644);
#11510=AXIS2_PLACEMENT_3D('',#15642,#12646,#12647);
#11511=AXIS2_PLACEMENT_3D('',#15644,#12649,#12650);
#11512=AXIS2_PLACEMENT_3D('',#15645,#12651,#12652);
#11513=AXIS2_PLACEMENT_3D('',#15647,#12653,#12654);
#11514=AXIS2_PLACEMENT_3D('',#15651,#12656,#12657);
#11515=AXIS2_PLACEMENT_3D('',#15652,#12658,#12659);
#11516=AXIS2_PLACEMENT_3D('',#15653,#12660,#12661);
#11517=AXIS2_PLACEMENT_3D('',#15660,#12662,#12663);
#11518=AXIS2_PLACEMENT_3D('',#15667,#12664,#12665);
#11519=AXIS2_PLACEMENT_3D('',#15669,#12666,#12667);
#11520=AXIS2_PLACEMENT_3D('',#15671,#12668,#12669);
#11521=AXIS2_PLACEMENT_3D('',#15680,#12670,#12671);
#11522=AXIS2_PLACEMENT_3D('',#15682,#12672,#12673);
#11523=AXIS2_PLACEMENT_3D('',#15684,#12674,#12675);
#11524=AXIS2_PLACEMENT_3D('',#15693,#12676,#12677);
#11525=AXIS2_PLACEMENT_3D('',#15695,#12678,#12679);
#11526=AXIS2_PLACEMENT_3D('',#15697,#12680,#12681);
#11527=AXIS2_PLACEMENT_3D('',#15706,#12682,#12683);
#11528=AXIS2_PLACEMENT_3D('',#15708,#12684,#12685);
#11529=AXIS2_PLACEMENT_3D('',#15709,#12686,#12687);
#11530=AXIS2_PLACEMENT_3D('',#15710,#12688,#12689);
#11531=AXIS2_PLACEMENT_3D('',#15714,#12692,#12693);
#11532=AXIS2_PLACEMENT_3D('',#15718,#12696,#12697);
#11533=AXIS2_PLACEMENT_3D('',#15722,#12700,#12701);
#11534=AXIS2_PLACEMENT_3D('',#15723,#12702,#12703);
#11535=AXIS2_PLACEMENT_3D('',#15727,#12706,#12707);
#11536=AXIS2_PLACEMENT_3D('',#15733,#12711,#12712);
#11537=AXIS2_PLACEMENT_3D('',#15739,#12716,#12717);
#11538=AXIS2_PLACEMENT_3D('',#15745,#12721,#12722);
#11539=AXIS2_PLACEMENT_3D('',#15747,#12724,#12725);
#11540=AXIS2_PLACEMENT_3D('',#15753,#12729,#12730);
#11541=AXIS2_PLACEMENT_3D('',#15755,#12732,#12733);
#11542=AXIS2_PLACEMENT_3D('',#15766,#12740,#12741);
#11543=AXIS2_PLACEMENT_3D('',#15769,#12744,#12745);
#11544=AXIS2_PLACEMENT_3D('',#15770,#12746,#12747);
#11545=AXIS2_PLACEMENT_3D('',#15771,#12748,#12749);
#11546=AXIS2_PLACEMENT_3D('',#15773,#12751,#12752);
#11547=AXIS2_PLACEMENT_3D('',#15775,#12754,#12755);
#11548=AXIS2_PLACEMENT_3D('',#15776,#12756,#12757);
#11549=AXIS2_PLACEMENT_3D('',#15778,#12758,#12759);
#11550=AXIS2_PLACEMENT_3D('',#15782,#12761,#12762);
#11551=AXIS2_PLACEMENT_3D('',#15783,#12763,#12764);
#11552=AXIS2_PLACEMENT_3D('',#15784,#12765,#12766);
#11553=AXIS2_PLACEMENT_3D('',#15791,#12767,#12768);
#11554=AXIS2_PLACEMENT_3D('',#15798,#12769,#12770);
#11555=AXIS2_PLACEMENT_3D('',#15800,#12771,#12772);
#11556=AXIS2_PLACEMENT_3D('',#15802,#12773,#12774);
#11557=AXIS2_PLACEMENT_3D('',#15811,#12775,#12776);
#11558=AXIS2_PLACEMENT_3D('',#15813,#12777,#12778);
#11559=AXIS2_PLACEMENT_3D('',#15815,#12779,#12780);
#11560=AXIS2_PLACEMENT_3D('',#15824,#12781,#12782);
#11561=AXIS2_PLACEMENT_3D('',#15826,#12783,#12784);
#11562=AXIS2_PLACEMENT_3D('',#15828,#12785,#12786);
#11563=AXIS2_PLACEMENT_3D('',#15837,#12787,#12788);
#11564=AXIS2_PLACEMENT_3D('',#15839,#12789,#12790);
#11565=AXIS2_PLACEMENT_3D('',#15840,#12791,#12792);
#11566=AXIS2_PLACEMENT_3D('',#15841,#12793,#12794);
#11567=AXIS2_PLACEMENT_3D('',#15845,#12797,#12798);
#11568=AXIS2_PLACEMENT_3D('',#15849,#12801,#12802);
#11569=AXIS2_PLACEMENT_3D('',#15853,#12805,#12806);
#11570=AXIS2_PLACEMENT_3D('',#15854,#12807,#12808);
#11571=AXIS2_PLACEMENT_3D('',#15858,#12811,#12812);
#11572=AXIS2_PLACEMENT_3D('',#15864,#12816,#12817);
#11573=AXIS2_PLACEMENT_3D('',#15870,#12821,#12822);
#11574=AXIS2_PLACEMENT_3D('',#15876,#12826,#12827);
#11575=AXIS2_PLACEMENT_3D('',#15878,#12829,#12830);
#11576=AXIS2_PLACEMENT_3D('',#15884,#12834,#12835);
#11577=AXIS2_PLACEMENT_3D('',#15886,#12837,#12838);
#11578=AXIS2_PLACEMENT_3D('',#15897,#12845,#12846);
#11579=AXIS2_PLACEMENT_3D('',#15900,#12849,#12850);
#11580=AXIS2_PLACEMENT_3D('',#15901,#12851,#12852);
#11581=AXIS2_PLACEMENT_3D('',#15902,#12853,#12854);
#11582=AXIS2_PLACEMENT_3D('',#15904,#12856,#12857);
#11583=AXIS2_PLACEMENT_3D('',#15906,#12859,#12860);
#11584=AXIS2_PLACEMENT_3D('',#15907,#12861,#12862);
#11585=AXIS2_PLACEMENT_3D('',#15937,#12864,#12865);
#11586=AXIS2_PLACEMENT_3D('',#15958,#12866,#12867);
#11587=AXIS2_PLACEMENT_3D('',#16036,#12869,#12870);
#11588=AXIS2_PLACEMENT_3D('',#16112,#12872,#12873);
#11589=AXIS2_PLACEMENT_3D('',#16188,#12875,#12876);
#11590=AXIS2_PLACEMENT_3D('',#16264,#12878,#12879);
#11591=AXIS2_PLACEMENT_3D('',#16340,#12881,#12882);
#11592=AXIS2_PLACEMENT_3D('',#16418,#12884,#12885);
#11593=AXIS2_PLACEMENT_3D('',#16496,#12887,#12888);
#11594=AXIS2_PLACEMENT_3D('',#16572,#12890,#12891);
#11595=AXIS2_PLACEMENT_3D('',#16648,#12893,#12894);
#11596=AXIS2_PLACEMENT_3D('',#16724,#12896,#12897);
#11597=AXIS2_PLACEMENT_3D('',#16800,#12899,#12900);
#11598=AXIS2_PLACEMENT_3D('',#16876,#12902,#12903);
#11599=AXIS2_PLACEMENT_3D('',#16954,#12905,#12906);
#11600=AXIS2_PLACEMENT_3D('',#17032,#12908,#12909);
#11601=AXIS2_PLACEMENT_3D('',#17108,#12911,#12912);
#11602=AXIS2_PLACEMENT_3D('',#17184,#12914,#12915);
#11603=AXIS2_PLACEMENT_3D('',#17260,#12917,#12918);
#11604=AXIS2_PLACEMENT_3D('',#17336,#12920,#12921);
#11605=AXIS2_PLACEMENT_3D('',#17358,#12923,#12924);
#11606=AXIS2_PLACEMENT_3D('',#17371,#12925,#12926);
#11607=AXIS2_PLACEMENT_3D('',#17449,#12928,#12929);
#11608=AXIS2_PLACEMENT_3D('',#17525,#12931,#12932);
#11609=AXIS2_PLACEMENT_3D('',#17601,#12934,#12935);
#11610=AXIS2_PLACEMENT_3D('',#17677,#12937,#12938);
#11611=AXIS2_PLACEMENT_3D('',#17753,#12940,#12941);
#11612=AXIS2_PLACEMENT_3D('',#17829,#12943,#12944);
#11613=AXIS2_PLACEMENT_3D('',#17909,#12946,#12947);
#11614=AXIS2_PLACEMENT_3D('',#17985,#12949,#12950);
#11615=AXIS2_PLACEMENT_3D('',#18061,#12952,#12953);
#11616=AXIS2_PLACEMENT_3D('',#18137,#12955,#12956);
#11617=AXIS2_PLACEMENT_3D('',#18213,#12958,#12959);
#11618=AXIS2_PLACEMENT_3D('',#18289,#12961,#12962);
#11619=AXIS2_PLACEMENT_3D('',#18367,#12964,#12965);
#11620=AXIS2_PLACEMENT_3D('',#18445,#12967,#12968);
#11621=AXIS2_PLACEMENT_3D('',#18521,#12970,#12971);
#11622=AXIS2_PLACEMENT_3D('',#18597,#12973,#12974);
#11623=AXIS2_PLACEMENT_3D('',#18673,#12976,#12977);
#11624=AXIS2_PLACEMENT_3D('',#18749,#12979,#12980);
#11625=AXIS2_PLACEMENT_3D('',#18762,#12982,#12983);
#11626=AXIS2_PLACEMENT_3D('',#18763,#12984,#12985);
#11627=AXIS2_PLACEMENT_3D('',#18841,#12987,#12988);
#11628=AXIS2_PLACEMENT_3D('',#18917,#12990,#12991);
#11629=AXIS2_PLACEMENT_3D('',#18993,#12993,#12994);
#11630=AXIS2_PLACEMENT_3D('',#19069,#12996,#12997);
#11631=AXIS2_PLACEMENT_3D('',#19145,#12999,#13000);
#11632=AXIS2_PLACEMENT_3D('',#19221,#13002,#13003);
#11633=AXIS2_PLACEMENT_3D('',#19299,#13005,#13006);
#11634=AXIS2_PLACEMENT_3D('',#19377,#13008,#13009);
#11635=AXIS2_PLACEMENT_3D('',#19453,#13011,#13012);
#11636=AXIS2_PLACEMENT_3D('',#19529,#13014,#13015);
#11637=AXIS2_PLACEMENT_3D('',#19605,#13017,#13018);
#11638=AXIS2_PLACEMENT_3D('',#19681,#13020,#13021);
#11639=AXIS2_PLACEMENT_3D('',#19759,#13023,#13024);
#11640=AXIS2_PLACEMENT_3D('',#19837,#13026,#13027);
#11641=AXIS2_PLACEMENT_3D('',#19913,#13029,#13030);
#11642=AXIS2_PLACEMENT_3D('',#19989,#13032,#13033);
#11643=AXIS2_PLACEMENT_3D('',#20065,#13035,#13036);
#11644=AXIS2_PLACEMENT_3D('',#20141,#13038,#13039);
#11645=AXIS2_PLACEMENT_3D('',#20181,#13041,#13042);
#11646=AXIS2_PLACEMENT_3D('',#20212,#13043,#13044);
#11647=AXIS2_PLACEMENT_3D('',#20288,#13046,#13047);
#11648=AXIS2_PLACEMENT_3D('',#20364,#13049,#13050);
#11649=AXIS2_PLACEMENT_3D('',#20440,#13052,#13053);
#11650=AXIS2_PLACEMENT_3D('',#20516,#13055,#13056);
#11651=AXIS2_PLACEMENT_3D('',#20592,#13058,#13059);
#11652=AXIS2_PLACEMENT_3D('',#20670,#13061,#13062);
#11653=AXIS2_PLACEMENT_3D('',#20748,#13064,#13065);
#11654=AXIS2_PLACEMENT_3D('',#20824,#13067,#13068);
#11655=AXIS2_PLACEMENT_3D('',#20900,#13070,#13071);
#11656=AXIS2_PLACEMENT_3D('',#20976,#13073,#13074);
#11657=AXIS2_PLACEMENT_3D('',#21052,#13076,#13077);
#11658=AXIS2_PLACEMENT_3D('',#21128,#13079,#13080);
#11659=AXIS2_PLACEMENT_3D('',#21208,#13082,#13083);
#11660=AXIS2_PLACEMENT_3D('',#21284,#13085,#13086);
#11661=AXIS2_PLACEMENT_3D('',#21360,#13088,#13089);
#11662=AXIS2_PLACEMENT_3D('',#21436,#13091,#13092);
#11663=AXIS2_PLACEMENT_3D('',#21512,#13094,#13095);
#11664=AXIS2_PLACEMENT_3D('',#21517,#13097,#13098);
#11665=AXIS2_PLACEMENT_3D('',#21532,#13099,#13100);
#11666=AXIS2_PLACEMENT_3D('',#21553,#13102,#13103);
#11667=AXIS2_PLACEMENT_3D('',#21592,#13104,#13105);
#11668=AXIS2_PLACEMENT_3D('',#21668,#13107,#13108);
#11669=AXIS2_PLACEMENT_3D('',#21744,#13110,#13111);
#11670=AXIS2_PLACEMENT_3D('',#21820,#13113,#13114);
#11671=AXIS2_PLACEMENT_3D('',#21898,#13116,#13117);
#11672=AXIS2_PLACEMENT_3D('',#21971,#13120,#13121);
#11673=AXIS2_PLACEMENT_3D('',#21976,#13123,#13124);
#11674=AXIS2_PLACEMENT_3D('',#21991,#13125,#13126);
#11675=AXIS2_PLACEMENT_3D('',#22012,#13128,#13129);
#11676=AXIS2_PLACEMENT_3D('',#22051,#13130,#13131);
#11677=AXIS2_PLACEMENT_3D('',#22127,#13133,#13134);
#11678=AXIS2_PLACEMENT_3D('',#22203,#13136,#13137);
#11679=AXIS2_PLACEMENT_3D('',#22279,#13139,#13140);
#11680=AXIS2_PLACEMENT_3D('',#22357,#13142,#13143);
#11681=AXIS2_PLACEMENT_3D('',#22430,#13146,#13147);
#11682=AXIS2_PLACEMENT_3D('',#22435,#13149,#13150);
#11683=AXIS2_PLACEMENT_3D('',#22450,#13151,#13152);
#11684=AXIS2_PLACEMENT_3D('',#22471,#13154,#13155);
#11685=AXIS2_PLACEMENT_3D('',#22510,#13156,#13157);
#11686=AXIS2_PLACEMENT_3D('',#22586,#13159,#13160);
#11687=AXIS2_PLACEMENT_3D('',#22662,#13162,#13163);
#11688=AXIS2_PLACEMENT_3D('',#22738,#13165,#13166);
#11689=AXIS2_PLACEMENT_3D('',#22816,#13168,#13169);
#11690=AXIS2_PLACEMENT_3D('',#22889,#13172,#13173);
#11691=AXIS2_PLACEMENT_3D('',#22894,#13175,#13176);
#11692=AXIS2_PLACEMENT_3D('',#22909,#13177,#13178);
#11693=AXIS2_PLACEMENT_3D('',#22930,#13180,#13181);
#11694=AXIS2_PLACEMENT_3D('',#22969,#13182,#13183);
#11695=AXIS2_PLACEMENT_3D('',#23045,#13185,#13186);
#11696=AXIS2_PLACEMENT_3D('',#23121,#13188,#13189);
#11697=AXIS2_PLACEMENT_3D('',#23197,#13191,#13192);
#11698=AXIS2_PLACEMENT_3D('',#23275,#13194,#13195);
#11699=AXIS2_PLACEMENT_3D('',#23348,#13198,#13199);
#11700=AXIS2_PLACEMENT_3D('',#23421,#13200,#13201);
#11701=AXIS2_PLACEMENT_3D('',#23494,#13202,#13203);
#11702=AXIS2_PLACEMENT_3D('',#23567,#13204,#13205);
#11703=AXIS2_PLACEMENT_3D('',#23640,#13206,#13207);
#11704=AXIS2_PLACEMENT_3D('',#23679,#13208,#13209);
#11705=AXIS2_PLACEMENT_3D('',#23712,#13210,#13211);
#11706=AXIS2_PLACEMENT_3D('',#23743,#13212,#13213);
#11707=AXIS2_PLACEMENT_3D('',#23768,#13214,#13215);
#11708=AXIS2_PLACEMENT_3D('',#23791,#13216,#13217);
#11709=AXIS2_PLACEMENT_3D('',#23808,#13218,#13219);
#11710=AXIS2_PLACEMENT_3D('',#23823,#13220,#13221);
#11711=AXIS2_PLACEMENT_3D('',#23832,#13222,#13223);
#11712=AXIS2_PLACEMENT_3D('',#23834,#13224,#13225);
#11713=AXIS2_PLACEMENT_3D('',#23837,#13227,#13228);
#11714=AXIS2_PLACEMENT_3D('',#23838,#13229,#13230);
#11715=AXIS2_PLACEMENT_3D('',#23840,#13231,#13232);
#11716=AXIS2_PLACEMENT_3D('',#23843,#13234,#13235);
#11717=AXIS2_PLACEMENT_3D('',#23844,#13236,#13237);
#11718=AXIS2_PLACEMENT_3D('',#23846,#13238,#13239);
#11719=AXIS2_PLACEMENT_3D('',#23849,#13241,#13242);
#11720=AXIS2_PLACEMENT_3D('',#23850,#13243,#13244);
#11721=AXIS2_PLACEMENT_3D('',#23853,#13246,#13247);
#11722=AXIS2_PLACEMENT_3D('',#23854,#13248,#13249);
#11723=AXIS2_PLACEMENT_3D('',#23898,#13250,#13251);
#11724=AXIS2_PLACEMENT_3D('',#23915,#13253,#13254);
#11725=AXIS2_PLACEMENT_3D('',#23916,#13255,#13256);
#11726=AXIS2_PLACEMENT_3D('',#23960,#13257,#13258);
#11727=AXIS2_PLACEMENT_3D('',#23977,#13260,#13261);
#11728=AXIS2_PLACEMENT_3D('',#23978,#13262,#13263);
#11729=AXIS2_PLACEMENT_3D('',#24022,#13264,#13265);
#11730=AXIS2_PLACEMENT_3D('',#24039,#13267,#13268);
#11731=AXIS2_PLACEMENT_3D('',#24040,#13269,#13270);
#11732=AXIS2_PLACEMENT_3D('',#24084,#13271,#13272);
#11733=AXIS2_PLACEMENT_3D('',#24101,#13274,#13275);
#11734=AXIS2_PLACEMENT_3D('',#24740,#13276,#13277);
#11735=AXIS2_PLACEMENT_3D('',#25682,#13279,#13280);
#11736=AXIS2_PLACEMENT_3D('',#25986,#13282,#13283);
#11737=AXIS2_PLACEMENT_3D('',#26630,#13285,#13286);
#11738=AXIS2_PLACEMENT_3D('',#26647,#13295,#13296);
#11739=AXIS2_PLACEMENT_3D('',#26648,#13297,#13298);
#11740=AXIS2_PLACEMENT_3D('',#26649,#13299,#13300);
#11741=AXIS2_PLACEMENT_3D('',#26650,#13301,#13302);
#11742=AXIS2_PLACEMENT_3D('',#26651,#13303,#13304);
#11743=AXIS2_PLACEMENT_3D('',#26652,#13305,#13306);
#11744=AXIS2_PLACEMENT_3D('',#28535,#13309,#13310);
#11745=AXIS2_PLACEMENT_3D('',#31061,#13314,#13315);
#11746=AXIS2_PLACEMENT_3D('',#33587,#13319,#13320);
#11747=AXIS2_PLACEMENT_3D('',#34231,#13322,#13323);
#11748=AXIS2_PLACEMENT_3D('',#34232,#13324,#13325);
#11749=AXIS2_PLACEMENT_3D('',#34233,#13326,#13327);
#11750=AXIS2_PLACEMENT_3D('',#34239,#13331,#13332);
#11751=AXIS2_PLACEMENT_3D('',#34243,#13335,#13336);
#11752=AXIS2_PLACEMENT_3D('',#34245,#13337,#13338);
#11753=AXIS2_PLACEMENT_3D('',#34248,#13340,#13341);
#11754=AXIS2_PLACEMENT_3D('',#34249,#13342,#13343);
#11755=AXIS2_PLACEMENT_3D('',#34253,#13346,#13347);
#11756=AXIS2_PLACEMENT_3D('',#34257,#13350,#13351);
#11757=AXIS2_PLACEMENT_3D('',#34259,#13352,#13353);
#11758=AXIS2_PLACEMENT_3D('',#34261,#13355,#13356);
#11759=AXIS2_PLACEMENT_3D('',#34265,#13359,#13360);
#11760=AXIS2_PLACEMENT_3D('',#34267,#13361,#13362);
#11761=AXIS2_PLACEMENT_3D('',#34269,#13364,#13365);
#11762=AXIS2_PLACEMENT_3D('',#34273,#13368,#13369);
#11763=AXIS2_PLACEMENT_3D('',#34275,#13370,#13371);
#11764=AXIS2_PLACEMENT_3D('',#34277,#13373,#13374);
#11765=AXIS2_PLACEMENT_3D('',#34281,#13377,#13378);
#11766=AXIS2_PLACEMENT_3D('',#34283,#13379,#13380);
#11767=AXIS2_PLACEMENT_3D('',#34285,#13382,#13383);
#11768=AXIS2_PLACEMENT_3D('',#34287,#13385,#13386);
#11769=AXIS2_PLACEMENT_3D('',#34289,#13387,#13388);
#11770=AXIS2_PLACEMENT_3D('',#34291,#13390,#13391);
#11771=AXIS2_PLACEMENT_3D('',#34293,#13392,#13393);
#11772=AXIS2_PLACEMENT_3D('',#34295,#13395,#13396);
#11773=AXIS2_PLACEMENT_3D('',#34297,#13398,#13399);
#11774=AXIS2_PLACEMENT_3D('',#34298,#13400,#13401);
#11775=AXIS2_PLACEMENT_3D('',#34303,#13403,#13404);
#11776=AXIS2_PLACEMENT_3D('',#34308,#13405,#13406);
#11777=AXIS2_PLACEMENT_3D('',#34309,#13407,#13408);
#11778=AXIS2_PLACEMENT_3D('',#34310,#13409,#13410);
#11779=AXIS2_PLACEMENT_3D('',#34315,#13411,#13412);
#11780=AXIS2_PLACEMENT_3D('',#34316,#13413,#13414);
#11781=AXIS2_PLACEMENT_3D('',#34320,#13416,#13417);
#11782=AXIS2_PLACEMENT_3D('',#34321,#13418,#13419);
#11783=AXIS2_PLACEMENT_3D('',#34323,#13420,#13421);
#11784=AXIS2_PLACEMENT_3D('',#34328,#13424,#13425);
#11785=AXIS2_PLACEMENT_3D('',#34330,#13427,#13428);
#11786=AXIS2_PLACEMENT_3D('',#34331,#13429,#13430);
#11787=AXIS2_PLACEMENT_3D('',#34332,#13431,#13432);
#11788=AXIS2_PLACEMENT_3D('',#34334,#13434,#13435);
#11789=AXIS2_PLACEMENT_3D('',#34335,#13436,#13437);
#11790=AXIS2_PLACEMENT_3D('',#34337,#13438,#13439);
#11791=AXIS2_PLACEMENT_3D('',#34340,#13441,#13442);
#11792=AXIS2_PLACEMENT_3D('',#34341,#13443,#13444);
#11793=AXIS2_PLACEMENT_3D('',#34343,#13445,#13446);
#11794=AXIS2_PLACEMENT_3D('',#34346,#13448,#13449);
#11795=AXIS2_PLACEMENT_3D('',#34347,#13450,#13451);
#11796=AXIS2_PLACEMENT_3D('',#34349,#13452,#13453);
#11797=AXIS2_PLACEMENT_3D('',#34352,#13455,#13456);
#11798=AXIS2_PLACEMENT_3D('',#34353,#13457,#13458);
#11799=AXIS2_PLACEMENT_3D('',#34355,#13459,#13460);
#11800=AXIS2_PLACEMENT_3D('',#34358,#13462,#13463);
#11801=AXIS2_PLACEMENT_3D('',#34359,#13464,#13465);
#11802=AXIS2_PLACEMENT_3D('',#34361,#13466,#13467);
#11803=AXIS2_PLACEMENT_3D('',#34364,#13469,#13470);
#11804=AXIS2_PLACEMENT_3D('',#34365,#13471,#13472);
#11805=AXIS2_PLACEMENT_3D('',#34367,#13473,#13474);
#11806=AXIS2_PLACEMENT_3D('',#34369,#13476,#13477);
#11807=AXIS2_PLACEMENT_3D('',#34371,#13478,#13479);
#11808=AXIS2_PLACEMENT_3D('',#34373,#13481,#13482);
#11809=AXIS2_PLACEMENT_3D('',#34375,#13483,#13484);
#11810=AXIS2_PLACEMENT_3D('',#34377,#13486,#13487);
#11811=AXIS2_PLACEMENT_3D('',#34379,#13488,#13489);
#11812=AXIS2_PLACEMENT_3D('',#34381,#13491,#13492);
#11813=AXIS2_PLACEMENT_3D('',#34383,#13493,#13494);
#11814=AXIS2_PLACEMENT_3D('',#34386,#13496,#13497);
#11815=AXIS2_PLACEMENT_3D('',#34387,#13498,#13499);
#11816=AXIS2_PLACEMENT_3D('',#34388,#13500,#13501);
#11817=AXIS2_PLACEMENT_3D('',#34389,#13502,#13503);
#11818=AXIS2_PLACEMENT_3D('',#34390,#13504,#13505);
#11819=AXIS2_PLACEMENT_3D('',#34391,#13506,#13507);
#11820=AXIS2_PLACEMENT_3D('',#34400,#13512,#13513);
#11821=AXIS2_PLACEMENT_3D('',#34406,#13517,#13518);
#11822=AXIS2_PLACEMENT_3D('',#34410,#13521,#13522);
#11823=AXIS2_PLACEMENT_3D('',#34414,#13525,#13526);
#11824=AXIS2_PLACEMENT_3D('',#34416,#13528,#13529);
#11825=AXIS2_PLACEMENT_3D('',#34425,#13534,#13535);
#11826=AXIS2_PLACEMENT_3D('',#34431,#13539,#13540);
#11827=AXIS2_PLACEMENT_3D('',#34448,#13549,#13550);
#11828=AXIS2_PLACEMENT_3D('',#34450,#13551,#13552);
#11829=AXIS2_PLACEMENT_3D('',#34452,#13553,#13554);
#11830=AXIS2_PLACEMENT_3D('',#34454,#13556,#13557);
#11831=AXIS2_PLACEMENT_3D('',#34456,#13558,#13559);
#11832=AXIS2_PLACEMENT_3D('',#34458,#13561,#13562);
#11833=AXIS2_PLACEMENT_3D('',#34460,#13563,#13564);
#11834=AXIS2_PLACEMENT_3D('',#34462,#13566,#13567);
#11835=AXIS2_PLACEMENT_3D('',#34468,#13571,#13572);
#11836=AXIS2_PLACEMENT_3D('',#34470,#13573,#13574);
#11837=AXIS2_PLACEMENT_3D('',#34472,#13576,#13577);
#11838=AXIS2_PLACEMENT_3D('',#34476,#13580,#13581);
#11839=AXIS2_PLACEMENT_3D('',#34478,#13582,#13583);
#11840=AXIS2_PLACEMENT_3D('',#34480,#13585,#13586);
#11841=AXIS2_PLACEMENT_3D('',#34484,#13589,#13590);
#11842=AXIS2_PLACEMENT_3D('',#34486,#13591,#13592);
#11843=AXIS2_PLACEMENT_3D('',#34488,#13594,#13595);
#11844=AXIS2_PLACEMENT_3D('',#34492,#13598,#13599);
#11845=AXIS2_PLACEMENT_3D('',#34494,#13600,#13601);
#11846=AXIS2_PLACEMENT_3D('',#34496,#13603,#13604);
#11847=AXIS2_PLACEMENT_3D('',#34500,#13607,#13608);
#11848=AXIS2_PLACEMENT_3D('',#34504,#13611,#13612);
#11849=AXIS2_PLACEMENT_3D('',#34506,#13613,#13614);
#11850=AXIS2_PLACEMENT_3D('',#34510,#13617,#13618);
#11851=AXIS2_PLACEMENT_3D('',#34514,#13621,#13622);
#11852=AXIS2_PLACEMENT_3D('',#34517,#13624,#13625);
#11853=AXIS2_PLACEMENT_3D('',#34518,#13626,#13627);
#11854=AXIS2_PLACEMENT_3D('',#34521,#13630,#13631);
#11855=AXIS2_PLACEMENT_3D('',#34525,#13634,#13635);
#11856=AXIS2_PLACEMENT_3D('',#34527,#13637,#13638);
#11857=AXIS2_PLACEMENT_3D('',#34528,#13639,#13640);
#11858=AXIS2_PLACEMENT_3D('',#34529,#13641,#13642);
#11859=AXIS2_PLACEMENT_3D('',#34531,#13643,#13644);
#11860=AXIS2_PLACEMENT_3D('',#34534,#13646,#13647);
#11861=AXIS2_PLACEMENT_3D('',#34535,#13648,#13649);
#11862=AXIS2_PLACEMENT_3D('',#34537,#13650,#13651);
#11863=AXIS2_PLACEMENT_3D('',#34540,#13653,#13654);
#11864=AXIS2_PLACEMENT_3D('',#34541,#13655,#13656);
#11865=AXIS2_PLACEMENT_3D('',#34543,#13657,#13658);
#11866=AXIS2_PLACEMENT_3D('',#34546,#13660,#13661);
#11867=AXIS2_PLACEMENT_3D('',#34547,#13662,#13663);
#11868=AXIS2_PLACEMENT_3D('',#34549,#13664,#13665);
#11869=AXIS2_PLACEMENT_3D('',#34552,#13667,#13668);
#11870=AXIS2_PLACEMENT_3D('',#34553,#13669,#13670);
#11871=AXIS2_PLACEMENT_3D('',#34555,#13671,#13672);
#11872=AXIS2_PLACEMENT_3D('',#34558,#13674,#13675);
#11873=AXIS2_PLACEMENT_3D('',#34559,#13676,#13677);
#11874=AXIS2_PLACEMENT_3D('',#34576,#13686,#13687);
#11875=AXIS2_PLACEMENT_3D('',#34593,#13696,#13697);
#11876=AXIS2_PLACEMENT_3D('',#34596,#13700,#13701);
#11877=AXIS2_PLACEMENT_3D('',#34598,#13703,#13704);
#11878=AXIS2_PLACEMENT_3D('',#34600,#13706,#13707);
#11879=AXIS2_PLACEMENT_3D('',#34603,#13710,#13711);
#11880=AXIS2_PLACEMENT_3D('',#34606,#13714,#13715);
#11881=AXIS2_PLACEMENT_3D('',#34607,#13716,#13717);
#11882=AXIS2_PLACEMENT_3D('',#34608,#13718,#13719);
#11883=AXIS2_PLACEMENT_3D('',#34609,#13720,#13721);
#11884=AXIS2_PLACEMENT_3D('',#34610,#13722,#13723);
#11885=AXIS2_PLACEMENT_3D('',#34611,#13724,#13725);
#11886=AXIS2_PLACEMENT_3D('',#34612,#13726,#13727);
#12439=DIRECTION('axis',(0.,0.,1.));
#12440=DIRECTION('refdir',(1.,0.,0.));
#12441=DIRECTION('center_axis',(0.,0.,1.));
#12442=DIRECTION('ref_axis',(1.,0.,0.));
#12443=DIRECTION('center_axis',(0.,0.,-1.));
#12444=DIRECTION('ref_axis',(-1.,0.,0.));
#12445=DIRECTION('',(0.,0.,-1.));
#12446=DIRECTION('center_axis',(0.,0.,1.));
#12447=DIRECTION('ref_axis',(-1.,0.,0.));
#12448=DIRECTION('center_axis',(0.,0.,1.));
#12449=DIRECTION('ref_axis',(-1.,0.,0.));
#12450=DIRECTION('center_axis',(0.,0.,-1.));
#12451=DIRECTION('ref_axis',(-1.,0.,0.));
#12452=DIRECTION('center_axis',(0.,-1.,0.));
#12453=DIRECTION('ref_axis',(1.,0.,0.));
#12454=DIRECTION('center_axis',(0.,1.,0.));
#12455=DIRECTION('ref_axis',(-0.662700408463881,0.,0.748884616360762));
#12456=DIRECTION('center_axis',(0.,0.,-1.));
#12457=DIRECTION('ref_axis',(-1.,0.,0.));
#12458=DIRECTION('center_axis',(-1.,-1.23033231110227E-14,1.91813075638571E-13));
#12459=DIRECTION('ref_axis',(-1.51799278823133E-13,0.662700408404006,-0.748884616413746));
#12460=DIRECTION('center_axis',(-1.,-6.87436171423541E-14,6.46003611483159E-13));
#12461=DIRECTION('ref_axis',(-5.29338589993441E-13,0.662700408303445,-0.748884616502734));
#12462=DIRECTION('center_axis',(0.,0.,-1.));
#12463=DIRECTION('ref_axis',(-1.,0.,0.));
#12464=DIRECTION('center_axis',(-2.42515865283882E-14,1.,-2.2795089778668E-13));
#12465=DIRECTION('ref_axis',(0.628654464794611,1.92519804155958E-13,0.777684745828154));
#12466=DIRECTION('center_axis',(2.42515865283884E-14,1.,2.27950897786681E-13));
#12467=DIRECTION('ref_axis',(0.628654464776,-1.92519804158937E-13,0.777684745843199));
#12468=DIRECTION('center_axis',(0.,0.,-1.));
#12469=DIRECTION('ref_axis',(-1.,0.,0.));
#12470=DIRECTION('center_axis',(-1.,-4.42963920865616E-14,-3.40131136130303E-13));
#12471=DIRECTION('ref_axis',(2.92361920824713E-13,-0.628654464727554,-0.777684745882361));
#12472=DIRECTION('center_axis',(-1.,-8.06737718791901E-14,-6.82057482811295E-13));
#12473=DIRECTION('ref_axis',(5.81141627215589E-13,-0.628654464429985,-0.777684746122906));
#12474=DIRECTION('center_axis',(0.,0.,-1.));
#12475=DIRECTION('ref_axis',(-1.,0.,0.));
#12476=DIRECTION('center_axis',(-4.02653252918805E-14,1.,3.02189686082951E-13));
#12477=DIRECTION('ref_axis',(-0.662700408561431,-2.52989054626112E-13,0.748884616274438));
#12478=DIRECTION('center_axis',(0.,0.,-1.));
#12479=DIRECTION('ref_axis',(-1.,0.,0.));
#12480=DIRECTION('',(0.,-1.,0.));
#12481=DIRECTION('',(-1.,0.,0.));
#12482=DIRECTION('center_axis',(0.,0.,-1.));
#12483=DIRECTION('ref_axis',(-1.,0.,0.));
#12484=DIRECTION('',(-1.,0.,0.));
#12485=DIRECTION('',(0.,-1.,0.));
#12486=DIRECTION('center_axis',(0.,0.,-1.));
#12487=DIRECTION('ref_axis',(-1.,0.,0.));
#12488=DIRECTION('',(0.,-1.,0.));
#12489=DIRECTION('',(-1.,0.,0.));
#12490=DIRECTION('center_axis',(0.,0.,-1.));
#12491=DIRECTION('ref_axis',(-1.,0.,0.));
#12492=DIRECTION('center_axis',(0.,0.,-1.));
#12493=DIRECTION('ref_axis',(-1.,0.,0.));
#12494=DIRECTION('',(0.,-1.,0.));
#12495=DIRECTION('',(-1.,0.,0.));
#12496=DIRECTION('center_axis',(1.,0.,0.));
#12497=DIRECTION('ref_axis',(0.,0.,-1.));
#12498=DIRECTION('',(0.,0.,-1.));
#12499=DIRECTION('',(0.,-1.,0.));
#12500=DIRECTION('',(0.,0.,-1.));
#12501=DIRECTION('center_axis',(1.,0.,0.));
#12502=DIRECTION('ref_axis',(0.,0.,-1.));
#12503=DIRECTION('',(0.,0.,-1.));
#12504=DIRECTION('',(0.,-1.,0.));
#12505=DIRECTION('',(0.,0.,-1.));
#12506=DIRECTION('center_axis',(1.,0.,0.));
#12507=DIRECTION('ref_axis',(0.,0.,-1.));
#12508=DIRECTION('',(0.,0.,-1.));
#12509=DIRECTION('',(0.,-1.,0.));
#12510=DIRECTION('',(0.,0.,-1.));
#12511=DIRECTION('center_axis',(0.,-1.,0.));
#12512=DIRECTION('ref_axis',(0.,0.,-1.));
#12513=DIRECTION('',(-1.,0.,0.));
#12514=DIRECTION('center_axis',(1.,0.,0.));
#12515=DIRECTION('ref_axis',(0.,0.,-1.));
#12516=DIRECTION('',(0.,0.,-1.));
#12517=DIRECTION('',(0.,-1.,0.));
#12518=DIRECTION('',(0.,0.,-1.));
#12519=DIRECTION('center_axis',(0.,1.,0.));
#12520=DIRECTION('ref_axis',(0.,0.,1.));
#12521=DIRECTION('',(1.,0.,0.));
#12522=DIRECTION('center_axis',(0.,0.,-1.));
#12523=DIRECTION('ref_axis',(-1.,0.,0.));
#12524=DIRECTION('',(-1.,0.,0.));
#12525=DIRECTION('',(0.,-1.,0.));
#12526=DIRECTION('',(-1.,0.,0.));
#12527=DIRECTION('',(-1.,0.,0.));
#12528=DIRECTION('',(0.,1.,0.));
#12529=DIRECTION('',(-1.,0.,0.));
#12530=DIRECTION('center_axis',(1.,0.,0.));
#12531=DIRECTION('ref_axis',(0.,0.,-1.));
#12532=DIRECTION('',(0.,0.,-1.));
#12533=DIRECTION('',(0.,0.,-1.));
#12534=DIRECTION('center_axis',(0.,-1.,0.));
#12535=DIRECTION('ref_axis',(0.,0.,-1.));
#12536=DIRECTION('center_axis',(0.,-1.,0.));
#12537=DIRECTION('ref_axis',(0.,0.,-1.));
#12538=DIRECTION('center_axis',(0.,-1.,0.));
#12539=DIRECTION('ref_axis',(0.,0.,-1.));
#12540=DIRECTION('',(0.,0.,-1.));
#12541=DIRECTION('center_axis',(-1.,0.,0.));
#12542=DIRECTION('ref_axis',(0.,0.,1.));
#12543=DIRECTION('',(0.,0.,-1.));
#12544=DIRECTION('center_axis',(0.,-1.,0.));
#12545=DIRECTION('ref_axis',(0.,0.,-1.));
#12546=DIRECTION('center_axis',(4.16203559120935E-32,4.16203559120936E-32,
1.));
#12547=DIRECTION('ref_axis',(-3.27821759239711E-15,1.,-4.16203559120935E-32));
#12548=DIRECTION('center_axis',(-4.16203559120935E-32,-4.16203559120936E-32,
-1.));
#12549=DIRECTION('ref_axis',(3.27821759239712E-15,-1.,4.16203559120935E-32));
#12550=DIRECTION('',(-4.16203559120935E-32,-4.16203559120936E-32,-1.));
#12551=DIRECTION('center_axis',(4.16203559120935E-32,4.16203559120936E-32,
1.));
#12552=DIRECTION('ref_axis',(3.27821759239712E-15,-1.,4.16203559120935E-32));
#12553=DIRECTION('center_axis',(4.16203559120935E-32,4.16203559120936E-32,
1.));
#12554=DIRECTION('ref_axis',(3.27821759239712E-15,-1.,4.16203559120935E-32));
#12555=DIRECTION('center_axis',(-4.16203559120935E-32,-4.16203559120936E-32,
-1.));
#12556=DIRECTION('ref_axis',(3.35689481461465E-15,-1.,0.));
#12557=DIRECTION('center_axis',(1.,3.49676543189026E-15,-4.16203559120936E-32));
#12558=DIRECTION('ref_axis',(-3.49676543189026E-15,1.,0.));
#12559=DIRECTION('center_axis',(-1.,-2.79620021808786E-14,1.10376610444469E-13));
#12560=DIRECTION('ref_axis',(-1.01189775835862E-13,0.6627004084464,-0.748884616376231));
#12561=DIRECTION('center_axis',(-4.16203559120935E-32,-4.16203559120936E-32,
-1.));
#12562=DIRECTION('ref_axis',(3.64246399155235E-15,-1.,4.16203559120935E-32));
#12563=DIRECTION('center_axis',(5.22244552899185E-14,-1.,3.38377885085167E-13));
#12564=DIRECTION('ref_axis',(-0.662700408929437,-2.88015160394313E-13,-0.748884615948783));
#12565=DIRECTION('center_axis',(9.67056193232502E-14,-1.,7.56380221927762E-13));
#12566=DIRECTION('ref_axis',(-0.662700408393056,-6.30528365788067E-13,-0.748884616423436));
#12567=DIRECTION('center_axis',(-4.16203559120935E-32,-4.16203559120936E-32,
-1.));
#12568=DIRECTION('ref_axis',(3.64246399155235E-15,-1.,4.16203559120935E-32));
#12569=DIRECTION('center_axis',(-1.,-3.21705988223668E-14,-2.26155687236952E-13));
#12570=DIRECTION('ref_axis',(1.96102018725182E-13,-0.62865446483494,-0.777684745795554));
#12571=DIRECTION('center_axis',(-1.,1.63325742344061E-14,2.29746108336374E-13));
#12572=DIRECTION('ref_axis',(-1.88937589565396E-13,-0.628654464884546,-0.777684745755454));
#12573=DIRECTION('center_axis',(-4.16203559120935E-32,-4.16203559120936E-32,
-1.));
#12574=DIRECTION('ref_axis',(3.64246399155235E-15,-1.,4.16203559120935E-32));
#12575=DIRECTION('center_axis',(4.81734732924783E-14,-1.,-3.00344109282818E-13));
#12576=DIRECTION('ref_axis',(0.628654464809676,2.6385750135564E-13,-0.777684745815976));
#12577=DIRECTION('center_axis',(7.6631840791126E-14,-1.,-6.44065666513476E-13));
#12578=DIRECTION('ref_axis',(0.628654464493172,5.49054993151786E-13,-0.777684746071827));
#12579=DIRECTION('center_axis',(-4.16203559120935E-32,-4.16203559120936E-32,
-1.));
#12580=DIRECTION('ref_axis',(3.64246399155235E-15,-1.,4.16203559120935E-32));
#12581=DIRECTION('center_axis',(-1.,-5.22244552898928E-14,3.38377885085076E-13));
#12582=DIRECTION('ref_axis',(-2.88015160457499E-13,0.662700408673497,-0.748884616175269));
#12583=DIRECTION('center_axis',(-4.16203559120935E-32,-4.16203559120936E-32,
-1.));
#12584=DIRECTION('ref_axis',(3.49148133884313E-15,-1.,4.16203559120935E-32));
#12585=DIRECTION('',(1.,3.49148133884313E-15,-4.16203559120936E-32));
#12586=DIRECTION('',(3.49148133884313E-15,-1.,4.16203559120935E-32));
#12587=DIRECTION('center_axis',(-4.16203559120935E-32,-4.16203559120936E-32,
-1.));
#12588=DIRECTION('ref_axis',(3.49148133884313E-15,-1.,4.16203559120935E-32));
#12589=DIRECTION('',(3.49148133884313E-15,-1.,4.16203559120935E-32));
#12590=DIRECTION('',(1.,3.49148133884313E-15,-4.16203559120936E-32));
#12591=DIRECTION('center_axis',(-4.16203559120935E-32,-4.16203559120936E-32,
-1.));
#12592=DIRECTION('ref_axis',(3.49148133884313E-15,-1.,4.16203559120935E-32));
#12593=DIRECTION('',(1.,3.49148133884313E-15,-4.16203559120936E-32));
#12594=DIRECTION('',(3.49148133884313E-15,-1.,4.16203559120935E-32));
#12595=DIRECTION('center_axis',(-4.16203559120935E-32,-4.16203559120936E-32,
-1.));
#12596=DIRECTION('ref_axis',(3.49148133884313E-15,-1.,4.16203559120935E-32));
#12597=DIRECTION('center_axis',(-4.16203559120935E-32,-4.16203559120936E-32,
-1.));
#12598=DIRECTION('ref_axis',(3.49148133884313E-15,-1.,4.16203559120935E-32));
#12599=DIRECTION('',(1.,3.49148133884313E-15,-4.16203559120936E-32));
#12600=DIRECTION('',(3.49148133884313E-15,-1.,4.16203559120935E-32));
#12601=DIRECTION('center_axis',(-3.49148133884313E-15,1.,-4.16203559120935E-32));
#12602=DIRECTION('ref_axis',(-4.16203559120935E-32,-4.16203559120937E-32,
-1.));
#12603=DIRECTION('',(-4.16203559120935E-32,-4.16203559120936E-32,-1.));
#12604=DIRECTION('',(1.,3.49148133884313E-15,-4.16203559120936E-32));
#12605=DIRECTION('',(-4.16203559120935E-32,-4.16203559120936E-32,-1.));
#12606=DIRECTION('center_axis',(-3.49148133884313E-15,1.,-4.16203559120935E-32));
#12607=DIRECTION('ref_axis',(-4.16203559120935E-32,-4.16203559120937E-32,
-1.));
#12608=DIRECTION('',(-4.16203559120935E-32,-4.16203559120936E-32,-1.));
#12609=DIRECTION('',(1.,3.49148133884313E-15,-4.16203559120936E-32));
#12610=DIRECTION('',(-4.16203559120935E-32,-4.16203559120936E-32,-1.));
#12611=DIRECTION('center_axis',(-3.49148133884313E-15,1.,-4.16203559120935E-32));
#12612=DIRECTION('ref_axis',(-4.16203559120935E-32,-4.16203559120937E-32,
-1.));
#12613=DIRECTION('',(-4.16203559120935E-32,-4.16203559120936E-32,-1.));
#12614=DIRECTION('',(1.,3.49148133884313E-15,-4.16203559120936E-32));
#12615=DIRECTION('',(-4.16203559120935E-32,-4.16203559120936E-32,-1.));
#12616=DIRECTION('center_axis',(1.,3.49148133884313E-15,-4.16203559120936E-32));
#12617=DIRECTION('ref_axis',(-4.16203559120935E-32,-4.16203559120936E-32,
-1.));
#12618=DIRECTION('',(3.49148133884313E-15,-1.,4.16203559120935E-32));
#12619=DIRECTION('center_axis',(-3.49148133884313E-15,1.,-4.16203559120935E-32));
#12620=DIRECTION('ref_axis',(-4.16203559120935E-32,-4.16203559120937E-32,
-1.));
#12621=DIRECTION('',(-4.16203559120935E-32,-4.16203559120936E-32,-1.));
#12622=DIRECTION('',(1.,3.49148133884313E-15,-4.16203559120936E-32));
#12623=DIRECTION('',(-4.16203559120935E-32,-4.16203559120936E-32,-1.));
#12624=DIRECTION('center_axis',(-1.,-3.49148133884313E-15,4.16203559120936E-32));
#12625=DIRECTION('ref_axis',(4.16203559120935E-32,4.16203559120936E-32,
1.));
#12626=DIRECTION('',(-3.49148133884313E-15,1.,-4.16203559120935E-32));
#12627=DIRECTION('center_axis',(-4.16203559120935E-32,-4.16203559120936E-32,
-1.));
#12628=DIRECTION('ref_axis',(3.49148133884313E-15,-1.,4.16203559120935E-32));
#12629=DIRECTION('',(3.49148133884313E-15,-1.,4.16203559120935E-32));
#12630=DIRECTION('',(1.,3.49148133884313E-15,-4.16203559120936E-32));
#12631=DIRECTION('',(3.49148133884313E-15,-1.,4.16203559120935E-32));
#12632=DIRECTION('',(3.49148133884313E-15,-1.,4.16203559120935E-32));
#12633=DIRECTION('',(-1.,-3.49148133884313E-15,4.16203559120936E-32));
#12634=DIRECTION('',(3.49148133884313E-15,-1.,4.16203559120935E-32));
#12635=DIRECTION('center_axis',(-3.49148133884313E-15,1.,-4.16203559120935E-32));
#12636=DIRECTION('ref_axis',(-4.16203559120935E-32,-4.16203559120937E-32,
-1.));
#12637=DIRECTION('',(-4.16203559120935E-32,-4.16203559120936E-32,-1.));
#12638=DIRECTION('',(-4.16203559120935E-32,-4.16203559120936E-32,-1.));
#12639=DIRECTION('center_axis',(1.,3.49148133884313E-15,-4.16203559120936E-32));
#12640=DIRECTION('ref_axis',(-4.16203559120935E-32,-4.16203559120936E-32,
-1.));
#12641=DIRECTION('center_axis',(1.,3.49148133884313E-15,-4.16203559120936E-32));
#12642=DIRECTION('ref_axis',(-4.16203559120935E-32,-4.16203559120936E-32,
-1.));
#12643=DIRECTION('center_axis',(1.,3.49148133884313E-15,-4.16203559120936E-32));
#12644=DIRECTION('ref_axis',(-4.16203559120935E-32,-4.16203559120936E-32,
-1.));
#12645=DIRECTION('',(-4.16203559120935E-32,-4.16203559120936E-32,-1.));
#12646=DIRECTION('center_axis',(3.49148133884313E-15,-1.,4.16203559120935E-32));
#12647=DIRECTION('ref_axis',(4.16203559120935E-32,4.16203559120937E-32,
1.));
#12648=DIRECTION('',(-4.16203559120935E-32,-4.16203559120936E-32,-1.));
#12649=DIRECTION('center_axis',(1.,3.49148133884313E-15,-4.16203559120936E-32));
#12650=DIRECTION('ref_axis',(-4.16203559120935E-32,-4.16203559120936E-32,
-1.));
#12651=DIRECTION('center_axis',(0.,8.3240711824187E-32,1.));
#12652=DIRECTION('ref_axis',(-1.,0.,0.));
#12653=DIRECTION('center_axis',(0.,-8.3240711824187E-32,-1.));
#12654=DIRECTION('ref_axis',(1.,0.,0.));
#12655=DIRECTION('',(0.,-8.3240711824187E-32,-1.));
#12656=DIRECTION('center_axis',(0.,8.3240711824187E-32,1.));
#12657=DIRECTION('ref_axis',(1.,0.,0.));
#12658=DIRECTION('center_axis',(0.,8.3240711824187E-32,1.));
#12659=DIRECTION('ref_axis',(1.,0.,0.));
#12660=DIRECTION('center_axis',(0.,-8.3240711824187E-32,-1.));
#12661=DIRECTION('ref_axis',(1.,0.,0.));
#12662=DIRECTION('center_axis',(0.,1.,-8.3240711824187E-32));
#12663=DIRECTION('ref_axis',(-1.,0.,0.));
#12664=DIRECTION('center_axis',(0.,-1.,0.));
#12665=DIRECTION('ref_axis',(-0.662700408463881,0.,-0.748884616360762));
#12666=DIRECTION('center_axis',(0.,-8.3240711824187E-32,-1.));
#12667=DIRECTION('ref_axis',(1.,0.,0.));
#12668=DIRECTION('center_axis',(1.,1.23033231110227E-14,1.91813075638571E-13));
#12669=DIRECTION('ref_axis',(-1.51799278823133E-13,0.662700408404006,0.748884616413746));
#12670=DIRECTION('center_axis',(1.,6.87436171423541E-14,6.46003611483159E-13));
#12671=DIRECTION('ref_axis',(-5.29338589993441E-13,0.662700408303445,0.748884616502734));
#12672=DIRECTION('center_axis',(0.,-8.3240711824187E-32,-1.));
#12673=DIRECTION('ref_axis',(1.,0.,0.));
#12674=DIRECTION('center_axis',(2.42515865283882E-14,-1.,-2.2795089778668E-13));
#12675=DIRECTION('ref_axis',(0.628654464794611,1.92519804155958E-13,-0.777684745828154));
#12676=DIRECTION('center_axis',(-2.42515865283884E-14,-1.,2.27950897786681E-13));
#12677=DIRECTION('ref_axis',(0.628654464776,-1.92519804158937E-13,-0.777684745843199));
#12678=DIRECTION('center_axis',(0.,-8.3240711824187E-32,-1.));
#12679=DIRECTION('ref_axis',(1.,0.,0.));
#12680=DIRECTION('center_axis',(1.,4.42963920865616E-14,-3.40131136130303E-13));
#12681=DIRECTION('ref_axis',(2.92361920824713E-13,-0.628654464727554,0.777684745882361));
#12682=DIRECTION('center_axis',(1.,8.06737718791901E-14,-6.82057482811295E-13));
#12683=DIRECTION('ref_axis',(5.81141627215589E-13,-0.628654464429985,0.777684746122906));
#12684=DIRECTION('center_axis',(0.,-8.3240711824187E-32,-1.));
#12685=DIRECTION('ref_axis',(1.,0.,0.));
#12686=DIRECTION('center_axis',(4.02653252918805E-14,-1.,3.02189686082951E-13));
#12687=DIRECTION('ref_axis',(-0.662700408561431,-2.52989054626112E-13,-0.748884616274438));
#12688=DIRECTION('center_axis',(0.,-8.3240711824187E-32,-1.));
#12689=DIRECTION('ref_axis',(1.,0.,0.));
#12690=DIRECTION('',(0.,1.,-8.3240711824187E-32));
#12691=DIRECTION('',(1.,0.,0.));
#12692=DIRECTION('center_axis',(0.,-8.3240711824187E-32,-1.));
#12693=DIRECTION('ref_axis',(1.,0.,0.));
#12694=DIRECTION('',(1.,0.,0.));
#12695=DIRECTION('',(0.,1.,-8.3240711824187E-32));
#12696=DIRECTION('center_axis',(0.,-8.3240711824187E-32,-1.));
#12697=DIRECTION('ref_axis',(1.,0.,0.));
#12698=DIRECTION('',(0.,1.,-8.3240711824187E-32));
#12699=DIRECTION('',(1.,0.,0.));
#12700=DIRECTION('center_axis',(0.,-8.3240711824187E-32,-1.));
#12701=DIRECTION('ref_axis',(1.,0.,0.));
#12702=DIRECTION('center_axis',(0.,-8.3240711824187E-32,-1.));
#12703=DIRECTION('ref_axis',(1.,0.,0.));
#12704=DIRECTION('',(0.,1.,-8.3240711824187E-32));
#12705=DIRECTION('',(1.,0.,0.));
#12706=DIRECTION('center_axis',(-1.,0.,0.));
#12707=DIRECTION('ref_axis',(0.,-8.3240711824187E-32,-1.));
#12708=DIRECTION('',(0.,-8.3240711824187E-32,-1.));
#12709=DIRECTION('',(0.,1.,-8.3240711824187E-32));
#12710=DIRECTION('',(0.,-8.3240711824187E-32,-1.));
#12711=DIRECTION('center_axis',(-1.,0.,0.));
#12712=DIRECTION('ref_axis',(0.,-8.3240711824187E-32,-1.));
#12713=DIRECTION('',(0.,-8.3240711824187E-32,-1.));
#12714=DIRECTION('',(0.,1.,-8.3240711824187E-32));
#12715=DIRECTION('',(0.,-8.3240711824187E-32,-1.));
#12716=DIRECTION('center_axis',(-1.,0.,0.));
#12717=DIRECTION('ref_axis',(0.,-8.3240711824187E-32,-1.));
#12718=DIRECTION('',(0.,-8.3240711824187E-32,-1.));
#12719=DIRECTION('',(0.,1.,-8.3240711824187E-32));
#12720=DIRECTION('',(0.,-8.3240711824187E-32,-1.));
#12721=DIRECTION('center_axis',(0.,1.,-8.3240711824187E-32));
#12722=DIRECTION('ref_axis',(0.,-8.3240711824187E-32,-1.));
#12723=DIRECTION('',(1.,0.,0.));
#12724=DIRECTION('center_axis',(-1.,0.,0.));
#12725=DIRECTION('ref_axis',(0.,-8.3240711824187E-32,-1.));
#12726=DIRECTION('',(0.,-8.3240711824187E-32,-1.));
#12727=DIRECTION('',(0.,1.,-8.3240711824187E-32));
#12728=DIRECTION('',(0.,-8.3240711824187E-32,-1.));
#12729=DIRECTION('center_axis',(0.,-1.,8.3240711824187E-32));
#12730=DIRECTION('ref_axis',(0.,8.3240711824187E-32,1.));
#12731=DIRECTION('',(-1.,0.,0.));
#12732=DIRECTION('center_axis',(0.,-8.3240711824187E-32,-1.));
#12733=DIRECTION('ref_axis',(1.,0.,0.));
#12734=DIRECTION('',(1.,0.,0.));
#12735=DIRECTION('',(0.,1.,-8.3240711824187E-32));
#12736=DIRECTION('',(1.,0.,0.));
#12737=DIRECTION('',(1.,0.,0.));
#12738=DIRECTION('',(0.,-1.,8.3240711824187E-32));
#12739=DIRECTION('',(1.,0.,0.));
#12740=DIRECTION('center_axis',(-1.,0.,0.));
#12741=DIRECTION('ref_axis',(0.,-8.3240711824187E-32,-1.));
#12742=DIRECTION('',(0.,-8.3240711824187E-32,-1.));
#12743=DIRECTION('',(0.,-8.3240711824187E-32,-1.));
#12744=DIRECTION('center_axis',(0.,1.,-8.3240711824187E-32));
#12745=DIRECTION('ref_axis',(0.,-8.3240711824187E-32,-1.));
#12746=DIRECTION('center_axis',(0.,1.,-8.3240711824187E-32));
#12747=DIRECTION('ref_axis',(0.,-8.3240711824187E-32,-1.));
#12748=DIRECTION('center_axis',(0.,1.,-8.3240711824187E-32));
#12749=DIRECTION('ref_axis',(0.,-8.3240711824187E-32,-1.));
#12750=DIRECTION('',(0.,-8.3240711824187E-32,-1.));
#12751=DIRECTION('center_axis',(1.,0.,0.));
#12752=DIRECTION('ref_axis',(0.,8.3240711824187E-32,1.));
#12753=DIRECTION('',(0.,-8.3240711824187E-32,-1.));
#12754=DIRECTION('center_axis',(0.,1.,-8.3240711824187E-32));
#12755=DIRECTION('ref_axis',(0.,-8.3240711824187E-32,-1.));
#12756=DIRECTION('center_axis',(-4.16203559120935E-32,4.16203559120931E-32,
1.));
#12757=DIRECTION('ref_axis',(1.03810223759242E-14,-1.,4.16203559120935E-32));
#12758=DIRECTION('center_axis',(4.16203559120935E-32,-4.16203559120931E-32,
-1.));
#12759=DIRECTION('ref_axis',(-1.03810223759242E-14,1.,-4.16203559120935E-32));
#12760=DIRECTION('',(4.16203559120935E-32,-4.16203559120931E-32,-1.));
#12761=DIRECTION('center_axis',(-4.16203559120935E-32,4.16203559120931E-32,
1.));
#12762=DIRECTION('ref_axis',(-9.83465277719135E-15,1.,-4.16203559120935E-32));
#12763=DIRECTION('center_axis',(-4.16203559120935E-32,4.16203559120931E-32,
1.));
#12764=DIRECTION('ref_axis',(-9.83465277719135E-15,1.,-4.16203559120935E-32));
#12765=DIRECTION('center_axis',(4.16203559120935E-32,-4.16203559120931E-32,
-1.));
#12766=DIRECTION('ref_axis',(-1.00706844438439E-14,1.,0.));
#12767=DIRECTION('center_axis',(-1.,-9.79094320929272E-15,-4.16203559120931E-32));
#12768=DIRECTION('ref_axis',(9.79094320929272E-15,-1.,0.));
#12769=DIRECTION('center_axis',(1.,3.18336478092136E-14,7.05643845663474E-14));
#12770=DIRECTION('ref_axis',(-7.39407534612729E-14,0.66270040877393,0.748884616086394));
#12771=DIRECTION('center_axis',(4.16203559120935E-32,-4.16203559120931E-32,
-1.));
#12772=DIRECTION('ref_axis',(-1.0927391974657E-14,1.,-4.16203559120936E-32));
#12773=DIRECTION('center_axis',(-4.81807131050712E-14,1.,3.00377672645013E-13));
#12774=DIRECTION('ref_axis',(-0.662700408385393,-2.56877596413992E-13,0.748884616430217));
#12775=DIRECTION('center_axis',(-5.66123905878238E-14,1.,5.32002974162615E-13));
#12776=DIRECTION('ref_axis',(-0.662700408320119,-4.35925897634763E-13,0.748884616487979));
#12777=DIRECTION('center_axis',(4.16203559120935E-32,-4.16203559120931E-32,
-1.));
#12778=DIRECTION('ref_axis',(-1.0927391974657E-14,1.,-4.16203559120936E-32));
#12779=DIRECTION('center_axis',(1.,3.62125299104317E-14,-2.64147503534732E-13));
#12780=DIRECTION('ref_axis',(2.28188652755739E-13,-0.628654464803139,0.777684745821261));
#12781=DIRECTION('center_axis',(1.,-8.41356194042581E-15,2.31541318886086E-13));
#12782=DIRECTION('ref_axis',(-1.85355374991887E-13,-0.628654464869737,0.777684745767425));
#12783=DIRECTION('center_axis',(4.16203559120935E-32,-4.16203559120931E-32,
-1.));
#12784=DIRECTION('ref_axis',(-1.0927391974657E-14,1.,-4.16203559120936E-32));
#12785=DIRECTION('center_axis',(-5.60924855864494E-14,1.,-2.98548898733053E-13));
#12786=DIRECTION('ref_axis',(0.628654464448989,2.67439715997863E-13,0.777684746107544));
#12787=DIRECTION('center_axis',(-8.06737718791917E-14,1.,-6.82057482811304E-13));
#12788=DIRECTION('ref_axis',(0.628654464496999,5.81141627184055E-13,0.777684746068734));
#12789=DIRECTION('center_axis',(4.16203559120935E-32,-4.16203559120931E-32,
-1.));
#12790=DIRECTION('ref_axis',(-1.0927391974657E-14,1.,-4.16203559120936E-32));
#12791=DIRECTION('center_axis',(1.,2.42624531090294E-14,2.28001274640695E-13));
#12792=DIRECTION('ref_axis',(-1.86825384661082E-13,0.662700408540891,0.748884616292614));
#12793=DIRECTION('center_axis',(4.16203559120935E-32,-4.16203559120931E-32,
-1.));
#12794=DIRECTION('ref_axis',(-1.04744440165294E-14,1.,-4.16203559120935E-32));
#12795=DIRECTION('',(-1.,-1.04744440165294E-14,-4.16203559120931E-32));
#12796=DIRECTION('',(-1.04744440165294E-14,1.,-4.16203559120935E-32));
#12797=DIRECTION('center_axis',(4.16203559120935E-32,-4.16203559120931E-32,
-1.));
#12798=DIRECTION('ref_axis',(-1.04744440165294E-14,1.,-4.16203559120935E-32));
#12799=DIRECTION('',(-1.04744440165294E-14,1.,-4.16203559120935E-32));
#12800=DIRECTION('',(-1.,-1.04744440165294E-14,-4.16203559120931E-32));
#12801=DIRECTION('center_axis',(4.16203559120935E-32,-4.16203559120931E-32,
-1.));
#12802=DIRECTION('ref_axis',(-1.04744440165294E-14,1.,-4.16203559120935E-32));
#12803=DIRECTION('',(-1.,-1.04744440165294E-14,-4.16203559120931E-32));
#12804=DIRECTION('',(-1.04744440165294E-14,1.,-4.16203559120935E-32));
#12805=DIRECTION('center_axis',(4.16203559120935E-32,-4.16203559120931E-32,
-1.));
#12806=DIRECTION('ref_axis',(-1.04744440165294E-14,1.,-4.16203559120935E-32));
#12807=DIRECTION('center_axis',(4.16203559120935E-32,-4.16203559120931E-32,
-1.));
#12808=DIRECTION('ref_axis',(-1.04744440165294E-14,1.,-4.16203559120935E-32));
#12809=DIRECTION('',(-1.,-1.04744440165294E-14,-4.16203559120931E-32));
#12810=DIRECTION('',(-1.04744440165294E-14,1.,-4.16203559120935E-32));
#12811=DIRECTION('center_axis',(1.04744440165294E-14,-1.,4.16203559120935E-32));
#12812=DIRECTION('ref_axis',(4.16203559120935E-32,-4.16203559120931E-32,
-1.));
#12813=DIRECTION('',(4.16203559120935E-32,-4.16203559120931E-32,-1.));
#12814=DIRECTION('',(-1.,-1.04744440165294E-14,-4.16203559120931E-32));
#12815=DIRECTION('',(4.16203559120935E-32,-4.16203559120931E-32,-1.));
#12816=DIRECTION('center_axis',(1.04744440165294E-14,-1.,4.16203559120935E-32));
#12817=DIRECTION('ref_axis',(4.16203559120935E-32,-4.16203559120931E-32,
-1.));
#12818=DIRECTION('',(4.16203559120935E-32,-4.16203559120931E-32,-1.));
#12819=DIRECTION('',(-1.,-1.04744440165294E-14,-4.16203559120931E-32));
#12820=DIRECTION('',(4.16203559120935E-32,-4.16203559120931E-32,-1.));
#12821=DIRECTION('center_axis',(1.04744440165294E-14,-1.,4.16203559120935E-32));
#12822=DIRECTION('ref_axis',(4.16203559120935E-32,-4.16203559120931E-32,
-1.));
#12823=DIRECTION('',(4.16203559120935E-32,-4.16203559120931E-32,-1.));
#12824=DIRECTION('',(-1.,-1.04744440165294E-14,-4.16203559120931E-32));
#12825=DIRECTION('',(4.16203559120935E-32,-4.16203559120931E-32,-1.));
#12826=DIRECTION('center_axis',(-1.,-1.04744440165294E-14,-4.16203559120931E-32));
#12827=DIRECTION('ref_axis',(4.16203559120935E-32,-4.16203559120931E-32,
-1.));
#12828=DIRECTION('',(-1.04744440165294E-14,1.,-4.16203559120935E-32));
#12829=DIRECTION('center_axis',(1.04744440165294E-14,-1.,4.16203559120935E-32));
#12830=DIRECTION('ref_axis',(4.16203559120935E-32,-4.16203559120931E-32,
-1.));
#12831=DIRECTION('',(4.16203559120935E-32,-4.16203559120931E-32,-1.));
#12832=DIRECTION('',(-1.,-1.04744440165294E-14,-4.16203559120931E-32));
#12833=DIRECTION('',(4.16203559120935E-32,-4.16203559120931E-32,-1.));
#12834=DIRECTION('center_axis',(1.,1.04744440165294E-14,4.16203559120931E-32));
#12835=DIRECTION('ref_axis',(-4.16203559120935E-32,4.16203559120931E-32,
1.));
#12836=DIRECTION('',(1.04744440165294E-14,-1.,4.16203559120935E-32));
#12837=DIRECTION('center_axis',(4.16203559120935E-32,-4.16203559120931E-32,
-1.));
#12838=DIRECTION('ref_axis',(-1.04744440165294E-14,1.,-4.16203559120935E-32));
#12839=DIRECTION('',(-1.04744440165294E-14,1.,-4.16203559120935E-32));
#12840=DIRECTION('',(-1.,-1.04744440165294E-14,-4.16203559120931E-32));
#12841=DIRECTION('',(-1.04744440165294E-14,1.,-4.16203559120935E-32));
#12842=DIRECTION('',(-1.04744440165294E-14,1.,-4.16203559120935E-32));
#12843=DIRECTION('',(1.,1.04744440165294E-14,4.16203559120931E-32));
#12844=DIRECTION('',(-1.04744440165294E-14,1.,-4.16203559120935E-32));
#12845=DIRECTION('center_axis',(1.04744440165294E-14,-1.,4.16203559120935E-32));
#12846=DIRECTION('ref_axis',(4.16203559120935E-32,-4.16203559120931E-32,
-1.));
#12847=DIRECTION('',(4.16203559120935E-32,-4.16203559120931E-32,-1.));
#12848=DIRECTION('',(4.16203559120935E-32,-4.16203559120931E-32,-1.));
#12849=DIRECTION('center_axis',(-1.,-1.04744440165294E-14,-4.16203559120931E-32));
#12850=DIRECTION('ref_axis',(4.16203559120935E-32,-4.16203559120931E-32,
-1.));
#12851=DIRECTION('center_axis',(-1.,-1.04744440165294E-14,-4.16203559120931E-32));
#12852=DIRECTION('ref_axis',(4.16203559120935E-32,-4.16203559120931E-32,
-1.));
#12853=DIRECTION('center_axis',(-1.,-1.04744440165294E-14,-4.16203559120931E-32));
#12854=DIRECTION('ref_axis',(4.16203559120935E-32,-4.16203559120931E-32,
-1.));
#12855=DIRECTION('',(4.16203559120935E-32,-4.16203559120931E-32,-1.));
#12856=DIRECTION('center_axis',(-1.04744440165294E-14,1.,-4.16203559120935E-32));
#12857=DIRECTION('ref_axis',(-4.16203559120935E-32,4.16203559120931E-32,
1.));
#12858=DIRECTION('',(4.16203559120935E-32,-4.16203559120931E-32,-1.));
#12859=DIRECTION('center_axis',(-1.,-1.04744440165294E-14,-4.16203559120931E-32));
#12860=DIRECTION('ref_axis',(4.16203559120935E-32,-4.16203559120931E-32,
-1.));
#12861=DIRECTION('center_axis',(0.,0.,1.));
#12862=DIRECTION('ref_axis',(1.,0.,0.));
#12863=DIRECTION('',(0.,0.,1.));
#12864=DIRECTION('center_axis',(0.,0.,1.));
#12865=DIRECTION('ref_axis',(-1.,0.,0.));
#12866=DIRECTION('center_axis',(0.,0.,1.));
#12867=DIRECTION('ref_axis',(1.,0.,0.));
#12868=DIRECTION('',(0.,0.,1.));
#12869=DIRECTION('center_axis',(0.,0.,1.));
#12870=DIRECTION('ref_axis',(1.,0.,0.));
#12871=DIRECTION('',(0.,0.,1.));
#12872=DIRECTION('center_axis',(0.,0.,1.));
#12873=DIRECTION('ref_axis',(1.,0.,0.));
#12874=DIRECTION('',(0.,0.,1.));
#12875=DIRECTION('center_axis',(0.,0.,1.));
#12876=DIRECTION('ref_axis',(1.,0.,0.));
#12877=DIRECTION('',(0.,0.,1.));
#12878=DIRECTION('center_axis',(0.,0.,1.));
#12879=DIRECTION('ref_axis',(1.,0.,0.));
#12880=DIRECTION('',(0.,0.,1.));
#12881=DIRECTION('center_axis',(0.,0.,1.));
#12882=DIRECTION('ref_axis',(1.,0.,0.));
#12883=DIRECTION('',(0.,0.,1.));
#12884=DIRECTION('center_axis',(0.,0.,1.));
#12885=DIRECTION('ref_axis',(1.,0.,0.));
#12886=DIRECTION('',(0.,0.,1.));
#12887=DIRECTION('center_axis',(0.,0.,1.));
#12888=DIRECTION('ref_axis',(1.,0.,0.));
#12889=DIRECTION('',(0.,0.,1.));
#12890=DIRECTION('center_axis',(0.,0.,1.));
#12891=DIRECTION('ref_axis',(1.,0.,0.));
#12892=DIRECTION('',(0.,0.,1.));
#12893=DIRECTION('center_axis',(0.,0.,1.));
#12894=DIRECTION('ref_axis',(1.,0.,0.));
#12895=DIRECTION('',(0.,0.,1.));
#12896=DIRECTION('center_axis',(0.,0.,1.));
#12897=DIRECTION('ref_axis',(1.,0.,0.));
#12898=DIRECTION('',(0.,0.,1.));
#12899=DIRECTION('center_axis',(0.,0.,1.));
#12900=DIRECTION('ref_axis',(1.,0.,0.));
#12901=DIRECTION('',(0.,0.,1.));
#12902=DIRECTION('center_axis',(0.,0.,1.));
#12903=DIRECTION('ref_axis',(1.,0.,0.));
#12904=DIRECTION('',(0.,0.,1.));
#12905=DIRECTION('center_axis',(0.,0.,1.));
#12906=DIRECTION('ref_axis',(1.,0.,0.));
#12907=DIRECTION('',(0.,0.,1.));
#12908=DIRECTION('center_axis',(0.,0.,1.));
#12909=DIRECTION('ref_axis',(1.,0.,0.));
#12910=DIRECTION('',(0.,0.,1.));
#12911=DIRECTION('center_axis',(0.,0.,1.));
#12912=DIRECTION('ref_axis',(1.,0.,0.));
#12913=DIRECTION('',(0.,0.,1.));
#12914=DIRECTION('center_axis',(0.,0.,1.));
#12915=DIRECTION('ref_axis',(1.,0.,0.));
#12916=DIRECTION('',(0.,0.,1.));
#12917=DIRECTION('center_axis',(0.,0.,1.));
#12918=DIRECTION('ref_axis',(1.,0.,0.));
#12919=DIRECTION('',(0.,0.,1.));
#12920=DIRECTION('center_axis',(0.,0.,1.));
#12921=DIRECTION('ref_axis',(1.,0.,0.));
#12922=DIRECTION('',(0.,0.,1.));
#12923=DIRECTION('center_axis',(0.,0.,1.));
#12924=DIRECTION('ref_axis',(-1.,0.,0.));
#12925=DIRECTION('center_axis',(0.,0.,1.));
#12926=DIRECTION('ref_axis',(1.,0.,0.));
#12927=DIRECTION('',(0.,0.,1.));
#12928=DIRECTION('center_axis',(0.,0.,1.));
#12929=DIRECTION('ref_axis',(1.,0.,0.));
#12930=DIRECTION('',(0.,0.,1.));
#12931=DIRECTION('center_axis',(0.,0.,1.));
#12932=DIRECTION('ref_axis',(1.,0.,0.));
#12933=DIRECTION('',(0.,0.,1.));
#12934=DIRECTION('center_axis',(0.,0.,1.));
#12935=DIRECTION('ref_axis',(1.,0.,0.));
#12936=DIRECTION('',(0.,0.,1.));
#12937=DIRECTION('center_axis',(0.,0.,1.));
#12938=DIRECTION('ref_axis',(1.,0.,0.));
#12939=DIRECTION('',(0.,0.,1.));
#12940=DIRECTION('center_axis',(0.,0.,1.));
#12941=DIRECTION('ref_axis',(1.,0.,0.));
#12942=DIRECTION('',(0.,0.,1.));
#12943=DIRECTION('center_axis',(0.,0.,1.));
#12944=DIRECTION('ref_axis',(1.,0.,0.));
#12945=DIRECTION('',(0.,0.,1.));
#12946=DIRECTION('center_axis',(0.,0.,1.));
#12947=DIRECTION('ref_axis',(1.,0.,0.));
#12948=DIRECTION('',(0.,0.,1.));
#12949=DIRECTION('center_axis',(0.,0.,1.));
#12950=DIRECTION('ref_axis',(1.,0.,0.));
#12951=DIRECTION('',(0.,0.,1.));
#12952=DIRECTION('center_axis',(0.,0.,1.));
#12953=DIRECTION('ref_axis',(1.,0.,0.));
#12954=DIRECTION('',(0.,0.,1.));
#12955=DIRECTION('center_axis',(0.,0.,1.));
#12956=DIRECTION('ref_axis',(1.,0.,0.));
#12957=DIRECTION('',(0.,0.,1.));
#12958=DIRECTION('center_axis',(0.,0.,1.));
#12959=DIRECTION('ref_axis',(1.,0.,0.));
#12960=DIRECTION('',(0.,0.,1.));
#12961=DIRECTION('center_axis',(0.,0.,1.));
#12962=DIRECTION('ref_axis',(1.,0.,0.));
#12963=DIRECTION('',(0.,0.,1.));
#12964=DIRECTION('center_axis',(0.,0.,1.));
#12965=DIRECTION('ref_axis',(1.,0.,0.));
#12966=DIRECTION('',(0.,0.,1.));
#12967=DIRECTION('center_axis',(0.,0.,1.));
#12968=DIRECTION('ref_axis',(1.,0.,0.));
#12969=DIRECTION('',(0.,0.,1.));
#12970=DIRECTION('center_axis',(0.,0.,1.));
#12971=DIRECTION('ref_axis',(1.,0.,0.));
#12972=DIRECTION('',(0.,0.,1.));
#12973=DIRECTION('center_axis',(0.,0.,1.));
#12974=DIRECTION('ref_axis',(1.,0.,0.));
#12975=DIRECTION('',(0.,0.,1.));
#12976=DIRECTION('center_axis',(0.,0.,1.));
#12977=DIRECTION('ref_axis',(1.,0.,0.));
#12978=DIRECTION('',(0.,0.,1.));
#12979=DIRECTION('center_axis',(0.,0.,1.));
#12980=DIRECTION('ref_axis',(1.,0.,0.));
#12981=DIRECTION('',(0.,0.,1.));
#12982=DIRECTION('center_axis',(0.,0.,1.));
#12983=DIRECTION('ref_axis',(-1.,-7.9041468616686E-13,0.));
#12984=DIRECTION('center_axis',(0.,0.,1.));
#12985=DIRECTION('ref_axis',(1.,0.,0.));
#12986=DIRECTION('',(0.,0.,1.));
#12987=DIRECTION('center_axis',(0.,0.,1.));
#12988=DIRECTION('ref_axis',(1.,0.,0.));
#12989=DIRECTION('',(0.,0.,1.));
#12990=DIRECTION('center_axis',(0.,0.,1.));
#12991=DIRECTION('ref_axis',(1.,0.,0.));
#12992=DIRECTION('',(0.,0.,1.));
#12993=DIRECTION('center_axis',(0.,0.,1.));
#12994=DIRECTION('ref_axis',(1.,0.,0.));
#12995=DIRECTION('',(0.,0.,1.));
#12996=DIRECTION('center_axis',(0.,0.,1.));
#12997=DIRECTION('ref_axis',(1.,0.,0.));
#12998=DIRECTION('',(0.,0.,1.));
#12999=DIRECTION('center_axis',(0.,0.,1.));
#13000=DIRECTION('ref_axis',(1.,0.,0.));
#13001=DIRECTION('',(0.,0.,1.));
#13002=DIRECTION('center_axis',(0.,0.,1.));
#13003=DIRECTION('ref_axis',(1.,0.,0.));
#13004=DIRECTION('',(0.,0.,1.));
#13005=DIRECTION('center_axis',(0.,0.,1.));
#13006=DIRECTION('ref_axis',(1.,0.,0.));
#13007=DIRECTION('',(0.,0.,1.));
#13008=DIRECTION('center_axis',(0.,0.,1.));
#13009=DIRECTION('ref_axis',(1.,0.,0.));
#13010=DIRECTION('',(0.,0.,1.));
#13011=DIRECTION('center_axis',(0.,0.,1.));
#13012=DIRECTION('ref_axis',(1.,0.,0.));
#13013=DIRECTION('',(0.,0.,1.));
#13014=DIRECTION('center_axis',(0.,0.,1.));
#13015=DIRECTION('ref_axis',(1.,0.,0.));
#13016=DIRECTION('',(0.,0.,1.));
#13017=DIRECTION('center_axis',(0.,0.,1.));
#13018=DIRECTION('ref_axis',(1.,0.,0.));
#13019=DIRECTION('',(0.,0.,1.));
#13020=DIRECTION('center_axis',(0.,0.,1.));
#13021=DIRECTION('ref_axis',(1.,0.,0.));
#13022=DIRECTION('',(0.,0.,1.));
#13023=DIRECTION('center_axis',(0.,0.,1.));
#13024=DIRECTION('ref_axis',(1.,0.,0.));
#13025=DIRECTION('',(0.,0.,1.));
#13026=DIRECTION('center_axis',(0.,0.,1.));
#13027=DIRECTION('ref_axis',(1.,0.,0.));
#13028=DIRECTION('',(0.,0.,1.));
#13029=DIRECTION('center_axis',(0.,0.,1.));
#13030=DIRECTION('ref_axis',(1.,0.,0.));
#13031=DIRECTION('',(0.,0.,1.));
#13032=DIRECTION('center_axis',(0.,0.,1.));
#13033=DIRECTION('ref_axis',(1.,0.,0.));
#13034=DIRECTION('',(0.,0.,1.));
#13035=DIRECTION('center_axis',(0.,0.,1.));
#13036=DIRECTION('ref_axis',(1.,0.,0.));
#13037=DIRECTION('',(0.,0.,1.));
#13038=DIRECTION('center_axis',(0.,0.,1.));
#13039=DIRECTION('ref_axis',(1.,0.,0.));
#13040=DIRECTION('',(0.,0.,1.));
#13041=DIRECTION('center_axis',(0.,0.,1.));
#13042=DIRECTION('ref_axis',(-1.,1.82123199577617E-15,0.));
#13043=DIRECTION('center_axis',(0.,0.,1.));
#13044=DIRECTION('ref_axis',(1.,0.,0.));
#13045=DIRECTION('',(0.,0.,1.));
#13046=DIRECTION('center_axis',(0.,0.,1.));
#13047=DIRECTION('ref_axis',(1.,0.,0.));
#13048=DIRECTION('',(0.,0.,1.));
#13049=DIRECTION('center_axis',(0.,0.,1.));
#13050=DIRECTION('ref_axis',(1.,0.,0.));
#13051=DIRECTION('',(0.,0.,1.));
#13052=DIRECTION('center_axis',(0.,0.,1.));
#13053=DIRECTION('ref_axis',(1.,0.,0.));
#13054=DIRECTION('',(0.,0.,1.));
#13055=DIRECTION('center_axis',(0.,0.,1.));
#13056=DIRECTION('ref_axis',(1.,0.,0.));
#13057=DIRECTION('',(0.,0.,1.));
#13058=DIRECTION('center_axis',(0.,0.,1.));
#13059=DIRECTION('ref_axis',(1.,0.,0.));
#13060=DIRECTION('',(0.,0.,1.));
#13061=DIRECTION('center_axis',(0.,0.,1.));
#13062=DIRECTION('ref_axis',(1.,0.,0.));
#13063=DIRECTION('',(0.,0.,1.));
#13064=DIRECTION('center_axis',(0.,0.,1.));
#13065=DIRECTION('ref_axis',(1.,0.,0.));
#13066=DIRECTION('',(0.,0.,1.));
#13067=DIRECTION('center_axis',(0.,0.,1.));
#13068=DIRECTION('ref_axis',(1.,0.,0.));
#13069=DIRECTION('',(0.,0.,1.));
#13070=DIRECTION('center_axis',(0.,0.,1.));
#13071=DIRECTION('ref_axis',(1.,0.,0.));
#13072=DIRECTION('',(0.,0.,1.));
#13073=DIRECTION('center_axis',(0.,0.,1.));
#13074=DIRECTION('ref_axis',(1.,0.,0.));
#13075=DIRECTION('',(0.,0.,1.));
#13076=DIRECTION('center_axis',(0.,0.,1.));
#13077=DIRECTION('ref_axis',(1.,0.,0.));
#13078=DIRECTION('',(0.,0.,1.));
#13079=DIRECTION('center_axis',(0.,0.,1.));
#13080=DIRECTION('ref_axis',(1.,0.,0.));
#13081=DIRECTION('',(0.,0.,1.));
#13082=DIRECTION('center_axis',(0.,0.,1.));
#13083=DIRECTION('ref_axis',(1.,0.,0.));
#13084=DIRECTION('',(0.,0.,1.));
#13085=DIRECTION('center_axis',(0.,0.,1.));
#13086=DIRECTION('ref_axis',(1.,0.,0.));
#13087=DIRECTION('',(0.,0.,1.));
#13088=DIRECTION('center_axis',(0.,0.,1.));
#13089=DIRECTION('ref_axis',(1.,0.,0.));
#13090=DIRECTION('',(0.,0.,1.));
#13091=DIRECTION('center_axis',(0.,0.,1.));
#13092=DIRECTION('ref_axis',(1.,0.,0.));
#13093=DIRECTION('',(0.,0.,1.));
#13094=DIRECTION('center_axis',(0.,0.,-1.));
#13095=DIRECTION('ref_axis',(-1.14926154660527E-15,1.,0.));
#13096=DIRECTION('',(0.,0.,1.));
#13097=DIRECTION('center_axis',(0.,0.,1.));
#13098=DIRECTION('ref_axis',(-1.14926154660527E-15,1.,0.));
#13099=DIRECTION('center_axis',(0.,0.,-1.));
#13100=DIRECTION('ref_axis',(-1.14926154660527E-15,1.,0.));
#13101=DIRECTION('',(0.,0.,1.));
#13102=DIRECTION('center_axis',(0.,0.,1.));
#13103=DIRECTION('ref_axis',(-1.14926154660527E-15,1.,0.));
#13104=DIRECTION('center_axis',(0.,0.,-1.));
#13105=DIRECTION('ref_axis',(-1.14926154660527E-15,1.,0.));
#13106=DIRECTION('',(0.,0.,1.));
#13107=DIRECTION('center_axis',(0.,0.,-1.));
#13108=DIRECTION('ref_axis',(-1.14926154660527E-15,1.,0.));
#13109=DIRECTION('',(0.,0.,1.));
#13110=DIRECTION('center_axis',(0.,0.,-1.));
#13111=DIRECTION('ref_axis',(-1.14926154660527E-15,1.,0.));
#13112=DIRECTION('',(0.,0.,1.));
#13113=DIRECTION('center_axis',(0.,0.,-1.));
#13114=DIRECTION('ref_axis',(-1.14926154660527E-15,1.,0.));
#13115=DIRECTION('',(0.,0.,1.));
#13116=DIRECTION('center_axis',(0.,0.,-1.));
#13117=DIRECTION('ref_axis',(-1.14926154660527E-15,1.,0.));
#13118=DIRECTION('',(0.,0.,1.));
#13119=DIRECTION('',(0.,0.,-1.));
#13120=DIRECTION('center_axis',(0.,0.,-1.));
#13121=DIRECTION('ref_axis',(1.,8.04483082623694E-15,0.));
#13122=DIRECTION('',(0.,0.,1.));
#13123=DIRECTION('center_axis',(0.,0.,1.));
#13124=DIRECTION('ref_axis',(1.,8.04483082623694E-15,0.));
#13125=DIRECTION('center_axis',(0.,0.,-1.));
#13126=DIRECTION('ref_axis',(1.,8.04483082623694E-15,0.));
#13127=DIRECTION('',(0.,0.,1.));
#13128=DIRECTION('center_axis',(0.,0.,1.));
#13129=DIRECTION('ref_axis',(1.,8.04483082623694E-15,0.));
#13130=DIRECTION('center_axis',(0.,0.,-1.));
#13131=DIRECTION('ref_axis',(1.,8.04483082623694E-15,0.));
#13132=DIRECTION('',(0.,0.,1.));
#13133=DIRECTION('center_axis',(0.,0.,-1.));
#13134=DIRECTION('ref_axis',(1.,8.04483082623694E-15,0.));
#13135=DIRECTION('',(0.,0.,1.));
#13136=DIRECTION('center_axis',(0.,0.,-1.));
#13137=DIRECTION('ref_axis',(1.,8.04483082623694E-15,0.));
#13138=DIRECTION('',(0.,0.,1.));
#13139=DIRECTION('center_axis',(0.,0.,-1.));
#13140=DIRECTION('ref_axis',(1.,8.04483082623694E-15,0.));
#13141=DIRECTION('',(0.,0.,1.));
#13142=DIRECTION('center_axis',(0.,0.,-1.));
#13143=DIRECTION('ref_axis',(1.,8.04483082623694E-15,0.));
#13144=DIRECTION('',(0.,0.,1.));
#13145=DIRECTION('',(0.,0.,-1.));
#13146=DIRECTION('center_axis',(0.,0.,-1.));
#13147=DIRECTION('ref_axis',(1.14926154660527E-15,-1.,0.));
#13148=DIRECTION('',(0.,0.,1.));
#13149=DIRECTION('center_axis',(0.,0.,1.));
#13150=DIRECTION('ref_axis',(1.14926154660527E-15,-1.,0.));
#13151=DIRECTION('center_axis',(0.,0.,-1.));
#13152=DIRECTION('ref_axis',(1.14926154660527E-15,-1.,0.));
#13153=DIRECTION('',(0.,0.,1.));
#13154=DIRECTION('center_axis',(0.,0.,1.));
#13155=DIRECTION('ref_axis',(1.14926154660527E-15,-1.,0.));
#13156=DIRECTION('center_axis',(0.,0.,-1.));
#13157=DIRECTION('ref_axis',(1.14926154660527E-15,-1.,0.));
#13158=DIRECTION('',(0.,0.,1.));
#13159=DIRECTION('center_axis',(0.,0.,-1.));
#13160=DIRECTION('ref_axis',(1.14926154660527E-15,-1.,0.));
#13161=DIRECTION('',(0.,0.,1.));
#13162=DIRECTION('center_axis',(0.,0.,-1.));
#13163=DIRECTION('ref_axis',(1.14926154660527E-15,-1.,0.));
#13164=DIRECTION('',(0.,0.,1.));
#13165=DIRECTION('center_axis',(0.,0.,-1.));
#13166=DIRECTION('ref_axis',(1.14926154660527E-15,-1.,0.));
#13167=DIRECTION('',(0.,0.,1.));
#13168=DIRECTION('center_axis',(0.,0.,-1.));
#13169=DIRECTION('ref_axis',(1.14926154660527E-15,-1.,0.));
#13170=DIRECTION('',(0.,0.,1.));
#13171=DIRECTION('',(0.,0.,-1.));
#13172=DIRECTION('center_axis',(0.,0.,-1.));
#13173=DIRECTION('ref_axis',(-1.,0.,0.));
#13174=DIRECTION('',(0.,0.,1.));
#13175=DIRECTION('center_axis',(0.,0.,1.));
#13176=DIRECTION('ref_axis',(-1.,0.,0.));
#13177=DIRECTION('center_axis',(0.,0.,-1.));
#13178=DIRECTION('ref_axis',(-1.,0.,0.));
#13179=DIRECTION('',(0.,0.,1.));
#13180=DIRECTION('center_axis',(0.,0.,1.));
#13181=DIRECTION('ref_axis',(-1.,0.,0.));
#13182=DIRECTION('center_axis',(0.,0.,-1.));
#13183=DIRECTION('ref_axis',(-1.,0.,0.));
#13184=DIRECTION('',(0.,0.,1.));
#13185=DIRECTION('center_axis',(0.,0.,-1.));
#13186=DIRECTION('ref_axis',(-1.,0.,0.));
#13187=DIRECTION('',(0.,0.,1.));
#13188=DIRECTION('center_axis',(0.,0.,-1.));
#13189=DIRECTION('ref_axis',(-1.,0.,0.));
#13190=DIRECTION('',(0.,0.,1.));
#13191=DIRECTION('center_axis',(0.,0.,-1.));
#13192=DIRECTION('ref_axis',(-1.,0.,0.));
#13193=DIRECTION('',(0.,0.,1.));
#13194=DIRECTION('center_axis',(0.,0.,-1.));
#13195=DIRECTION('ref_axis',(-1.,0.,0.));
#13196=DIRECTION('',(0.,0.,1.));
#13197=DIRECTION('',(0.,0.,-1.));
#13198=DIRECTION('center_axis',(0.,0.,-1.));
#13199=DIRECTION('ref_axis',(-1.,0.,0.));
#13200=DIRECTION('center_axis',(0.,0.,-1.));
#13201=DIRECTION('ref_axis',(1.14926154660527E-15,-1.,0.));
#13202=DIRECTION('center_axis',(0.,0.,-1.));
#13203=DIRECTION('ref_axis',(1.,8.04483082623694E-15,0.));
#13204=DIRECTION('center_axis',(0.,0.,-1.));
#13205=DIRECTION('ref_axis',(-1.14926154660527E-15,1.,0.));
#13206=DIRECTION('center_axis',(0.,0.,1.));
#13207=DIRECTION('ref_axis',(1.,0.,0.));
#13208=DIRECTION('center_axis',(0.,0.,1.));
#13209=DIRECTION('ref_axis',(-1.,-5.46369598732852E-15,0.));
#13210=DIRECTION('center_axis',(0.,0.,1.));
#13211=DIRECTION('ref_axis',(1.,0.,0.));
#13212=DIRECTION('center_axis',(0.,0.,1.));
#13213=DIRECTION('ref_axis',(-1.,-3.64246399155235E-15,0.));
#13214=DIRECTION('center_axis',(0.,0.,1.));
#13215=DIRECTION('ref_axis',(1.,0.,0.));
#13216=DIRECTION('center_axis',(0.,0.,1.));
#13217=DIRECTION('ref_axis',(-1.,1.82123199577617E-15,0.));
#13218=DIRECTION('center_axis',(0.,0.,1.));
#13219=DIRECTION('ref_axis',(1.,0.,0.));
#13220=DIRECTION('center_axis',(0.,0.,1.));
#13221=DIRECTION('ref_axis',(-1.,-9.10615997888087E-16,0.));
#13222=DIRECTION('center_axis',(0.,0.,1.));
#13223=DIRECTION('ref_axis',(1.,0.,0.));
#13224=DIRECTION('center_axis',(0.,0.,1.));
#13225=DIRECTION('ref_axis',(-1.,0.,0.));
#13226=DIRECTION('',(0.,0.,1.));
#13227=DIRECTION('center_axis',(0.,0.,-1.));
#13228=DIRECTION('ref_axis',(1.,0.,0.));
#13229=DIRECTION('center_axis',(0.,0.,1.));
#13230=DIRECTION('ref_axis',(1.,0.,0.));
#13231=DIRECTION('center_axis',(0.,0.,1.));
#13232=DIRECTION('ref_axis',(1.,0.,0.));
#13233=DIRECTION('',(0.,0.,1.));
#13234=DIRECTION('center_axis',(0.,0.,1.));
#13235=DIRECTION('ref_axis',(1.,0.,0.));
#13236=DIRECTION('center_axis',(0.,0.,-1.));
#13237=DIRECTION('ref_axis',(-1.,0.,0.));
#13238=DIRECTION('center_axis',(0.,0.,-1.));
#13239=DIRECTION('ref_axis',(-1.,0.,0.));
#13240=DIRECTION('',(-0.707106781186555,8.65956056235503E-17,0.70710678118654));
#13241=DIRECTION('center_axis',(0.,0.,1.));
#13242=DIRECTION('ref_axis',(-1.,0.,0.));
#13243=DIRECTION('center_axis',(0.,0.,-1.));
#13244=DIRECTION('ref_axis',(-1.,0.,0.));
#13245=DIRECTION('',(0.,0.,1.));
#13246=DIRECTION('center_axis',(0.,0.,1.));
#13247=DIRECTION('ref_axis',(1.,0.,0.));
#13248=DIRECTION('center_axis',(4.16203559120935E-32,4.16203559120936E-32,
1.));
#13249=DIRECTION('ref_axis',(-3.21990436376205E-15,1.,-4.16203559120935E-32));
#13250=DIRECTION('center_axis',(9.19047099336175E-15,3.40905954562136E-15,
1.));
#13251=DIRECTION('ref_axis',(0.596254243270102,0.802795663529891,-8.21663554738274E-15));
#13252=DIRECTION('',(2.36341181601185E-15,-0.707106781186549,0.707106781186546));
#13253=DIRECTION('center_axis',(0.,0.,-1.));
#13254=DIRECTION('ref_axis',(-1.,0.,0.));
#13255=DIRECTION('center_axis',(0.,8.3240711824187E-32,1.));
#13256=DIRECTION('ref_axis',(-1.,0.,0.));
#13257=DIRECTION('center_axis',(0.,0.,1.));
#13258=DIRECTION('ref_axis',(-0.802795663529893,0.5962542432701,0.));
#13259=DIRECTION('',(0.707106781186549,8.65956056235496E-17,0.707106781186546));
#13260=DIRECTION('center_axis',(0.,0.,-1.));
#13261=DIRECTION('ref_axis',(-1.,0.,0.));
#13262=DIRECTION('center_axis',(-4.16203559120935E-32,4.16203559120931E-32,
1.));
#13263=DIRECTION('ref_axis',(1.04646891822267E-14,-1.,4.16203559120935E-32));
#13264=DIRECTION('center_axis',(9.19047099336175E-15,3.40905954562148E-15,
1.));
#13265=DIRECTION('ref_axis',(-0.596254243270094,-0.802795663529897,8.21663554738278E-15));
#13266=DIRECTION('',(-7.48624828938557E-15,0.707106781186549,0.707106781186546));
#13267=DIRECTION('center_axis',(0.,0.,-1.));
#13268=DIRECTION('ref_axis',(-1.,0.,0.));
#13269=DIRECTION('center_axis',(0.,0.,1.));
#13270=DIRECTION('ref_axis',(1.,0.,0.));
#13271=DIRECTION('center_axis',(0.,0.,1.));
#13272=DIRECTION('ref_axis',(0.802795663529893,-0.5962542432701,0.));
#13273=DIRECTION('',(-0.707106781186549,-8.65956056235495E-17,0.707106781186546));
#13274=DIRECTION('center_axis',(0.,0.,-1.));
#13275=DIRECTION('ref_axis',(-1.,0.,0.));
#13276=DIRECTION('center_axis',(2.88512032359387E-6,-9.62952063919659E-7,
-0.999999999995374));
#13277=DIRECTION('ref_axis',(-0.910167431629583,0.414240565845088,-3.02483636272151E-6));
#13278=DIRECTION('',(0.509030150079891,0.700633705437601,0.500000717113906));
#13279=DIRECTION('center_axis',(-5.73319914530485E-6,1.03122865517202E-5,
-0.999999999930394));
#13280=DIRECTION('ref_axis',(-0.400826900807492,0.916153805564928,1.17456610143768E-5));
#13281=DIRECTION('',(-0.509034825310574,-0.700630697427327,0.500000172443501));
#13282=DIRECTION('center_axis',(-0.809020620080864,0.587780261877828,-5.55040215556246E-6));
#13283=DIRECTION('ref_axis',(-0.587780261886882,-0.809020620093325,3.00207577931475E-21));
#13284=DIRECTION('',(-4.49056928125163E-6,3.26216978819017E-6,0.999999999984597));
#13285=DIRECTION('center_axis',(0.,0.,1.));
#13286=DIRECTION('ref_axis',(1.,0.,0.));
#13287=DIRECTION('',(-1.,1.63653158111019E-16,0.));
#13288=DIRECTION('',(-0.707106781186551,0.707106781186544,0.));
#13289=DIRECTION('',(3.27306316222039E-16,1.,0.));
#13290=DIRECTION('',(0.707106781186551,0.707106781186544,0.));
#13291=DIRECTION('',(-1.,-1.63653158111019E-16,0.));
#13292=DIRECTION('',(0.707106781186551,-0.707106781186544,0.));
#13293=DIRECTION('',(0.,-1.,0.));
#13294=DIRECTION('',(-0.707106781186551,-0.707106781186544,0.));
#13295=DIRECTION('center_axis',(9.62952046063973E-7,2.88512025876916E-6,
-0.999999999995374));
#13296=DIRECTION('ref_axis',(-0.414240565845042,-0.910167431629604,-3.02483629632364E-6));
#13297=DIRECTION('center_axis',(-1.03122864674752E-5,-5.73319909310356E-6,
-0.999999999930394));
#13298=DIRECTION('ref_axis',(-0.916153805570372,-0.40082690079505,1.17456609162565E-5));
#13299=DIRECTION('center_axis',(-2.88512008141766E-6,9.62951976338086E-7,
-0.999999999995374));
#13300=DIRECTION('ref_axis',(0.910167431629613,-0.414240565845021,-3.0248361060208E-6));
#13301=DIRECTION('center_axis',(5.73319910393675E-6,-1.03122864820549E-5,
-0.999999999930394));
#13302=DIRECTION('ref_axis',(0.400826900807403,-0.916153805564967,1.17456609339711E-5));
#13303=DIRECTION('center_axis',(-9.62952042711932E-7,-2.88512027353277E-6,
-0.999999999995374));
#13304=DIRECTION('ref_axis',(0.41424056584503,0.910167431629609,-3.02483630837245E-6));
#13305=DIRECTION('center_axis',(1.0312286495339E-5,5.73319911396724E-6,
-0.999999999930394));
#13306=DIRECTION('ref_axis',(0.916153805564476,0.400826900808526,1.17456609501632E-5));
#13307=DIRECTION('',(0.700633705437605,-0.509030150079883,0.500000717113908));
#13308=DIRECTION('',(-0.700630697427374,0.509034825310594,0.500000172443415));
#13309=DIRECTION('center_axis',(0.58778026187782,0.80902062008087,-5.55040215556246E-6));
#13310=DIRECTION('ref_axis',(-0.809020620093331,0.587780261886873,-9.35224649526989E-22));
#13311=DIRECTION('',(3.26216982371735E-6,4.49056924572438E-6,0.999999999984597));
#13312=DIRECTION('',(-0.509030150079891,-0.700633705437601,0.500000717113906));
#13313=DIRECTION('',(0.509034825310574,0.700630697427327,0.500000172443501));
#13314=DIRECTION('center_axis',(0.809020620080864,-0.587780261877828,-5.55040215556246E-6));
#13315=DIRECTION('ref_axis',(0.587780261886882,0.809020620093325,3.00207577931475E-21));
#13316=DIRECTION('',(4.49056928125163E-6,-3.26216978819017E-6,0.999999999984597));
#13317=DIRECTION('',(-0.700633705437603,0.509030150079887,0.500000717113907));
#13318=DIRECTION('',(0.700630697427361,-0.509034825310594,0.500000172443434));
#13319=DIRECTION('center_axis',(-0.587780261877825,-0.809020620080866,-5.55040215556247E-6));
#13320=DIRECTION('ref_axis',(0.809020620093328,-0.587780261886879,3.26781804448781E-21));
#13321=DIRECTION('',(-3.26216982371737E-6,-4.4905692457244E-6,0.999999999984597));
#13322=DIRECTION('center_axis',(0.,0.,1.));
#13323=DIRECTION('ref_axis',(1.,0.,0.));
#13324=DIRECTION('center_axis',(0.,0.,1.));
#13325=DIRECTION('ref_axis',(1.,0.,0.));
#13326=DIRECTION('center_axis',(0.707106781186544,-0.707106781186551,0.));
#13327=DIRECTION('ref_axis',(0.707106781186551,0.707106781186544,0.));
#13328=DIRECTION('',(0.,0.,-1.));
#13329=DIRECTION('',(0.707106781186551,0.707106781186544,0.));
#13330=DIRECTION('',(0.,0.,-1.));
#13331=DIRECTION('center_axis',(1.,1.02283223819387E-16,0.));
#13332=DIRECTION('ref_axis',(-1.02283223819387E-16,1.,0.));
#13333=DIRECTION('',(0.,0.,-1.));
#13334=DIRECTION('',(-1.02283223819387E-16,1.,0.));
#13335=DIRECTION('center_axis',(-0.707106781186551,-0.707106781186544,0.));
#13336=DIRECTION('ref_axis',(0.707106781186544,-0.707106781186551,0.));
#13337=DIRECTION('center_axis',(0.382683432365102,0.923879532511282,1.23463181525019E-15));
#13338=DIRECTION('ref_axis',(0.923879532511282,-0.382683432365102,-1.12630623213688E-12));
#13339=DIRECTION('',(-0.707106781186551,-0.707106781186544,0.));
#13340=DIRECTION('center_axis',(0.923879532511286,0.382683432365093,-1.27204490056077E-15));
#13341=DIRECTION('ref_axis',(0.382683432365093,-0.923879532511286,2.44180953280602E-12));
#13342=DIRECTION('center_axis',(0.,-1.,0.));
#13343=DIRECTION('ref_axis',(0.,0.,-1.));
#13344=DIRECTION('',(1.,0.,0.));
#13345=DIRECTION('',(0.,0.,-1.));
#13346=DIRECTION('center_axis',(0.707106781186544,0.707106781186551,0.));
#13347=DIRECTION('ref_axis',(-0.707106781186551,0.707106781186544,0.));
#13348=DIRECTION('',(0.,0.,-1.));
#13349=DIRECTION('',(-0.707106781186551,0.707106781186544,0.));
#13350=DIRECTION('center_axis',(1.02283223819387E-16,-1.,0.));
#13351=DIRECTION('ref_axis',(1.,1.02283223819387E-16,0.));
#13352=DIRECTION('center_axis',(-0.382683432365102,0.923879532511282,-4.48957023727334E-16));
#13353=DIRECTION('ref_axis',(0.923879532511282,0.382683432365102,2.16580847215386E-12));
#13354=DIRECTION('',(1.02283223819387E-16,-1.,0.));
#13355=DIRECTION('center_axis',(-2.04566447638774E-16,1.,0.));
#13356=DIRECTION('ref_axis',(-1.,-2.04566447638774E-16,0.));
#13357=DIRECTION('',(0.,0.,-1.));
#13358=DIRECTION('',(-1.,-2.04566447638774E-16,0.));
#13359=DIRECTION('center_axis',(0.707106781186551,-0.707106781186544,0.));
#13360=DIRECTION('ref_axis',(0.707106781186544,0.707106781186551,0.));
#13361=DIRECTION('center_axis',(0.923879532511285,-0.382683432365095,4.56439640789447E-15));
#13362=DIRECTION('ref_axis',(0.382683432365095,0.923879532511285,-1.55608578712059E-12));
#13363=DIRECTION('',(0.707106781186551,-0.707106781186544,0.));
#13364=DIRECTION('center_axis',(-0.707106781186544,0.707106781186551,0.));
#13365=DIRECTION('ref_axis',(-0.707106781186551,-0.707106781186544,0.));
#13366=DIRECTION('',(0.,0.,-1.));
#13367=DIRECTION('',(-0.707106781186551,-0.707106781186544,0.));
#13368=DIRECTION('center_axis',(1.,2.04566447638774E-16,0.));
#13369=DIRECTION('ref_axis',(-2.04566447638774E-16,1.,0.));
#13370=DIRECTION('center_axis',(0.923879532511291,0.382683432365081,1.79582809490932E-14));
#13371=DIRECTION('ref_axis',(0.382683432365081,-0.92387953251129,-4.11849825226955E-13));
#13372=DIRECTION('',(1.,2.04566447638774E-16,0.));
#13373=DIRECTION('center_axis',(-1.,0.,0.));
#13374=DIRECTION('ref_axis',(0.,0.,1.));
#13375=DIRECTION('',(0.,0.,-1.));
#13376=DIRECTION('',(0.,-1.,0.));
#13377=DIRECTION('center_axis',(0.707106781186551,0.707106781186544,0.));
#13378=DIRECTION('ref_axis',(-0.707106781186544,0.707106781186551,0.));
#13379=DIRECTION('center_axis',(0.382683432365092,0.923879532511286,-1.31694060293351E-14));
#13380=DIRECTION('ref_axis',(0.923879532511286,-0.382683432365092,-1.05940768985082E-12));
#13381=DIRECTION('',(0.707106781186551,0.707106781186544,0.));
#13382=DIRECTION('center_axis',(-0.707106781186544,-0.707106781186551,0.));
#13383=DIRECTION('ref_axis',(0.707106781186551,-0.707106781186544,0.));
#13384=DIRECTION('',(0.707106781186551,-0.707106781186544,0.));
#13385=DIRECTION('center_axis',(0.,1.,0.));
#13386=DIRECTION('ref_axis',(0.,0.,1.));
#13387=DIRECTION('center_axis',(-0.382683432365094,0.923879532511285,8.45535728019809E-15));
#13388=DIRECTION('ref_axis',(0.923879532511285,0.382683432365094,-2.63399123634393E-12));
#13389=DIRECTION('',(0.,1.,0.));
#13390=DIRECTION('center_axis',(-0.707106781186551,0.707106781186544,0.));
#13391=DIRECTION('ref_axis',(-0.707106781186544,-0.707106781186551,0.));
#13392=DIRECTION('center_axis',(0.923879532511292,-0.382683432365078,1.6162452854184E-14));
#13393=DIRECTION('ref_axis',(0.382683432365078,0.923879532511292,-1.85973161387526E-12));
#13394=DIRECTION('',(-0.707106781186551,0.707106781186544,0.));
#13395=DIRECTION('center_axis',(-1.,0.,0.));
#13396=DIRECTION('ref_axis',(0.,0.,1.));
#13397=DIRECTION('',(-1.,0.,0.));
#13398=DIRECTION('center_axis',(0.,0.,-1.));
#13399=DIRECTION('ref_axis',(-1.,0.,0.));
#13400=DIRECTION('center_axis',(0.,0.,-1.));
#13401=DIRECTION('ref_axis',(-1.,0.,0.));
#13402=DIRECTION('',(-0.707106781186547,8.65956056235493E-17,0.707106781186548));
#13403=DIRECTION('center_axis',(0.,0.,-1.));
#13404=DIRECTION('ref_axis',(1.,-8.88178419700125E-16,0.));
#13405=DIRECTION('center_axis',(0.,0.,1.));
#13406=DIRECTION('ref_axis',(1.,0.,0.));
#13407=DIRECTION('center_axis',(0.,0.,-1.));
#13408=DIRECTION('ref_axis',(-1.,0.,0.));
#13409=DIRECTION('center_axis',(0.,0.,1.));
#13410=DIRECTION('ref_axis',(1.,0.,0.));
#13411=DIRECTION('center_axis',(0.,0.,-1.));
#13412=DIRECTION('ref_axis',(1.,-8.88178419700125E-16,0.));
#13413=DIRECTION('center_axis',(0.,0.,1.));
#13414=DIRECTION('ref_axis',(1.,0.,0.));
#13415=DIRECTION('',(-0.707106781186549,-8.65956056235495E-17,0.707106781186546));
#13416=DIRECTION('center_axis',(0.,0.,1.));
#13417=DIRECTION('ref_axis',(1.,0.,0.));
#13418=DIRECTION('center_axis',(0.,0.,-1.));
#13419=DIRECTION('ref_axis',(-1.,0.,0.));
#13420=DIRECTION('center_axis',(0.,0.,1.));
#13421=DIRECTION('ref_axis',(-1.,0.,0.));
#13422=DIRECTION('',(0.,0.,1.));
#13423=DIRECTION('',(0.,0.,-1.));
#13424=DIRECTION('center_axis',(0.,0.,-1.));
#13425=DIRECTION('ref_axis',(-1.,0.,0.));
#13426=DIRECTION('',(0.,0.,1.));
#13427=DIRECTION('center_axis',(0.,0.,1.));
#13428=DIRECTION('ref_axis',(1.,0.,0.));
#13429=DIRECTION('center_axis',(0.,0.,-1.));
#13430=DIRECTION('ref_axis',(-1.,0.,0.));
#13431=DIRECTION('center_axis',(0.,0.,-1.));
#13432=DIRECTION('ref_axis',(-1.,0.,0.));
#13433=DIRECTION('',(1.,0.,0.));
#13434=DIRECTION('center_axis',(0.,-1.,0.));
#13435=DIRECTION('ref_axis',(0.,0.,-1.));
#13436=DIRECTION('center_axis',(0.,0.,-1.));
#13437=DIRECTION('ref_axis',(-1.,0.,0.));
#13438=DIRECTION('center_axis',(0.,0.,-1.));
#13439=DIRECTION('ref_axis',(-1.,0.,0.));
#13440=DIRECTION('',(0.,0.,-1.));
#13441=DIRECTION('center_axis',(0.,0.,-1.));
#13442=DIRECTION('ref_axis',(-1.,0.,0.));
#13443=DIRECTION('center_axis',(0.,0.,-1.));
#13444=DIRECTION('ref_axis',(-1.,0.,0.));
#13445=DIRECTION('center_axis',(0.,0.,-1.));
#13446=DIRECTION('ref_axis',(-1.,0.,0.));
#13447=DIRECTION('',(0.707106781186532,-8.65956056235475E-17,-0.707106781186563));
#13448=DIRECTION('center_axis',(0.,0.,1.));
#13449=DIRECTION('ref_axis',(-1.,0.,0.));
#13450=DIRECTION('center_axis',(0.,0.,-1.));
#13451=DIRECTION('ref_axis',(-1.,0.,0.));
#13452=DIRECTION('center_axis',(0.,0.,-1.));
#13453=DIRECTION('ref_axis',(-1.,0.,0.));
#13454=DIRECTION('',(0.707106781186532,-8.65956056235475E-17,-0.707106781186563));
#13455=DIRECTION('center_axis',(0.,0.,1.));
#13456=DIRECTION('ref_axis',(-1.,0.,0.));
#13457=DIRECTION('center_axis',(0.,0.,-1.));
#13458=DIRECTION('ref_axis',(-1.,0.,0.));
#13459=DIRECTION('center_axis',(0.,0.,-1.));
#13460=DIRECTION('ref_axis',(-1.,0.,0.));
#13461=DIRECTION('',(0.707106781186532,-8.65956056235475E-17,-0.707106781186563));
#13462=DIRECTION('center_axis',(0.,0.,1.));
#13463=DIRECTION('ref_axis',(-1.,0.,0.));
#13464=DIRECTION('center_axis',(0.,0.,-1.));
#13465=DIRECTION('ref_axis',(-1.,0.,0.));
#13466=DIRECTION('center_axis',(0.,0.,-1.));
#13467=DIRECTION('ref_axis',(-1.,0.,0.));
#13468=DIRECTION('',(0.707106781186532,-8.65956056235475E-17,-0.707106781186563));
#13469=DIRECTION('center_axis',(0.,0.,1.));
#13470=DIRECTION('ref_axis',(-1.,0.,0.));
#13471=DIRECTION('center_axis',(0.,0.,-1.));
#13472=DIRECTION('ref_axis',(-1.,0.,0.));
#13473=DIRECTION('center_axis',(0.,0.,-1.));
#13474=DIRECTION('ref_axis',(-1.,0.,0.));
#13475=DIRECTION('',(0.,0.,-1.));
#13476=DIRECTION('center_axis',(0.,0.,-1.));
#13477=DIRECTION('ref_axis',(-1.,0.,0.));
#13478=DIRECTION('center_axis',(0.,0.,-1.));
#13479=DIRECTION('ref_axis',(-1.,0.,0.));
#13480=DIRECTION('',(0.,0.,-1.));
#13481=DIRECTION('center_axis',(0.,0.,-1.));
#13482=DIRECTION('ref_axis',(-1.,0.,0.));
#13483=DIRECTION('center_axis',(0.,0.,-1.));
#13484=DIRECTION('ref_axis',(-1.,0.,0.));
#13485=DIRECTION('',(0.,0.,-1.));
#13486=DIRECTION('center_axis',(0.,0.,-1.));
#13487=DIRECTION('ref_axis',(-1.,0.,0.));
#13488=DIRECTION('center_axis',(0.,0.,-1.));
#13489=DIRECTION('ref_axis',(-1.,0.,0.));
#13490=DIRECTION('',(0.,0.,-1.));
#13491=DIRECTION('center_axis',(0.,0.,1.));
#13492=DIRECTION('ref_axis',(1.,0.,0.));
#13493=DIRECTION('center_axis',(0.,0.,1.));
#13494=DIRECTION('ref_axis',(-1.,0.,0.));
#13495=DIRECTION('',(0.,0.,1.));
#13496=DIRECTION('center_axis',(0.,0.,-1.));
#13497=DIRECTION('ref_axis',(1.,0.,0.));
#13498=DIRECTION('center_axis',(0.,0.,-1.));
#13499=DIRECTION('ref_axis',(-1.,0.,0.));
#13500=DIRECTION('center_axis',(0.,0.,-1.));
#13501=DIRECTION('ref_axis',(-1.,0.,0.));
#13502=DIRECTION('center_axis',(0.,0.,-1.));
#13503=DIRECTION('ref_axis',(-1.,0.,0.));
#13504=DIRECTION('center_axis',(0.,0.,-1.));
#13505=DIRECTION('ref_axis',(-1.,0.,0.));
#13506=DIRECTION('center_axis',(0.,1.,0.));
#13507=DIRECTION('ref_axis',(0.,0.,1.));
#13508=DIRECTION('',(1.,0.,0.));
#13509=DIRECTION('',(0.,0.,-1.));
#13510=DIRECTION('',(-1.,0.,0.));
#13511=DIRECTION('',(2.64713952874444E-16,0.,1.));
#13512=DIRECTION('center_axis',(0.,0.,-1.));
#13513=DIRECTION('ref_axis',(-1.,0.,0.));
#13514=DIRECTION('',(-1.,0.,0.));
#13515=DIRECTION('',(0.,1.,0.));
#13516=DIRECTION('',(0.,1.,0.));
#13517=DIRECTION('center_axis',(-1.,0.,2.64713952874444E-16));
#13518=DIRECTION('ref_axis',(2.64713952874444E-16,0.,1.));
#13519=DIRECTION('',(2.64713952874444E-16,0.,1.));
#13520=DIRECTION('',(0.,1.,0.));
#13521=DIRECTION('center_axis',(0.,0.,1.));
#13522=DIRECTION('ref_axis',(1.,0.,0.));
#13523=DIRECTION('',(1.,0.,0.));
#13524=DIRECTION('',(0.,1.,0.));
#13525=DIRECTION('center_axis',(1.,0.,0.));
#13526=DIRECTION('ref_axis',(0.,0.,-1.));
#13527=DIRECTION('',(0.,0.,-1.));
#13528=DIRECTION('center_axis',(0.,-1.,0.));
#13529=DIRECTION('ref_axis',(0.,0.,-1.));
#13530=DIRECTION('',(0.,0.,-1.));
#13531=DIRECTION('',(-1.,0.,0.));
#13532=DIRECTION('',(1.90771507937448E-16,0.,1.));
#13533=DIRECTION('',(1.,0.,0.));
#13534=DIRECTION('center_axis',(0.,0.,1.));
#13535=DIRECTION('ref_axis',(1.,0.,0.));
#13536=DIRECTION('',(0.,-1.,0.));
#13537=DIRECTION('',(-1.,0.,0.));
#13538=DIRECTION('',(0.,-1.,0.));
#13539=DIRECTION('center_axis',(0.,0.,-1.));
#13540=DIRECTION('ref_axis',(-1.,0.,0.));
#13541=DIRECTION('',(-1.,-2.04566447638774E-16,0.));
#13542=DIRECTION('',(-0.707106781186551,0.707106781186544,0.));
#13543=DIRECTION('',(-1.02283223819387E-16,1.,0.));
#13544=DIRECTION('',(0.707106781186551,0.707106781186544,0.));
#13545=DIRECTION('',(1.,0.,0.));
#13546=DIRECTION('',(0.707106781186551,-0.707106781186544,0.));
#13547=DIRECTION('',(0.,-1.,0.));
#13548=DIRECTION('',(-0.707106781186551,-0.707106781186544,0.));
#13549=DIRECTION('center_axis',(0.707106781186551,0.707106781186544,0.));
#13550=DIRECTION('ref_axis',(-0.707106781186544,0.707106781186551,0.));
#13551=DIRECTION('center_axis',(-0.923879532511288,-0.382683432365087,-4.48957023727335E-16));
#13552=DIRECTION('ref_axis',(0.382683432365087,-0.923879532511288,-3.69328470883498E-12));
#13553=DIRECTION('center_axis',(-0.382683432365071,-0.923879532511295,2.72741391914358E-14));
#13554=DIRECTION('ref_axis',(0.923879532511295,-0.382683432365071,-5.58285843927778E-12));
#13555=DIRECTION('',(-0.707106781186551,-0.707106781186544,0.));
#13556=DIRECTION('center_axis',(-1.02283223819387E-16,1.,0.));
#13557=DIRECTION('ref_axis',(-1.,-1.02283223819387E-16,0.));
#13558=DIRECTION('center_axis',(0.382683432365102,-0.923879532511282,-4.48957023727337E-16));
#13559=DIRECTION('ref_axis',(0.923879532511282,0.382683432365102,-3.82113308819835E-12));
#13560=DIRECTION('',(1.02283223819387E-16,-1.,0.));
#13561=DIRECTION('center_axis',(-0.707106781186551,0.707106781186544,0.));
#13562=DIRECTION('ref_axis',(-0.707106781186544,-0.707106781186551,0.));
#13563=DIRECTION('center_axis',(-0.923879532511285,0.382683432365094,2.39443745987918E-15));
#13564=DIRECTION('ref_axis',(0.382683432365094,0.923879532511285,-7.29302575246149E-12));
#13565=DIRECTION('',(0.707106781186551,-0.707106781186544,0.));
#13566=DIRECTION('center_axis',(1.,1.02283223819387E-16,0.));
#13567=DIRECTION('ref_axis',(-1.02283223819387E-16,1.,0.));
#13568=DIRECTION('',(0.,0.,-1.));
#13569=DIRECTION('',(0.,0.,-1.));
#13570=DIRECTION('',(0.,-1.,0.));
#13571=DIRECTION('center_axis',(-1.,-2.04566447638774E-16,0.));
#13572=DIRECTION('ref_axis',(2.04566447638774E-16,-1.,0.));
#13573=DIRECTION('center_axis',(-0.923879532511293,-0.382683432365076,1.27204490056078E-14));
#13574=DIRECTION('ref_axis',(0.382683432365076,-0.923879532511293,1.41474115456993E-12));
#13575=DIRECTION('',(1.,2.04566447638774E-16,0.));
#13576=DIRECTION('center_axis',(0.707106781186544,0.707106781186551,0.));
#13577=DIRECTION('ref_axis',(-0.707106781186551,0.707106781186544,0.));
#13578=DIRECTION('',(0.,0.,-1.));
#13579=DIRECTION('',(0.707106781186551,-0.707106781186544,0.));
#13580=DIRECTION('center_axis',(-0.707106781186551,-0.707106781186544,0.));
#13581=DIRECTION('ref_axis',(0.707106781186544,-0.707106781186551,0.));
#13582=DIRECTION('center_axis',(-0.382683432365091,-0.923879532511286,-5.83644130845536E-15));
#13583=DIRECTION('ref_axis',(0.923879532511286,-0.382683432365091,1.78782837061874E-12));
#13584=DIRECTION('',(0.707106781186551,0.707106781186544,0.));
#13585=DIRECTION('center_axis',(-2.04566447638774E-16,1.,0.));
#13586=DIRECTION('ref_axis',(-1.,-2.04566447638774E-16,0.));
#13587=DIRECTION('',(0.,0.,-1.));
#13588=DIRECTION('',(-1.,-1.63653158111019E-16,0.));
#13589=DIRECTION('center_axis',(0.,-1.,0.));
#13590=DIRECTION('ref_axis',(0.,0.,-1.));
#13591=DIRECTION('center_axis',(0.382683432365094,-0.923879532511285,8.45535728019803E-15));
#13592=DIRECTION('ref_axis',(0.923879532511285,0.382683432365094,-1.28017687415757E-12));
#13593=DIRECTION('',(0.,1.,0.));
#13594=DIRECTION('center_axis',(-0.707106781186544,0.707106781186551,0.));
#13595=DIRECTION('ref_axis',(-0.707106781186551,-0.707106781186544,0.));
#13596=DIRECTION('',(0.,0.,-1.));
#13597=DIRECTION('',(0.707106781186551,0.707106781186544,0.));
#13598=DIRECTION('center_axis',(0.707106781186551,-0.707106781186544,0.));
#13599=DIRECTION('ref_axis',(0.707106781186544,0.707106781186551,0.));
#13600=DIRECTION('center_axis',(-0.923879532511291,0.382683432365079,1.50400602948654E-14));
#13601=DIRECTION('ref_axis',(0.382683432365079,0.923879532511291,-1.73217448820192E-12));
#13602=DIRECTION('',(-0.707106781186551,0.707106781186544,0.));
#13603=DIRECTION('center_axis',(-1.,0.,0.));
#13604=DIRECTION('ref_axis',(0.,0.,1.));
#13605=DIRECTION('',(0.,0.,-1.));
#13606=DIRECTION('',(3.27306316222039E-16,1.,0.));
#13607=DIRECTION('center_axis',(0.707106781186544,-0.707106781186551,0.));
#13608=DIRECTION('ref_axis',(0.707106781186551,0.707106781186544,0.));
#13609=DIRECTION('',(0.,0.,-1.));
#13610=DIRECTION('',(-0.707106781186551,-0.707106781186544,0.));
#13611=DIRECTION('center_axis',(1.,0.,-1.90771507937448E-16));
#13612=DIRECTION('ref_axis',(-1.90771507937448E-16,0.,-1.));
#13613=DIRECTION('center_axis',(1.,0.,-1.90771507937448E-16));
#13614=DIRECTION('ref_axis',(-1.90771507937448E-16,0.,-1.));
#13615=DIRECTION('',(1.90771507937448E-16,0.,1.));
#13616=DIRECTION('',(0.,-1.,0.));
#13617=DIRECTION('center_axis',(0.,0.,-1.));
#13618=DIRECTION('ref_axis',(-1.,0.,0.));
#13619=DIRECTION('',(1.,0.,0.));
#13620=DIRECTION('',(0.,-1.,0.));
#13621=DIRECTION('center_axis',(-1.,0.,0.));
#13622=DIRECTION('ref_axis',(0.,0.,1.));
#13623=DIRECTION('',(0.,0.,-1.));
#13624=DIRECTION('center_axis',(-1.,0.,0.));
#13625=DIRECTION('ref_axis',(0.,0.,1.));
#13626=DIRECTION('center_axis',(1.,0.,0.));
#13627=DIRECTION('ref_axis',(0.,0.,-1.));
#13628=DIRECTION('',(-1.,0.,0.));
#13629=DIRECTION('',(-1.,0.,0.));
#13630=DIRECTION('center_axis',(-0.707106781186544,-0.707106781186551,0.));
#13631=DIRECTION('ref_axis',(0.707106781186551,-0.707106781186544,0.));
#13632=DIRECTION('',(0.,0.,-1.));
#13633=DIRECTION('',(-0.707106781186551,0.707106781186544,0.));
#13634=DIRECTION('center_axis',(0.,-1.,0.));
#13635=DIRECTION('ref_axis',(0.,0.,-1.));
#13636=DIRECTION('',(-1.,1.63653158111019E-16,0.));
#13637=DIRECTION('center_axis',(0.,0.,1.));
#13638=DIRECTION('ref_axis',(1.,0.,0.));
#13639=DIRECTION('center_axis',(0.,0.,-1.));
#13640=DIRECTION('ref_axis',(-1.,0.,0.));
#13641=DIRECTION('center_axis',(0.,0.,1.));
#13642=DIRECTION('ref_axis',(1.,0.,0.));
#13643=DIRECTION('center_axis',(0.,0.,-1.));
#13644=DIRECTION('ref_axis',(1.,0.,0.));
#13645=DIRECTION('',(0.,0.,1.));
#13646=DIRECTION('center_axis',(0.,0.,1.));
#13647=DIRECTION('ref_axis',(-1.,0.,0.));
#13648=DIRECTION('center_axis',(0.,0.,1.));
#13649=DIRECTION('ref_axis',(1.,0.,0.));
#13650=DIRECTION('center_axis',(0.,0.,1.));
#13651=DIRECTION('ref_axis',(1.,0.,0.));
#13652=DIRECTION('',(0.,0.,1.));
#13653=DIRECTION('center_axis',(0.,0.,1.));
#13654=DIRECTION('ref_axis',(-1.,0.,0.));
#13655=DIRECTION('center_axis',(0.,0.,1.));
#13656=DIRECTION('ref_axis',(1.,0.,0.));
#13657=DIRECTION('center_axis',(0.,0.,1.));
#13658=DIRECTION('ref_axis',(1.,0.,0.));
#13659=DIRECTION('',(0.,0.,1.));
#13660=DIRECTION('center_axis',(0.,0.,1.));
#13661=DIRECTION('ref_axis',(-1.,0.,0.));
#13662=DIRECTION('center_axis',(0.,0.,1.));
#13663=DIRECTION('ref_axis',(1.,0.,0.));
#13664=DIRECTION('center_axis',(0.,0.,1.));
#13665=DIRECTION('ref_axis',(1.,0.,0.));
#13666=DIRECTION('',(0.,0.,1.));
#13667=DIRECTION('center_axis',(0.,0.,1.));
#13668=DIRECTION('ref_axis',(-1.,0.,0.));
#13669=DIRECTION('center_axis',(0.,0.,1.));
#13670=DIRECTION('ref_axis',(1.,0.,0.));
#13671=DIRECTION('center_axis',(0.,0.,1.));
#13672=DIRECTION('ref_axis',(1.,0.,0.));
#13673=DIRECTION('',(0.,0.,1.));
#13674=DIRECTION('center_axis',(0.,0.,1.));
#13675=DIRECTION('ref_axis',(-1.,0.,0.));
#13676=DIRECTION('center_axis',(0.,0.,1.));
#13677=DIRECTION('ref_axis',(1.,0.,0.));
#13678=DIRECTION('',(0.707106781186552,-0.707106781186543,0.));
#13679=DIRECTION('',(-2.38943891978177E-16,-1.,0.));
#13680=DIRECTION('',(0.707106781186551,0.707106781186544,0.));
#13681=DIRECTION('',(1.,0.,0.));
#13682=DIRECTION('',(0.707106781186551,-0.707106781186544,0.));
#13683=DIRECTION('',(-2.38943891978177E-16,1.,0.));
#13684=DIRECTION('',(0.707106781186551,0.707106781186544,0.));
#13685=DIRECTION('',(1.,0.,0.));
#13686=DIRECTION('center_axis',(0.,0.,-1.));
#13687=DIRECTION('ref_axis',(-1.,0.,0.));
#13688=DIRECTION('',(0.707106781186551,-0.707106781186544,0.));
#13689=DIRECTION('',(1.,0.,0.));
#13690=DIRECTION('',(0.707106781186551,0.707106781186544,0.));
#13691=DIRECTION('',(-2.38943891978177E-16,1.,0.));
#13692=DIRECTION('',(0.707106781186551,-0.707106781186544,0.));
#13693=DIRECTION('',(1.,0.,0.));
#13694=DIRECTION('',(0.707106781186552,0.707106781186543,0.));
#13695=DIRECTION('',(-2.38943891978177E-16,-1.,0.));
#13696=DIRECTION('center_axis',(0.,-1.,0.));
#13697=DIRECTION('ref_axis',(0.,0.,-1.));
#13698=DIRECTION('',(0.,0.,1.));
#13699=DIRECTION('',(0.,0.,1.));
#13700=DIRECTION('center_axis',(-0.707106781186544,-0.707106781186551,0.));
#13701=DIRECTION('ref_axis',(0.707106781186551,-0.707106781186544,0.));
#13702=DIRECTION('',(0.,0.,1.));
#13703=DIRECTION('center_axis',(0.707106781186544,-0.707106781186551,0.));
#13704=DIRECTION('ref_axis',(0.707106781186551,0.707106781186544,0.));
#13705=DIRECTION('',(0.,0.,1.));
#13706=DIRECTION('center_axis',(0.707106781186543,-0.707106781186552,0.));
#13707=DIRECTION('ref_axis',(0.707106781186552,0.707106781186543,0.));
#13708=DIRECTION('',(0.,0.,1.));
#13709=DIRECTION('',(0.,0.,1.));
#13710=DIRECTION('center_axis',(-0.707106781186544,-0.707106781186551,0.));
#13711=DIRECTION('ref_axis',(0.707106781186551,-0.707106781186544,0.));
#13712=DIRECTION('',(0.,0.,1.));
#13713=DIRECTION('',(0.,0.,1.));
#13714=DIRECTION('center_axis',(1.,2.38943891978177E-16,0.));
#13715=DIRECTION('ref_axis',(-2.38943891978177E-16,1.,0.));
#13716=DIRECTION('center_axis',(0.,-1.,0.));
#13717=DIRECTION('ref_axis',(0.,0.,-1.));
#13718=DIRECTION('center_axis',(-1.,2.38943891978176E-16,0.));
#13719=DIRECTION('ref_axis',(-2.38943891978176E-16,-1.,0.));
#13720=DIRECTION('center_axis',(0.,0.,1.));
#13721=DIRECTION('ref_axis',(1.,0.,0.));
#13722=DIRECTION('center_axis',(0.,0.,1.));
#13723=DIRECTION('ref_axis',(1.,0.,0.));
#13724=DIRECTION('center_axis',(0.,0.,1.));
#13725=DIRECTION('ref_axis',(1.,0.,0.));
#13726=DIRECTION('center_axis',(0.,0.,1.));
#13727=DIRECTION('ref_axis',(1.,0.,0.));
#15382=CARTESIAN_POINT('',(0.,0.,0.));
#15383=CARTESIAN_POINT('Origin',(15.5,15.5,-45.9992561210692));
#15384=CARTESIAN_POINT('',(12.325,15.5,-33.844));
#15385=CARTESIAN_POINT('Origin',(15.5,15.5,-33.844));
#15386=CARTESIAN_POINT('',(12.325,15.5,-34.479));
#15387=CARTESIAN_POINT('',(12.325,15.5,-45.9992561210692));
#15388=CARTESIAN_POINT('',(18.675,15.5,-34.479));
#15389=CARTESIAN_POINT('Origin',(15.5,15.5,-34.479));
#15390=CARTESIAN_POINT('Origin',(15.5,15.5,-34.479));
#15391=CARTESIAN_POINT('Origin',(15.5,15.5,-34.479));
#15392=CARTESIAN_POINT('',(17.913,15.1825,-35.6336740328739));
#15393=CARTESIAN_POINT('',(17.913,15.5,-35.6429742265188));
#15394=CARTESIAN_POINT('Ctrl Pts',(17.913,15.5,-35.6429742265188));
#15395=CARTESIAN_POINT('Ctrl Pts',(17.913,15.3977178848389,-35.6429742265188));
#15396=CARTESIAN_POINT('Ctrl Pts',(17.913,15.2910620631233,-35.6401598997242));
#15397=CARTESIAN_POINT('Ctrl Pts',(17.913,15.1824999999999,-35.6336740328742));
#15398=CARTESIAN_POINT('Origin',(17.405,15.5,-34.479));
#15399=CARTESIAN_POINT('',(17.913,15.8175,-35.6336740328742));
#15400=CARTESIAN_POINT('Ctrl Pts',(17.913,15.8175000000001,-35.6336740328742));
#15401=CARTESIAN_POINT('Ctrl Pts',(17.913,15.7089379368767,-35.6401598997242));
#15402=CARTESIAN_POINT('Ctrl Pts',(17.913,15.6022821151611,-35.6429742265188));
#15403=CARTESIAN_POINT('Ctrl Pts',(17.913,15.5,-35.6429742265188));
#15404=CARTESIAN_POINT('',(17.3783553311341,15.8175,-35.749));
#15405=CARTESIAN_POINT('Origin',(17.3559153980514,15.8175,-34.4373099752802));
#15406=CARTESIAN_POINT('',(15.8175,17.3783553311341,-35.749));
#15407=CARTESIAN_POINT('Origin',(15.5,15.5,-35.749));
#15408=CARTESIAN_POINT('',(15.8175,17.913,-35.6336740328739));
#15409=CARTESIAN_POINT('Origin',(15.8175000000003,17.3559153980479,-34.4373099752707));
#15410=CARTESIAN_POINT('',(15.1825,17.913,-35.633674032875));
#15411=CARTESIAN_POINT('Ctrl Pts',(15.8175,17.913,-35.6336740328742));
#15412=CARTESIAN_POINT('Ctrl Pts',(15.7089379368767,17.913,-35.6401598997242));
#15413=CARTESIAN_POINT('Ctrl Pts',(15.6022821151611,17.913,-35.6429742265188));
#15414=CARTESIAN_POINT('Ctrl Pts',(15.3977178848389,17.913,-35.6429742265188));
#15415=CARTESIAN_POINT('Ctrl Pts',(15.2910620631233,17.913,-35.6401598997242));
#15416=CARTESIAN_POINT('Ctrl Pts',(15.1825,17.913,-35.6336740328742));
#15417=CARTESIAN_POINT('',(15.1825,17.3783553311341,-35.749));
#15418=CARTESIAN_POINT('Origin',(15.1825000000009,17.3559153980454,-34.4373099752573));
#15419=CARTESIAN_POINT('',(13.6216446688659,15.8175,-35.749));
#15420=CARTESIAN_POINT('Origin',(15.5,15.5,-35.749));
#15421=CARTESIAN_POINT('',(13.087,15.8175,-35.6336740328739));
#15422=CARTESIAN_POINT('Origin',(13.6451071230427,15.8175000000003,-34.4325038145077));
#15423=CARTESIAN_POINT('',(13.087,15.1825,-35.6336740328739));
#15424=CARTESIAN_POINT('Ctrl Pts',(13.087,15.1825,-35.6336740328742));
#15425=CARTESIAN_POINT('Ctrl Pts',(13.087,15.2910620631233,-35.6401598997242));
#15426=CARTESIAN_POINT('Ctrl Pts',(13.087,15.3977178848389,-35.6429742265188));
#15427=CARTESIAN_POINT('Ctrl Pts',(13.087,15.6022821151611,-35.6429742265188));
#15428=CARTESIAN_POINT('Ctrl Pts',(13.087,15.7089379368767,-35.6401598997242));
#15429=CARTESIAN_POINT('Ctrl Pts',(13.087,15.8175,-35.6336740328742));
#15430=CARTESIAN_POINT('',(13.6216446688659,15.1825,-35.749));
#15431=CARTESIAN_POINT('Origin',(13.6451071230429,15.1824999999997,-34.4325038145053));
#15432=CARTESIAN_POINT('',(15.1825,13.6216446688659,-35.749));
#15433=CARTESIAN_POINT('Origin',(15.5,15.5,-35.749));
#15434=CARTESIAN_POINT('',(15.1825,13.087,-35.6336740328739));
#15435=CARTESIAN_POINT('Origin',(15.1824999999996,13.6451071230448,-34.4325038144978));
#15436=CARTESIAN_POINT('',(15.8175,13.087,-35.633674032875));
#15437=CARTESIAN_POINT('Ctrl Pts',(15.1825,13.087,-35.6336740328742));
#15438=CARTESIAN_POINT('Ctrl Pts',(15.2910620631233,13.087,-35.6401598997242));
#15439=CARTESIAN_POINT('Ctrl Pts',(15.3977178848389,13.087,-35.6429742265188));
#15440=CARTESIAN_POINT('Ctrl Pts',(15.6022821151611,13.087,-35.6429742265188));
#15441=CARTESIAN_POINT('Ctrl Pts',(15.7089379368767,13.087,-35.6401598997242));
#15442=CARTESIAN_POINT('Ctrl Pts',(15.8175,13.087,-35.6336740328742));
#15443=CARTESIAN_POINT('',(15.8175,13.6216446688659,-35.749));
#15444=CARTESIAN_POINT('Origin',(15.8174999999991,13.6451071230564,-34.4325038144518));
#15445=CARTESIAN_POINT('',(17.3783553311341,15.1825,-35.749));
#15446=CARTESIAN_POINT('Origin',(15.5,15.5,-35.749));
#15447=CARTESIAN_POINT('Origin',(17.3559153980526,15.1824999999996,-34.4373099752921));
#15448=CARTESIAN_POINT('Origin',(0.,0.,-35.749));
#15449=CARTESIAN_POINT('',(15.1825,15.8175,-35.749));
#15450=CARTESIAN_POINT('',(15.1825,17.913,-35.749));
#15451=CARTESIAN_POINT('',(17.913,15.8175,-35.749));
#15452=CARTESIAN_POINT('Origin',(0.,0.,-35.749));
#15453=CARTESIAN_POINT('',(15.1825,15.1825,-35.749));
#15454=CARTESIAN_POINT('',(17.913,15.1825,-35.749));
#15455=CARTESIAN_POINT('',(15.1825,17.913,-35.749));
#15456=CARTESIAN_POINT('Origin',(0.,0.,-35.749));
#15457=CARTESIAN_POINT('',(15.8175,15.1825,-35.749));
#15458=CARTESIAN_POINT('',(15.8175,17.913,-35.749));
#15459=CARTESIAN_POINT('',(17.913,15.1825,-35.749));
#15460=CARTESIAN_POINT('Origin',(15.5,15.5,-33.844));
#15461=CARTESIAN_POINT('Origin',(0.,0.,-35.749));
#15462=CARTESIAN_POINT('',(15.8175,15.8175,-35.749));
#15463=CARTESIAN_POINT('',(15.8175,17.913,-35.749));
#15464=CARTESIAN_POINT('',(17.913,15.8175,-35.749));
#15465=CARTESIAN_POINT('Origin',(15.8175,17.913,-34.987));
#15466=CARTESIAN_POINT('',(15.8175,15.8175,-34.987));
#15467=CARTESIAN_POINT('',(15.8175,15.8175,-34.987));
#15468=CARTESIAN_POINT('',(15.8175,17.913,-34.987));
#15469=CARTESIAN_POINT('',(15.8175,17.913,-34.987));
#15470=CARTESIAN_POINT('',(15.8175,17.913,-34.987));
#15471=CARTESIAN_POINT('Origin',(15.1825,17.913,-34.987));
#15472=CARTESIAN_POINT('',(15.1825,17.913,-34.987));
#15473=CARTESIAN_POINT('',(15.1825,17.913,-34.987));
#15474=CARTESIAN_POINT('',(15.1825,15.8175,-34.987));
#15475=CARTESIAN_POINT('',(15.1825,17.913,-34.987));
#15476=CARTESIAN_POINT('',(15.1825,15.8175,-34.987));
#15477=CARTESIAN_POINT('Origin',(15.8175,17.913,-34.987));
#15478=CARTESIAN_POINT('',(15.8175,13.087,-34.987));
#15479=CARTESIAN_POINT('',(15.8175,13.087,-34.987));
#15480=CARTESIAN_POINT('',(15.8175,15.1825,-34.987));
#15481=CARTESIAN_POINT('',(15.8175,17.913,-34.987));
#15482=CARTESIAN_POINT('',(15.8175,15.1825,-34.987));
#15483=CARTESIAN_POINT('Origin',(15.8175,17.913,-34.987));
#15484=CARTESIAN_POINT('',(15.8175,17.913,-34.987));
#15485=CARTESIAN_POINT('Origin',(15.1825,17.913,-34.987));
#15486=CARTESIAN_POINT('',(15.1825,15.1825,-34.987));
#15487=CARTESIAN_POINT('',(15.1825,15.1825,-34.987));
#15488=CARTESIAN_POINT('',(15.1825,13.087,-34.987));
#15489=CARTESIAN_POINT('',(15.1825,17.913,-34.987));
#15490=CARTESIAN_POINT('',(15.1825,13.087,-34.987));
#15491=CARTESIAN_POINT('Origin',(15.1825,13.087,-34.987));
#15492=CARTESIAN_POINT('',(15.1825,13.087,-34.987));
#15493=CARTESIAN_POINT('Origin',(0.,0.,-34.987));
#15494=CARTESIAN_POINT('',(13.087,15.1825,-34.987));
#15495=CARTESIAN_POINT('',(17.913,15.1825,-34.987));
#15496=CARTESIAN_POINT('',(13.087,15.8175,-34.987));
#15497=CARTESIAN_POINT('',(13.087,15.8175,-34.987));
#15498=CARTESIAN_POINT('',(17.913,15.8175,-34.987));
#15499=CARTESIAN_POINT('',(17.913,15.8175,-34.987));
#15500=CARTESIAN_POINT('',(17.913,15.8175,-34.987));
#15501=CARTESIAN_POINT('',(17.913,15.1825,-34.987));
#15502=CARTESIAN_POINT('',(17.913,15.1825,-34.987));
#15503=CARTESIAN_POINT('',(17.913,15.1825,-34.987));
#15504=CARTESIAN_POINT('Origin',(13.087,15.8175,-34.987));
#15505=CARTESIAN_POINT('',(13.087,15.8175,-34.987));
#15506=CARTESIAN_POINT('',(13.087,15.1825,-34.987));
#15507=CARTESIAN_POINT('Origin',(17.913,15.8175,-34.987));
#15508=CARTESIAN_POINT('Origin',(17.913,15.1825,-34.987));
#15509=CARTESIAN_POINT('Origin',(17.913,15.1825,-34.987));
#15510=CARTESIAN_POINT('',(17.913,15.1825,-34.987));
#15511=CARTESIAN_POINT('Origin',(17.913,15.1825,-34.987));
#15512=CARTESIAN_POINT('',(17.913,15.8175,-34.987));
#15513=CARTESIAN_POINT('Origin',(17.913,15.8175,-34.987));
#15514=CARTESIAN_POINT('Origin',(-15.5000000000001,15.5,-45.9992561210692));
#15515=CARTESIAN_POINT('',(-15.5,12.3249999999999,-33.844));
#15516=CARTESIAN_POINT('Origin',(-15.5000000000001,15.5,-33.844));
#15517=CARTESIAN_POINT('',(-15.5000000000001,12.325,-34.479));
#15518=CARTESIAN_POINT('',(-15.5000000000001,12.325,-45.9992561210692));
#15519=CARTESIAN_POINT('',(-15.5000000000001,18.675,-34.479));
#15520=CARTESIAN_POINT('Origin',(-15.5000000000001,15.5,-34.479));
#15521=CARTESIAN_POINT('Origin',(-15.5000000000001,15.5,-34.479));
#15522=CARTESIAN_POINT('Origin',(-15.5000000000001,15.5,-34.479));
#15523=CARTESIAN_POINT('',(-15.1825000000001,17.913,-35.6336740328739));
#15524=CARTESIAN_POINT('',(-15.5000000000001,17.913,-35.6429742265188));
#15525=CARTESIAN_POINT('Ctrl Pts',(-15.5000000000001,17.913,-35.6429742265188));
#15526=CARTESIAN_POINT('Ctrl Pts',(-15.397717884839,17.913,-35.6429742265188));
#15527=CARTESIAN_POINT('Ctrl Pts',(-15.2910620631234,17.913,-35.6401598997242));
#15528=CARTESIAN_POINT('Ctrl Pts',(-15.1825,17.913,-35.6336740328742));
#15529=CARTESIAN_POINT('Origin',(-15.5000000000001,17.405,-34.479));
#15530=CARTESIAN_POINT('',(-15.8175000000001,17.913,-35.6336740328742));
#15531=CARTESIAN_POINT('Ctrl Pts',(-15.8175000000002,17.913,-35.6336740328742));
#15532=CARTESIAN_POINT('Ctrl Pts',(-15.7089379368768,17.913,-35.6401598997242));
#15533=CARTESIAN_POINT('Ctrl Pts',(-15.6022821151612,17.913,-35.6429742265188));
#15534=CARTESIAN_POINT('Ctrl Pts',(-15.5000000000001,17.913,-35.6429742265188));
#15535=CARTESIAN_POINT('',(-15.8175000000001,17.3783553311341,-35.749));
#15536=CARTESIAN_POINT('Origin',(-15.8174999999999,17.3559153980509,-34.4373099752779));
#15537=CARTESIAN_POINT('',(-17.3783553311342,15.8174999999999,-35.749));
#15538=CARTESIAN_POINT('Origin',(-15.5000000000001,15.5,-35.749));
#15539=CARTESIAN_POINT('',(-17.9130000000001,15.8174999999999,-35.6336740328739));
#15540=CARTESIAN_POINT('Origin',(-17.3559153980642,15.8175000000004,-34.4373099753428));
#15541=CARTESIAN_POINT('',(-17.913,15.1824999999999,-35.633674032875));
#15542=CARTESIAN_POINT('Ctrl Pts',(-17.9130000000001,15.8174999999999,-35.6336740328742));
#15543=CARTESIAN_POINT('Ctrl Pts',(-17.9130000000001,15.7089379368766,-35.6401598997242));
#15544=CARTESIAN_POINT('Ctrl Pts',(-17.9130000000001,15.6022821151611,-35.6429742265188));
#15545=CARTESIAN_POINT('Ctrl Pts',(-17.9130000000001,15.3977178848389,-35.6429742265188));
#15546=CARTESIAN_POINT('Ctrl Pts',(-17.9130000000001,15.2910620631233,-35.6401598997242));
#15547=CARTESIAN_POINT('Ctrl Pts',(-17.9130000000001,15.1824999999999,-35.6336740328742));
#15548=CARTESIAN_POINT('',(-17.3783553311342,15.1824999999999,-35.749));
#15549=CARTESIAN_POINT('Origin',(-17.3559153980482,15.1825000000009,-34.4373099752696));
#15550=CARTESIAN_POINT('',(-15.8175,13.6216446688658,-35.749));
#15551=CARTESIAN_POINT('Origin',(-15.5000000000001,15.5,-35.749));
#15552=CARTESIAN_POINT('',(-15.8175,13.087,-35.6336740328739));
#15553=CARTESIAN_POINT('Origin',(-15.8175000000003,13.6451071230414,-34.4325038145137));
#15554=CARTESIAN_POINT('',(-15.1825,13.087,-35.6336740328739));
#15555=CARTESIAN_POINT('Ctrl Pts',(-15.1825,13.087,-35.6336740328742));
#15556=CARTESIAN_POINT('Ctrl Pts',(-15.2910620631233,13.087,-35.6401598997242));
#15557=CARTESIAN_POINT('Ctrl Pts',(-15.397717884839,13.087,-35.6429742265188));
#15558=CARTESIAN_POINT('Ctrl Pts',(-15.6022821151612,13.087,-35.6429742265188));
#15559=CARTESIAN_POINT('Ctrl Pts',(-15.7089379368768,13.087,-35.6401598997242));
#15560=CARTESIAN_POINT('Ctrl Pts',(-15.8175,13.087,-35.6336740328742));
#15561=CARTESIAN_POINT('',(-15.1825,13.6216446688658,-35.749));
#15562=CARTESIAN_POINT('Origin',(-15.1824999999997,13.6451071230399,-34.4325038145209));
#15563=CARTESIAN_POINT('',(-13.6216446688659,15.1825,-35.749));
#15564=CARTESIAN_POINT('Origin',(-15.5000000000001,15.5,-35.749));
#15565=CARTESIAN_POINT('',(-13.0870000000001,15.1825,-35.6336740328739));
#15566=CARTESIAN_POINT('Origin',(-13.6451071230419,15.1824999999996,-34.4325038145103));
#15567=CARTESIAN_POINT('',(-13.0870000000001,15.8175,-35.633674032875));
#15568=CARTESIAN_POINT('Ctrl Pts',(-13.0870000000001,15.1825,-35.6336740328742));
#15569=CARTESIAN_POINT('Ctrl Pts',(-13.0870000000001,15.2910620631233,-35.6401598997242));
#15570=CARTESIAN_POINT('Ctrl Pts',(-13.0870000000001,15.3977178848389,-35.6429742265188));
#15571=CARTESIAN_POINT('Ctrl Pts',(-13.0870000000001,15.6022821151611,-35.6429742265188));
#15572=CARTESIAN_POINT('Ctrl Pts',(-13.0870000000001,15.7089379368767,-35.6401598997242));
#15573=CARTESIAN_POINT('Ctrl Pts',(-13.0870000000001,15.8175,-35.6336740328742));
#15574=CARTESIAN_POINT('',(-13.6216446688659,15.8175,-35.749));
#15575=CARTESIAN_POINT('Origin',(-13.6451071230542,15.8174999999991,-34.4325038144614));
#15576=CARTESIAN_POINT('',(-15.1825000000001,17.378355331134,-35.749));
#15577=CARTESIAN_POINT('Origin',(-15.5000000000001,15.5,-35.749));
#15578=CARTESIAN_POINT('Origin',(-15.1824999999996,17.3559153980558,-34.4373099753074));
#15579=CARTESIAN_POINT('Origin',(-1.48788610350143E-30,-1.48788610350144E-30,
-35.749));
#15580=CARTESIAN_POINT('',(-15.8175000000001,15.1825,-35.749));
#15581=CARTESIAN_POINT('',(-17.913,15.1824999999999,-35.749));
#15582=CARTESIAN_POINT('',(-15.8175000000001,17.913,-35.749));
#15583=CARTESIAN_POINT('Origin',(-1.48788610350143E-30,-1.48788610350144E-30,
-35.749));
#15584=CARTESIAN_POINT('',(-15.1825000000001,15.1825,-35.749));
#15585=CARTESIAN_POINT('',(-15.1825000000001,17.913,-35.749));
#15586=CARTESIAN_POINT('',(-17.913,15.1824999999999,-35.749));
#15587=CARTESIAN_POINT('Origin',(-1.48788610350143E-30,-1.48788610350144E-30,
-35.749));
#15588=CARTESIAN_POINT('',(-15.1825000000001,15.8175,-35.749));
#15589=CARTESIAN_POINT('',(-17.9130000000001,15.8174999999999,-35.749));
#15590=CARTESIAN_POINT('',(-15.1825000000001,17.913,-35.749));
#15591=CARTESIAN_POINT('Origin',(-15.5000000000001,15.5,-33.844));
#15592=CARTESIAN_POINT('Origin',(-1.48788610350143E-30,-1.48788610350144E-30,
-35.749));
#15593=CARTESIAN_POINT('',(-15.8175000000001,15.8174999999999,-35.749));
#15594=CARTESIAN_POINT('',(-17.9130000000001,15.8174999999999,-35.749));
#15595=CARTESIAN_POINT('',(-15.8175000000001,17.913,-35.749));
#15596=CARTESIAN_POINT('Origin',(-17.9130000000001,15.8174999999999,-34.987));
#15597=CARTESIAN_POINT('',(-15.8175000000001,15.8174999999999,-34.987));
#15598=CARTESIAN_POINT('',(-15.8175000000001,15.8174999999999,-34.987));
#15599=CARTESIAN_POINT('',(-17.9130000000001,15.8174999999999,-34.987));
#15600=CARTESIAN_POINT('',(-17.9130000000001,15.8174999999999,-34.987));
#15601=CARTESIAN_POINT('',(-17.9130000000001,15.8174999999999,-34.987));
#15602=CARTESIAN_POINT('Origin',(-17.913,15.1824999999999,-34.987));
#15603=CARTESIAN_POINT('',(-17.913,15.1824999999999,-34.987));
#15604=CARTESIAN_POINT('',(-17.913,15.1824999999999,-34.987));
#15605=CARTESIAN_POINT('',(-15.8175000000001,15.1825,-34.987));
#15606=CARTESIAN_POINT('',(-17.913,15.1824999999999,-34.987));
#15607=CARTESIAN_POINT('',(-15.8175000000001,15.1825,-34.987));
#15608=CARTESIAN_POINT('Origin',(-17.9130000000001,15.8174999999999,-34.987));
#15609=CARTESIAN_POINT('',(-13.0870000000001,15.8175,-34.987));
#15610=CARTESIAN_POINT('',(-13.0870000000001,15.8175,-34.987));
#15611=CARTESIAN_POINT('',(-15.1825000000001,15.8175,-34.987));
#15612=CARTESIAN_POINT('',(-17.9130000000001,15.8174999999999,-34.987));
#15613=CARTESIAN_POINT('',(-15.1825000000001,15.8175,-34.987));
#15614=CARTESIAN_POINT('Origin',(-17.9130000000001,15.8174999999999,-34.987));
#15615=CARTESIAN_POINT('',(-17.9130000000001,15.8174999999999,-34.987));
#15616=CARTESIAN_POINT('Origin',(-17.913,15.1824999999999,-34.987));
#15617=CARTESIAN_POINT('',(-15.1825000000001,15.1825,-34.987));
#15618=CARTESIAN_POINT('',(-15.1825000000001,15.1825,-34.987));
#15619=CARTESIAN_POINT('',(-13.0870000000001,15.1825,-34.987));
#15620=CARTESIAN_POINT('',(-17.913,15.1824999999999,-34.987));
#15621=CARTESIAN_POINT('',(-13.0870000000001,15.1825,-34.987));
#15622=CARTESIAN_POINT('Origin',(-13.0870000000001,15.1825,-34.987));
#15623=CARTESIAN_POINT('',(-13.0870000000001,15.1825,-34.987));
#15624=CARTESIAN_POINT('Origin',(-1.45617139229641E-30,-1.45617139229642E-30,
-34.987));
#15625=CARTESIAN_POINT('',(-15.1825,13.087,-34.987));
#15626=CARTESIAN_POINT('',(-15.1825000000001,17.913,-34.987));
#15627=CARTESIAN_POINT('',(-15.8175,13.087,-34.987));
#15628=CARTESIAN_POINT('',(-15.8175,13.087,-34.987));
#15629=CARTESIAN_POINT('',(-15.8175000000001,17.913,-34.987));
#15630=CARTESIAN_POINT('',(-15.8175000000001,17.913,-34.987));
#15631=CARTESIAN_POINT('',(-15.8175000000001,17.913,-34.987));
#15632=CARTESIAN_POINT('',(-15.1825000000001,17.913,-34.987));
#15633=CARTESIAN_POINT('',(-15.1825000000001,17.913,-34.987));
#15634=CARTESIAN_POINT('',(-15.1825000000001,17.913,-34.987));
#15635=CARTESIAN_POINT('Origin',(-15.8175,13.087,-34.987));
#15636=CARTESIAN_POINT('',(-15.8175,13.087,-34.987));
#15637=CARTESIAN_POINT('',(-15.1825,13.087,-34.987));
#15638=CARTESIAN_POINT('Origin',(-15.8175000000001,17.913,-34.987));
#15639=CARTESIAN_POINT('Origin',(-15.1825000000001,17.913,-34.987));
#15640=CARTESIAN_POINT('Origin',(-15.1825000000001,17.913,-34.987));
#15641=CARTESIAN_POINT('',(-15.1825000000001,17.913,-34.987));
#15642=CARTESIAN_POINT('Origin',(-15.1825000000001,17.913,-34.987));
#15643=CARTESIAN_POINT('',(-15.8175000000001,17.913,-34.987));
#15644=CARTESIAN_POINT('Origin',(-15.8175000000001,17.913,-34.987));
#15645=CARTESIAN_POINT('Origin',(-15.5,-15.5,-45.9992561210692));
#15646=CARTESIAN_POINT('',(-12.325,-15.5,-33.844));
#15647=CARTESIAN_POINT('Origin',(-15.5,-15.5,-33.844));
#15648=CARTESIAN_POINT('',(-12.325,-15.5,-34.479));
#15649=CARTESIAN_POINT('',(-12.325,-15.5,-45.9992561210692));
#15650=CARTESIAN_POINT('',(-18.675,-15.5,-34.479));
#15651=CARTESIAN_POINT('Origin',(-15.5,-15.5,-34.479));
#15652=CARTESIAN_POINT('Origin',(-15.5,-15.5,-34.479));
#15653=CARTESIAN_POINT('Origin',(-15.5,-15.5,-34.479));
#15654=CARTESIAN_POINT('',(-17.913,-15.1825,-35.6336740328739));
#15655=CARTESIAN_POINT('',(-17.913,-15.5,-35.6429742265188));
#15656=CARTESIAN_POINT('Ctrl Pts',(-17.913,-15.5,-35.6429742265188));
#15657=CARTESIAN_POINT('Ctrl Pts',(-17.913,-15.3977178848389,-35.6429742265188));
#15658=CARTESIAN_POINT('Ctrl Pts',(-17.913,-15.2910620631233,-35.6401598997242));
#15659=CARTESIAN_POINT('Ctrl Pts',(-17.913,-15.1824999999999,-35.6336740328742));
#15660=CARTESIAN_POINT('Origin',(-17.405,-15.5,-34.479));
#15661=CARTESIAN_POINT('',(-17.913,-15.8175,-35.6336740328742));
#15662=CARTESIAN_POINT('Ctrl Pts',(-17.913,-15.8175000000001,-35.6336740328742));
#15663=CARTESIAN_POINT('Ctrl Pts',(-17.913,-15.7089379368767,-35.6401598997242));
#15664=CARTESIAN_POINT('Ctrl Pts',(-17.913,-15.6022821151611,-35.6429742265188));
#15665=CARTESIAN_POINT('Ctrl Pts',(-17.913,-15.5,-35.6429742265188));
#15666=CARTESIAN_POINT('',(-17.3783553311341,-15.8175,-35.749));
#15667=CARTESIAN_POINT('Origin',(-17.3559153980514,-15.8175,-34.4373099752802));
#15668=CARTESIAN_POINT('',(-15.8175,-17.3783553311341,-35.749));
#15669=CARTESIAN_POINT('Origin',(-15.5,-15.5,-35.749));
#15670=CARTESIAN_POINT('',(-15.8175,-17.913,-35.6336740328739));
#15671=CARTESIAN_POINT('Origin',(-15.8175000000003,-17.3559153980479,-34.4373099752707));
#15672=CARTESIAN_POINT('',(-15.1825,-17.913,-35.633674032875));
#15673=CARTESIAN_POINT('Ctrl Pts',(-15.8175,-17.913,-35.6336740328742));
#15674=CARTESIAN_POINT('Ctrl Pts',(-15.7089379368767,-17.913,-35.6401598997242));
#15675=CARTESIAN_POINT('Ctrl Pts',(-15.6022821151611,-17.913,-35.6429742265188));
#15676=CARTESIAN_POINT('Ctrl Pts',(-15.3977178848389,-17.913,-35.6429742265188));
#15677=CARTESIAN_POINT('Ctrl Pts',(-15.2910620631233,-17.913,-35.6401598997242));
#15678=CARTESIAN_POINT('Ctrl Pts',(-15.1825,-17.913,-35.6336740328742));
#15679=CARTESIAN_POINT('',(-15.1825,-17.3783553311341,-35.749));
#15680=CARTESIAN_POINT('Origin',(-15.1825000000009,-17.3559153980454,-34.4373099752573));
#15681=CARTESIAN_POINT('',(-13.6216446688659,-15.8175,-35.749));
#15682=CARTESIAN_POINT('Origin',(-15.5,-15.5,-35.749));
#15683=CARTESIAN_POINT('',(-13.087,-15.8175,-35.6336740328739));
#15684=CARTESIAN_POINT('Origin',(-13.6451071230427,-15.8175000000003,-34.4325038145077));
#15685=CARTESIAN_POINT('',(-13.087,-15.1825,-35.6336740328739));
#15686=CARTESIAN_POINT('Ctrl Pts',(-13.087,-15.1825,-35.6336740328742));
#15687=CARTESIAN_POINT('Ctrl Pts',(-13.087,-15.2910620631233,-35.6401598997242));
#15688=CARTESIAN_POINT('Ctrl Pts',(-13.087,-15.3977178848389,-35.6429742265188));
#15689=CARTESIAN_POINT('Ctrl Pts',(-13.087,-15.6022821151611,-35.6429742265188));
#15690=CARTESIAN_POINT('Ctrl Pts',(-13.087,-15.7089379368767,-35.6401598997242));
#15691=CARTESIAN_POINT('Ctrl Pts',(-13.087,-15.8175,-35.6336740328742));
#15692=CARTESIAN_POINT('',(-13.6216446688659,-15.1825,-35.749));
#15693=CARTESIAN_POINT('Origin',(-13.6451071230429,-15.1824999999997,-34.4325038145053));
#15694=CARTESIAN_POINT('',(-15.1825,-13.6216446688659,-35.749));
#15695=CARTESIAN_POINT('Origin',(-15.5,-15.5,-35.749));
#15696=CARTESIAN_POINT('',(-15.1825,-13.087,-35.6336740328739));
#15697=CARTESIAN_POINT('Origin',(-15.1824999999996,-13.6451071230448,-34.4325038144978));
#15698=CARTESIAN_POINT('',(-15.8175,-13.087,-35.633674032875));
#15699=CARTESIAN_POINT('Ctrl Pts',(-15.1825,-13.087,-35.6336740328742));
#15700=CARTESIAN_POINT('Ctrl Pts',(-15.2910620631233,-13.087,-35.6401598997242));
#15701=CARTESIAN_POINT('Ctrl Pts',(-15.3977178848389,-13.087,-35.6429742265188));
#15702=CARTESIAN_POINT('Ctrl Pts',(-15.6022821151611,-13.087,-35.6429742265188));
#15703=CARTESIAN_POINT('Ctrl Pts',(-15.7089379368767,-13.087,-35.6401598997242));
#15704=CARTESIAN_POINT('Ctrl Pts',(-15.8175,-13.087,-35.6336740328742));
#15705=CARTESIAN_POINT('',(-15.8175,-13.6216446688659,-35.749));
#15706=CARTESIAN_POINT('Origin',(-15.8174999999991,-13.6451071230564,-34.4325038144518));
#15707=CARTESIAN_POINT('',(-17.3783553311341,-15.1825,-35.749));
#15708=CARTESIAN_POINT('Origin',(-15.5,-15.5,-35.749));
#15709=CARTESIAN_POINT('Origin',(-17.3559153980526,-15.1824999999996,-34.4373099752921));
#15710=CARTESIAN_POINT('Origin',(0.,-2.97577220700286E-30,-35.749));
#15711=CARTESIAN_POINT('',(-15.1825,-15.8175,-35.749));
#15712=CARTESIAN_POINT('',(-15.1825,-17.913,-35.749));
#15713=CARTESIAN_POINT('',(-17.913,-15.8175,-35.749));
#15714=CARTESIAN_POINT('Origin',(0.,-2.97577220700286E-30,-35.749));
#15715=CARTESIAN_POINT('',(-15.1825,-15.1825,-35.749));
#15716=CARTESIAN_POINT('',(-17.913,-15.1825,-35.749));
#15717=CARTESIAN_POINT('',(-15.1825,-17.913,-35.749));
#15718=CARTESIAN_POINT('Origin',(0.,-2.97577220700286E-30,-35.749));
#15719=CARTESIAN_POINT('',(-15.8175,-15.1825,-35.749));
#15720=CARTESIAN_POINT('',(-15.8175,-17.913,-35.749));
#15721=CARTESIAN_POINT('',(-17.913,-15.1825,-35.749));
#15722=CARTESIAN_POINT('Origin',(-15.5,-15.5,-33.844));
#15723=CARTESIAN_POINT('Origin',(0.,-2.97577220700286E-30,-35.749));
#15724=CARTESIAN_POINT('',(-15.8175,-15.8175,-35.749));
#15725=CARTESIAN_POINT('',(-15.8175,-17.913,-35.749));
#15726=CARTESIAN_POINT('',(-17.913,-15.8175,-35.749));
#15727=CARTESIAN_POINT('Origin',(-15.8175,-17.913,-34.987));
#15728=CARTESIAN_POINT('',(-15.8175,-15.8175,-34.987));
#15729=CARTESIAN_POINT('',(-15.8175,-15.8175,-34.987));
#15730=CARTESIAN_POINT('',(-15.8175,-17.913,-34.987));
#15731=CARTESIAN_POINT('',(-15.8175,-17.913,-34.987));
#15732=CARTESIAN_POINT('',(-15.8175,-17.913,-34.987));
#15733=CARTESIAN_POINT('Origin',(-15.1825,-17.913,-34.987));
#15734=CARTESIAN_POINT('',(-15.1825,-17.913,-34.987));
#15735=CARTESIAN_POINT('',(-15.1825,-17.913,-34.987));
#15736=CARTESIAN_POINT('',(-15.1825,-15.8175,-34.987));
#15737=CARTESIAN_POINT('',(-15.1825,-17.913,-34.987));
#15738=CARTESIAN_POINT('',(-15.1825,-15.8175,-34.987));
#15739=CARTESIAN_POINT('Origin',(-15.8175,-17.913,-34.987));
#15740=CARTESIAN_POINT('',(-15.8175,-13.087,-34.987));
#15741=CARTESIAN_POINT('',(-15.8175,-13.087,-34.987));
#15742=CARTESIAN_POINT('',(-15.8175,-15.1825,-34.987));
#15743=CARTESIAN_POINT('',(-15.8175,-17.913,-34.987));
#15744=CARTESIAN_POINT('',(-15.8175,-15.1825,-34.987));
#15745=CARTESIAN_POINT('Origin',(-15.8175,-17.913,-34.987));
#15746=CARTESIAN_POINT('',(-15.8175,-17.913,-34.987));
#15747=CARTESIAN_POINT('Origin',(-15.1825,-17.913,-34.987));
#15748=CARTESIAN_POINT('',(-15.1825,-15.1825,-34.987));
#15749=CARTESIAN_POINT('',(-15.1825,-15.1825,-34.987));
#15750=CARTESIAN_POINT('',(-15.1825,-13.087,-34.987));
#15751=CARTESIAN_POINT('',(-15.1825,-17.913,-34.987));
#15752=CARTESIAN_POINT('',(-15.1825,-13.087,-34.987));
#15753=CARTESIAN_POINT('Origin',(-15.1825,-13.087,-34.987));
#15754=CARTESIAN_POINT('',(-15.1825,-13.087,-34.987));
#15755=CARTESIAN_POINT('Origin',(0.,-2.91234278459283E-30,-34.987));
#15756=CARTESIAN_POINT('',(-13.087,-15.1825,-34.987));
#15757=CARTESIAN_POINT('',(-17.913,-15.1825,-34.987));
#15758=CARTESIAN_POINT('',(-13.087,-15.8175,-34.987));
#15759=CARTESIAN_POINT('',(-13.087,-15.8175,-34.987));
#15760=CARTESIAN_POINT('',(-17.913,-15.8175,-34.987));
#15761=CARTESIAN_POINT('',(-17.913,-15.8175,-34.987));
#15762=CARTESIAN_POINT('',(-17.913,-15.8175,-34.987));
#15763=CARTESIAN_POINT('',(-17.913,-15.1825,-34.987));
#15764=CARTESIAN_POINT('',(-17.913,-15.1825,-34.987));
#15765=CARTESIAN_POINT('',(-17.913,-15.1825,-34.987));
#15766=CARTESIAN_POINT('Origin',(-13.087,-15.8175,-34.987));
#15767=CARTESIAN_POINT('',(-13.087,-15.8175,-34.987));
#15768=CARTESIAN_POINT('',(-13.087,-15.1825,-34.987));
#15769=CARTESIAN_POINT('Origin',(-17.913,-15.8175,-34.987));
#15770=CARTESIAN_POINT('Origin',(-17.913,-15.1825,-34.987));
#15771=CARTESIAN_POINT('Origin',(-17.913,-15.1825,-34.987));
#15772=CARTESIAN_POINT('',(-17.913,-15.1825,-34.987));
#15773=CARTESIAN_POINT('Origin',(-17.913,-15.1825,-34.987));
#15774=CARTESIAN_POINT('',(-17.913,-15.8175,-34.987));
#15775=CARTESIAN_POINT('Origin',(-17.913,-15.8175,-34.987));
#15776=CARTESIAN_POINT('Origin',(15.5000000000002,-15.4999999999998,-45.9992561210692));
#15777=CARTESIAN_POINT('',(15.5000000000001,-12.3249999999998,-33.844));
#15778=CARTESIAN_POINT('Origin',(15.5000000000002,-15.4999999999998,-33.844));
#15779=CARTESIAN_POINT('',(15.5000000000002,-12.3249999999998,-34.479));
#15780=CARTESIAN_POINT('',(15.5000000000002,-12.3249999999998,-45.9992561210692));
#15781=CARTESIAN_POINT('',(15.5000000000002,-18.6749999999998,-34.479));
#15782=CARTESIAN_POINT('Origin',(15.5000000000002,-15.4999999999998,-34.479));
#15783=CARTESIAN_POINT('Origin',(15.5000000000002,-15.4999999999998,-34.479));
#15784=CARTESIAN_POINT('Origin',(15.5000000000002,-15.4999999999998,-34.479));
#15785=CARTESIAN_POINT('',(15.1825000000002,-17.9129999999998,-35.6336740328739));
#15786=CARTESIAN_POINT('',(15.5000000000002,-17.9129999999998,-35.6429742265188));
#15787=CARTESIAN_POINT('Ctrl Pts',(15.5000000000002,-17.9129999999998,-35.6429742265188));
#15788=CARTESIAN_POINT('Ctrl Pts',(15.3977178848391,-17.9129999999998,-35.6429742265188));
#15789=CARTESIAN_POINT('Ctrl Pts',(15.2910620631235,-17.9129999999998,-35.6401598997242));
#15790=CARTESIAN_POINT('Ctrl Pts',(15.1825000000001,-17.9129999999998,-35.6336740328742));
#15791=CARTESIAN_POINT('Origin',(15.5000000000002,-17.4049999999998,-34.479));
#15792=CARTESIAN_POINT('',(15.8175000000002,-17.9129999999998,-35.6336740328742));
#15793=CARTESIAN_POINT('Ctrl Pts',(15.8175000000002,-17.9129999999998,-35.6336740328742));
#15794=CARTESIAN_POINT('Ctrl Pts',(15.7089379368769,-17.9129999999998,-35.6401598997242));
#15795=CARTESIAN_POINT('Ctrl Pts',(15.6022821151613,-17.9129999999998,-35.6429742265188));
#15796=CARTESIAN_POINT('Ctrl Pts',(15.5000000000002,-17.9129999999998,-35.6429742265188));
#15797=CARTESIAN_POINT('',(15.8175000000002,-17.378355331134,-35.749));
#15798=CARTESIAN_POINT('Origin',(15.8175000000001,-17.3559153980596,-34.4373099753218));
#15799=CARTESIAN_POINT('',(17.3783553311343,-15.8174999999998,-35.749));
#15800=CARTESIAN_POINT('Origin',(15.5000000000002,-15.4999999999998,-35.749));
#15801=CARTESIAN_POINT('',(17.9130000000002,-15.8174999999998,-35.6336740328739));
#15802=CARTESIAN_POINT('Origin',(17.3559153980476,-15.8175000000002,-34.4373099752683));
#15803=CARTESIAN_POINT('',(17.9130000000002,-15.1824999999998,-35.633674032875));
#15804=CARTESIAN_POINT('Ctrl Pts',(17.9130000000002,-15.8174999999998,-35.6336740328742));
#15805=CARTESIAN_POINT('Ctrl Pts',(17.9130000000002,-15.7089379368765,-35.6401598997242));
#15806=CARTESIAN_POINT('Ctrl Pts',(17.9130000000002,-15.6022821151609,-35.6429742265188));
#15807=CARTESIAN_POINT('Ctrl Pts',(17.9130000000002,-15.3977178848387,-35.6429742265188));
#15808=CARTESIAN_POINT('Ctrl Pts',(17.9130000000002,-15.2910620631231,-35.6401598997242));
#15809=CARTESIAN_POINT('Ctrl Pts',(17.9130000000002,-15.1824999999999,-35.6336740328742));
#15810=CARTESIAN_POINT('',(17.3783553311343,-15.1824999999998,-35.749));
#15811=CARTESIAN_POINT('Origin',(17.3559153980464,-15.1825000000005,-34.4373099752598));
#15812=CARTESIAN_POINT('',(15.8175000000001,-13.6216446688657,-35.749));
#15813=CARTESIAN_POINT('Origin',(15.5000000000002,-15.4999999999998,-35.749));
#15814=CARTESIAN_POINT('',(15.8175000000001,-13.0869999999998,-35.6336740328739));
#15815=CARTESIAN_POINT('Origin',(15.8175000000005,-13.6451071230423,-34.4325038145089));
#15816=CARTESIAN_POINT('',(15.1825000000001,-13.0869999999998,-35.6336740328739));
#15817=CARTESIAN_POINT('Ctrl Pts',(15.1825000000001,-13.0869999999998,-35.6336740328742));
#15818=CARTESIAN_POINT('Ctrl Pts',(15.2910620631234,-13.0869999999998,-35.6401598997242));
#15819=CARTESIAN_POINT('Ctrl Pts',(15.3977178848391,-13.0869999999998,-35.6429742265188));
#15820=CARTESIAN_POINT('Ctrl Pts',(15.6022821151612,-13.0869999999998,-35.6429742265188));
#15821=CARTESIAN_POINT('Ctrl Pts',(15.7089379368768,-13.0869999999998,-35.6401598997242));
#15822=CARTESIAN_POINT('Ctrl Pts',(15.8175000000001,-13.0869999999998,-35.6336740328742));
#15823=CARTESIAN_POINT('',(15.1825000000001,-13.6216446688657,-35.749));
#15824=CARTESIAN_POINT('Origin',(15.1824999999998,-13.6451071230404,-34.4325038145186));
#15825=CARTESIAN_POINT('',(13.621644668866,-15.1824999999999,-35.749));
#15826=CARTESIAN_POINT('Origin',(15.5000000000002,-15.4999999999998,-35.749));
#15827=CARTESIAN_POINT('',(13.0870000000002,-15.1824999999999,-35.6336740328739));
#15828=CARTESIAN_POINT('Origin',(13.6451071230549,-15.1824999999995,-34.4325038144557));
#15829=CARTESIAN_POINT('',(13.0870000000002,-15.8174999999999,-35.633674032875));
#15830=CARTESIAN_POINT('Ctrl Pts',(13.0870000000002,-15.1824999999999,-35.6336740328742));
#15831=CARTESIAN_POINT('Ctrl Pts',(13.0870000000002,-15.2910620631232,-35.6401598997242));
#15832=CARTESIAN_POINT('Ctrl Pts',(13.0870000000002,-15.3977178848388,-35.6429742265188));
#15833=CARTESIAN_POINT('Ctrl Pts',(13.0870000000002,-15.6022821151609,-35.6429742265188));
#15834=CARTESIAN_POINT('Ctrl Pts',(13.0870000000002,-15.7089379368765,-35.6401598997242));
#15835=CARTESIAN_POINT('Ctrl Pts',(13.0870000000002,-15.8174999999999,-35.6336740328742));
#15836=CARTESIAN_POINT('',(13.621644668866,-15.8174999999999,-35.749));
#15837=CARTESIAN_POINT('Origin',(13.6451071230544,-15.817499999999,-34.4325038144617));
#15838=CARTESIAN_POINT('',(15.1825000000002,-17.3783553311339,-35.749));
#15839=CARTESIAN_POINT('Origin',(15.5000000000002,-15.4999999999998,-35.749));
#15840=CARTESIAN_POINT('Origin',(15.1824999999999,-17.3559153980519,-34.4373099752894));
#15841=CARTESIAN_POINT('Origin',(1.48788610350143E-30,-1.48788610350141E-30,
-35.749));
#15842=CARTESIAN_POINT('',(15.8175000000002,-15.1824999999998,-35.749));
#15843=CARTESIAN_POINT('',(17.9130000000002,-15.1824999999998,-35.749));
#15844=CARTESIAN_POINT('',(15.8175000000002,-17.9129999999998,-35.749));
#15845=CARTESIAN_POINT('Origin',(1.48788610350143E-30,-1.48788610350141E-30,
-35.749));
#15846=CARTESIAN_POINT('',(15.1825000000002,-15.1824999999998,-35.749));
#15847=CARTESIAN_POINT('',(15.1825000000002,-17.9129999999998,-35.749));
#15848=CARTESIAN_POINT('',(17.9130000000002,-15.1824999999998,-35.749));
#15849=CARTESIAN_POINT('Origin',(1.48788610350143E-30,-1.48788610350141E-30,
-35.749));
#15850=CARTESIAN_POINT('',(15.1825000000002,-15.8174999999998,-35.749));
#15851=CARTESIAN_POINT('',(17.9130000000002,-15.8174999999998,-35.749));
#15852=CARTESIAN_POINT('',(15.1825000000002,-17.9129999999998,-35.749));
#15853=CARTESIAN_POINT('Origin',(15.5000000000002,-15.4999999999998,-33.844));
#15854=CARTESIAN_POINT('Origin',(1.48788610350143E-30,-1.48788610350141E-30,
-35.749));
#15855=CARTESIAN_POINT('',(15.8175000000002,-15.8174999999998,-35.749));
#15856=CARTESIAN_POINT('',(17.9130000000002,-15.8174999999998,-35.749));
#15857=CARTESIAN_POINT('',(15.8175000000002,-17.9129999999998,-35.749));
#15858=CARTESIAN_POINT('Origin',(17.9130000000002,-15.8174999999998,-34.987));
#15859=CARTESIAN_POINT('',(15.8175000000002,-15.8174999999998,-34.987));
#15860=CARTESIAN_POINT('',(15.8175000000002,-15.8174999999998,-34.987));
#15861=CARTESIAN_POINT('',(17.9130000000002,-15.8174999999998,-34.987));
#15862=CARTESIAN_POINT('',(17.9130000000002,-15.8174999999998,-34.987));
#15863=CARTESIAN_POINT('',(17.9130000000002,-15.8174999999998,-34.987));
#15864=CARTESIAN_POINT('Origin',(17.9130000000002,-15.1824999999998,-34.987));
#15865=CARTESIAN_POINT('',(17.9130000000002,-15.1824999999998,-34.987));
#15866=CARTESIAN_POINT('',(17.9130000000002,-15.1824999999998,-34.987));
#15867=CARTESIAN_POINT('',(15.8175000000002,-15.1824999999998,-34.987));
#15868=CARTESIAN_POINT('',(17.9130000000002,-15.1824999999998,-34.987));
#15869=CARTESIAN_POINT('',(15.8175000000002,-15.1824999999998,-34.987));
#15870=CARTESIAN_POINT('Origin',(17.9130000000002,-15.8174999999998,-34.987));
#15871=CARTESIAN_POINT('',(13.0870000000002,-15.8174999999999,-34.987));
#15872=CARTESIAN_POINT('',(13.0870000000002,-15.8174999999999,-34.987));
#15873=CARTESIAN_POINT('',(15.1825000000002,-15.8174999999998,-34.987));
#15874=CARTESIAN_POINT('',(17.9130000000002,-15.8174999999998,-34.987));
#15875=CARTESIAN_POINT('',(15.1825000000002,-15.8174999999998,-34.987));
#15876=CARTESIAN_POINT('Origin',(17.9130000000002,-15.8174999999998,-34.987));
#15877=CARTESIAN_POINT('',(17.9130000000002,-15.8174999999998,-34.987));
#15878=CARTESIAN_POINT('Origin',(17.9130000000002,-15.1824999999998,-34.987));
#15879=CARTESIAN_POINT('',(15.1825000000002,-15.1824999999998,-34.987));
#15880=CARTESIAN_POINT('',(15.1825000000002,-15.1824999999998,-34.987));
#15881=CARTESIAN_POINT('',(13.0870000000002,-15.1824999999999,-34.987));
#15882=CARTESIAN_POINT('',(17.9130000000002,-15.1824999999998,-34.987));
#15883=CARTESIAN_POINT('',(13.0870000000002,-15.1824999999999,-34.987));
#15884=CARTESIAN_POINT('Origin',(13.0870000000002,-15.1824999999999,-34.987));
#15885=CARTESIAN_POINT('',(13.0870000000002,-15.1824999999999,-34.987));
#15886=CARTESIAN_POINT('Origin',(1.45617139229641E-30,-1.4561713922964E-30,
-34.987));
#15887=CARTESIAN_POINT('',(15.1825000000001,-13.0869999999998,-34.987));
#15888=CARTESIAN_POINT('',(15.1825000000002,-17.9129999999998,-34.987));
#15889=CARTESIAN_POINT('',(15.8175000000001,-13.0869999999998,-34.987));
#15890=CARTESIAN_POINT('',(15.8175000000001,-13.0869999999998,-34.987));
#15891=CARTESIAN_POINT('',(15.8175000000002,-17.9129999999998,-34.987));
#15892=CARTESIAN_POINT('',(15.8175000000002,-17.9129999999998,-34.987));
#15893=CARTESIAN_POINT('',(15.8175000000002,-17.9129999999998,-34.987));
#15894=CARTESIAN_POINT('',(15.1825000000002,-17.9129999999998,-34.987));
#15895=CARTESIAN_POINT('',(15.1825000000002,-17.9129999999998,-34.987));
#15896=CARTESIAN_POINT('',(15.1825000000002,-17.9129999999998,-34.987));
#15897=CARTESIAN_POINT('Origin',(15.8175000000001,-13.0869999999998,-34.987));
#15898=CARTESIAN_POINT('',(15.8175000000001,-13.0869999999998,-34.987));
#15899=CARTESIAN_POINT('',(15.1825000000001,-13.0869999999998,-34.987));
#15900=CARTESIAN_POINT('Origin',(15.8175000000002,-17.9129999999998,-34.987));
#15901=CARTESIAN_POINT('Origin',(15.1825000000002,-17.9129999999998,-34.987));
#15902=CARTESIAN_POINT('Origin',(15.1825000000002,-17.9129999999998,-34.987));
#15903=CARTESIAN_POINT('',(15.1825000000002,-17.9129999999998,-34.987));
#15904=CARTESIAN_POINT('Origin',(15.1825000000002,-17.9129999999998,-34.987));
#15905=CARTESIAN_POINT('',(15.8175000000002,-17.9129999999998,-34.987));
#15906=CARTESIAN_POINT('Origin',(15.8175000000002,-17.9129999999998,-34.987));
#15907=CARTESIAN_POINT('Origin',(-15.5,-15.5,-1.713));
#15908=CARTESIAN_POINT('',(-17.405,-15.5,10.4245));
#15909=CARTESIAN_POINT('',(-17.405,-15.5,10.487));
#15910=CARTESIAN_POINT('',(-17.405,-15.5,-1.713));
#15911=CARTESIAN_POINT('',(-14.1407339385556,-16.8346987578456,10.7369999999971));
#15912=CARTESIAN_POINT('Ctrl Pts',(-17.405,-15.5,10.4245));
#15913=CARTESIAN_POINT('Ctrl Pts',(-17.405,-15.2720840652369,10.4331343389953));
#15914=CARTESIAN_POINT('Ctrl Pts',(-17.3641001824124,-15.0457843881672,
10.4426020195728));
#15915=CARTESIAN_POINT('Ctrl Pts',(-17.1966348744043,-14.5985988585374,
10.4632059864524));
#15916=CARTESIAN_POINT('Ctrl Pts',(-17.0643347591089,-14.3846734577823,
10.4742040131023));
#15917=CARTESIAN_POINT('Ctrl Pts',(-16.730376764707,-14.0257798182943,10.4951047132884));
#15918=CARTESIAN_POINT('Ctrl Pts',(-16.5341453810794,-13.8820757914142,
10.5042617943533));
#15919=CARTESIAN_POINT('Ctrl Pts',(-16.0882488808044,-13.6705967759069,
10.5237673280487));
#15920=CARTESIAN_POINT('Ctrl Pts',(-15.8409345899176,-13.6088375595572,
10.534585975944));
#15921=CARTESIAN_POINT('Ctrl Pts',(-15.3427841976526,-13.5855895851824,
10.5563773316861));
#15922=CARTESIAN_POINT('Ctrl Pts',(-15.0968410526987,-13.6219267784699,
10.5671359994444));
#15923=CARTESIAN_POINT('Ctrl Pts',(-14.6347738095753,-13.785399372733,10.5873489147167));
#15924=CARTESIAN_POINT('Ctrl Pts',(-14.4226768590876,-13.9100795241097,
10.5961644815545));
#15925=CARTESIAN_POINT('Ctrl Pts',(-14.050029015234,-14.2387855609376,10.6167677930241));
#15926=CARTESIAN_POINT('Ctrl Pts',(-13.895491040028,-14.4423528711417,10.6278598074432));
#15927=CARTESIAN_POINT('Ctrl Pts',(-13.6791847013386,-14.8893109807355,
10.6495234227835));
#15928=CARTESIAN_POINT('Ctrl Pts',(-13.6161046016384,-15.1268137316682,
10.659900652251));
#15929=CARTESIAN_POINT('Ctrl Pts',(-13.5822720286564,-15.6205573481791,
10.6793455691953));
#15930=CARTESIAN_POINT('Ctrl Pts',(-13.6148906767425,-15.8722903791592,
10.6890388567062));
#15931=CARTESIAN_POINT('Ctrl Pts',(-13.7413712296963,-16.2461760980631,
10.7059695131874));
#15932=CARTESIAN_POINT('Ctrl Pts',(-13.802449717033,-16.3762850572176,10.7122344697735));
#15933=CARTESIAN_POINT('Ctrl Pts',(-13.9523779911651,-16.6199506503624,
10.7247447379606));
#15934=CARTESIAN_POINT('Ctrl Pts',(-14.040662315962,-16.7327851541203,10.7309503245344));
#15935=CARTESIAN_POINT('Ctrl Pts',(-14.1407339385535,-16.8346987578475,
10.7369999999987));
#15936=CARTESIAN_POINT('',(-13.5949999999999,-15.5,10.737));
#15937=CARTESIAN_POINT('Origin',(-15.5,-15.5,10.737));
#15938=CARTESIAN_POINT('Ctrl Pts',(-13.595,-15.5000000000012,10.7370000000001));
#15939=CARTESIAN_POINT('Ctrl Pts',(-13.5949999999998,-15.2559720572982,
10.727755275695));
#15940=CARTESIAN_POINT('Ctrl Pts',(-13.6418882041557,-15.0141454724656,
10.7175683960863));
#15941=CARTESIAN_POINT('Ctrl Pts',(-13.8269533696929,-14.5550979526125,
10.6961301022759));
#15942=CARTESIAN_POINT('Ctrl Pts',(-13.9657493860806,-14.3432783686507,
10.6850697720519));
#15943=CARTESIAN_POINT('Ctrl Pts',(-14.3151146891572,-13.9879371350501,
10.6639666580166));
#15944=CARTESIAN_POINT('Ctrl Pts',(-14.5213561808095,-13.8469618146069,
10.6548103158002));
#15945=CARTESIAN_POINT('Ctrl Pts',(-14.9736930923868,-13.6528623367304,
10.635023049327));
#15946=CARTESIAN_POINT('Ctrl Pts',(-15.2150758005425,-13.6006007016105,
10.6244638757419));
#15947=CARTESIAN_POINT('Ctrl Pts',(-15.7140940963548,-13.5900452778231,
10.6026345539653));
#15948=CARTESIAN_POINT('Ctrl Pts',(-15.9670093270509,-13.6356819789821,
10.5915708955796));
#15949=CARTESIAN_POINT('Ctrl Pts',(-16.4284043448797,-13.8190288012306,
10.5713873864882));
#15950=CARTESIAN_POINT('Ctrl Pts',(-16.6342169389518,-13.9504340066446,
10.5625623379533));
#15951=CARTESIAN_POINT('Ctrl Pts',(-16.9896936418914,-14.2870989847445,
10.5420330827009));
#15952=CARTESIAN_POINT('Ctrl Pts',(-17.1345401136243,-14.4907494677001,
10.5311498925172));
#15953=CARTESIAN_POINT('Ctrl Pts',(-17.3401653577434,-14.9463862640391,
10.5093911146263));
#15954=CARTESIAN_POINT('Ctrl Pts',(-17.3972469301894,-15.1947525769663,
10.4987335327075));
#15955=CARTESIAN_POINT('Ctrl Pts',(-17.4047548059783,-15.464697685363,10.4883427514567));
#15956=CARTESIAN_POINT('Ctrl Pts',(-17.405,-15.4823535402015,10.4876685162936));
#15957=CARTESIAN_POINT('Ctrl Pts',(-17.405,-15.5,10.487));
#15958=CARTESIAN_POINT('Origin',(-15.5,-15.5,-1.713));
#15959=CARTESIAN_POINT('',(-17.405,-15.5,9.92450000000002));
#15960=CARTESIAN_POINT('',(-17.405,-15.5,9.98699999999996));
#15961=CARTESIAN_POINT('',(-17.405,-15.5,-1.713));
#15962=CARTESIAN_POINT('Ctrl Pts',(-17.405,-15.5,9.92450000000002));
#15963=CARTESIAN_POINT('Ctrl Pts',(-17.405,-15.4858928849603,9.92503443219593));
#15964=CARTESIAN_POINT('Ctrl Pts',(-17.4048432990239,-15.4717795650996,
9.9255725268598));
#15965=CARTESIAN_POINT('Ctrl Pts',(-17.3989206140259,-15.2053500729653,
9.93579545122571));
#15966=CARTESIAN_POINT('Ctrl Pts',(-17.3432288158043,-14.9566768843941,
9.9464342612718));
#15967=CARTESIAN_POINT('Ctrl Pts',(-17.1401035489678,-14.4997826626639,
9.96818599514227));
#15968=CARTESIAN_POINT('Ctrl Pts',(-16.9962976665314,-14.2952281465799,
9.97908067355896));
#15969=CARTESIAN_POINT('Ctrl Pts',(-16.6426392387018,-13.9566550887119,
9.99964244447171));
#15970=CARTESIAN_POINT('Ctrl Pts',(-16.4376668624969,-13.8241974768803,
10.0084822019904));
#15971=CARTESIAN_POINT('Ctrl Pts',(-15.97729573678,-13.6382690782196,10.0286209214006));
#15972=CARTESIAN_POINT('Ctrl Pts',(-15.7244880114004,-13.5912198115294,
10.0396798770165));
#15973=CARTESIAN_POINT('Ctrl Pts',(-15.2251502351818,-13.5991005423923,
10.0615231743139));
#15974=CARTESIAN_POINT('Ctrl Pts',(-14.9833692139113,-13.6501161077889,
10.0720997719197));
#15975=CARTESIAN_POINT('Ctrl Pts',(-14.5302405900597,-13.8417861959255,
10.0919216714758));
#15976=CARTESIAN_POINT('Ctrl Pts',(-14.3235335496068,-13.9814347470377,
10.1010361828006));
#15977=CARTESIAN_POINT('Ctrl Pts',(-13.9719423166695,-14.3349729707548,
10.1221196779632));
#15978=CARTESIAN_POINT('Ctrl Pts',(-13.8316815321583,-14.546608011966,10.1332050547907));
#15979=CARTESIAN_POINT('Ctrl Pts',(-13.6450105327502,-15.0033955585007,
10.1545928552778));
#15980=CARTESIAN_POINT('Ctrl Pts',(-13.5969735500697,-15.2428689153515,
10.164715711879));
#15981=CARTESIAN_POINT('Ctrl Pts',(-13.5930648657893,-15.7372102120197,
10.1835287680117));
#15982=CARTESIAN_POINT('Ctrl Pts',(-13.6412030815586,-15.9874435647518,
10.1939768176186));
#15983=CARTESIAN_POINT('Ctrl Pts',(-13.8307623126648,-16.4509887967258,
10.2156837975944));
#15984=CARTESIAN_POINT('Ctrl Pts',(-13.9688638816563,-16.6603281599289,
10.2266349783049));
#15985=CARTESIAN_POINT('Ctrl Pts',(-14.3126694773338,-17.0091454193476,
10.2473693355128));
#15986=CARTESIAN_POINT('Ctrl Pts',(-14.5131893701912,-17.1472610561492,
10.2563324308918));
#15987=CARTESIAN_POINT('Ctrl Pts',(-14.9653264274279,-17.3457762984031,
10.2761109548304));
#15988=CARTESIAN_POINT('Ctrl Pts',(-15.2143646253066,-17.4003051378336,
10.2870050142302));
#15989=CARTESIAN_POINT('Ctrl Pts',(-15.7123217853693,-17.4089955584802,
10.3087879171201));
#15990=CARTESIAN_POINT('Ctrl Pts',(-15.9564269263558,-17.3657527498055,
10.3194661822552));
#15991=CARTESIAN_POINT('Ctrl Pts',(-16.4143747649841,-17.1891034921468,
10.3394988961059));
#15992=CARTESIAN_POINT('Ctrl Pts',(-16.6239526754419,-17.0575253746799,
10.3484116271306));
#15993=CARTESIAN_POINT('Ctrl Pts',(-16.9869359893406,-16.7172558558466,
10.3692416229483));
#15994=CARTESIAN_POINT('Ctrl Pts',(-17.1349074509725,-16.5098314274038,
10.3803361354248));
#15995=CARTESIAN_POINT('Ctrl Pts',(-17.3375323162512,-16.0580819096674,
10.4018820230515));
#15996=CARTESIAN_POINT('Ctrl Pts',(-17.3936448790322,-15.8195492548674,
10.4121458734487));
#15997=CARTESIAN_POINT('Ctrl Pts',(-17.4044832913812,-15.5512533747567,
10.4225470219212));
#15998=CARTESIAN_POINT('Ctrl Pts',(-17.405,-15.5256168999003,10.4235295325425));
#15999=CARTESIAN_POINT('Ctrl Pts',(-17.405,-15.5,10.4245));
#16000=CARTESIAN_POINT('Ctrl Pts',(-17.405,-15.5,10.487));
#16001=CARTESIAN_POINT('Ctrl Pts',(-17.405,-15.7233674488027,10.4785379752825));
#16002=CARTESIAN_POINT('Ctrl Pts',(-17.3657160047092,-15.9451655039957,
10.4692761752847));
#16003=CARTESIAN_POINT('Ctrl Pts',(-17.2026181913531,-16.3904274326593,
10.44884060887));
#16004=CARTESIAN_POINT('Ctrl Pts',(-17.0709111954349,-16.6063497886673,
10.4377799026799));
#16005=CARTESIAN_POINT('Ctrl Pts',(-16.7320504038859,-16.974252258311,10.4164306778067));
#16006=CARTESIAN_POINT('Ctrl Pts',(-16.5284556753648,-17.1228467103087,
10.4069893121333));
#16007=CARTESIAN_POINT('Ctrl Pts',(-16.0806603218491,-17.3306844436351,
10.3874007139918));
#16008=CARTESIAN_POINT('Ctrl Pts',(-15.8416446290644,-17.3899290558279,
10.3769450843861));
#16009=CARTESIAN_POINT('Ctrl Pts',(-15.3446905793098,-17.4155239047065,
10.3552060620872));
#16010=CARTESIAN_POINT('Ctrl Pts',(-15.0913104239464,-17.3778548751218,
10.3441220657895));
#16011=CARTESIAN_POINT('Ctrl Pts',(-14.6242327547708,-17.2091194672544,
10.3236899717749));
#16012=CARTESIAN_POINT('Ctrl Pts',(-14.4136338488466,-17.0836247288672,
10.3148992200213));
#16013=CARTESIAN_POINT('Ctrl Pts',(-14.0480376738827,-16.7576783955241,
10.2945546927935));
#16014=CARTESIAN_POINT('Ctrl Pts',(-13.8974752650319,-16.5591758882452,
10.2837415073847));
#16015=CARTESIAN_POINT('Ctrl Pts',(-13.6780183424,-16.1108202101679,10.2619560363234));
#16016=CARTESIAN_POINT('Ctrl Pts',(-13.6131998190904,-15.8643163431901,
10.2511997864289));
#16017=CARTESIAN_POINT('Ctrl Pts',(-13.5841010569675,-15.3717108225541,
10.2319015241377));
#16018=CARTESIAN_POINT('Ctrl Pts',(-13.6156809758626,-15.1305503131339,
10.2225514740956));
#16019=CARTESIAN_POINT('Ctrl Pts',(-13.7698309070763,-14.6646055022332,
10.2015280703944));
#16020=CARTESIAN_POINT('Ctrl Pts',(-13.8941011075487,-14.4452691828191,
10.1905006896061));
#16021=CARTESIAN_POINT('Ctrl Pts',(-14.2217833654884,-14.0651557923405,
10.1689333675832));
#16022=CARTESIAN_POINT('Ctrl Pts',(-14.4227033327979,-13.9087673550772,
10.1591258384604));
#16023=CARTESIAN_POINT('Ctrl Pts',(-14.865863187593,-13.6872389907069,10.1397400180406));
#16024=CARTESIAN_POINT('Ctrl Pts',(-15.1023316570555,-13.6211517131275,
10.1293958155269));
#16025=CARTESIAN_POINT('Ctrl Pts',(-15.5968004017892,-13.5807343117028,
10.1077655117328));
#16026=CARTESIAN_POINT('Ctrl Pts',(-15.8504040187405,-13.6105083795636,
10.0966717402126));
#16027=CARTESIAN_POINT('Ctrl Pts',(-16.3229596847464,-13.7646616321221,
10.0760000137906));
#16028=CARTESIAN_POINT('Ctrl Pts',(-16.5383839359081,-13.8843207578509,
10.0671630489989));
#16029=CARTESIAN_POINT('Ctrl Pts',(-16.9138012019442,-14.1997074181159,
10.0470037535998));
#16030=CARTESIAN_POINT('Ctrl Pts',(-17.0697776365901,-14.3930311503321,
10.0362683432509));
#16031=CARTESIAN_POINT('Ctrl Pts',(-17.3024997474288,-14.8338683737813,
10.0144775606673));
#16032=CARTESIAN_POINT('Ctrl Pts',(-17.3748167573771,-15.0783138076581,
10.0036352833029));
#16033=CARTESIAN_POINT('Ctrl Pts',(-17.4024647865506,-15.3864522508245,
9.99135707970488));
#16034=CARTESIAN_POINT('Ctrl Pts',(-17.405,-15.4432562982936,9.98914967135526));
#16035=CARTESIAN_POINT('Ctrl Pts',(-17.405,-15.4999999999999,9.98699999999995));
#16036=CARTESIAN_POINT('Origin',(-15.5,-15.5,-1.713));
#16037=CARTESIAN_POINT('',(-17.405,-15.4999999999999,9.42450000000002));
#16038=CARTESIAN_POINT('',(-17.405,-15.5,9.48699999999995));
#16039=CARTESIAN_POINT('',(-17.405,-15.5,-1.713));
#16040=CARTESIAN_POINT('Ctrl Pts',(-17.405,-15.4999999999999,9.42450000000001));
#16041=CARTESIAN_POINT('Ctrl Pts',(-17.405,-15.4466613264519,9.42652067569103));
#16042=CARTESIAN_POINT('Ctrl Pts',(-17.4027599096894,-15.3932664486905,
9.42859247646646));
#16043=CARTESIAN_POINT('Ctrl Pts',(-17.3770562589371,-15.088400244482,9.44070418700785));
#16044=CARTESIAN_POINT('Ctrl Pts',(-17.3060564179067,-14.8435749018795,
9.45153204731841));
#16045=CARTESIAN_POINT('Ctrl Pts',(-17.075654363384,-14.4013836246713,9.47332338181777));
#16046=CARTESIAN_POINT('Ctrl Pts',(-16.9206199127688,-14.2071364928725,
9.48407317079667));
#16047=CARTESIAN_POINT('Ctrl Pts',(-16.546929902058,-13.8898817511187,9.5042654573752));
#16048=CARTESIAN_POINT('Ctrl Pts',(-16.3323671058024,-13.7691883827222,
9.51308849055973));
#16049=CARTESIAN_POINT('Ctrl Pts',(-15.8607715005188,-13.6124415613253,
9.53371821957476));
#16050=CARTESIAN_POINT('Ctrl Pts',(-15.607190250997,-13.5812680673282,9.54481101264221));
#16051=CARTESIAN_POINT('Ctrl Pts',(-15.1122489846817,-13.6190638884743,
9.56646198667174));
#16052=CARTESIAN_POINT('Ctrl Pts',(-14.8753143328217,-13.6839438427397,
9.57682658211618));
#16053=CARTESIAN_POINT('Ctrl Pts',(-14.4313224334131,-13.9030386696172,
9.59624879993806));
#16054=CARTESIAN_POINT('Ctrl Pts',(-14.2299234575674,-14.0580267748202,
9.60598525050875));
#16055=CARTESIAN_POINT('Ctrl Pts',(-13.9002267209048,-14.4359673346765,
9.62751431850032));
#16056=CARTESIAN_POINT('Ctrl Pts',(-13.7746222022327,-14.6547120499756,
9.63854847159431));
#16057=CARTESIAN_POINT('Ctrl Pts',(-13.6177893545292,-15.1199384076246,
9.65960333896465));
#16058=CARTESIAN_POINT('Ctrl Pts',(-13.5848498401192,-15.3609429627073,
9.66900997345517));
#16059=CARTESIAN_POINT('Ctrl Pts',(-13.6111852189762,-15.8537185271427,
9.6882542362108));
#16060=CARTESIAN_POINT('Ctrl Pts',(-13.6746168216891,-16.1005756101188,
9.69899353220021));
#16061=CARTESIAN_POINT('Ctrl Pts',(-13.8916050354316,-16.5502717829196,
9.72077579013989));
#16062=CARTESIAN_POINT('Ctrl Pts',(-14.0411524564435,-16.7497115841666,
9.73160228379306));
#16063=CARTESIAN_POINT('Ctrl Pts',(-14.4049344021493,-17.0775919354096,
9.75198039781016));
#16064=CARTESIAN_POINT('Ctrl Pts',(-14.6146612252727,-17.2041533666905,
9.76077126969677));
#16065=CARTESIAN_POINT('Ctrl Pts',(-15.0807225085978,-17.3755390853041,
9.78115890238817));
#16066=CARTESIAN_POINT('Ctrl Pts',(-15.3340363632444,-17.414649518979,9.79223999839198));
#16067=CARTESIAN_POINT('Ctrl Pts',(-15.8313968608293,-17.3917694317577,
9.81399680056106));
#16068=CARTESIAN_POINT('Ctrl Pts',(-16.0708559082174,-17.333782344077,9.8244718245063));
#16069=CARTESIAN_POINT('Ctrl Pts',(-16.5194826772159,-17.1284350223924,
9.84409679252898));
#16070=CARTESIAN_POINT('Ctrl Pts',(-16.7235594195928,-16.9812365666504,
9.85348036806906));
#16071=CARTESIAN_POINT('Ctrl Pts',(-17.0644138088265,-16.6155512875477,
9.87478920166968));
#16072=CARTESIAN_POINT('Ctrl Pts',(-17.1974549309092,-16.4002718265706,
9.88585473286657));
#16073=CARTESIAN_POINT('Ctrl Pts',(-17.3644129937763,-15.9524068452289,
9.90647334540993));
#16074=CARTESIAN_POINT('Ctrl Pts',(-17.405,-15.7270401289098,9.91589883992502));
#16075=CARTESIAN_POINT('Ctrl Pts',(-17.405,-15.5,9.92450000000002));
#16076=CARTESIAN_POINT('Ctrl Pts',(-17.405,-15.4999999999999,9.98699999999996));
#16077=CARTESIAN_POINT('Ctrl Pts',(-17.405,-15.683604244378,9.98004435958553));
#16078=CARTESIAN_POINT('Ctrl Pts',(-17.3784600973982,-15.8665326447994,
9.97253383495133));
#16079=CARTESIAN_POINT('Ctrl Pts',(-17.2549772020074,-16.2816926262105,
9.95410511499368));
#16080=CARTESIAN_POINT('Ctrl Pts',(-17.1379301675275,-16.5040765573527,
9.94312026586847));
#16081=CARTESIAN_POINT('Ctrl Pts',(-16.8227314123397,-16.8939633578098,
9.92145573168694));
#16082=CARTESIAN_POINT('Ctrl Pts',(-16.6266061190295,-17.056749276571,9.91128285735042));
#16083=CARTESIAN_POINT('Ctrl Pts',(-16.1910184997219,-17.2917483583643,
9.89222828082777));
#16084=CARTESIAN_POINT('Ctrl Pts',(-15.9575035818148,-17.3650834538561,
9.88201328004444));
#16085=CARTESIAN_POINT('Ctrl Pts',(-15.4661861766118,-17.4212969458065,
9.86052083012306));
#16086=CARTESIAN_POINT('Ctrl Pts',(-15.2126060379952,-17.3999835540545,
9.84942808565165));
#16087=CARTESIAN_POINT('Ctrl Pts',(-14.7343503144704,-17.2616058287939,
9.82850701288154));
#16088=CARTESIAN_POINT('Ctrl Pts',(-14.5136523266074,-17.148207639327,9.81953350173553));
#16089=CARTESIAN_POINT('Ctrl Pts',(-14.1279075199582,-16.8440925289149,
9.79957532961759));
#16090=CARTESIAN_POINT('Ctrl Pts',(-13.9663939196341,-16.6563994788957,
9.78893212097399));
#16091=CARTESIAN_POINT('Ctrl Pts',(-13.7199253192794,-16.2239384011735,
9.76715799238112));
#16092=CARTESIAN_POINT('Ctrl Pts',(-13.6397527520202,-15.9819239268847,
9.7562359903493));
#16093=CARTESIAN_POINT('Ctrl Pts',(-13.5797699101727,-15.4915856352516,
9.73634811467448));
#16094=CARTESIAN_POINT('Ctrl Pts',(-13.5962938465972,-15.2484754744938,
9.72744297672526));
#16095=CARTESIAN_POINT('Ctrl Pts',(-13.7209832734784,-14.7749510096144,
9.70677679433944));
#16096=CARTESIAN_POINT('Ctrl Pts',(-13.8304461678666,-14.5496419268634,
9.6958470114628));
#16097=CARTESIAN_POINT('Ctrl Pts',(-14.1320990097588,-14.1503612026893,
9.67412287885901));
#16098=CARTESIAN_POINT('Ctrl Pts',(-14.3226854240572,-13.9812388909141,
9.66354731343935));
#16099=CARTESIAN_POINT('Ctrl Pts',(-14.7495292931239,-13.7324475034692,
9.64478608875415));
#16100=CARTESIAN_POINT('Ctrl Pts',(-14.9796780285392,-13.6515497085524,
9.63476124109627));
#16101=CARTESIAN_POINT('Ctrl Pts',(-15.4672143701705,-13.5788006729456,
9.61343419203103));
#16102=CARTESIAN_POINT('Ctrl Pts',(-15.7204741931685,-13.5912105377042,
9.60235545961642));
#16103=CARTESIAN_POINT('Ctrl Pts',(-16.204531811323,-13.7127816421253,9.58118058568141));
#16104=CARTESIAN_POINT('Ctrl Pts',(-16.4309078311172,-13.8195490204609,
9.57196759941106));
#16105=CARTESIAN_POINT('Ctrl Pts',(-16.827331201323,-14.1118245911351,9.55222439056537));
#16106=CARTESIAN_POINT('Ctrl Pts',(-16.9943879667994,-14.2935066477241,
9.5416876600686));
#16107=CARTESIAN_POINT('Ctrl Pts',(-17.2557532352398,-14.7183342332122,
9.51987689386206));
#16108=CARTESIAN_POINT('Ctrl Pts',(-17.3442983332949,-14.9593985818345,
9.50880776005274));
#16109=CARTESIAN_POINT('Ctrl Pts',(-17.3976475212624,-15.3066648662753,
9.49448509958961));
#16110=CARTESIAN_POINT('Ctrl Pts',(-17.405,-15.4033638686422,9.49066095121076));
#16111=CARTESIAN_POINT('Ctrl Pts',(-17.405,-15.5,9.48699999999995));
#16112=CARTESIAN_POINT('Origin',(-15.5,-15.5,-1.713));
#16113=CARTESIAN_POINT('',(-17.405,-15.5,8.92450000000001));
#16114=CARTESIAN_POINT('',(-17.405,-15.5,8.98699999999994));
#16115=CARTESIAN_POINT('',(-17.405,-15.5,-1.713));
#16116=CARTESIAN_POINT('Ctrl Pts',(-17.405,-15.5,8.92450000000001));
#16117=CARTESIAN_POINT('Ctrl Pts',(-17.405,-15.409275326029,8.92793700229262));
#16118=CARTESIAN_POINT('Ctrl Pts',(-17.398519492809,-15.3184805274955,8.93151840455227));
#16119=CARTESIAN_POINT('Ctrl Pts',(-17.3492242597744,-14.9763792634779,
8.945556724842));
#16120=CARTESIAN_POINT('Ctrl Pts',(-17.2628017286436,-14.7342827990601,
8.95661853384977));
#16121=CARTESIAN_POINT('Ctrl Pts',(-17.0050165166439,-14.306748335673,8.97845354313614));
#16122=CARTESIAN_POINT('Ctrl Pts',(-16.8394181021722,-14.1234462369798,
8.98901974966593));
#16123=CARTESIAN_POINT('Ctrl Pts',(-16.4458406175058,-13.8279968550024,
9.00882094881983));
#16124=CARTESIAN_POINT('Ctrl Pts',(-16.2210003870653,-13.7194452026138,
9.01796017554389));
#16125=CARTESIAN_POINT('Ctrl Pts',(-15.7384782505255,-13.5933449252129,
9.03906788055439));
#16126=CARTESIAN_POINT('Ctrl Pts',(-15.4851026556293,-13.5785478536479,
9.0501516773565));
#16127=CARTESIAN_POINT('Ctrl Pts',(-14.9965585940993,-13.6468643236345,
9.07152280865702));
#16128=CARTESIAN_POINT('Ctrl Pts',(-14.7654772361706,-13.7257210633924,
9.08163135449816));
#16129=CARTESIAN_POINT('Ctrl Pts',(-14.3362611084979,-13.9708249691623,
9.1004072131015));
#16130=CARTESIAN_POINT('Ctrl Pts',(-14.1441559139415,-14.1382325258434,
9.110899685755));
#16131=CARTESIAN_POINT('Ctrl Pts',(-13.838794743977,-14.5350681676457,9.13261229869945));
#16132=CARTESIAN_POINT('Ctrl Pts',(-13.7272817555302,-14.7596137954321,
9.14355799914543));
#16133=CARTESIAN_POINT('Ctrl Pts',(-13.5985427525879,-15.2321288692101,
9.16427451528865));
#16134=CARTESIAN_POINT('Ctrl Pts',(-13.5799328172441,-15.4749447987811,
9.17322125843685));
#16135=CARTESIAN_POINT('Ctrl Pts',(-13.635611148507,-15.9656408622825,9.19302853849637));
#16136=CARTESIAN_POINT('Ctrl Pts',(-13.71366210364,-16.2083400222125,9.20393007460936));
#16137=CARTESIAN_POINT('Ctrl Pts',(-13.9564334096459,-16.6431144964178,
9.2257109754222));
#16138=CARTESIAN_POINT('Ctrl Pts',(-14.1164652592955,-16.8323493150796,
9.23638018299291));
#16139=CARTESIAN_POINT('Ctrl Pts',(-14.4994156161444,-17.1395315764847,
9.25639342972927));
#16140=CARTESIAN_POINT('Ctrl Pts',(-14.7186656759076,-17.2546375642761,
9.26532089570884));
#16141=CARTESIAN_POINT('Ctrl Pts',(-15.1953865887207,-17.3973296525557,
9.28617482890278));
#16142=CARTESIAN_POINT('Ctrl Pts',(-15.4490001598685,-17.4209476505201,
9.29726903586463));
#16143=CARTESIAN_POINT('Ctrl Pts',(-15.9412261503245,-17.3690277360049,
9.31880123142265));
#16144=CARTESIAN_POINT('Ctrl Pts',(-16.175568605205,-17.2976581050846,9.32905243242355));
#16145=CARTESIAN_POINT('Ctrl Pts',(-16.61501213862,-17.0653840664801,9.348275684104));
#16146=CARTESIAN_POINT('Ctrl Pts',(-16.8137940051543,-16.9027340340602,
9.35842798312882));
#16147=CARTESIAN_POINT('Ctrl Pts',(-17.1324353710775,-16.5130185407986,
9.38016132522746));
#16148=CARTESIAN_POINT('Ctrl Pts',(-17.2507523336409,-16.2911516811955,
9.39115436188346));
#16149=CARTESIAN_POINT('Ctrl Pts',(-17.3774665425925,-15.8732814570085,
9.40975643249182));
#16150=CARTESIAN_POINT('Ctrl Pts',(-17.405,-15.6870089843509,9.41741537483886));
#16151=CARTESIAN_POINT('Ctrl Pts',(-17.405,-15.4999999999999,9.42450000000001));
#16152=CARTESIAN_POINT('Ctrl Pts',(-17.405,-15.5,9.48699999999995));
#16153=CARTESIAN_POINT('Ctrl Pts',(-17.405,-15.644525241093,9.48152482369748));
#16154=CARTESIAN_POINT('Ctrl Pts',(-17.3885555369914,-15.7888822922063,
9.47569634141479));
#16155=CARTESIAN_POINT('Ctrl Pts',(-17.2998877500828,-16.1712951301782,
9.45926969548867));
#16156=CARTESIAN_POINT('Ctrl Pts',(-17.1975903445424,-16.3991170818372,
9.44840144087596));
#16157=CARTESIAN_POINT('Ctrl Pts',(-16.9087708563741,-16.8069302128147,
9.42663476215735));
#16158=CARTESIAN_POINT('Ctrl Pts',(-16.723440169658,-16.9818639361858,9.41595399261335));
#16159=CARTESIAN_POINT('Ctrl Pts',(-16.3048257342699,-17.2434054274864,
9.39688974093776));
#16160=CARTESIAN_POINT('Ctrl Pts',(-16.077809888832,-17.331223199864,9.38727602313356));
#16161=CARTESIAN_POINT('Ctrl Pts',(-15.594132191259,-17.4190668232392,9.36611776864656));
#16162=CARTESIAN_POINT('Ctrl Pts',(-15.3414349406903,-17.4148203408526,
9.35506364569956));
#16163=CARTESIAN_POINT('Ctrl Pts',(-14.8522409502503,-17.3088796253594,
9.33366408356309));
#16164=CARTESIAN_POINT('Ctrl Pts',(-14.6205362430131,-17.2082632388532,
9.32414643406416));
#16165=CARTESIAN_POINT('Ctrl Pts',(-14.2144656677214,-16.9268481307298,
9.30460365539883));
#16166=CARTESIAN_POINT('Ctrl Pts',(-14.0425721856135,-16.7507512830307,
9.29417272431012));
#16167=CARTESIAN_POINT('Ctrl Pts',(-13.7692533807776,-16.3353303098051,
9.27245686610818));
#16168=CARTESIAN_POINT('Ctrl Pts',(-13.6735865683392,-16.0979023164427,
9.26136972349921));
#16169=CARTESIAN_POINT('Ctrl Pts',(-13.5826657913141,-15.6095993801634,
9.24088227222742));
#16170=CARTESIAN_POINT('Ctrl Pts',(-13.5843440818462,-15.3641860826945,
9.23208791148313));
#16171=CARTESIAN_POINT('Ctrl Pts',(-13.68059784426,-14.8838478203405,9.21178554845534));
#16172=CARTESIAN_POINT('Ctrl Pts',(-13.7755756290199,-14.6537037713375,
9.20098942048743));
#16173=CARTESIAN_POINT('Ctrl Pts',(-14.0511332418958,-14.2376577107011,
9.17920091374667));
#16174=CARTESIAN_POINT('Ctrl Pts',(-14.2309465084974,-14.0570001865435,
9.168423982924));
#16175=CARTESIAN_POINT('Ctrl Pts',(-14.6410908924904,-13.7826192882917,
9.1490585839653));
#16176=CARTESIAN_POINT('Ctrl Pts',(-14.8650573151847,-13.6878215260928,
9.13977527055186));
#16177=CARTESIAN_POINT('Ctrl Pts',(-15.3447514535787,-13.5850121306314,
9.11879127499656));
#16178=CARTESIAN_POINT('Ctrl Pts',(-15.596633383431,-13.5811614681987,9.10777281787266));
#16179=CARTESIAN_POINT('Ctrl Pts',(-16.0907406760179,-13.6713557098377,
9.08615832563351));
#16180=CARTESIAN_POINT('Ctrl Pts',(-16.3278520255412,-13.7657721397032,
9.07625894007863));
#16181=CARTESIAN_POINT('Ctrl Pts',(-16.7433789328809,-14.0363858974374,
9.05691852702171));
#16182=CARTESIAN_POINT('Ctrl Pts',(-16.9198464447732,-14.2068750648706,
9.04659999220047));
#16183=CARTESIAN_POINT('Ctrl Pts',(-17.2045925732363,-14.6127415422356,
9.02499615387264));
#16184=CARTESIAN_POINT('Ctrl Pts',(-17.3071205372726,-14.8464033193435,
9.01390162120042));
#16185=CARTESIAN_POINT('Ctrl Pts',(-17.3903396172592,-15.227177625558,8.99765622477507));
#16186=CARTESIAN_POINT('Ctrl Pts',(-17.405,-15.363540262961,8.99216962374751));
#16187=CARTESIAN_POINT('Ctrl Pts',(-17.405,-15.5,8.98699999999994));
#16188=CARTESIAN_POINT('Origin',(-15.5,-15.5,-1.713));
#16189=CARTESIAN_POINT('',(-17.405,-15.5,8.4245));
#16190=CARTESIAN_POINT('',(-17.405,-15.5000000000001,8.48699999999992));
#16191=CARTESIAN_POINT('',(-17.405,-15.5,-1.713));
#16192=CARTESIAN_POINT('Ctrl Pts',(-17.405,-15.5,8.4245));
#16193=CARTESIAN_POINT('Ctrl Pts',(-17.405,-15.3693362200014,8.42945005043016));
#16194=CARTESIAN_POINT('Ctrl Pts',(-17.3915584459371,-15.2387320065154,
8.43469184149533));
#16195=CARTESIAN_POINT('Ctrl Pts',(-17.3129587506065,-14.8626848265213,
8.45065711964764));
#16196=CARTESIAN_POINT('Ctrl Pts',(-17.2124302981695,-14.6278980119052,
8.46175053925174));
#16197=CARTESIAN_POINT('Ctrl Pts',(-16.9310050713234,-14.2191957001966,
8.48338917433258));
#16198=CARTESIAN_POINT('Ctrl Pts',(-16.7558615754538,-14.0470486187207,
8.49374155813311));
#16199=CARTESIAN_POINT('Ctrl Pts',(-16.3431083496375,-13.7732503683779,
8.51314194541293));
#16200=CARTESIAN_POINT('Ctrl Pts',(-16.10760158395,-13.6769965436411,8.52292075310797));
#16201=CARTESIAN_POINT('Ctrl Pts',(-15.614921506734,-13.58213919731,8.54447281247875));
#16202=CARTESIAN_POINT('Ctrl Pts',(-15.3627726883948,-13.5836059425745,
8.55550294451459));
#16203=CARTESIAN_POINT('Ctrl Pts',(-14.8818895105323,-13.6820079646112,
8.57653895404487));
#16204=CARTESIAN_POINT('Ctrl Pts',(-14.6570308346313,-13.7747367447764,
8.58591132001061));
#16205=CARTESIAN_POINT('Ctrl Pts',(-14.2443587524093,-14.0453161543274,
8.60518799033095));
#16206=CARTESIAN_POINT('Ctrl Pts',(-14.0628886413264,-14.22429314795,8.61593749508648));
#16207=CARTESIAN_POINT('Ctrl Pts',(-13.7833699390011,-14.6379403929234,
8.63772176339421));
#16208=CARTESIAN_POINT('Ctrl Pts',(-13.6862146574259,-14.8674191403123,
8.6485403139478));
#16209=CARTESIAN_POINT('Ctrl Pts',(-13.5857011635114,-15.3467664469454,
8.66889830571233));
#16210=CARTESIAN_POINT('Ctrl Pts',(-13.5817741305567,-15.5918085739254,
8.67768878488976));
#16211=CARTESIAN_POINT('Ctrl Pts',(-13.6680606652279,-16.0808563942445,
8.69810309387477));
#16212=CARTESIAN_POINT('Ctrl Pts',(-13.7616155090868,-16.3193911022531,
8.70918596958557));
#16213=CARTESIAN_POINT('Ctrl Pts',(-14.0313990140255,-16.7376546749684,
8.73093219145427));
#16214=CARTESIAN_POINT('Ctrl Pts',(-14.2018673807692,-16.9154322879258,
8.74139562594321));
#16215=CARTESIAN_POINT('Ctrl Pts',(-14.6050603235757,-17.2001034951633,
8.76099881792033));
#16216=CARTESIAN_POINT('Ctrl Pts',(-14.8351557382453,-17.3025719947771,
8.77041669896072));
#16217=CARTESIAN_POINT('Ctrl Pts',(-15.3228295720101,-17.4132202940157,
8.79174976255499));
#16218=CARTESIAN_POINT('Ctrl Pts',(-15.5757225522784,-17.4199127641496,
8.80281244760611));
#16219=CARTESIAN_POINT('Ctrl Pts',(-16.0605729834542,-17.336589793723,8.82402200277566));
#16220=CARTESIAN_POINT('Ctrl Pts',(-16.288521032735,-17.2508562853564,8.83375085279399));
#16221=CARTESIAN_POINT('Ctrl Pts',(-16.7096322391058,-16.9931544551816,
8.85272425326287));
#16222=CARTESIAN_POINT('Ctrl Pts',(-16.8965692920554,-16.8199580436126,
8.86337434157162));
#16223=CARTESIAN_POINT('Ctrl Pts',(-17.1892894534501,-16.4146779656935,
8.88513037498472));
#16224=CARTESIAN_POINT('Ctrl Pts',(-17.2937559827386,-16.1875913998802,
8.89601821398283));
#16225=CARTESIAN_POINT('Ctrl Pts',(-17.3872334019742,-15.800224289686,8.91273774450063));
#16226=CARTESIAN_POINT('Ctrl Pts',(-17.405,-15.6502231589476,8.91880896448446));
#16227=CARTESIAN_POINT('Ctrl Pts',(-17.405,-15.5,8.92450000000001));
#16228=CARTESIAN_POINT('Ctrl Pts',(-17.405,-15.5,8.98699999999994));
#16229=CARTESIAN_POINT('Ctrl Pts',(-17.405,-15.6069532063804,8.98294819799899));
#16230=CARTESIAN_POINT('Ctrl Pts',(-17.3959938933646,-15.7139509549833,
8.97869772460645));
#16231=CARTESIAN_POINT('Ctrl Pts',(-17.3366571088536,-16.0623240399535,
8.96420217194528));
#16232=CARTESIAN_POINT('Ctrl Pts',(-17.2487949895943,-16.2944938491879,
8.95348493605647));
#16233=CARTESIAN_POINT('Ctrl Pts',(-16.9862734772024,-16.7180851373411,
8.93169571590957));
#16234=CARTESIAN_POINT('Ctrl Pts',(-16.8119645569091,-16.9041043960273,
8.92083605432768));
#16235=CARTESIAN_POINT('Ctrl Pts',(-16.4101359120342,-17.1908103010399,
8.90118562039972));
#16236=CARTESIAN_POINT('Ctrl Pts',(-16.1890042445451,-17.2923371627356,
8.89214016817789));
#16237=CARTESIAN_POINT('Ctrl Pts',(-15.7132171293496,-17.4093048847077,
8.87132708352367));
#16238=CARTESIAN_POINT('Ctrl Pts',(-15.4623440480321,-17.4208031583863,
8.86035275800674));
#16239=CARTESIAN_POINT('Ctrl Pts',(-14.9667524644239,-17.3461827321486,
8.83867333615161));
#16240=CARTESIAN_POINT('Ctrl Pts',(-14.7271333943903,-17.2593674662084,
8.82841398151906));
#16241=CARTESIAN_POINT('Ctrl Pts',(-14.3042167827687,-17.0026282822229,
8.80943756151516));
#16242=CARTESIAN_POINT('Ctrl Pts',(-14.1229232827256,-16.8384414931528,
8.79925222991752));
#16243=CARTESIAN_POINT('Ctrl Pts',(-13.8259745669977,-16.443435989778,8.77779294914667));
#16244=CARTESIAN_POINT('Ctrl Pts',(-13.7160577376719,-16.214135444877,8.76670202562747));
#16245=CARTESIAN_POINT('Ctrl Pts',(-13.5931416459568,-15.7314445909808,
8.74572737175581));
#16246=CARTESIAN_POINT('Ctrl Pts',(-13.5792212868598,-15.4832891137937,
8.73671204307076));
#16247=CARTESIAN_POINT('Ctrl Pts',(-13.646465330172,-14.9964612904171,8.71679833861015));
#16248=CARTESIAN_POINT('Ctrl Pts',(-13.7265888079429,-14.7623421438691,
8.70617651589325));
#16249=CARTESIAN_POINT('Ctrl Pts',(-13.9760322448844,-14.3288654728532,
8.684298846273));
#16250=CARTESIAN_POINT('Ctrl Pts',(-14.1462917827891,-14.1356225733931,
8.67325409434886));
#16251=CARTESIAN_POINT('Ctrl Pts',(-14.5420854715896,-13.8357340475546,
8.65323624981342));
#16252=CARTESIAN_POINT('Ctrl Pts',(-14.7606109991447,-13.7278002038347,
8.64434422575922));
#16253=CARTESIAN_POINT('Ctrl Pts',(-15.2326334687793,-13.5976133907746,
8.62369582376294));
#16254=CARTESIAN_POINT('Ctrl Pts',(-15.4823561387463,-13.5789997324337,
8.61277182245205));
#16255=CARTESIAN_POINT('Ctrl Pts',(-15.9790897547409,-13.6390449845805,
8.59104244292473));
#16256=CARTESIAN_POINT('Ctrl Pts',(-16.2211008083728,-13.7187866834218,
8.58045578266087));
#16257=CARTESIAN_POINT('Ctrl Pts',(-16.6506886170301,-13.962686677952,8.56166366504681));
#16258=CARTESIAN_POINT('Ctrl Pts',(-16.8362688360923,-14.1209223401415,
8.55168424624599));
#16259=CARTESIAN_POINT('Ctrl Pts',(-17.1441810272607,-14.505661419594,8.53037410135452));
#16260=CARTESIAN_POINT('Ctrl Pts',(-17.2607621679606,-14.730739908857,8.51929736207643));
#16261=CARTESIAN_POINT('Ctrl Pts',(-17.3799675670468,-15.1439263203452,
8.50103696713371));
#16262=CARTESIAN_POINT('Ctrl Pts',(-17.405,-15.3216860808434,8.49375522239003));
#16263=CARTESIAN_POINT('Ctrl Pts',(-17.405,-15.5000000000001,8.48699999999992));
#16264=CARTESIAN_POINT('Origin',(-15.5,-15.5,-1.713));
#16265=CARTESIAN_POINT('',(-17.405,-15.5000000000001,7.92449999999999));
#16266=CARTESIAN_POINT('',(-17.405,-15.5,7.98699999999992));
#16267=CARTESIAN_POINT('',(-17.405,-15.5,-1.713));
#16268=CARTESIAN_POINT('Ctrl Pts',(-17.405,-15.5000000000001,7.92449999999999));
#16269=CARTESIAN_POINT('Ctrl Pts',(-17.405,-15.3278413248805,7.93102203788868));
#16270=CARTESIAN_POINT('Ctrl Pts',(-17.3816660200934,-15.1561469939484,
7.93803685163428));
#16271=CARTESIAN_POINT('Ctrl Pts',(-17.2680352205322,-14.7475265742745,
7.95600233998613));
#16272=CARTESIAN_POINT('Ctrl Pts',(-17.1534769956326,-14.521136506178,7.96708452120161));
#16273=CARTESIAN_POINT('Ctrl Pts',(-16.848921312095,-14.133273473672,7.98843959911533));
#16274=CARTESIAN_POINT('Ctrl Pts',(-16.6646523308701,-13.9731930129781,
7.99853444759402));
#16275=CARTESIAN_POINT('Ctrl Pts',(-16.2371009035877,-13.7253616488697,
8.01727477877572));
#16276=CARTESIAN_POINT('Ctrl Pts',(-15.9958294371788,-13.6434241389121,
8.02781017335167));
#16277=CARTESIAN_POINT('Ctrl Pts',(-15.4993610024274,-13.5788909397874,
8.04952795264963));
#16278=CARTESIAN_POINT('Ctrl Pts',(-15.2492635663799,-13.5953222638203,
8.06046834792729));
#16279=CARTESIAN_POINT('Ctrl Pts',(-14.7760729185293,-13.7214484695683,
8.08116785133282));
#16280=CARTESIAN_POINT('Ctrl Pts',(-14.5567507407337,-13.8274006779497,
8.09009978680586));
#16281=CARTESIAN_POINT('Ctrl Pts',(-14.1604663446654,-14.1221691213376,
8.10993439565284));
#16282=CARTESIAN_POINT('Ctrl Pts',(-13.989866276221,-14.3116203521669,8.12084295264752));
#16283=CARTESIAN_POINT('Ctrl Pts',(-13.7360278325154,-14.7399496784566,
8.14262174965563));
#16284=CARTESIAN_POINT('Ctrl Pts',(-13.6528638148051,-14.9733341365597,
8.15328224302487));
#16285=CARTESIAN_POINT('Ctrl Pts',(-13.5796822980195,-15.4588708210738,
8.17327690013998));
#16286=CARTESIAN_POINT('Ctrl Pts',(-13.5903664666448,-15.7064344398994,
8.18221919083499));
#16287=CARTESIAN_POINT('Ctrl Pts',(-13.7066735949874,-16.1903551164184,
8.20309588214965));
#16288=CARTESIAN_POINT('Ctrl Pts',(-13.8136966525045,-16.4214026244029,
8.21418969405491));
#16289=CARTESIAN_POINT('Ctrl Pts',(-14.1058795957532,-16.8207346051826,
8.23570864031575));
#16290=CARTESIAN_POINT('Ctrl Pts',(-14.285295796027,-16.9874232356291,8.24594769056184));
#16291=CARTESIAN_POINT('Ctrl Pts',(-14.7071162134803,-17.2507600222599,
8.2651500770754));
#16292=CARTESIAN_POINT('Ctrl Pts',(-14.9479255966595,-17.3409451581515,
8.27534976363324));
#16293=CARTESIAN_POINT('Ctrl Pts',(-15.4452236897676,-17.4204195301753,
8.29710383594769));
#16294=CARTESIAN_POINT('Ctrl Pts',(-15.6964128671484,-17.4111349486261,
8.30809198893899));
#16295=CARTESIAN_POINT('Ctrl Pts',(-16.1733455540415,-17.2982695729136,
8.32895518609092));
#16296=CARTESIAN_POINT('Ctrl Pts',(-16.3952937613701,-17.1987059718314,
8.33806187032001));
#16297=CARTESIAN_POINT('Ctrl Pts',(-16.7995631993888,-16.9155887815292,
8.35762973550196));
#16298=CARTESIAN_POINT('Ctrl Pts',(-16.9754956046028,-16.7311166563296,
8.36846629496478));
#16299=CARTESIAN_POINT('Ctrl Pts',(-17.2418429542412,-16.3096851418179,
8.39025737424484));
#16300=CARTESIAN_POINT('Ctrl Pts',(-17.3317854922963,-16.07808427619,8.40099855981789));
#16301=CARTESIAN_POINT('Ctrl Pts',(-17.395064708575,-15.7246982043178,8.4157702537691));
#16302=CARTESIAN_POINT('Ctrl Pts',(-17.405,-15.6123354215797,8.42024429882621));
#16303=CARTESIAN_POINT('Ctrl Pts',(-17.405,-15.5,8.4245));
#16304=CARTESIAN_POINT('Ctrl Pts',(-17.405,-15.5000000000001,8.48699999999993));
#16305=CARTESIAN_POINT('Ctrl Pts',(-17.405,-15.5689194556288,8.48438906389365));
#16306=CARTESIAN_POINT('Ctrl Pts',(-17.4012601389503,-15.6379154614805,
8.48169342853276));
#16307=CARTESIAN_POINT('Ctrl Pts',(-17.3672272759638,-15.9497398290679,
8.46913593704795));
#16308=CARTESIAN_POINT('Ctrl Pts',(-17.2941571210807,-16.1854094743916,
8.45860964758196));
#16309=CARTESIAN_POINT('Ctrl Pts',(-17.0583701713612,-16.6247714749451,
8.43680771718842));
#16310=CARTESIAN_POINT('Ctrl Pts',(-16.8945577340746,-16.8224418097889,
8.42573624955095));
#16311=CARTESIAN_POINT('Ctrl Pts',(-16.5082695847493,-17.1343575800066,
8.40547067406924));
#16312=CARTESIAN_POINT('Ctrl Pts',(-16.2924627289198,-17.2492106825419,
8.39666591115141));
#16313=CARTESIAN_POINT('Ctrl Pts',(-15.8245395354151,-17.3933751001279,
8.37619683007072));
#16314=CARTESIAN_POINT('Ctrl Pts',(-15.5762512021136,-17.4194718333346,
8.3653355731459));
#16315=CARTESIAN_POINT('Ctrl Pts',(-15.0785906620799,-17.3748649011662,
8.34356564576035));
#16316=CARTESIAN_POINT('Ctrl Pts',(-14.8341899508767,-17.302616329701,8.33287445104456));
#16317=CARTESIAN_POINT('Ctrl Pts',(-14.3976635436967,-17.0722738647,8.31377880768586));
#16318=CARTESIAN_POINT('Ctrl Pts',(-14.2076380393395,-16.9202201791062,
8.30420322719795));
#16319=CARTESIAN_POINT('Ctrl Pts',(-13.8885764919547,-16.5463990738807,
8.283062835803));
#16320=CARTESIAN_POINT('Ctrl Pts',(-13.7652102985012,-16.3259192551278,
8.27201190750953));
#16321=CARTESIAN_POINT('Ctrl Pts',(-13.6106874984648,-15.849658596069,8.25058954401056));
#16322=CARTESIAN_POINT('Ctrl Pts',(-13.5811365169908,-15.5985255332951,
8.24103575486708));
#16323=CARTESIAN_POINT('Ctrl Pts',(-13.6203436374559,-15.1058544769991,
8.22151391712892));
#16324=CARTESIAN_POINT('Ctrl Pts',(-13.6861534992362,-14.8688107237936,
8.21109437019214));
#16325=CARTESIAN_POINT('Ctrl Pts',(-13.9077988343148,-14.4238428734001,
8.18938937763538));
#16326=CARTESIAN_POINT('Ctrl Pts',(-14.0648875575496,-14.2218437822689,
8.17830098279379));
#16327=CARTESIAN_POINT('Ctrl Pts',(-14.4412856912249,-13.8976998272933,
8.15778847333054));
#16328=CARTESIAN_POINT('Ctrl Pts',(-14.6543836160393,-13.7757102786005,
8.14899109291169));
#16329=CARTESIAN_POINT('Ctrl Pts',(-15.1180563845774,-13.6174618962045,
8.12870794468166));
#16330=CARTESIAN_POINT('Ctrl Pts',(-15.3646752632665,-13.5838824110931,
8.11791971726744));
#16331=CARTESIAN_POINT('Ctrl Pts',(-15.8627838435254,-13.6129089088121,
8.09613019057195));
#16332=CARTESIAN_POINT('Ctrl Pts',(-16.1093548999957,-13.6775199454088,
8.08534405511831));
#16333=CARTESIAN_POINT('Ctrl Pts',(-16.5527418706616,-13.8941183052364,
8.06594829962111));
#16334=CARTESIAN_POINT('Ctrl Pts',(-16.7472855708635,-14.0400614101336,
8.05669383732974));
#16335=CARTESIAN_POINT('Ctrl Pts',(-17.0772690199196,-14.4029753150022,
8.03572776622165));
#16336=CARTESIAN_POINT('Ctrl Pts',(-17.207202564757,-14.6186949936846,8.02471352762786));
#16337=CARTESIAN_POINT('Ctrl Pts',(-17.3668134813419,-15.0609521367506,
8.00446806047157));
#16338=CARTESIAN_POINT('Ctrl Pts',(-17.405,-15.2797715610955,7.99534310685587));
#16339=CARTESIAN_POINT('Ctrl Pts',(-17.405,-15.5,7.98699999999992));
#16340=CARTESIAN_POINT('Origin',(-15.5,-15.5,-1.713));
#16341=CARTESIAN_POINT('',(-17.405,-15.5,7.42449999999999));
#16342=CARTESIAN_POINT('',(-17.405,-15.5,7.48699999999992));
#16343=CARTESIAN_POINT('',(-17.405,-15.5,-1.713));
#16344=CARTESIAN_POINT('Ctrl Pts',(-17.405,-15.5000000000001,7.42449999999999));
#16345=CARTESIAN_POINT('Ctrl Pts',(-17.405,-15.2859601869197,7.43260865772304));
#16346=CARTESIAN_POINT('Ctrl Pts',(-17.3689300191348,-15.0731745590006,
7.44145873426585));
#16347=CARTESIAN_POINT('Ctrl Pts',(-17.2155449818739,-14.6349786335938,
7.46141417266776));
#16348=CARTESIAN_POINT('Ctrl Pts',(-17.0875354560809,-14.4178315681802,
7.4724404035471));
#16349=CARTESIAN_POINT('Ctrl Pts',(-16.7607672669738,-14.0516852550486,
7.49345860578802));
#16350=CARTESIAN_POINT('Ctrl Pts',(-16.5675714828386,-13.9039370875409,
7.50279958517755));
#16351=CARTESIAN_POINT('Ctrl Pts',(-16.1262099173826,-13.6832438287778,
7.52210674027187));
#16352=CARTESIAN_POINT('Ctrl Pts',(-15.8802588412845,-13.6163539874434,
7.53286575497432));
#16353=CARTESIAN_POINT('Ctrl Pts',(-15.3822323784215,-13.5826948657237,
7.55465168948277));
#16354=CARTESIAN_POINT('Ctrl Pts',(-15.1350938622725,-13.6140566743586,
7.56546264819445));
#16355=CARTESIAN_POINT('Ctrl Pts',(-14.6701450480656,-13.7681179537064,
7.58580161644495));
#16356=CARTESIAN_POINT('Ctrl Pts',(-14.4562443785121,-13.8879677841051,
7.59459260542679));
#16357=CARTESIAN_POINT('Ctrl Pts',(-14.076872315963,-14.2084654789811,7.61503202698809));
#16358=CARTESIAN_POINT('Ctrl Pts',(-13.917761136657,-14.4091925780489,7.62611646953724));
#16359=CARTESIAN_POINT('Ctrl Pts',(-13.6918725906919,-14.8525296745866,
7.64785249145431));
#16360=CARTESIAN_POINT('Ctrl Pts',(-13.6238888493654,-15.089185426922,7.65830488708587));
#16361=CARTESIAN_POINT('Ctrl Pts',(-13.5804095704248,-15.5809930040761,
7.67788745467378));
#16362=CARTESIAN_POINT('Ctrl Pts',(-13.6075392032479,-15.8316550604089,
7.68733863994873));
#16363=CARTESIAN_POINT('Ctrl Pts',(-13.7572048353041,-16.3089652109285,
7.70869452498207));
#16364=CARTESIAN_POINT('Ctrl Pts',(-13.8785477285808,-16.5308492590566,
7.71975439676735));
#16365=CARTESIAN_POINT('Ctrl Pts',(-14.1942719736145,-16.9079615850459,
7.74094647799673));
#16366=CARTESIAN_POINT('Ctrl Pts',(-14.3829499933764,-17.0618712024457,
7.75063517031373));
#16367=CARTESIAN_POINT('Ctrl Pts',(-14.8173920364941,-17.2963209333944,
7.76963963414216));
#16368=CARTESIAN_POINT('Ctrl Pts',(-15.0610947982815,-17.3708446298938,
7.78030029738747));
#16369=CARTESIAN_POINT('Ctrl Pts',(-15.5585256515928,-17.4201228531586,
7.80206017723487));
#16370=CARTESIAN_POINT('Ctrl Pts',(-15.8072711156938,-17.39628309016,7.81294143113256));
#16371=CARTESIAN_POINT('Ctrl Pts',(-16.2764462266497,-17.2563443110142,
7.83346527675619));
#16372=CARTESIAN_POINT('Ctrl Pts',(-16.493071388795,-17.1435995165235,7.84228813470852));
#16373=CARTESIAN_POINT('Ctrl Pts',(-16.8822650416203,-16.8353316053453,
7.86247906509631));
#16374=CARTESIAN_POINT('Ctrl Pts',(-17.0480504967237,-16.6389867478324,
7.87354347288548));
#16375=CARTESIAN_POINT('Ctrl Pts',(-17.2880064817722,-16.2013715692635,
7.89537041314125));
#16376=CARTESIAN_POINT('Ctrl Pts',(-17.3632254230871,-15.9661516439027,
7.90592666430032));
#16377=CARTESIAN_POINT('Ctrl Pts',(-17.4006389639305,-15.6489266856316,
7.9187626941778));
#16378=CARTESIAN_POINT('Ctrl Pts',(-17.405,-15.574423595628,7.92168054573687));
#16379=CARTESIAN_POINT('Ctrl Pts',(-17.405,-15.5000000000001,7.92449999999999));
#16380=CARTESIAN_POINT('Ctrl Pts',(-17.405,-15.5,7.98699999999992));
#16381=CARTESIAN_POINT('Ctrl Pts',(-17.405,-15.532209736732,7.98577977032979));
#16382=CARTESIAN_POINT('Ctrl Pts',(-17.4041831077522,-15.5644482771286,
7.9845405821808));
#16383=CARTESIAN_POINT('Ctrl Pts',(-17.3902066369061,-15.839474090864,7.97381584128779));
#16384=CARTESIAN_POINT('Ctrl Pts',(-17.3315088500334,-16.0776482928075,
7.96350902576525));
#16385=CARTESIAN_POINT('Ctrl Pts',(-17.1237985933374,-16.5276682568169,
7.94191743130374));
#16386=CARTESIAN_POINT('Ctrl Pts',(-16.9733813555449,-16.7336858868427,
7.93082271913725));
#16387=CARTESIAN_POINT('Ctrl Pts',(-16.6067956491012,-17.0696781001648,
7.91007597174301));
#16388=CARTESIAN_POINT('Ctrl Pts',(-16.3962887405343,-17.1986907762383,
7.901207731432));
#16389=CARTESIAN_POINT('Ctrl Pts',(-15.9368085129371,-17.3704762421015,
7.88110798394306));
#16390=CARTESIAN_POINT('Ctrl Pts',(-15.6920027968328,-17.411178820638,7.87039907247744));
#16391=CARTESIAN_POINT('Ctrl Pts',(-15.1939245631539,-17.3971187727929,
7.8486108732789));
#16392=CARTESIAN_POINT('Ctrl Pts',(-14.9454974477225,-17.3399153220138,
7.83774354539477));
#16393=CARTESIAN_POINT('Ctrl Pts',(-14.4956487774217,-17.1366061828828,
7.81806512587155));
#16394=CARTESIAN_POINT('Ctrl Pts',(-14.2967173925019,-16.9964370779171,
7.80903898604087));
#16395=CARTESIAN_POINT('Ctrl Pts',(-13.9565177536094,-16.6439111116339,
7.78824299908806));
#16396=CARTESIAN_POINT('Ctrl Pts',(-13.8205296831303,-16.4328694086849,
7.77727355415141));
#16397=CARTESIAN_POINT('Ctrl Pts',(-13.635959276609,-15.9670032617552,7.7555877658196));
#16398=CARTESIAN_POINT('Ctrl Pts',(-13.5905662864574,-15.7162261608564,
7.74528846041283));
#16399=CARTESIAN_POINT('Ctrl Pts',(-13.599927086301,-15.2216539588205,7.72634740656811));
#16400=CARTESIAN_POINT('Ctrl Pts',(-13.6507049183005,-14.9824695442845,
7.71617554763647));
#16401=CARTESIAN_POINT('Ctrl Pts',(-13.8428022508102,-14.5273301187568,
7.69473149816027));
#16402=CARTESIAN_POINT('Ctrl Pts',(-13.9856920186994,-14.317093015566,7.68364157881967));
#16403=CARTESIAN_POINT('Ctrl Pts',(-14.3411746028942,-13.9680431210495,
7.66264300629398));
#16404=CARTESIAN_POINT('Ctrl Pts',(-14.5488518054332,-13.8311442236975,
7.65360753257075));
#16405=CARTESIAN_POINT('Ctrl Pts',(-15.0036218345933,-13.6445446066163,
7.63371383050773));
#16406=CARTESIAN_POINT('Ctrl Pts',(-15.2462142286056,-13.5961399934897,
7.62310173978103));
#16407=CARTESIAN_POINT('Ctrl Pts',(-15.7461742493181,-13.5938550022295,
7.60123122268949));
#16408=CARTESIAN_POINT('Ctrl Pts',(-15.9987330092648,-13.6438552027474,
7.59018315794992));
#16409=CARTESIAN_POINT('Ctrl Pts',(-16.4569491101971,-13.8351696420944,
7.57013870909023));
#16410=CARTESIAN_POINT('Ctrl Pts',(-16.66017366989,-13.9698316825174,7.56125974628438));
#16411=CARTESIAN_POINT('Ctrl Pts',(-17.0100084290185,-14.3123994329133,
7.54063027323432));
#16412=CARTESIAN_POINT('Ctrl Pts',(-17.1516134171614,-14.5188338184068,
7.52971251662349));
#16413=CARTESIAN_POINT('Ctrl Pts',(-17.3494687636066,-14.9783214237974,
7.50797780042861));
#16414=CARTESIAN_POINT('Ctrl Pts',(-17.4022393975719,-15.227612456327,7.49737947654021));
#16415=CARTESIAN_POINT('Ctrl Pts',(-17.4049648675835,-15.4866391454631,
7.48750692938117));
#16416=CARTESIAN_POINT('Ctrl Pts',(-17.405,-15.4933203150895,7.48725305235433));
#16417=CARTESIAN_POINT('Ctrl Pts',(-17.405,-15.5,7.48699999999992));
#16418=CARTESIAN_POINT('Origin',(-15.5,-15.5,-1.713));
#16419=CARTESIAN_POINT('',(-17.405,-15.5000000009028,6.92449999993158));
#16420=CARTESIAN_POINT('',(-17.405,-15.5,6.98699999999991));
#16421=CARTESIAN_POINT('',(-17.405,-15.5,-1.713));
#16422=CARTESIAN_POINT('Ctrl Pts',(-17.405,-15.5000000018056,6.92449999993158));
#16423=CARTESIAN_POINT('Ctrl Pts',(-17.4050000000007,-15.4993165450942,
6.92452589192082));
#16424=CARTESIAN_POINT('Ctrl Pts',(-17.4049996321956,-15.4986330720564,
6.92455179257323));
#16425=CARTESIAN_POINT('Ctrl Pts',(-17.4047272898079,-15.245605544446,6.93414341278151));
#16426=CARTESIAN_POINT('Ctrl Pts',(-17.3543192201274,-14.9958416071321,
6.9447079775017));
#16427=CARTESIAN_POINT('Ctrl Pts',(-17.1607411027068,-14.5343054481261,
6.96642674815675));
#16428=CARTESIAN_POINT('Ctrl Pts',(-17.0209296753586,-14.326370698519,6.97736211513677));
#16429=CARTESIAN_POINT('Ctrl Pts',(-16.6741899445924,-13.980587243007,6.99804571627696));
#16430=CARTESIAN_POINT('Ctrl Pts',(-16.4723615303824,-13.8441490441949,
7.00696449998315));
#16431=CARTESIAN_POINT('Ctrl Pts',(-16.0183602662677,-13.6495751788062,
7.02682457277907));
#16432=CARTESIAN_POINT('Ctrl Pts',(-15.7688428179189,-13.5972454552154,
7.03773959676634));
#16433=CARTESIAN_POINT('Ctrl Pts',(-15.2710283860677,-13.5929566539516,
7.05951625607742));
#16434=CARTESIAN_POINT('Ctrl Pts',(-15.0275172627361,-13.638275717184,7.07016853618816));
#16435=CARTESIAN_POINT('Ctrl Pts',(-14.5708371583004,-13.8189161112692,
7.09014579360003));
#16436=CARTESIAN_POINT('Ctrl Pts',(-14.3620213984788,-13.9526166083722,
7.09910262354388));
#16437=CARTESIAN_POINT('Ctrl Pts',(-14.0020253277836,-14.296403346199,7.12000052747168));
#16438=CARTESIAN_POINT('Ctrl Pts',(-13.8560796735194,-14.5049667163631,
7.1310938784775));
#16439=CARTESIAN_POINT('Ctrl Pts',(-13.6576577760441,-14.9581002563818,
7.15260026980298));
#16440=CARTESIAN_POINT('Ctrl Pts',(-13.603677776513,-15.1969076419803,7.16282788407705));
#16441=CARTESIAN_POINT('Ctrl Pts',(-13.587861043887,-15.6941342999381,7.18201070487947));
#16442=CARTESIAN_POINT('Ctrl Pts',(-13.6309452992921,-15.9479281211301,
7.19225545851312));
#16443=CARTESIAN_POINT('Ctrl Pts',(-13.8123031142063,-16.4179614599662,
7.21402884956801));
#16444=CARTESIAN_POINT('Ctrl Pts',(-13.9465467660043,-16.6303806971777,
7.22501232645237));
#16445=CARTESIAN_POINT('Ctrl Pts',(-14.2837864249233,-16.9859346325971,
7.24585828314302));
#16446=CARTESIAN_POINT('Ctrl Pts',(-14.4814296775109,-17.1277830688267,
7.25494311800115));
#16447=CARTESIAN_POINT('Ctrl Pts',(-14.9294025575922,-17.3349866726149,
7.27453948195923));
#16448=CARTESIAN_POINT('Ctrl Pts',(-15.1773104399173,-17.3943623235028,
7.28538409623418));
#16449=CARTESIAN_POINT('Ctrl Pts',(-15.675444267082,-17.4127966111112,7.30717472734376));
#16450=CARTESIAN_POINT('Ctrl Pts',(-15.9208011461287,-17.3741693632993,
7.31790774917433));
#16451=CARTESIAN_POINT('Ctrl Pts',(-16.3815184534768,-17.2063427592322,
7.33806161213794));
#16452=CARTESIAN_POINT('Ctrl Pts',(-16.5927821005162,-17.0794014782496,
7.346901104432));
#16453=CARTESIAN_POINT('Ctrl Pts',(-16.962269571994,-16.7468831279773,7.36757971660608));
#16454=CARTESIAN_POINT('Ctrl Pts',(-17.1146586683044,-16.5420253559275,
7.37867361787087));
#16455=CARTESIAN_POINT('Ctrl Pts',(-17.3264778968817,-16.093447168092,7.40030046478855));
#16456=CARTESIAN_POINT('Ctrl Pts',(-17.3872685002348,-15.8555835898382,
7.41064128732047));
#16457=CARTESIAN_POINT('Ctrl Pts',(-17.4038899094754,-15.5751324644401,
7.42162941084344));
#16458=CARTESIAN_POINT('Ctrl Pts',(-17.405,-15.5375478446883,7.42307754211034));
#16459=CARTESIAN_POINT('Ctrl Pts',(-17.405,-15.5000000000001,7.42449999999999));
#16460=CARTESIAN_POINT('Ctrl Pts',(-17.405,-15.5,7.48699999999992));
#16461=CARTESIAN_POINT('Ctrl Pts',(-17.405,-15.7347872455801,7.47810534911817));
#16462=CARTESIAN_POINT('Ctrl Pts',(-17.3615945711204,-15.9676689740826,
7.4683335115242));
#16463=CARTESIAN_POINT('Ctrl Pts',(-17.186386324715,-16.4209223251271,7.44733031644295));
#16464=CARTESIAN_POINT('Ctrl Pts',(-17.0505427522955,-16.6348205435384,
7.43625581612895));
#16465=CARTESIAN_POINT('Ctrl Pts',(-16.7055108783205,-16.9958209729757,
7.4150330917345));
#16466=CARTESIAN_POINT('Ctrl Pts',(-16.5004180729049,-17.1400882671737,
7.40576282033707));
#16467=CARTESIAN_POINT('Ctrl Pts',(-16.0500445276086,-17.3401676914711,
7.38606144040285));
#16468=CARTESIAN_POINT('Ctrl Pts',(-15.8096683757708,-17.395482444622,7.37554629815274));
#16469=CARTESIAN_POINT('Ctrl Pts',(-15.3114950305751,-17.412602840006,7.35375393834541));
#16470=CARTESIAN_POINT('Ctrl Pts',(-15.0583476117071,-17.3704389219874,
7.34268012299687));
#16471=CARTESIAN_POINT('Ctrl Pts',(-14.5944564284417,-17.193449456036,7.32238742031684));
#16472=CARTESIAN_POINT('Ctrl Pts',(-14.3865677951402,-17.0646250499273,
7.31358744261619));
#16473=CARTESIAN_POINT('Ctrl Pts',(-14.0266526607683,-16.7326405909047,
7.29313842501508));
#16474=CARTESIAN_POINT('Ctrl Pts',(-13.8792830440329,-16.5312238716456,
7.28228467155956));
#16475=CARTESIAN_POINT('Ctrl Pts',(-13.6675732369669,-16.0787216942403,
7.26051156200427));
#16476=CARTESIAN_POINT('Ctrl Pts',(-13.607098221749,-15.8311399539857,7.24980948045646));
#16477=CARTESIAN_POINT('Ctrl Pts',(-13.58664223745,-15.3380197430459,7.23068075683691));
#16478=CARTESIAN_POINT('Ctrl Pts',(-13.6224829650516,-15.0973368538402,
7.22114444460773));
#16479=CARTESIAN_POINT('Ctrl Pts',(-13.7850502774532,-14.6336626550652,
7.20002295329454));
#16480=CARTESIAN_POINT('Ctrl Pts',(-13.9134974868911,-14.4162086949334,
7.18897552292067));
#16481=CARTESIAN_POINT('Ctrl Pts',(-14.2474727228465,-14.0429233005055,
7.16752923016414));
#16482=CARTESIAN_POINT('Ctrl Pts',(-14.4498931260941,-13.8909154772963,
7.15793643367915));
#16483=CARTESIAN_POINT('Ctrl Pts',(-14.8956570181038,-13.6770378253324,
7.13843670087031));
#16484=CARTESIAN_POINT('Ctrl Pts',(-15.1335716879282,-13.6147594565805,
7.12802923499873));
#16485=CARTESIAN_POINT('Ctrl Pts',(-15.6294813482876,-13.5826035126581,
7.10633589902499));
#16486=CARTESIAN_POINT('Ctrl Pts',(-15.8829894175019,-13.6167831150686,
7.09524630719585));
#16487=CARTESIAN_POINT('Ctrl Pts',(-16.3525063151051,-13.7790877500325,
7.07470751027532));
#16488=CARTESIAN_POINT('Ctrl Pts',(-16.5652284844368,-13.9020030374803,
7.065906024606));
#16489=CARTESIAN_POINT('Ctrl Pts',(-16.9351884517455,-14.2232753518093,
7.04564312130783));
#16490=CARTESIAN_POINT('Ctrl Pts',(-17.0881738164499,-14.4194981933583,
7.03486330293791));
#16491=CARTESIAN_POINT('Ctrl Pts',(-17.3135468307644,-14.8645672137614,
7.01307294487737));
#16492=CARTESIAN_POINT('Ctrl Pts',(-17.3816998785812,-15.1101868669613,
7.00227725882102));
#16493=CARTESIAN_POINT('Ctrl Pts',(-17.403334109118,-15.4079593231243,6.99052329439176));
#16494=CARTESIAN_POINT('Ctrl Pts',(-17.405,-15.4540028611883,6.98874254989983));
#16495=CARTESIAN_POINT('Ctrl Pts',(-17.405,-15.4999999999999,6.98699999999991));
#16496=CARTESIAN_POINT('Origin',(-15.5,-15.5,-1.713));
#16497=CARTESIAN_POINT('',(-17.405,-15.5,6.42449999999997));
#16498=CARTESIAN_POINT('',(-17.405,-15.5,6.48699999999991));
#16499=CARTESIAN_POINT('',(-17.405,-15.5,-1.713));
#16500=CARTESIAN_POINT('Ctrl Pts',(-17.405,-15.4999999999999,6.42449999999997));
#16501=CARTESIAN_POINT('Ctrl Pts',(-17.405,-15.4601322430178,6.42601034515914));
#16502=CARTESIAN_POINT('Ctrl Pts',(-17.4037484985812,-15.420226760854,6.42754949266624));
#16503=CARTESIAN_POINT('Ctrl Pts',(-17.3853827382776,-15.1284149916749,
6.4390061543191));
#16504=CARTESIAN_POINT('Ctrl Pts',(-17.3196132846632,-14.8821582325296,
6.44977384181169));
#16505=CARTESIAN_POINT('Ctrl Pts',(-17.0984664394437,-14.4347306341274,
6.47156111605405));
#16506=CARTESIAN_POINT('Ctrl Pts',(-16.9472105586335,-14.2368744594976,
6.48236498368003));
#16507=CARTESIAN_POINT('Ctrl Pts',(-16.5803702499558,-13.912257525636,6.5026863601263));
#16508=CARTESIAN_POINT('Ctrl Pts',(-16.3691697008814,-13.7874961889225,
6.51147857826408));
#16509=CARTESIAN_POINT('Ctrl Pts',(-15.9013957690298,-13.6205861373532,
6.53194112996362));
#16510=CARTESIAN_POINT('Ctrl Pts',(-15.6479745696036,-13.5839087567736,
6.54302692171455));
#16511=CARTESIAN_POINT('Ctrl Pts',(-15.1513086183574,-13.6113697582875,
6.56475334127912));
#16512=CARTESIAN_POINT('Ctrl Pts',(-14.912601829198,-13.671478039929,6.57519545804024));
#16513=CARTESIAN_POINT('Ctrl Pts',(-14.4653810695128,-13.8810306020189,
6.5947589208436));
#16514=CARTESIAN_POINT('Ctrl Pts',(-14.2621189473946,-14.0305901642359,
6.60424165704099));
#16515=CARTESIAN_POINT('Ctrl Pts',(-13.924637934564,-14.4000201554789,6.62561857146581));
#16516=CARTESIAN_POINT('Ctrl Pts',(-13.79385298758,-14.6163813593607,6.63667573561485));
#16517=CARTESIAN_POINT('Ctrl Pts',(-13.6265497449183,-15.0787563566687,
6.65785159366709));
#16518=CARTESIAN_POINT('Ctrl Pts',(-13.5883173202284,-15.3191853793069,
6.66750387599365));
#16519=CARTESIAN_POINT('Ctrl Pts',(-13.6039452571242,-15.8125714288761,
6.68653707027394));
#16520=CARTESIAN_POINT('Ctrl Pts',(-13.6619870155715,-16.0607208315224,
6.6972074362341));
#16521=CARTESIAN_POINT('Ctrl Pts',(-13.8693367441029,-16.5154799558981,
6.71897068289104));
#16522=CARTESIAN_POINT('Ctrl Pts',(-14.0148996961614,-16.7185021911561,
6.72984574366513));
#16523=CARTESIAN_POINT('Ctrl Pts',(-14.3716324066437,-17.0538459441022,
6.75035241751871));
#16524=CARTESIAN_POINT('Ctrl Pts',(-14.5780288600434,-17.1845225613327,
6.75916880402621));
#16525=CARTESIAN_POINT('Ctrl Pts',(-15.0401307441502,-17.3660783945052,
6.77938323465207));
#16526=CARTESIAN_POINT('Ctrl Pts',(-15.2931160658331,-17.4107358839109,
6.79044995913515));
#16527=CARTESIAN_POINT('Ctrl Pts',(-15.7919046780419,-17.3983278051984,
6.81226923350999));
#16528=CARTESIAN_POINT('Ctrl Pts',(-16.0330075000311,-17.3452038021689,
6.82281616360576));
#16529=CARTESIAN_POINT('Ctrl Pts',(-16.4847932651915,-17.1494192766576,
6.84257932043693));
#16530=CARTESIAN_POINT('Ctrl Pts',(-16.690711503981,-17.0075201088409,6.85176618727098));
#16531=CARTESIAN_POINT('Ctrl Pts',(-17.0391100613201,-16.650333546496,6.87291806459168));
#16532=CARTESIAN_POINT('Ctrl Pts',(-17.1772184238653,-16.4375824178345,
6.88399864479192));
#16533=CARTESIAN_POINT('Ctrl Pts',(-17.3592350532944,-15.9800551998517,
6.90531266528233));
#16534=CARTESIAN_POINT('Ctrl Pts',(-17.4049999997715,-15.7410811218703,
6.91536691268471));
#16535=CARTESIAN_POINT('Ctrl Pts',(-17.405,-15.5000000018056,6.92449999993158));
#16536=CARTESIAN_POINT('Ctrl Pts',(-17.405,-15.4999999999999,6.98699999999991));
#16537=CARTESIAN_POINT('Ctrl Pts',(-17.405,-15.6943874704945,6.97963584918515));
#16538=CARTESIAN_POINT('Ctrl Pts',(-17.3752506427565,-15.8878971634581,
6.97165426613153));
#16539=CARTESIAN_POINT('Ctrl Pts',(-17.2414283784515,-16.3115578174224,
6.95267736232273));
#16540=CARTESIAN_POINT('Ctrl Pts',(-17.120368366469,-16.5322806509859,6.94166766910084));
#16541=CARTESIAN_POINT('Ctrl Pts',(-16.7975501002715,-16.9175902999785,
6.92000987918617));
#16542=CARTESIAN_POINT('Ctrl Pts',(-16.5977824941516,-17.0773521697487,
6.91002198137144));
#16543=CARTESIAN_POINT('Ctrl Pts',(-16.156625631238,-17.3046970326897,6.89072378089403));
#16544=CARTESIAN_POINT('Ctrl Pts',(-15.9212944056835,-17.3736536130528,
6.88042932658281));
#16545=CARTESIAN_POINT('Ctrl Pts',(-15.4280081963133,-17.4203124218493,
6.85885075224467));
#16546=CARTESIAN_POINT('Ctrl Pts',(-15.174381278281,-17.3938754826517,6.84775596142961));
#16547=CARTESIAN_POINT('Ctrl Pts',(-14.69955590838,-17.2459242149106,6.82698494787315));
#16548=CARTESIAN_POINT('Ctrl Pts',(-14.4820651847725,-17.1287321615361,
6.81810481278379));
#16549=CARTESIAN_POINT('Ctrl Pts',(-14.102551540606,-16.8177953917989,6.79802449941344));
#16550=CARTESIAN_POINT('Ctrl Pts',(-13.9443589834925,-16.6266828292324,
6.78732438512114));
#16551=CARTESIAN_POINT('Ctrl Pts',(-13.7061578526639,-16.1891108490807,
6.76553746402708));
#16552=CARTESIAN_POINT('Ctrl Pts',(-13.6307204217205,-15.9455969914062,
6.75466222770199));
#16553=CARTESIAN_POINT('Ctrl Pts',(-13.5803266843897,-15.4544806575515,
6.73495461221655));
#16554=CARTESIAN_POINT('Ctrl Pts',(-13.6015021726823,-15.2120161132821,
6.72594783691514));
#16555=CARTESIAN_POINT('Ctrl Pts',(-13.735237407317,-14.7407603202715,6.70516974829986));
#16556=CARTESIAN_POINT('Ctrl Pts',(-13.8492739824694,-14.5171820856897,
6.6942054998984));
#16557=CARTESIAN_POINT('Ctrl Pts',(-14.1591310117816,-14.1234803305985,
6.67251327609788));
#16558=CARTESIAN_POINT('Ctrl Pts',(-14.3530787555558,-13.9581645755139,
6.66217153300273));
#16559=CARTESIAN_POINT('Ctrl Pts',(-14.7852233534807,-13.717638997849,6.64326756983889));
#16560=CARTESIAN_POINT('Ctrl Pts',(-15.0174283305894,-13.6412861257118,
6.63310987180263));
#16561=CARTESIAN_POINT('Ctrl Pts',(-15.507270799116,-13.5784654785805,6.61168194229578));
#16562=CARTESIAN_POINT('Ctrl Pts',(-15.7607595796635,-13.5962252141327,
6.60059319424033));
#16563=CARTESIAN_POINT('Ctrl Pts',(-16.2413554964388,-13.7279224646686,
6.57956975081185));
#16564=CARTESIAN_POINT('Ctrl Pts',(-16.4643034860068,-13.8386814298334,
6.57051235094214));
#16565=CARTESIAN_POINT('Ctrl Pts',(-16.8543319185472,-14.1380699108652,
6.55063954926042));
#16566=CARTESIAN_POINT('Ctrl Pts',(-17.0180921883204,-14.3233740897399,
6.54003770056315));
#16567=CARTESIAN_POINT('Ctrl Pts',(-17.2713800244962,-14.7542397872394,
6.51817485901714));
#16568=CARTESIAN_POINT('Ctrl Pts',(-17.3551426119534,-14.9975970924926,
6.50712346346707));
#16569=CARTESIAN_POINT('Ctrl Pts',(-17.3995286879098,-15.3332027678794,
6.49343859564043));
#16570=CARTESIAN_POINT('Ctrl Pts',(-17.405,-15.416638718226,6.49015804845609));
#16571=CARTESIAN_POINT('Ctrl Pts',(-17.405,-15.4999999999999,6.48699999999991));
#16572=CARTESIAN_POINT('Origin',(-15.5,-15.5,-1.713));
#16573=CARTESIAN_POINT('',(-17.405,-15.5,5.92449999999997));
#16574=CARTESIAN_POINT('',(-17.405,-15.5000000034284,5.98699999974014));
#16575=CARTESIAN_POINT('',(-17.405,-15.5,-1.713));
#16576=CARTESIAN_POINT('Ctrl Pts',(-17.405,-15.5,5.92449999999997));
#16577=CARTESIAN_POINT('Ctrl Pts',(-17.405,-15.4144176700989,5.92774219036784));
#16578=CARTESIAN_POINT('Ctrl Pts',(-17.3992332699381,-15.3287564795742,
5.93111349973546));
#16579=CARTESIAN_POINT('Ctrl Pts',(-17.3546716311612,-15.0006921244555,
5.94451651307743));
#16580=CARTESIAN_POINT('Ctrl Pts',(-17.2751038305769,-14.7664430467097,
5.95513110417249));
#16581=CARTESIAN_POINT('Ctrl Pts',(-17.0267333284629,-14.3324868603746,
5.97700347217566));
#16582=CARTESIAN_POINT('Ctrl Pts',(-16.8569786447406,-14.1388871358369,
5.98805069971181));
#16583=CARTESIAN_POINT('Ctrl Pts',(-16.4619306836403,-13.8380453788742,
6.00808834558228));
#16584=CARTESIAN_POINT('Ctrl Pts',(-16.2436228778207,-13.7295663669768,
6.01697056527465));
#16585=CARTESIAN_POINT('Ctrl Pts',(-15.7719223056613,-13.5982668894319,
6.03760488601653));
#16586=CARTESIAN_POINT('Ctrl Pts',(-15.5223056300077,-13.5790558352873,
6.04852425061521));
#16587=CARTESIAN_POINT('Ctrl Pts',(-15.0352776596755,-13.6367139569718,
6.06982906121628));
#16588=CARTESIAN_POINT('Ctrl Pts',(-14.8021355362915,-13.7109192081023,
6.0800277543179));
#16589=CARTESIAN_POINT('Ctrl Pts',(-14.3675310337485,-13.9475127920323,
6.09903932485781));
#16590=CARTESIAN_POINT('Ctrl Pts',(-14.1720287921778,-14.1110291910389,
6.10925947498833));
#16591=CARTESIAN_POINT('Ctrl Pts',(-13.8583617609821,-14.5020202981999,
6.13093234231348));
#16592=CARTESIAN_POINT('Ctrl Pts',(-13.7421793491084,-14.7247517553509,
6.1419114458153));
#16593=CARTESIAN_POINT('Ctrl Pts',(-13.6041850136687,-15.1949217251059,
6.16274155542265));
#16594=CARTESIAN_POINT('Ctrl Pts',(-13.5808290435917,-15.4370968267385,
6.17180703306081));
#16595=CARTESIAN_POINT('Ctrl Pts',(-13.6267406199668,-15.9285535022321,
6.19142950699013));
#16596=CARTESIAN_POINT('Ctrl Pts',(-13.6999541275731,-16.1727358500583,
6.20228142607045));
#16597=CARTESIAN_POINT('Ctrl Pts',(-13.9342528540802,-16.612643260009,6.22407146787201));
#16598=CARTESIAN_POINT('Ctrl Pts',(-14.0908682124153,-16.8053351301606,
6.23479691554574));
#16599=CARTESIAN_POINT('Ctrl Pts',(-14.4674616885799,-17.119446886757,6.25493363903315));
#16600=CARTESIAN_POINT('Ctrl Pts',(-14.6834759111022,-17.2383997168824,
6.26378153591858));
#16601=CARTESIAN_POINT('Ctrl Pts',(-15.1566843563942,-17.3907795398349,
6.28448181786488));
#16602=CARTESIAN_POINT('Ctrl Pts',(-15.4102989723853,-17.419598005697,6.29557607053292));
#16603=CARTESIAN_POINT('Ctrl Pts',(-15.9044371223974,-17.3773918906524,
6.3171919126157));
#16604=CARTESIAN_POINT('Ctrl Pts',(-16.1405836197149,-17.3104815732564,
6.3275220306086));
#16605=CARTESIAN_POINT('Ctrl Pts',(-16.5831726506165,-17.0872896027469,
6.34688288060429));
#16606=CARTESIAN_POINT('Ctrl Pts',(-16.7837641373552,-16.9299401273163,
6.35674048961191));
#16607=CARTESIAN_POINT('Ctrl Pts',(-17.1100623193184,-16.5483409084119,
6.37833382769666));
#16608=CARTESIAN_POINT('Ctrl Pts',(-17.2334173550748,-16.3286040401448,
6.38935636610198));
#16609=CARTESIAN_POINT('Ctrl Pts',(-17.3733223438246,-15.9001673121539,
6.40864724907353));
#16610=CARTESIAN_POINT('Ctrl Pts',(-17.405,-15.700587196877,6.41690097952011));
#16611=CARTESIAN_POINT('Ctrl Pts',(-17.405,-15.4999999999999,6.42449999999997));
#16612=CARTESIAN_POINT('Ctrl Pts',(-17.405,-15.4999999999999,6.48699999999991));
#16613=CARTESIAN_POINT('Ctrl Pts',(-17.405,-15.6573653676441,6.48103838993624));
#16614=CARTESIAN_POINT('Ctrl Pts',(-17.3855039144757,-15.8144320154612,
6.47466167296953));
#16615=CARTESIAN_POINT('Ctrl Pts',(-17.2858671110078,-16.2079255525943,
6.45757532996358));
#16616=CARTESIAN_POINT('Ctrl Pts',(-17.1786901034823,-16.434062405774,6.44666418546016));
#16617=CARTESIAN_POINT('Ctrl Pts',(-16.8811149668584,-16.8361165529484,
6.42492417349771));
#16618=CARTESIAN_POINT('Ctrl Pts',(-16.6921893369319,-17.0071153860193,
6.41431384329561));
#16619=CARTESIAN_POINT('Ctrl Pts',(-16.2679653059451,-17.2599951864708,
6.3954550354746));
#16620=CARTESIAN_POINT('Ctrl Pts',(-16.0388328778226,-17.3431118415628,
6.38557099203068));
#16621=CARTESIAN_POINT('Ctrl Pts',(-15.5525225818871,-17.4207271638321,
6.36429757576055));
#16622=CARTESIAN_POINT('Ctrl Pts',(-15.2994157965646,-17.410947629751,6.35322553790743));
#16623=CARTESIAN_POINT('Ctrl Pts',(-14.813683679078,-17.2943880200312,6.33197741378292));
#16624=CARTESIAN_POINT('Ctrl Pts',(-14.5856038048897,-17.1895935173748,
6.32267510107439));
#16625=CARTESIAN_POINT('Ctrl Pts',(-14.186058208372,-16.9008155654491,6.30299610541913));
#16626=CARTESIAN_POINT('Ctrl Pts',(-14.0174177953425,-16.7209255269853,
6.2924926255542));
#16627=CARTESIAN_POINT('Ctrl Pts',(-13.7521525220174,-16.2991036698075,
6.27071042604193));
#16628=CARTESIAN_POINT('Ctrl Pts',(-13.6612898194952,-16.0591930631974,
6.25963430919053));
#16629=CARTESIAN_POINT('Ctrl Pts',(-13.5808752867126,-15.5692252954415,
6.23931358301802));
#16630=CARTESIAN_POINT('Ctrl Pts',(-13.5876496855473,-15.3246422120223,
6.23051753534931));
#16631=CARTESIAN_POINT('Ctrl Pts',(-13.69358258658,-14.8465705637078,6.21008933575238));
#16632=CARTESIAN_POINT('Ctrl Pts',(-13.7935051225893,-14.6179683833791,
6.19924346683156));
#16633=CARTESIAN_POINT('Ctrl Pts',(-14.0780384376739,-14.2074310799854,
6.17746733422077));
#16634=CARTESIAN_POINT('Ctrl Pts',(-14.2615952673923,-14.0306168913634,
6.16675412363653));
#16635=CARTESIAN_POINT('Ctrl Pts',(-14.6774696299874,-13.7648903345165,
6.1475912570579));
#16636=CARTESIAN_POINT('Ctrl Pts',(-14.9034802016442,-13.6747996097228,
6.13809447936804));
#16637=CARTESIAN_POINT('Ctrl Pts',(-15.3858696864533,-13.5820526462828,
6.11699257714542));
#16638=CARTESIAN_POINT('Ctrl Pts',(-15.638328177964,-13.583645740638,6.10594889860164));
#16639=CARTESIAN_POINT('Ctrl Pts',(-16.1291525866983,-13.6844547122694,
6.08447801458002));
#16640=CARTESIAN_POINT('Ctrl Pts',(-16.3626155095225,-13.7830517490666,
6.07484396541252));
#16641=CARTESIAN_POINT('Ctrl Pts',(-16.7790766551765,-14.06587592793,6.0550205403597));
#16642=CARTESIAN_POINT('Ctrl Pts',(-16.9576323622296,-14.2477879182273,
6.0442235911034));
#16643=CARTESIAN_POINT('Ctrl Pts',(-17.2301952244117,-14.665614301179,6.02243314083661));
#16644=CARTESIAN_POINT('Ctrl Pts',(-17.3235315529603,-14.8962457352792,
6.01165445119898));
#16645=CARTESIAN_POINT('Ctrl Pts',(-17.3934468662726,-15.2577349531895,
5.99643063218933));
#16646=CARTESIAN_POINT('Ctrl Pts',(-17.405000000436,-15.3788627644953,5.99158914799085));
#16647=CARTESIAN_POINT('Ctrl Pts',(-17.405,-15.5000000068569,5.98699999974014));
#16648=CARTESIAN_POINT('Origin',(-15.5,-15.5,-1.713));
#16649=CARTESIAN_POINT('',(-17.405,-15.5,5.42449999999996));
#16650=CARTESIAN_POINT('',(-17.405,-15.5,5.48699999999989));
#16651=CARTESIAN_POINT('',(-17.405,-15.5,-1.713));
#16652=CARTESIAN_POINT('Ctrl Pts',(-17.405,-15.5,5.42449999999996));
#16653=CARTESIAN_POINT('Ctrl Pts',(-17.405,-15.3760434359275,5.42919595509413));
#16654=CARTESIAN_POINT('Ctrl Pts',(-17.3929028862534,-15.2521105344024,
5.43415560504857));
#16655=CARTESIAN_POINT('Ctrl Pts',(-17.3208126200574,-14.8880510179744,
5.44952436807631));
#16656=CARTESIAN_POINT('Ctrl Pts',(-17.226391501484,-14.6577403242684,5.46031463364058));
#16657=CARTESIAN_POINT('Ctrl Pts',(-16.9518486544494,-14.2410878161607,
5.48210391973371));
#16658=CARTESIAN_POINT('Ctrl Pts',(-16.7724610386279,-14.0600036767685,
5.49288770244791));
#16659=CARTESIAN_POINT('Ctrl Pts',(-16.3629640389708,-13.7846532854336,
5.5122756697999));
#16660=CARTESIAN_POINT('Ctrl Pts',(-16.1392237783365,-13.6893274580866,
5.52153745501584));
#16661=CARTESIAN_POINT('Ctrl Pts',(-15.659834124758,-13.5853971651835,5.5425081310254));
#16662=CARTESIAN_POINT('Ctrl Pts',(-15.408023639897,-13.5809403932743,5.55352346282159));
#16663=CARTESIAN_POINT('Ctrl Pts',(-14.913556107456,-13.6699452666455,5.57515371358453));
#16664=CARTESIAN_POINT('Ctrl Pts',(-14.6760350732985,-13.7638927857631,
5.58508484305015));
#16665=CARTESIAN_POINT('Ctrl Pts',(-14.2598042431201,-14.033696179453,5.6044099527637));
#16666=CARTESIAN_POINT('Ctrl Pts',(-14.0830030766772,-14.203762905526,5.61471978164992));
#16667=CARTESIAN_POINT('Ctrl Pts',(-13.79741831993,-14.6089053564775,5.63631453375179));
#16668=CARTESIAN_POINT('Ctrl Pts',(-13.6943846727369,-14.8422789569263,
5.64740920961171));
#16669=CARTESIAN_POINT('Ctrl Pts',(-13.5870911327856,-15.3278163767363,
5.66815000182601));
#16670=CARTESIAN_POINT('Ctrl Pts',(-13.5808071130259,-15.5745934078983,
5.67701545681125));
#16671=CARTESIAN_POINT('Ctrl Pts',(-13.6621313310384,-16.0583284637951,
5.69711996057826));
#16672=CARTESIAN_POINT('Ctrl Pts',(-13.7494664034097,-16.2906393684339,
5.70783101399816));
#16673=CARTESIAN_POINT('Ctrl Pts',(-14.0110168099278,-16.7147717784116,
5.72961949365117));
#16674=CARTESIAN_POINT('Ctrl Pts',(-14.1849125956826,-16.9011803082986,
5.74048486614643));
#16675=CARTESIAN_POINT('Ctrl Pts',(-14.586121554684,-17.1887935215797,5.76015611849404));
#16676=CARTESIAN_POINT('Ctrl Pts',(-14.8070478925458,-17.2908173313166,
5.76918713440696));
#16677=CARTESIAN_POINT('Ctrl Pts',(-15.2825443775373,-17.408819662251,5.78998750557895));
#16678=CARTESIAN_POINT('Ctrl Pts',(-15.5333346762825,-17.4208758725757,
5.80095820981103));
#16679=CARTESIAN_POINT('Ctrl Pts',(-16.0290349471213,-17.3473935266342,
5.8226423861382));
#16680=CARTESIAN_POINT('Ctrl Pts',(-16.2688452203251,-17.2611273017974,
5.83293139227933));
#16681=CARTESIAN_POINT('Ctrl Pts',(-16.6922941478763,-17.0053894491118,
5.8518815209281));
#16682=CARTESIAN_POINT('Ctrl Pts',(-16.8739280570934,-16.8416634991693,
5.8620568396734));
#16683=CARTESIAN_POINT('Ctrl Pts',(-17.1717436625757,-16.4474570381807,
5.88350481046489));
#16684=CARTESIAN_POINT('Ctrl Pts',(-17.2821880097861,-16.2184804825159,
5.89459499802755));
#16685=CARTESIAN_POINT('Ctrl Pts',(-17.3849003572026,-15.8192563713138,
5.9119657065058));
#16686=CARTESIAN_POINT('Ctrl Pts',(-17.405,-15.6597824535574,5.91844682135343));
#16687=CARTESIAN_POINT('Ctrl Pts',(-17.405,-15.5,5.92449999999997));
#16688=CARTESIAN_POINT('Ctrl Pts',(-17.405,-15.5000000068569,5.98699999974013));
#16689=CARTESIAN_POINT('Ctrl Pts',(-17.4049999995636,-15.6212520006587,
5.98240650424101));
#16690=CARTESIAN_POINT('Ctrl Pts',(-17.3934249672455,-15.7424940251675,
5.97756021424145));
#16691=CARTESIAN_POINT('Ctrl Pts',(-17.3221315854689,-16.1107514310504,
5.9620498485584));
#16692=CARTESIAN_POINT('Ctrl Pts',(-17.2248764986786,-16.3473310510096,
5.95096010646316));
#16693=CARTESIAN_POINT('Ctrl Pts',(-16.9489044613018,-16.7605841853532,
5.92926834219268));
#16694=CARTESIAN_POINT('Ctrl Pts',(-16.7759444872425,-16.935403161333,5.91886249524204));
#16695=CARTESIAN_POINT('Ctrl Pts',(-16.3676999304369,-17.2143489102531,
5.89936571557253));
#16696=CARTESIAN_POINT('Ctrl Pts',(-16.1347682830141,-17.313555727457,5.88976764142664));
#16697=CARTESIAN_POINT('Ctrl Pts',(-15.6444331987704,-17.4159141380227,
5.86831816267583));
#16698=CARTESIAN_POINT('Ctrl Pts',(-15.3918998457965,-17.4183069254304,
5.8572712093524));
#16699=CARTESIAN_POINT('Ctrl Pts',(-14.9091203529905,-17.3270377526458,
5.83615224641251));
#16700=CARTESIAN_POINT('Ctrl Pts',(-14.6828074455978,-17.2376334387652,
5.82662110337859));
#16701=CARTESIAN_POINT('Ctrl Pts',(-14.2661037299997,-16.9731704217253,
5.80748796475579));
#16702=CARTESIAN_POINT('Ctrl Pts',(-14.0820088260293,-16.7969225078747,
5.7967844379516));
#16703=CARTESIAN_POINT('Ctrl Pts',(-13.7961776710268,-16.3872035965591,
5.77501092250489));
#16704=CARTESIAN_POINT('Ctrl Pts',(-13.6955369747897,-16.1588346230077,
5.76415818056918));
#16705=CARTESIAN_POINT('Ctrl Pts',(-13.5881963560233,-15.6810970911766,
5.74371184862297));
#16706=CARTESIAN_POINT('Ctrl Pts',(-13.5806847269442,-15.4366308122503,
5.73491243701307));
#16707=CARTESIAN_POINT('Ctrl Pts',(-13.6595783657715,-14.9464290612334,
5.71461611204482));
#16708=CARTESIAN_POINT('Ctrl Pts',(-13.7497409224647,-14.7061669365763,
5.70354199210313));
#16709=CARTESIAN_POINT('Ctrl Pts',(-14.0138290100348,-14.2834314875499,
5.68175092991055));
#16710=CARTESIAN_POINT('Ctrl Pts',(-14.1819919720835,-14.1029975163744,
5.67123728670109));
#16711=CARTESIAN_POINT('Ctrl Pts',(-14.5805926662016,-13.8131593223387,
5.65153879212186));
#16712=CARTESIAN_POINT('Ctrl Pts',(-14.8081547979217,-13.7077660171985,
5.64226444453527));
#16713=CARTESIAN_POINT('Ctrl Pts',(-15.2933813077319,-13.5896850205772,
5.62103843798188));
#16714=CARTESIAN_POINT('Ctrl Pts',(-15.5465373051868,-13.5791082285566,
5.60996424736706));
#16715=CARTESIAN_POINT('Ctrl Pts',(-16.0332209521069,-13.6552489250426,
5.58867449903284));
#16716=CARTESIAN_POINT('Ctrl Pts',(-16.262660718492,-13.7376920430767,5.57874860458176));
#16717=CARTESIAN_POINT('Ctrl Pts',(-16.6876819207768,-13.9893307180406,
5.55991937946208));
#16718=CARTESIAN_POINT('Ctrl Pts',(-16.8771141741595,-14.1597611584412,
5.54931950117439));
#16719=CARTESIAN_POINT('Ctrl Pts',(-17.1759309590692,-14.560977049772,5.52758408793076));
#16720=CARTESIAN_POINT('Ctrl Pts',(-17.283803098501,-14.7868647889453,5.5166671767215));
#16721=CARTESIAN_POINT('Ctrl Pts',(-17.3850463837683,-15.181917730531,5.49948662003355));
#16722=CARTESIAN_POINT('Ctrl Pts',(-17.405,-15.3407987939666,5.49303115873733));
#16723=CARTESIAN_POINT('Ctrl Pts',(-17.405,-15.5,5.48699999999989));
#16724=CARTESIAN_POINT('Origin',(-15.5,-15.5,-1.713));
#16725=CARTESIAN_POINT('',(-17.405,-15.5,4.92449999999995));
#16726=CARTESIAN_POINT('',(-17.405,-15.5,4.98699999999988));
#16727=CARTESIAN_POINT('',(-17.405,-15.5,-1.713));
#16728=CARTESIAN_POINT('Ctrl Pts',(-17.405,-15.5000000000001,4.92449999999995));
#16729=CARTESIAN_POINT('Ctrl Pts',(-17.405,-15.3380084622269,4.93063686731884));
#16730=CARTESIAN_POINT('Ctrl Pts',(-17.3843408041619,-15.1763710006228,
4.93721218428607));
#16731=CARTESIAN_POINT('Ctrl Pts',(-17.2806376985815,-14.7789600840496,
4.95453587205002));
#16732=CARTESIAN_POINT('Ctrl Pts',(-17.1717102736454,-14.5534548816947,
4.96546137276711));
#16733=CARTESIAN_POINT('Ctrl Pts',(-16.8710112518389,-14.1535201252274,
4.98718942044254));
#16734=CARTESIAN_POINT('Ctrl Pts',(-16.6808125325853,-13.983956326939,4.99777323131334));
#16735=CARTESIAN_POINT('Ctrl Pts',(-16.2545819583126,-13.7342053939596,
5.01655739315566));
#16736=CARTESIAN_POINT('Ctrl Pts',(-16.0246727565372,-13.6527867878846,
5.02654843584694));
#16737=CARTESIAN_POINT('Ctrl Pts',(-15.5374231761305,-13.5788933923025,
5.04786294067662));
#16738=CARTESIAN_POINT('Ctrl Pts',(-15.2841969270122,-13.5906848771702,
5.05894020441759));
#16739=CARTESIAN_POINT('Ctrl Pts',(-14.7997439961544,-13.7110798223801,
5.08013237112176));
#16740=CARTESIAN_POINT('Ctrl Pts',(-14.5729685123419,-13.8173840698908,
5.08936559945493));
#16741=CARTESIAN_POINT('Ctrl Pts',(-14.1758098743663,-14.1088374455546,
5.10909374233906));
#16742=CARTESIAN_POINT('Ctrl Pts',(-14.0083786203189,-14.2900988616466,
5.11962272825705));
#16743=CARTESIAN_POINT('Ctrl Pts',(-13.7460922865542,-14.7142219875609,
5.14142695259023));
#16744=CARTESIAN_POINT('Ctrl Pts',(-13.6570003466679,-14.9550166456319,
5.15249783014614));
#16745=CARTESIAN_POINT('Ctrl Pts',(-13.5804275330516,-15.4455720839554,
5.17275679245414));
#16746=CARTESIAN_POINT('Ctrl Pts',(-13.5890640079251,-15.6898618051801,
5.18156286747393));
#16747=CARTESIAN_POINT('Ctrl Pts',(-13.6985559912454,-16.1670865051149,
5.2020368265779));
#16748=CARTESIAN_POINT('Ctrl Pts',(-13.8002936525146,-16.3950946904093,
5.21289989356697));
#16749=CARTESIAN_POINT('Ctrl Pts',(-14.088104367486,-16.8035545086014,5.23466900714812));
#16750=CARTESIAN_POINT('Ctrl Pts',(-14.2730183848475,-16.9789334799628,
5.24535753090881));
#16751=CARTESIAN_POINT('Ctrl Pts',(-14.6909876344324,-17.2414631089392,
5.26444510539403));
#16752=CARTESIAN_POINT('Ctrl Pts',(-14.9177651172584,-17.3298174134956,
5.27403040757896));
#16753=CARTESIAN_POINT('Ctrl Pts',(-15.4011395799388,-17.4188210052778,
5.29517539719754));
#16754=CARTESIAN_POINT('Ctrl Pts',(-15.6537828372131,-17.4152022158959,
5.30622715823318));
#16755=CARTESIAN_POINT('Ctrl Pts',(-16.1433642866381,-17.3104730906201,
5.32764366958161));
#16756=CARTESIAN_POINT('Ctrl Pts',(-16.375483745341,-17.2103334121474,5.33718808787432));
#16757=CARTESIAN_POINT('Ctrl Pts',(-16.7822911123883,-16.9297542878312,
5.35671531153807));
#16758=CARTESIAN_POINT('Ctrl Pts',(-16.9545470277676,-16.7540897545839,
5.36713779211663));
#16759=CARTESIAN_POINT('Ctrl Pts',(-17.2287667612673,-16.3394015430889,
5.38884559581544));
#16760=CARTESIAN_POINT('Ctrl Pts',(-17.3249725708871,-16.1022598955999,
5.39993367962256));
#16761=CARTESIAN_POINT('Ctrl Pts',(-17.3939902026772,-15.7365117366992,
5.4152992094953));
#16762=CARTESIAN_POINT('Ctrl Pts',(-17.405,-15.6182543353654,5.42002006743066));
#16763=CARTESIAN_POINT('Ctrl Pts',(-17.405,-15.5,5.42449999999996));
#16764=CARTESIAN_POINT('Ctrl Pts',(-17.405,-15.5,5.48699999999989));
#16765=CARTESIAN_POINT('Ctrl Pts',(-17.405,-15.5814768755342,5.4839133401559));
#16766=CARTESIAN_POINT('Ctrl Pts',(-17.3997732389571,-15.6630288598788,
5.4807095137914));
#16767=CARTESIAN_POINT('Ctrl Pts',(-17.3566182979129,-15.9969615452074,
5.46711495302279));
#16768=CARTESIAN_POINT('Ctrl Pts',(-17.2735392416782,-16.2406370700203,
5.45606645245911));
#16769=CARTESIAN_POINT('Ctrl Pts',(-17.021409045366,-16.6723479860623,5.4341969109657));
#16770=CARTESIAN_POINT('Ctrl Pts',(-16.8581230029901,-16.8581616545989,
5.42358613325307));
#16771=CARTESIAN_POINT('Ctrl Pts',(-16.4690036002391,-17.1585557089554,
5.40369511909761));
#16772=CARTESIAN_POINT('Ctrl Pts',(-16.2465361768677,-17.2698769738081,
5.39465687562847));
#16773=CARTESIAN_POINT('Ctrl Pts',(-15.7664355311582,-17.4029987099506,
5.37365509760093));
#16774=CARTESIAN_POINT('Ctrl Pts',(-15.5129232590213,-17.4215146350884,
5.36256532191691));
#16775=CARTESIAN_POINT('Ctrl Pts',(-15.0227594117968,-17.3600985674522,
5.34112333384936));
#16776=CARTESIAN_POINT('Ctrl Pts',(-14.7902722396957,-17.2843865373322,
5.33095329132526));
#16777=CARTESIAN_POINT('Ctrl Pts',(-14.3573886143867,-17.0450337541717,
5.31201699975444));
#16778=CARTESIAN_POINT('Ctrl Pts',(-14.162974515436,-16.8802544045959,5.30171227628098));
#16779=CARTESIAN_POINT('Ctrl Pts',(-13.8519761651499,-16.4873592914475,
5.28002564792785));
#16780=CARTESIAN_POINT('Ctrl Pts',(-13.7372974953326,-16.2640320949588,
5.26905686575707));
#16781=CARTESIAN_POINT('Ctrl Pts',(-13.6022888935652,-15.7930997383418,
5.2482631787414));
#16782=CARTESIAN_POINT('Ctrl Pts',(-13.5804608845042,-15.5507227020883,
5.23923957595381));
#16783=CARTESIAN_POINT('Ctrl Pts',(-13.6295123736636,-15.0595029086655,
5.21955739902793));
#16784=CARTESIAN_POINT('Ctrl Pts',(-13.7042844979505,-14.8157866894146,
5.20868904822613));
#16785=CARTESIAN_POINT('Ctrl Pts',(-13.941319488103,-14.3775117194336,5.18690100129162));
#16786=CARTESIAN_POINT('Ctrl Pts',(-14.0990413745835,-14.1859249151819,
5.17619321551943));
#16787=CARTESIAN_POINT('Ctrl Pts',(-14.4776810473978,-13.8740364453775,
5.15609596379566));
#16788=CARTESIAN_POINT('Ctrl Pts',(-14.6947281052106,-13.7563163073901,
5.1472262421167));
#16789=CARTESIAN_POINT('Ctrl Pts',(-15.1690701263999,-13.6070357747158,
5.12647637242337));
#16790=CARTESIAN_POINT('Ctrl Pts',(-15.4226956206289,-13.5798847323188,
5.11538164389191));
#16791=CARTESIAN_POINT('Ctrl Pts',(-15.9162414890316,-13.6252091599672,
5.09379171089091));
#16792=CARTESIAN_POINT('Ctrl Pts',(-16.1518191026795,-13.6935529003981,
5.08348647844787));
#16793=CARTESIAN_POINT('Ctrl Pts',(-16.5934068526385,-13.9196514534064,
5.06416942901834));
#16794=CARTESIAN_POINT('Ctrl Pts',(-16.7934223159308,-14.078687343901,5.05422142208812));
#16795=CARTESIAN_POINT('Ctrl Pts',(-17.1172886667511,-14.4628832908677,
5.03258289953719));
#16796=CARTESIAN_POINT('Ctrl Pts',(-17.2390389883794,-14.6833123338815,
5.02156923760385));
#16797=CARTESIAN_POINT('Ctrl Pts',(-17.3746778120002,-15.1084162217768,
5.00249792623135));
#16798=CARTESIAN_POINT('Ctrl Pts',(-17.405,-15.3037503177909,4.9944346986122));
#16799=CARTESIAN_POINT('Ctrl Pts',(-17.405,-15.5000000000001,4.98699999999988));
#16800=CARTESIAN_POINT('Origin',(-15.5,-15.5,-1.713));
#16801=CARTESIAN_POINT('',(-17.405,-15.5,4.42449999999995));
#16802=CARTESIAN_POINT('',(-17.405,-15.4999999574994,4.48700000322005));
#16803=CARTESIAN_POINT('',(-17.405,-15.5,-1.713));
#16804=CARTESIAN_POINT('Ctrl Pts',(-17.405,-15.5000000000001,4.42449999999995));
#16805=CARTESIAN_POINT('Ctrl Pts',(-17.405,-15.300946180348,4.43204093020726));
#16806=CARTESIAN_POINT('Ctrl Pts',(-17.3738049147864,-15.1028665454003,
4.44022726172271));
#16807=CARTESIAN_POINT('Ctrl Pts',(-17.2354136557939,-14.6756034049486,
4.45944057594965));
#16808=CARTESIAN_POINT('Ctrl Pts',(-17.1126253999981,-14.4556205858719,
4.47046003516288));
#16809=CARTESIAN_POINT('Ctrl Pts',(-16.7871854121762,-14.0731029611838,
4.49206939536787));
#16810=CARTESIAN_POINT('Ctrl Pts',(-16.586797360482,-13.9151580380625,4.50195855815905));
#16811=CARTESIAN_POINT('Ctrl Pts',(-16.1445619233844,-13.6909379581971,
4.52130394035929));
#16812=CARTESIAN_POINT('Ctrl Pts',(-15.90861573014,-13.6235199477863,4.53162529614427));
#16813=CARTESIAN_POINT('Ctrl Pts',(-15.4146849504325,-13.5802098264281,
4.55323206691012));
#16814=CARTESIAN_POINT('Ctrl Pts',(-15.1610652756953,-13.6084381761364,
4.56432654087063));
#16815=CARTESIAN_POINT('Ctrl Pts',(-14.6874548542244,-13.7597218463035,
4.58504440707669));
#16816=CARTESIAN_POINT('Ctrl Pts',(-14.4710755985286,-13.8782384657527,
4.59389962874866));
#16817=CARTESIAN_POINT('Ctrl Pts',(-14.0937570674529,-14.1915632010929,
4.61402239541429));
#16818=CARTESIAN_POINT('Ctrl Pts',(-13.9367488918255,-14.383864345526,4.62474163268767));
#16819=CARTESIAN_POINT('Ctrl Pts',(-13.7014796361299,-14.8231954715791,
4.64653107029409));
#16820=CARTESIAN_POINT('Ctrl Pts',(-13.6277136965757,-15.0672138774326,
4.65738886155556));
#16821=CARTESIAN_POINT('Ctrl Pts',(-13.5806899402637,-15.5585874680381,
4.67703251380268));
#16822=CARTESIAN_POINT('Ctrl Pts',(-13.6035044448897,-15.8008336512809,
4.6860827562014));
#16823=CARTESIAN_POINT('Ctrl Pts',(-13.7404400945265,-16.2712745947072,
4.70689997548424));
#16824=CARTESIAN_POINT('Ctrl Pts',(-13.8560896031551,-16.4942184303239,
4.71787546890398));
#16825=CARTESIAN_POINT('Ctrl Pts',(-14.1688115759052,-16.8858866889789,
4.73955331878264));
#16826=CARTESIAN_POINT('Ctrl Pts',(-14.3639288494479,-17.0498517421699,
4.74980309927576));
#16827=CARTESIAN_POINT('Ctrl Pts',(-14.7979250943807,-17.2874251666292,
4.76878806187125));
#16828=CARTESIAN_POINT('Ctrl Pts',(-15.0308360672455,-17.3621653543147,
4.77897664336141));
#16829=CARTESIAN_POINT('Ctrl Pts',(-15.521478859006,-17.4214529261841,4.80043958263354));
#16830=CARTESIAN_POINT('Ctrl Pts',(-15.7750225343709,-17.4017918333695,
4.81153073203709));
#16831=CARTESIAN_POINT('Ctrl Pts',(-16.2543703574976,-17.2665159232243,
4.83249957819312));
#16832=CARTESIAN_POINT('Ctrl Pts',(-16.4761118588062,-17.154343863983,4.84151015383185));
#16833=CARTESIAN_POINT('Ctrl Pts',(-16.8638520975196,-16.8524267802324,
4.86142870080129));
#16834=CARTESIAN_POINT('Ctrl Pts',(-17.0264160255427,-16.6658427318232,
4.87205286921227));
#16835=CARTESIAN_POINT('Ctrl Pts',(-17.2767855078975,-16.2328557607738,
4.89393224181132));
#16836=CARTESIAN_POINT('Ctrl Pts',(-17.3588258334554,-15.9887011344888,
4.9049761732021));
#16837=CARTESIAN_POINT('Ctrl Pts',(-17.4001334338982,-15.6573136012298,
4.91843390822054));
#16838=CARTESIAN_POINT('Ctrl Pts',(-17.405,-15.5786191688494,4.92152160116145));
#16839=CARTESIAN_POINT('Ctrl Pts',(-17.405,-15.5000000000001,4.92449999999995));
#16840=CARTESIAN_POINT('Ctrl Pts',(-17.405,-15.5000000000001,4.98699999999988));
#16841=CARTESIAN_POINT('Ctrl Pts',(-17.405,-15.5441523099634,4.98532733936716));
#16842=CARTESIAN_POINT('Ctrl Pts',(-17.4034650555517,-15.588348432899,4.98361944621604));
#16843=CARTESIAN_POINT('Ctrl Pts',(-17.3828269524683,-15.8843303780855,
4.97195510084708));
#16844=CARTESIAN_POINT('Ctrl Pts',(-17.3153906860251,-16.1301442874987,
4.96116773324529));
#16845=CARTESIAN_POINT('Ctrl Pts',(-17.0912870699373,-16.5759274289171,
4.93937808612846));
#16846=CARTESIAN_POINT('Ctrl Pts',(-16.9388204662768,-16.7726434333998,
4.92859093131468));
#16847=CARTESIAN_POINT('Ctrl Pts',(-16.5697988216603,-17.0949234111697,
4.90831037706324));
#16848=CARTESIAN_POINT('Ctrl Pts',(-16.3575362863681,-17.2183950289438,
4.89951252346313));
#16849=CARTESIAN_POINT('Ctrl Pts',(-15.8885431733751,-17.382089147163,4.87899663925522));
#16850=CARTESIAN_POINT('Ctrl Pts',(-15.6350588011372,-17.4170216974866,
4.86790808403922));
#16851=CARTESIAN_POINT('Ctrl Pts',(-15.1389165413175,-17.3862801935719,
4.84620457311099));
#16852=CARTESIAN_POINT('Ctrl Pts',(-14.9007609710995,-17.3246551866247,
4.83578656916445));
#16853=CARTESIAN_POINT('Ctrl Pts',(-14.4545564524755,-17.1120822196972,
4.81626756135064));
#16854=CARTESIAN_POINT('Ctrl Pts',(-14.2518816904769,-16.9608150588265,
4.80670882748964));
#16855=CARTESIAN_POINT('Ctrl Pts',(-13.9168450172487,-16.5886930567592,
4.78528339250663));
#16856=CARTESIAN_POINT('Ctrl Pts',(-13.7876907953647,-16.371566588569,4.77423290483257));
#16857=CARTESIAN_POINT('Ctrl Pts',(-13.623693143634,-15.9082831048492,4.75309493055782));
#16858=CARTESIAN_POINT('Ctrl Pts',(-13.5871296959008,-15.6676780010439,
4.74352443397239));
#16859=CARTESIAN_POINT('Ctrl Pts',(-13.6061249022657,-15.1744757364315,
4.72442455236517));
#16860=CARTESIAN_POINT('Ctrl Pts',(-13.6658641934304,-14.9267196306907,
4.7137319571291));
#16861=CARTESIAN_POINT('Ctrl Pts',(-13.8762571974879,-14.4735300670181,
4.69196160818337));
#16862=CARTESIAN_POINT('Ctrl Pts',(-14.023081911278,-14.2716258629011,4.68110130517412));
#16863=CARTESIAN_POINT('Ctrl Pts',(-14.3820348473883,-13.9386239728758,
4.66063478879943));
#16864=CARTESIAN_POINT('Ctrl Pts',(-14.5894703723234,-13.8092386072515,
4.65183069237424));
#16865=CARTESIAN_POINT('Ctrl Pts',(-15.0528208481337,-13.6308641948418,
4.63156164268873));
#16866=CARTESIAN_POINT('Ctrl Pts',(-15.305921621302,-13.5879444772796,4.62048986783447));
#16867=CARTESIAN_POINT('Ctrl Pts',(-15.8042860608109,-13.6036374054734,
4.59868914869584));
#16868=CARTESIAN_POINT('Ctrl Pts',(-16.0448845797942,-13.6582889446888,
4.58816427909903));
#16869=CARTESIAN_POINT('Ctrl Pts',(-16.4956875029771,-13.8570659644062,
4.56844411623013));
#16870=CARTESIAN_POINT('Ctrl Pts',(-16.7010308675647,-14.0006130954559,
4.55919998756135));
#16871=CARTESIAN_POINT('Ctrl Pts',(-17.0470873642231,-14.360456424669,4.53799868778837));
#16872=CARTESIAN_POINT('Ctrl Pts',(-17.1836196412927,-14.5740087589079,
4.52692222737616));
#16873=CARTESIAN_POINT('Ctrl Pts',(-17.3608848628781,-15.0285694828898,
4.50582451323252));
#16874=CARTESIAN_POINT('Ctrl Pts',(-17.4049999947116,-15.2633019929779,
4.4959670380467));
#16875=CARTESIAN_POINT('Ctrl Pts',(-17.405,-15.499999957438,4.48700000161229));
#16876=CARTESIAN_POINT('Origin',(-15.5,-15.5,-1.713));
#16877=CARTESIAN_POINT('',(-17.405,-15.4999999913089,3.92450000065845));
#16878=CARTESIAN_POINT('',(-17.405,-15.5,3.98699999999987));
#16879=CARTESIAN_POINT('',(-17.405,-15.5,-1.713));
#16880=CARTESIAN_POINT('Ctrl Pts',(-17.405,-15.4999999826177,3.92450000065845));
#16881=CARTESIAN_POINT('Ctrl Pts',(-17.4049999978143,-15.2604577159144,
3.9335747902183));
#16882=CARTESIAN_POINT('Ctrl Pts',(-17.359817730218,-15.0229721283851,3.94355990332549));
#16883=CARTESIAN_POINT('Ctrl Pts',(-17.1794744215171,-14.5664812063353,
3.96479806559331));
#16884=CARTESIAN_POINT('Ctrl Pts',(-17.0419187944687,-14.3534475582947,
3.97587725914485));
#16885=CARTESIAN_POINT('Ctrl Pts',(-16.6943411737859,-13.9953278652344,
3.99704653132888));
#16886=CARTESIAN_POINT('Ctrl Pts',(-16.4886247886422,-13.8528507646097,
4.00625307136287));
#16887=CARTESIAN_POINT('Ctrl Pts',(-16.0371837458011,-13.6560148499806,
4.02600114847753));
#16888=CARTESIAN_POINT('Ctrl Pts',(-15.7962570520486,-13.6023535784996,
4.03654037392603));
#16889=CARTESIAN_POINT('Ctrl Pts',(-15.297615099849,-13.5887906112471,4.05835323272741));
#16890=CARTESIAN_POINT('Ctrl Pts',(-15.0445879002524,-13.6328373649071,
4.06942178914021));
#16891=CARTESIAN_POINT('Ctrl Pts',(-14.5820463480311,-13.8132755459749,
4.08965545284191));
#16892=CARTESIAN_POINT('Ctrl Pts',(-14.3752851451608,-13.9434981112106,
4.09846707133362));
#16893=CARTESIAN_POINT('Ctrl Pts',(-14.0177708750154,-14.2780184110088,
4.11895964407112));
#16894=CARTESIAN_POINT('Ctrl Pts',(-13.8717630623921,-14.4806481670653,
4.12982956632042));
#16895=CARTESIAN_POINT('Ctrl Pts',(-13.6633412943098,-14.9348574141291,
4.15159542942769));
#16896=CARTESIAN_POINT('Ctrl Pts',(-13.6047019998018,-15.1828698074392,
4.1622736744108));
#16897=CARTESIAN_POINT('Ctrl Pts',(-13.5878892661774,-15.6761920399413,
4.18133036524241));
#16898=CARTESIAN_POINT('Ctrl Pts',(-13.6255339615237,-15.916682506097,4.19095339529093));
#16899=CARTESIAN_POINT('Ctrl Pts',(-13.7916727576322,-16.3793784160295,
4.21211594167251));
#16900=CARTESIAN_POINT('Ctrl Pts',(-13.9218837745339,-16.596010533555,4.223170815929));
#16901=CARTESIAN_POINT('Ctrl Pts',(-14.2585051113859,-16.9663893557281,
4.24456487268541));
#16902=CARTESIAN_POINT('Ctrl Pts',(-14.4615603940353,-17.1165497929753,
4.25407394549568));
#16903=CARTESIAN_POINT('Ctrl Pts',(-14.9084234963101,-17.3271671728719,
4.27362176274305));
#16904=CARTESIAN_POINT('Ctrl Pts',(-15.146936993668,-17.3878108216528,4.28405542404481));
#16905=CARTESIAN_POINT('Ctrl Pts',(-15.6434206839156,-17.4164292828546,
4.30577387068733));
#16906=CARTESIAN_POINT('Ctrl Pts',(-15.8968654809846,-17.3803672954393,
4.3168606947061));
#16907=CARTESIAN_POINT('Ctrl Pts',(-16.3650702726416,-17.2145908692008,
4.33734209416616));
#16908=CARTESIAN_POINT('Ctrl Pts',(-16.5766448830822,-17.0902845045195,
4.34613585570338));
#16909=CARTESIAN_POINT('Ctrl Pts',(-16.9442556557284,-16.7664921099221,
4.36644284719931));
#16910=CARTESIAN_POINT('Ctrl Pts',(-17.095939925573,-16.5690376427327,4.37724086642937));
#16911=CARTESIAN_POINT('Ctrl Pts',(-17.3181320330473,-16.1221883712515,
4.39902909366046));
#16912=CARTESIAN_POINT('Ctrl Pts',(-17.3844902892752,-15.8760866337007,
4.40980378678158));
#16913=CARTESIAN_POINT('Ctrl Pts',(-17.4036517297875,-15.5828007286006,
4.42133369774593));
#16914=CARTESIAN_POINT('Ctrl Pts',(-17.405,-15.5413804235327,4.42293234916886));
#16915=CARTESIAN_POINT('Ctrl Pts',(-17.405,-15.5000000000001,4.42449999999995));
#16916=CARTESIAN_POINT('Ctrl Pts',(-17.405,-15.499999957438,4.48700000161229));
#16917=CARTESIAN_POINT('Ctrl Pts',(-17.4050000001085,-15.5048557134102,
4.48681604675312));
#16918=CARTESIAN_POINT('Ctrl Pts',(-17.4049814345791,-15.5097122660366,
4.48663165565055));
#16919=CARTESIAN_POINT('Ctrl Pts',(-17.4030142719686,-15.7669161853031,
4.47684474798026));
#16920=CARTESIAN_POINT('Ctrl Pts',(-17.3509618993671,-16.0163535166326,
4.46625659172986));
#16921=CARTESIAN_POINT('Ctrl Pts',(-17.1544054843015,-16.4764685333068,
4.44452651733637));
#16922=CARTESIAN_POINT('Ctrl Pts',(-17.0133444914353,-16.6833609452157,
4.43360330731903));
#16923=CARTESIAN_POINT('Ctrl Pts',(-16.6644503982568,-17.02690772249,4.41295731943203));
#16924=CARTESIAN_POINT('Ctrl Pts',(-16.4616519094173,-17.1621103410901,
4.40406701266038));
#16925=CARTESIAN_POINT('Ctrl Pts',(-16.0039662811969,-17.3547409853283,
4.38404576908119));
#16926=CARTESIAN_POINT('Ctrl Pts',(-15.751473444106,-17.4054630353252,4.37300058810609));
#16927=CARTESIAN_POINT('Ctrl Pts',(-15.2513705135099,-17.4045485352596,
4.3511238194886));
#16928=CARTESIAN_POINT('Ctrl Pts',(-15.008583912302,-17.3567842193863,4.34050323325904));
#16929=CARTESIAN_POINT('Ctrl Pts',(-14.5534149045375,-17.1714240828892,
4.32059207806375));
#16930=CARTESIAN_POINT('Ctrl Pts',(-14.3455007806179,-17.0351933676591,
4.31157422775254));
#16931=CARTESIAN_POINT('Ctrl Pts',(-13.9890741217456,-16.6872392691384,
4.29059651917396));
#16932=CARTESIAN_POINT('Ctrl Pts',(-13.8455457084443,-16.4773475914728,
4.27950571726879));
#16933=CARTESIAN_POINT('Ctrl Pts',(-13.6521281424843,-16.0226193093072,
4.25804836699955));
#16934=CARTESIAN_POINT('Ctrl Pts',(-13.6006825475756,-15.7835100066402,
4.24786474810868));
#16935=CARTESIAN_POINT('Ctrl Pts',(-13.5899924845278,-15.2888905024329,
4.22889282827602));
#16936=CARTESIAN_POINT('Ctrl Pts',(-13.6347157041402,-15.0379852516787,
4.21862841815223));
#16937=CARTESIAN_POINT('Ctrl Pts',(-13.8180666535794,-14.571561386154,4.196948173568));
#16938=CARTESIAN_POINT('Ctrl Pts',(-13.9535367820056,-14.3601081049675,
4.18597446501882));
#16939=CARTESIAN_POINT('Ctrl Pts',(-14.2928560730081,-14.0066800250512,
4.16516355770824));
#16940=CARTESIAN_POINT('Ctrl Pts',(-14.491402872933,-13.8660108828828,4.15612060923297));
#16941=CARTESIAN_POINT('Ctrl Pts',(-14.9406933821584,-13.6615396576274,
4.13646660620472));
#16942=CARTESIAN_POINT('Ctrl Pts',(-15.1889677026202,-13.6036879578437,
4.125605962265));
#16943=CARTESIAN_POINT('Ctrl Pts',(-15.6870665518806,-13.5883237572087,
4.10381686124748));
#16944=CARTESIAN_POINT('Ctrl Pts',(-15.9320384291794,-13.6284081520162,
4.09310068113817));
#16945=CARTESIAN_POINT('Ctrl Pts',(-16.3918885303663,-13.7990130324649,
4.07298475370218));
#16946=CARTESIAN_POINT('Ctrl Pts',(-16.6026210354757,-13.9274064325583,
4.0641257857171));
#16947=CARTESIAN_POINT('Ctrl Pts',(-16.9700749212964,-14.2623619608257,
4.04339932292059));
#16948=CARTESIAN_POINT('Ctrl Pts',(-17.1210819760315,-14.4680350747609,
4.03230476172588));
#16949=CARTESIAN_POINT('Ctrl Pts',(-17.3300204514864,-14.9176282407073,
4.01070247210187));
#16950=CARTESIAN_POINT('Ctrl Pts',(-17.3893434322323,-15.15571156755,4.00038542487369));
#16951=CARTESIAN_POINT('Ctrl Pts',(-17.4041002263905,-15.4323602839601,
3.98958213469807));
#16952=CARTESIAN_POINT('Ctrl Pts',(-17.405,-15.4661957188126,3.98828063719431));
#16953=CARTESIAN_POINT('Ctrl Pts',(-17.405,-15.5,3.98699999999987));
#16954=CARTESIAN_POINT('Origin',(-15.5,-15.5,-1.713));
#16955=CARTESIAN_POINT('',(-17.405,-15.5,3.42449999999993));
#16956=CARTESIAN_POINT('',(-17.405,-15.4999999999999,3.48699999999987));
#16957=CARTESIAN_POINT('',(-17.405,-15.5,-1.713));
#16958=CARTESIAN_POINT('Ctrl Pts',(-17.405,-15.4999999999999,3.42449999999993));
#16959=CARTESIAN_POINT('Ctrl Pts',(-17.405,-15.4614919273425,3.42595883504683));
#16960=CARTESIAN_POINT('Ctrl Pts',(-17.4038324068547,-15.422945623307,3.42744465635428));
#16961=CARTESIAN_POINT('Ctrl Pts',(-17.3867253555674,-15.1415209695274,
3.43848028299768));
#16962=CARTESIAN_POINT('Ctrl Pts',(-17.3255583499887,-14.9037152031145,
3.44882714816257));
#16963=CARTESIAN_POINT('Ctrl Pts',(-17.1130008469439,-14.4554002870608,
3.47046016906023));
#16964=CARTESIAN_POINT('Ctrl Pts',(-16.9602578707828,-14.2507531198155,
3.48155383195293));
#16965=CARTESIAN_POINT('Ctrl Pts',(-16.5902498287586,-13.9188606573106,
3.50222011912992));
#16966=CARTESIAN_POINT('Ctrl Pts',(-16.3788495907395,-13.7922914531921,
3.51105513601302));
#16967=CARTESIAN_POINT('Ctrl Pts',(-15.917910107173,-13.6251789794874,3.53121871797131));
#16968=CARTESIAN_POINT('Ctrl Pts',(-15.6724556370897,-13.5869268055474,
3.5419560088761));
#16969=CARTESIAN_POINT('Ctrl Pts',(-15.1743158902438,-13.6061504385889,
3.56374689893934));
#16970=CARTESIAN_POINT('Ctrl Pts',(-14.9265037515429,-13.6659174378174,
3.57458732495425));
#16971=CARTESIAN_POINT('Ctrl Pts',(-14.4788704801155,-13.8738228385912,
3.59416883289068));
#16972=CARTESIAN_POINT('Ctrl Pts',(-14.2814591404654,-14.0159749912975,
3.60326496379597));
#16973=CARTESIAN_POINT('Ctrl Pts',(-13.9447558345002,-14.3720760147507,
3.62411991504735));
#16974=CARTESIAN_POINT('Ctrl Pts',(-13.8108291603664,-14.5847429374719,
3.63510584219906));
#16975=CARTESIAN_POINT('Ctrl Pts',(-13.6311050735004,-15.0528032762474,
3.65676875503005));
#16976=CARTESIAN_POINT('Ctrl Pts',(-13.5883709031569,-15.3040785387128,
3.66693274229893));
#16977=CARTESIAN_POINT('Ctrl Pts',(-13.6030062776106,-15.7988175390939,
3.6859954820102));
#16978=CARTESIAN_POINT('Ctrl Pts',(-13.6564327241794,-16.0376931449921,
3.69621357327602));
#16979=CARTESIAN_POINT('Ctrl Pts',(-13.8537624689396,-16.4911796393931,
3.71770944802686));
#16980=CARTESIAN_POINT('Ctrl Pts',(-13.9991810599468,-16.7000354706043,
3.72880235052296));
#16981=CARTESIAN_POINT('Ctrl Pts',(-14.358399335272,-17.0447335767602,3.74971776846828));
#16982=CARTESIAN_POINT('Ctrl Pts',(-14.5670178084669,-17.1789859548373,
3.75868713072889));
#16983=CARTESIAN_POINT('Ctrl Pts',(-15.0233682881308,-17.3606593439805,
3.77864996885944));
#16984=CARTESIAN_POINT('Ctrl Pts',(-15.2667228742052,-17.4065145378553,
3.78929540132114));
#16985=CARTESIAN_POINT('Ctrl Pts',(-15.7644940064487,-17.4033641976423,
3.81107016651116));
#16986=CARTESIAN_POINT('Ctrl Pts',(-16.0141322276006,-17.3516042446948,
3.82199047364817));
#16987=CARTESIAN_POINT('Ctrl Pts',(-16.4686139608441,-17.1580516102408,
3.84187156434124));
#16988=CARTESIAN_POINT('Ctrl Pts',(-16.6707818008129,-17.0220465010016,
3.85077996346433));
#16989=CARTESIAN_POINT('Ctrl Pts',(-17.0182773444189,-16.6770468578599,
3.8714504020934));
#16990=CARTESIAN_POINT('Ctrl Pts',(-17.158527732642,-16.4694767325026,3.88238155676259));
#16991=CARTESIAN_POINT('Ctrl Pts',(-17.3531512510743,-16.008436647136,3.90410439951443));
#16992=CARTESIAN_POINT('Ctrl Pts',(-17.4041360722943,-15.758785953557,3.91467728898608));
#16993=CARTESIAN_POINT('Ctrl Pts',(-17.4049963723817,-15.5042929847283,
3.92433728575485));
#16994=CARTESIAN_POINT('Ctrl Pts',(-17.4050000000196,-15.5021464040978,
3.92441868589383));
#16995=CARTESIAN_POINT('Ctrl Pts',(-17.405,-15.4999999826177,3.92450000065845));
#16996=CARTESIAN_POINT('Ctrl Pts',(-17.405,-15.5,3.98699999999987));
#16997=CARTESIAN_POINT('Ctrl Pts',(-17.405,-15.7183764833957,3.97872705239665));
#16998=CARTESIAN_POINT('Ctrl Pts',(-17.3674531932618,-15.9353913916047,
3.96968445279574));
#16999=CARTESIAN_POINT('Ctrl Pts',(-17.2097145334027,-16.3764419074438,
3.94952564785269));
#17000=CARTESIAN_POINT('Ctrl Pts',(-17.0803549969663,-16.5925903400615,
3.93850772126244));
#17001=CARTESIAN_POINT('Ctrl Pts',(-16.7513322330662,-16.9564719188534,
3.91752600327675));
#17002=CARTESIAN_POINT('Ctrl Pts',(-16.5571928795373,-17.1029549283145,
3.90824640767878));
#17003=CARTESIAN_POINT('Ctrl Pts',(-16.1144115409643,-17.3207811248282,
3.88887714527401));
#17004=CARTESIAN_POINT('Ctrl Pts',(-15.8680240062267,-17.3860756932498,
3.87809903789266));
#17005=CARTESIAN_POINT('Ctrl Pts',(-15.3699354945413,-17.4164903327027,
3.85631038908753));
#17006=CARTESIAN_POINT('Ctrl Pts',(-15.1231588456645,-17.3835747241081,
3.8455152600903));
#17007=CARTESIAN_POINT('Ctrl Pts',(-14.6591026105995,-17.2265810198167,
3.82521533729657));
#17008=CARTESIAN_POINT('Ctrl Pts',(-14.4457643415342,-17.1052342882286,
3.81642064056864));
#17009=CARTESIAN_POINT('Ctrl Pts',(-14.0684720259498,-16.7821838800442,
3.79593000111182));
#17010=CARTESIAN_POINT('Ctrl Pts',(-13.9107751972146,-16.5805645695418,
3.78484269318721));
#17011=CARTESIAN_POINT('Ctrl Pts',(-13.6878549632812,-16.1360821099788,
3.76312820418961));
#17012=CARTESIAN_POINT('Ctrl Pts',(-13.6213923552747,-15.8991527642048,
3.75269871441071));
#17013=CARTESIAN_POINT('Ctrl Pts',(-13.5809017461053,-15.4067401086061,
3.73315859308621));
#17014=CARTESIAN_POINT('Ctrl Pts',(-13.6097237057755,-15.155749122147,3.7236364016455));
#17015=CARTESIAN_POINT('Ctrl Pts',(-13.7627857675895,-14.6791704166862,
3.702233938971));
#17016=CARTESIAN_POINT('Ctrl Pts',(-13.8855451897592,-14.4582664818264,
3.69118021497846));
#17017=CARTESIAN_POINT('Ctrl Pts',(-14.2036046789724,-14.0834550905506,
3.67002422499248));
#17018=CARTESIAN_POINT('Ctrl Pts',(-14.3932240200836,-13.9308436246418,
3.66041539719665));
#17019=CARTESIAN_POINT('Ctrl Pts',(-14.8291239419257,-13.6992634410876,
3.64134715914579));
#17020=CARTESIAN_POINT('Ctrl Pts',(-15.0733167129576,-13.6263288506664,
3.63066506067544));
#17021=CARTESIAN_POINT('Ctrl Pts',(-15.57091270054,-13.5803148558224,3.60889795710666));
#17022=CARTESIAN_POINT('Ctrl Pts',(-15.8193408380043,-13.6057324145129,
3.59803058451417));
#17023=CARTESIAN_POINT('Ctrl Pts',(-16.2876421974074,-13.7486242565046,
3.57754496074325));
#17024=CARTESIAN_POINT('Ctrl Pts',(-16.5036951881227,-13.8628408826526,
3.56873551144344));
#17025=CARTESIAN_POINT('Ctrl Pts',(-16.8908612944749,-14.1736570247294,
3.54849239122817));
#17026=CARTESIAN_POINT('Ctrl Pts',(-17.0552700892148,-14.3709294205846,
3.53742295537314));
#17027=CARTESIAN_POINT('Ctrl Pts',(-17.292316215799,-14.8097683997458,3.51561329800583));
#17028=CARTESIAN_POINT('Ctrl Pts',(-17.3660349623944,-15.0453043822237,
3.50507788603606));
#17029=CARTESIAN_POINT('Ctrl Pts',(-17.4010777344063,-15.3587618909951,
3.49243643583445));
#17030=CARTESIAN_POINT('Ctrl Pts',(-17.405,-15.4294197625975,3.48967385295681));
#17031=CARTESIAN_POINT('Ctrl Pts',(-17.405,-15.4999999999999,3.48699999999987));
#17032=CARTESIAN_POINT('Origin',(-15.5,-15.5,-1.713));
#17033=CARTESIAN_POINT('',(-17.405,-15.4999999999999,2.92449999999993));
#17034=CARTESIAN_POINT('',(-17.405,-15.5,2.98699999999986));
#17035=CARTESIAN_POINT('',(-17.405,-15.5,-1.713));
#17036=CARTESIAN_POINT('Ctrl Pts',(-17.405,-15.4999999999999,2.92449999999993));
#17037=CARTESIAN_POINT('Ctrl Pts',(-17.405,-15.4246029704291,2.92735633171377));
#17038=CARTESIAN_POINT('Ctrl Pts',(-17.4005241425492,-15.3491261289197,
2.93031358415772));
#17039=CARTESIAN_POINT('Ctrl Pts',(-17.3625026971922,-15.030949658235,2.94319895726262));
#17040=CARTESIAN_POINT('Ctrl Pts',(-17.2869039689406,-14.7958112749887,
2.95376042609122));
#17041=CARTESIAN_POINT('Ctrl Pts',(-17.0462119101931,-14.3585090291066,
2.97559161084361));
#17042=CARTESIAN_POINT('Ctrl Pts',(-16.8800785444847,-14.1624005620978,
2.98665467283752));
#17043=CARTESIAN_POINT('Ctrl Pts',(-16.4903722843864,-13.8547788324716,
3.00683233524616));
#17044=CARTESIAN_POINT('Ctrl Pts',(-16.2736016230491,-13.7424065889116,
3.01565915909658));
#17045=CARTESIAN_POINT('Ctrl Pts',(-15.8042055235872,-13.6032175602641,
3.03619267175896));
#17046=CARTESIAN_POINT('Ctrl Pts',(-15.5553810743812,-13.5797787576298,
3.04707738082309));
#17047=CARTESIAN_POINT('Ctrl Pts',(-15.0579955564868,-13.6298855017054,
3.06883527749388));
#17048=CARTESIAN_POINT('Ctrl Pts',(-14.8144188605694,-13.7048120123677,
3.07949042604668));
#17049=CARTESIAN_POINT('Ctrl Pts',(-14.3803478613073,-13.9399897068444,
3.09847865873529));
#17050=CARTESIAN_POINT('Ctrl Pts',(-14.1919085752892,-14.0942297674633,
3.10818823180623));
#17051=CARTESIAN_POINT('Ctrl Pts',(-13.8767794458615,-14.4719269225963,
3.12938945210352));
#17052=CARTESIAN_POINT('Ctrl Pts',(-13.7557980800781,-14.6940588916751,
3.14045080866986));
#17053=CARTESIAN_POINT('Ctrl Pts',(-13.6069962562461,-15.1715532833019,
3.16179478002723));
#17054=CARTESIAN_POINT('Ctrl Pts',(-13.5802964278705,-15.4221320121638,
3.17122845836935));
#17055=CARTESIAN_POINT('Ctrl Pts',(-13.6245367961492,-15.913784746089,3.190821806644));
#17056=CARTESIAN_POINT('Ctrl Pts',(-13.6929081588293,-16.1503692156979,
3.20127997996693));
#17057=CARTESIAN_POINT('Ctrl Pts',(-13.9195525061294,-16.5934112583634,
3.22302135518752));
#17058=CARTESIAN_POINT('Ctrl Pts',(-14.0790234790521,-16.7939093902312,
3.23410499307334));
#17059=CARTESIAN_POINT('Ctrl Pts',(-14.4589246323286,-17.1137556039747,
3.25453130641737));
#17060=CARTESIAN_POINT('Ctrl Pts',(-14.6729691488013,-17.2332242138591,
3.26332192251953));
#17061=CARTESIAN_POINT('Ctrl Pts',(-15.1381451842514,-17.3865362903766,
3.28367083045699));
#17062=CARTESIAN_POINT('Ctrl Pts',(-15.3853746064769,-17.4175006398182,
3.29448576581245));
#17063=CARTESIAN_POINT('Ctrl Pts',(-15.8833818147483,-17.3830125865093,
3.3162708580378));
#17064=CARTESIAN_POINT('Ctrl Pts',(-16.1292196923062,-17.3157156943741,
3.32702492092311));
#17065=CARTESIAN_POINT('Ctrl Pts',(-16.570217563795,-17.0942905219578,3.34631616639506));
#17066=CARTESIAN_POINT('Ctrl Pts',(-16.7631725989519,-16.9462183677401,
3.35567342316665));
#17067=CARTESIAN_POINT('Ctrl Pts',(-17.0893626738479,-16.5794927492161,
3.37670092707341));
#17068=CARTESIAN_POINT('Ctrl Pts',(-17.2170253917602,-16.3620913328898,
3.38772920827698));
#17069=CARTESIAN_POINT('Ctrl Pts',(-17.3693031954026,-15.9246324502421,
3.40763250693426));
#17070=CARTESIAN_POINT('Ctrl Pts',(-17.405,-15.7129299879628,3.41643338675393));
#17071=CARTESIAN_POINT('Ctrl Pts',(-17.405,-15.4999999999999,3.42449999999993));
#17072=CARTESIAN_POINT('Ctrl Pts',(-17.405,-15.4999999999999,3.48699999999987));
#17073=CARTESIAN_POINT('Ctrl Pts',(-17.405,-15.6764531477386,3.4803152708433));
#17074=CARTESIAN_POINT('Ctrl Pts',(-17.3804873179637,-15.8523801803092,
3.47311432506748));
#17075=CARTESIAN_POINT('Ctrl Pts',(-17.2629771594338,-16.2641939190073,
3.45494301104277));
#17076=CARTESIAN_POINT('Ctrl Pts',(-17.147005924465,-16.4896706537741,3.4438645247018));
#17077=CARTESIAN_POINT('Ctrl Pts',(-16.8400905328106,-16.8753750105602,
3.42253961362769));
#17078=CARTESIAN_POINT('Ctrl Pts',(-16.6549001286324,-17.0341609160333,
3.41252056555695));
#17079=CARTESIAN_POINT('Ctrl Pts',(-16.2259290516944,-17.2792504677336,
3.39375542658327));
#17080=CARTESIAN_POINT('Ctrl Pts',(-15.9841393868079,-17.3596471123229,
3.38317845086646));
#17081=CARTESIAN_POINT('Ctrl Pts',(-15.4875102619216,-17.4210491324768,
3.36145364225377));
#17082=CARTESIAN_POINT('Ctrl Pts',(-15.2376720328314,-17.4030964029156,
3.35052458586313));
#17083=CARTESIAN_POINT('Ctrl Pts',(-14.7652944961111,-17.2741400167745,
3.3298606516234));
#17084=CARTESIAN_POINT('Ctrl Pts',(-14.546527920475,-17.1668079458835,3.32095721717422));
#17085=CARTESIAN_POINT('Ctrl Pts',(-14.1499117418974,-16.8679726763458,
3.30096128435465));
#17086=CARTESIAN_POINT('Ctrl Pts',(-13.9790956107818,-16.6751252050885,
3.28991933882874));
#17087=CARTESIAN_POINT('Ctrl Pts',(-13.7284685714235,-16.2421809384311,
3.26803595068229));
#17088=CARTESIAN_POINT('Ctrl Pts',(-13.6477317959478,-16.0082067494623,
3.25740620530981));
#17089=CARTESIAN_POINT('Ctrl Pts',(-13.5792898836175,-15.5216378862272,
3.23747611115332));
#17090=CARTESIAN_POINT('Ctrl Pts',(-13.5925554052722,-15.2736030156638,
3.22847667356028));
#17091=CARTESIAN_POINT('Ctrl Pts',(-13.7141357063192,-14.7906605136231,
3.2075217030503));
#17092=CARTESIAN_POINT('Ctrl Pts',(-13.8234698343903,-14.5610040823231,
3.19643004217174));
#17093=CARTESIAN_POINT('Ctrl Pts',(-14.1194602955704,-14.1651196850214,
3.17495842469075));
#17094=CARTESIAN_POINT('Ctrl Pts',(-14.3003771223459,-14.0004255695162,
3.16476211229926));
#17095=CARTESIAN_POINT('Ctrl Pts',(-14.7227040856981,-13.7425835691326,
3.14575681027953));
#17096=CARTESIAN_POINT('Ctrl Pts',(-14.9621109288452,-13.6551633959072,
3.13552970564974));
#17097=CARTESIAN_POINT('Ctrl Pts',(-15.4575797798197,-13.5792882748642,
3.11385565267621));
#17098=CARTESIAN_POINT('Ctrl Pts',(-15.7085427300214,-13.5901710364673,
3.10287739588699));
#17099=CARTESIAN_POINT('Ctrl Pts',(-16.1846495764087,-13.7059977045008,
3.08205032474143));
#17100=CARTESIAN_POINT('Ctrl Pts',(-16.4060079774435,-13.8069773445162,
3.07298847944479));
#17101=CARTESIAN_POINT('Ctrl Pts',(-16.8085181321564,-14.0926836357192,
3.05336100859792));
#17102=CARTESIAN_POINT('Ctrl Pts',(-16.9832809666978,-14.2782731379037,
3.04250769972486));
#17103=CARTESIAN_POINT('Ctrl Pts',(-17.2468705889534,-14.7012659478552,
3.02071779026886));
#17104=CARTESIAN_POINT('Ctrl Pts',(-17.3353128781264,-14.9332790215386,
3.00999380249955));
#17105=CARTESIAN_POINT('Ctrl Pts',(-17.3957395224265,-15.2830534969887,
2.99542132203213));
#17106=CARTESIAN_POINT('Ctrl Pts',(-17.405,-15.3915468179105,2.99110862689446));
#17107=CARTESIAN_POINT('Ctrl Pts',(-17.405,-15.5,2.98699999999986));
#17108=CARTESIAN_POINT('Origin',(-15.5,-15.5,-1.713));
#17109=CARTESIAN_POINT('',(-17.405,-15.5,2.42449999999992));
#17110=CARTESIAN_POINT('',(-17.405,-15.5,2.48699999999985));
#17111=CARTESIAN_POINT('',(-17.405,-15.5,-1.713));
#17112=CARTESIAN_POINT('Ctrl Pts',(-17.405,-15.5,2.42449999999992));
#17113=CARTESIAN_POINT('Ctrl Pts',(-17.405,-15.3866287216877,2.42879494344165));
#17114=CARTESIAN_POINT('Ctrl Pts',(-17.3948806441803,-15.2732338375239,
2.43331211440638));
#17115=CARTESIAN_POINT('Ctrl Pts',(-17.330832577681,-14.9188879456016,2.44813698655778));
#17116=CARTESIAN_POINT('Ctrl Pts',(-17.2404900805375,-14.6873986588248,
2.45888269310303));
#17117=CARTESIAN_POINT('Ctrl Pts',(-16.973408577859,-14.2663867214871,2.48067393476401));
#17118=CARTESIAN_POINT('Ctrl Pts',(-16.7971653949025,-14.0822139660179,
2.49150595035454));
#17119=CARTESIAN_POINT('Ctrl Pts',(-16.3924276582491,-13.799788061525,2.51105786970293));
#17120=CARTESIAN_POINT('Ctrl Pts',(-16.1703213448218,-13.7006022327362,
2.52017710652558));
#17121=CARTESIAN_POINT('Ctrl Pts',(-15.6931687253924,-13.5885289569252,
2.54104992452337));
#17122=CARTESIAN_POINT('Ctrl Pts',(-15.4419207498431,-13.5796720432962,
2.55204064961302));
#17123=CARTESIAN_POINT('Ctrl Pts',(-14.9448705760937,-13.6599948516569,
2.57378387681115));
#17124=CARTESIAN_POINT('Ctrl Pts',(-14.7043542991087,-13.7505153330003,
2.58395864765043));
#17125=CARTESIAN_POINT('Ctrl Pts',(-14.2830278447516,-14.0144258842274,
2.60317196649853));
#17126=CARTESIAN_POINT('Ctrl Pts',(-14.1038402602375,-14.1814147098486,
2.61341738895667));
#17127=CARTESIAN_POINT('Ctrl Pts',(-13.8122359953876,-14.5812645112853,
2.63494329526319));
#17128=CARTESIAN_POINT('Ctrl Pts',(-13.7055635984876,-14.8125202663001,
2.64603732663082));
#17129=CARTESIAN_POINT('Ctrl Pts',(-13.5900531890772,-15.2965866386149,
2.66690211141856));
#17130=CARTESIAN_POINT('Ctrl Pts',(-13.5797585477662,-15.5440797481913,
2.67583654661438));
#17131=CARTESIAN_POINT('Ctrl Pts',(-13.6536576949259,-16.0294590950737,
2.69584093937257));
#17132=CARTESIAN_POINT('Ctrl Pts',(-13.7371892876536,-16.2627520080675,
2.70650600435679));
#17133=CARTESIAN_POINT('Ctrl Pts',(-13.9917092405621,-16.6907175631168,
2.7282859264509));
#17134=CARTESIAN_POINT('Ctrl Pts',(-14.1626016047602,-16.8799033597708,
2.73919082094069));
#17135=CARTESIAN_POINT('Ctrl Pts',(-14.5593214870997,-17.1740429974242,
2.7590111332608));
#17136=CARTESIAN_POINT('Ctrl Pts',(-14.7787835918848,-17.2796492651576,
2.76795072580402));
#17137=CARTESIAN_POINT('Ctrl Pts',(-15.252177850505,-17.4050640088115,2.78865913606738));
#17138=CARTESIAN_POINT('Ctrl Pts',(-15.5023389993631,-17.4211126319878,
2.79960231843214));
#17139=CARTESIAN_POINT('Ctrl Pts',(-15.9987461698247,-17.3557948735195,
2.82131741775242));
#17140=CARTESIAN_POINT('Ctrl Pts',(-16.2398924930437,-17.2734770843301,
2.83183027289843));
#17141=CARTESIAN_POINT('Ctrl Pts',(-16.6670901386329,-17.0249503089065,
2.85058921094883));
#17142=CARTESIAN_POINT('Ctrl Pts',(-16.8511310705029,-16.8645487287507,
2.86069123672124));
#17143=CARTESIAN_POINT('Ctrl Pts',(-17.1551013135425,-16.4761253349775,
2.88205473838143));
#17144=CARTESIAN_POINT('Ctrl Pts',(-17.2693013185321,-16.2495057733069,
2.89313777862186));
#17145=CARTESIAN_POINT('Ctrl Pts',(-17.3819592475714,-15.8416977694031,
2.91105121063268));
#17146=CARTESIAN_POINT('Ctrl Pts',(-17.405,-15.6710735741344,2.91801906994232));
#17147=CARTESIAN_POINT('Ctrl Pts',(-17.405,-15.4999999999999,2.92449999999993));
#17148=CARTESIAN_POINT('Ctrl Pts',(-17.405,-15.5,2.98699999999986));
#17149=CARTESIAN_POINT('Ctrl Pts',(-17.405,-15.6348413314497,2.98189168772884));
#17150=CARTESIAN_POINT('Ctrl Pts',(-17.3906852736361,-15.7695966035171,
2.97647354021857));
#17151=CARTESIAN_POINT('Ctrl Pts',(-17.3087652033694,-16.1490564386062,
2.96030635334035));
#17152=CARTESIAN_POINT('Ctrl Pts',(-17.2067942988799,-16.3830339576779,
2.94921204329331));
#17153=CARTESIAN_POINT('Ctrl Pts',(-16.922972583008,-16.7896948145866,2.92759832978747));
#17154=CARTESIAN_POINT('Ctrl Pts',(-16.7468731843496,-16.9606478650304,
2.91727027275038));
#17155=CARTESIAN_POINT('Ctrl Pts',(-16.3321205610298,-17.2321519637799,
2.89791306547092));
#17156=CARTESIAN_POINT('Ctrl Pts',(-16.0954586961872,-17.3270829461848,
2.88804806195041));
#17157=CARTESIAN_POINT('Ctrl Pts',(-15.6017485836216,-17.418582659013,2.86645094416539));
#17158=CARTESIAN_POINT('Ctrl Pts',(-15.3497898078031,-17.4153981809549,
2.85542912545068));
#17159=CARTESIAN_POINT('Ctrl Pts',(-14.8697620227219,-17.3138206140289,
2.83443053467723));
#17160=CARTESIAN_POINT('Ctrl Pts',(-14.6455467021456,-17.2196022923227,
2.82512303677297));
#17161=CARTESIAN_POINT('Ctrl Pts',(-14.2346929933562,-16.9462855801242,
2.80578243876608));
#17162=CARTESIAN_POINT('Ctrl Pts',(-14.0544139525623,-16.7660972674064,
2.79501309595437));
#17163=CARTESIAN_POINT('Ctrl Pts',(-13.7777445899928,-16.3507193868928,
2.7732255859815));
#17164=CARTESIAN_POINT('Ctrl Pts',(-13.6821563903077,-16.1207596787417,
2.76242309040195));
#17165=CARTESIAN_POINT('Ctrl Pts',(-13.5847088675459,-15.6406980901775,
2.74210509860585));
#17166=CARTESIAN_POINT('Ctrl Pts',(-13.5823994058797,-15.3953897232232,
2.73331256079938));
#17167=CARTESIAN_POINT('Ctrl Pts',(-13.6720198072411,-14.9068760737457,
2.71284556905731));
#17168=CARTESIAN_POINT('Ctrl Pts',(-13.7670951492794,-14.6691356899221,
2.70175952868478));
#17169=CARTESIAN_POINT('Ctrl Pts',(-14.0394246976334,-14.2529140471301,
2.6800349752972));
#17170=CARTESIAN_POINT('Ctrl Pts',(-14.2109198649204,-14.0763443783639,
2.66959484396155));
#17171=CARTESIAN_POINT('Ctrl Pts',(-14.6161830495051,-13.7940142570894,
2.65003506051579));
#17172=CARTESIAN_POINT('Ctrl Pts',(-14.847434530759,-13.6928766622502,2.64054617100783));
#17173=CARTESIAN_POINT('Ctrl Pts',(-15.3362030982655,-13.5856111981726,
2.61916521879844));
#17174=CARTESIAN_POINT('Ctrl Pts',(-15.5889576943258,-13.5806775350222,
2.60810858729974));
#17175=CARTESIAN_POINT('Ctrl Pts',(-16.072966293995,-13.6672512129721,2.58693585765542));
#17176=CARTESIAN_POINT('Ctrl Pts',(-16.30024349174,-13.7544824009695,2.57729050033427));
#17177=CARTESIAN_POINT('Ctrl Pts',(-16.719562151595,-14.0149434292219,2.5582517778019));
#17178=CARTESIAN_POINT('Ctrl Pts',(-16.9053469084664,-14.18938943058,2.54757955351491));
#17179=CARTESIAN_POINT('Ctrl Pts',(-17.1952671189457,-14.5964930079793,
2.52581568014487));
#17180=CARTESIAN_POINT('Ctrl Pts',(-17.2981758603756,-14.8241099078218,
2.51494182238855));
#17181=CARTESIAN_POINT('Ctrl Pts',(-17.3881884443977,-15.2079235803331,
2.4984326936604));
#17182=CARTESIAN_POINT('Ctrl Pts',(-17.405,-15.3538704367668,2.49253595424323));
#17183=CARTESIAN_POINT('Ctrl Pts',(-17.405,-15.5,2.48699999999985));
#17184=CARTESIAN_POINT('Origin',(-15.5,-15.5,-1.713));
#17185=CARTESIAN_POINT('',(-17.405,-15.5,1.92449999999991));
#17186=CARTESIAN_POINT('',(-17.405,-15.5000000000001,1.98699999999984));
#17187=CARTESIAN_POINT('',(-17.405,-15.5,-1.713));
#17188=CARTESIAN_POINT('Ctrl Pts',(-17.405,-15.5,1.92449999999991));
#17189=CARTESIAN_POINT('Ctrl Pts',(-17.405,-15.3486986793144,1.93023188046098));
#17190=CARTESIAN_POINT('Ctrl Pts',(-17.3869774740474,-15.1976302972843,
1.93634912978389));
#17191=CARTESIAN_POINT('Ctrl Pts',(-17.2925795312766,-14.8093323449348,
1.95312405814599));
#17192=CARTESIAN_POINT('Ctrl Pts',(-17.1877032252396,-14.582387157065,1.96401550394565));
#17193=CARTESIAN_POINT('Ctrl Pts',(-16.8942477032967,-14.1775904447064,
1.9857693095993));
#17194=CARTESIAN_POINT('Ctrl Pts',(-16.7070086756833,-14.0047243622716,
1.99641348863026));
#17195=CARTESIAN_POINT('Ctrl Pts',(-16.2854263826576,-13.7477497935979,
2.01536964134727));
#17196=CARTESIAN_POINT('Ctrl Pts',(-16.0573006855409,-13.6624109872575,
2.02512114236464));
#17197=CARTESIAN_POINT('Ctrl Pts',(-15.5722291432103,-13.579946666267,2.04634036993816));
#17198=CARTESIAN_POINT('Ctrl Pts',(-15.3193016253507,-13.5871036514588,
2.05740456582003));
#17199=CARTESIAN_POINT('Ctrl Pts',(-14.8319183237239,-13.6986435441608,
2.07872492022189));
#17200=CARTESIAN_POINT('Ctrl Pts',(-14.6021272930825,-13.8014628299617,
2.08812467256909));
#17201=CARTESIAN_POINT('Ctrl Pts',(-14.1994820415506,-14.0867521555902,
2.10773930201741));
#17202=CARTESIAN_POINT('Ctrl Pts',(-14.029286629017,-14.2648482619827,2.11820883214505));
#17203=CARTESIAN_POINT('Ctrl Pts',(-13.7601789517598,-14.6836493550942,
2.13996063548694));
#17204=CARTESIAN_POINT('Ctrl Pts',(-13.6670272894183,-14.9223925914719,
2.15104259256723));
#17205=CARTESIAN_POINT('Ctrl Pts',(-13.5816226349698,-15.4115802655974,
2.17144291103771));
#17206=CARTESIAN_POINT('Ctrl Pts',(-13.5859774200922,-15.6565526410676,
2.18023347656324));
#17207=CARTESIAN_POINT('Ctrl Pts',(-13.6873032473563,-16.1357098037595,
2.20060203250936));
#17208=CARTESIAN_POINT('Ctrl Pts',(-13.7848735554849,-16.3650593087161,
2.21142476442983));
#17209=CARTESIAN_POINT('Ctrl Pts',(-14.0651457198649,-16.7782445247767,
2.23320800921402));
#17210=CARTESIAN_POINT('Ctrl Pts',(-14.2469301421843,-16.9568990841518,
2.24395217360948));
#17211=CARTESIAN_POINT('Ctrl Pts',(-14.6600831874615,-17.2267522515104,
2.26321185081259));
#17212=CARTESIAN_POINT('Ctrl Pts',(-14.8851133202991,-17.319086036431,2.27260207000412));
#17213=CARTESIAN_POINT('Ctrl Pts',(-15.3662227564387,-17.4166438315601,
2.29364797709685));
#17214=CARTESIAN_POINT('Ctrl Pts',(-15.6184201448337,-17.4176538394308,
2.30468023380706));
#17215=CARTESIAN_POINT('Ctrl Pts',(-16.1108249144034,-17.3219057393829,
2.32622024997372));
#17216=CARTESIAN_POINT('Ctrl Pts',(-16.3460254825939,-17.2253010985772,
2.33597673494084));
#17217=CARTESIAN_POINT('Ctrl Pts',(-16.7582463484608,-16.9508932005934,
2.35538857411786));
#17218=CARTESIAN_POINT('Ctrl Pts',(-16.9331340337932,-16.7784291356177,
2.36574737132588));
#17219=CARTESIAN_POINT('Ctrl Pts',(-17.2139188972246,-16.3691856695095,
2.38739250123395));
#17220=CARTESIAN_POINT('Ctrl Pts',(-17.3140623235137,-16.1341848427474,
2.39848560705332));
#17221=CARTESIAN_POINT('Ctrl Pts',(-17.3917862251892,-15.759050717556,2.41439713955902));
#17222=CARTESIAN_POINT('Ctrl Pts',(-17.405,-15.6295518546112,2.41959207361318));
#17223=CARTESIAN_POINT('Ctrl Pts',(-17.405,-15.5,2.42449999999992));
#17224=CARTESIAN_POINT('Ctrl Pts',(-17.405,-15.5,2.48699999999985));
#17225=CARTESIAN_POINT('Ctrl Pts',(-17.405,-15.5949683349577,2.48340223138093));
#17226=CARTESIAN_POINT('Ctrl Pts',(-17.3978991014891,-15.6900019365671,
2.47964667746751));
#17227=CARTESIAN_POINT('Ctrl Pts',(-17.3457037805944,-16.035815620742,2.46540428482014));
#17228=CARTESIAN_POINT('Ctrl Pts',(-17.2577563440206,-16.277172943574,2.45433712422308));
#17229=CARTESIAN_POINT('Ctrl Pts',(-16.9973983370484,-16.7027671265982,
2.43251934742135));
#17230=CARTESIAN_POINT('Ctrl Pts',(-16.8307514409228,-16.8849073795883,
2.42197422344043));
#17231=CARTESIAN_POINT('Ctrl Pts',(-16.4351306847412,-17.1780794189316,
2.40221460787432));
#17232=CARTESIAN_POINT('Ctrl Pts',(-16.2091894631102,-17.2853513335075,
2.3930231611159));
#17233=CARTESIAN_POINT('Ctrl Pts',(-15.7255640317756,-17.4082035102829,
2.37186719299102));
#17234=CARTESIAN_POINT('Ctrl Pts',(-15.4722692826481,-17.4212876437741,
2.36078693274924));
#17235=CARTESIAN_POINT('Ctrl Pts',(-14.9844212984852,-17.3497866434107,
2.33944625102733));
#17236=CARTESIAN_POINT('Ctrl Pts',(-14.7540109523672,-17.2694561740815,
2.32938405397293));
#17237=CARTESIAN_POINT('Ctrl Pts',(-14.3265001644784,-17.0217099393331,
2.31064783669698));
#17238=CARTESIAN_POINT('Ctrl Pts',(-14.1354929276868,-16.853069236674,2.30008131215583));
#17239=CARTESIAN_POINT('Ctrl Pts',(-13.8328034235953,-16.4545030489022,
2.27836157480911));
#17240=CARTESIAN_POINT('Ctrl Pts',(-13.7227580108401,-16.2294088619722,
2.26742719202244));
#17241=CARTESIAN_POINT('Ctrl Pts',(-13.5969187251782,-15.7561699905676,
2.24674667900731));
#17242=CARTESIAN_POINT('Ctrl Pts',(-13.5798018576392,-15.5131442345915,
2.23783037236436));
#17243=CARTESIAN_POINT('Ctrl Pts',(-13.6385605200307,-15.0227027697103,
2.21796536366566));
#17244=CARTESIAN_POINT('Ctrl Pts',(-13.7181303906783,-14.7804916560613,
2.2070490945133));
#17245=CARTESIAN_POINT('Ctrl Pts',(-13.9635498436067,-14.3473695137498,
2.18527286946309));
#17246=CARTESIAN_POINT('Ctrl Pts',(-14.1246435540447,-14.1592368872228,
2.17462219190088));
#17247=CARTESIAN_POINT('Ctrl Pts',(-14.5095940750912,-13.8542486731349,
2.15464831605754));
#17248=CARTESIAN_POINT('Ctrl Pts',(-14.7298789167439,-13.7403639765452,
2.14568858631908));
#17249=CARTESIAN_POINT('Ctrl Pts',(-15.2076990152618,-13.6007564602427,
2.12478656976098));
#17250=CARTESIAN_POINT('Ctrl Pts',(-15.4612907383838,-13.5787868978837,
2.1136933185308));
#17251=CARTESIAN_POINT('Ctrl Pts',(-15.9528706723896,-13.6337786144342,
2.0921893844098));
#17252=CARTESIAN_POINT('Ctrl Pts',(-16.1866229664858,-13.706554770831,2.08196399971618));
#17253=CARTESIAN_POINT('Ctrl Pts',(-16.6250552312494,-13.9417184916321,
2.06278498550955));
#17254=CARTESIAN_POINT('Ctrl Pts',(-16.8232548833612,-14.1060742689683,
2.05253139336743));
#17255=CARTESIAN_POINT('Ctrl Pts',(-17.1394238328743,-14.4983732171102,
2.03075425733394));
#17256=CARTESIAN_POINT('Ctrl Pts',(-17.2561233330502,-14.7208972749967,
2.01977170102725));
#17257=CARTESIAN_POINT('Ctrl Pts',(-17.3787284650258,-15.1353123617131,
2.00139039924266));
#17258=CARTESIAN_POINT('Ctrl Pts',(-17.405,-15.3173263053678,1.99392038758316));
#17259=CARTESIAN_POINT('Ctrl Pts',(-17.405,-15.5000000000001,1.98699999999984));
#17260=CARTESIAN_POINT('Origin',(-15.5,-15.5,-1.713));
#17261=CARTESIAN_POINT('',(-17.405,-15.5000000000001,1.4244999999999));
#17262=CARTESIAN_POINT('',(-17.405,-15.5,1.48699999999984));
#17263=CARTESIAN_POINT('',(-17.405,-15.5,-1.713));
#17264=CARTESIAN_POINT('Ctrl Pts',(-17.405,-15.5000000000001,1.42449999999991));
#17265=CARTESIAN_POINT('Ctrl Pts',(-17.405,-15.3118633378577,1.4316273459666));
#17266=CARTESIAN_POINT('Ctrl Pts',(-17.3771334387433,-15.1244839044587,
1.43933551001286));
#17267=CARTESIAN_POINT('Ctrl Pts',(-17.24934219222,-14.7057213235397,1.45799494380515));
#17268=CARTESIAN_POINT('Ctrl Pts',(-17.1306051942564,-14.4840272327072,
1.46899062243645));
#17269=CARTESIAN_POINT('Ctrl Pts',(-16.8113229405752,-14.0949843783885,
1.49071250003231));
#17270=CARTESIAN_POINT('Ctrl Pts',(-16.6123900156071,-13.9327769674847,
1.5008390194396));
#17271=CARTESIAN_POINT('Ctrl Pts',(-16.1726839958291,-13.7012553587294,
1.52007375346314));
#17272=CARTESIAN_POINT('Ctrl Pts',(-15.9381891396067,-13.6302529558287,
1.53033162118941));
#17273=CARTESIAN_POINT('Ctrl Pts',(-15.4457978890103,-13.5791344218338,
1.5518710459749));
#17274=CARTESIAN_POINT('Ctrl Pts',(-15.1921803263023,-13.603182159575,1.56296542754568));
#17275=CARTESIAN_POINT('Ctrl Pts',(-14.7157470931694,-13.7466772505015,
1.58380677632663));
#17276=CARTESIAN_POINT('Ctrl Pts',(-14.4967660670359,-13.8621014312398,
1.59272638657522));
#17277=CARTESIAN_POINT('Ctrl Pts',(-14.114338281745,-14.1698558360362,1.61274987849671));
#17278=CARTESIAN_POINT('Ctrl Pts',(-13.954584909938,-14.3593774914536,1.62342386161404));
#17279=CARTESIAN_POINT('Ctrl Pts',(-13.7125069078124,-14.7945807372207,
1.64520584182867));
#17280=CARTESIAN_POINT('Ctrl Pts',(-13.634853063525,-15.0374057231972,1.65610345900596));
#17281=CARTESIAN_POINT('Ctrl Pts',(-13.5799789460238,-15.5281670839837,
1.67589562280244));
#17282=CARTESIAN_POINT('Ctrl Pts',(-13.5989789668469,-15.7709288370138,
1.68485086346852));
#17283=CARTESIAN_POINT('Ctrl Pts',(-13.7284765422896,-16.243253711504,1.705576765825));
#17284=CARTESIAN_POINT('Ctrl Pts',(-13.8403731054317,-16.4676542695703,
1.71652536011545));
#17285=CARTESIAN_POINT('Ctrl Pts',(-14.1464186600125,-16.8640172845373,
1.73823503716585));
#17286=CARTESIAN_POINT('Ctrl Pts',(-14.3388048877782,-17.0311085657265,
1.74870406333214));
#17287=CARTESIAN_POINT('Ctrl Pts',(-14.768468555141,-17.27551976469,1.76749949934977));
#17288=CARTESIAN_POINT('Ctrl Pts',(-14.9997221812654,-17.3539974482555,
1.77761558098252));
#17289=CARTESIAN_POINT('Ctrl Pts',(-15.4884672042666,-17.4214811002394,
1.79899550324855));
#17290=CARTESIAN_POINT('Ctrl Pts',(-15.7418621364513,-17.4062346806301,
1.8100801459513));
#17291=CARTESIAN_POINT('Ctrl Pts',(-16.2240935842588,-17.2792838313506,
1.83117513491927));
#17292=CARTESIAN_POINT('Ctrl Pts',(-16.4486458433526,-17.1703969211375,
1.84030125781118));
#17293=CARTESIAN_POINT('Ctrl Pts',(-16.8416862876065,-16.8743501327491,
1.8601133427447));
#17294=CARTESIAN_POINT('Ctrl Pts',(-17.0070079317082,-16.6907437705779,
1.87068502235921));
#17295=CARTESIAN_POINT('Ctrl Pts',(-17.2641149130594,-16.2627020426674,
1.89252441435073));
#17296=CARTESIAN_POINT('Ctrl Pts',(-17.3501358504591,-16.0204129092833,
1.90358473864083));
#17297=CARTESIAN_POINT('Ctrl Pts',(-17.3986777732664,-15.6792907617315,
1.91756948960221));
#17298=CARTESIAN_POINT('Ctrl Pts',(-17.405,-15.589609821744,1.92110523263075));
#17299=CARTESIAN_POINT('Ctrl Pts',(-17.405,-15.5,1.92449999999991));
#17300=CARTESIAN_POINT('Ctrl Pts',(-17.405,-15.5000000000001,1.98699999999985));
#17301=CARTESIAN_POINT('Ctrl Pts',(-17.405,-15.5576762506347,1.98481500007663));
#17302=CARTESIAN_POINT('Ctrl Pts',(-17.4023807755921,-15.6154139218634,
1.98257038493044));
#17303=CARTESIAN_POINT('Ctrl Pts',(-17.3741939527039,-15.9244464994239,
1.97024652341651));
#17304=CARTESIAN_POINT('Ctrl Pts',(-17.3015165680925,-16.1687866178387,
1.95940035359952));
#17305=CARTESIAN_POINT('Ctrl Pts',(-17.0681604473867,-16.6092508752271,
1.93760983318351));
#17306=CARTESIAN_POINT('Ctrl Pts',(-16.9119269620305,-16.8023209402444,
1.92687841044976));
#17307=CARTESIAN_POINT('Ctrl Pts',(-16.5360369434423,-17.1171954523915,
1.90672817703692));
#17308=CARTESIAN_POINT('Ctrl Pts',(-16.3203758924028,-17.2365708955179,
1.89788695942264));
#17309=CARTESIAN_POINT('Ctrl Pts',(-15.8475577563769,-17.3900120669935,
1.87720375137252));
#17310=CARTESIAN_POINT('Ctrl Pts',(-15.5939493045371,-17.4194023058029,
1.86610976835241));
#17311=CARTESIAN_POINT('Ctrl Pts',(-15.0996125733408,-17.3782663055323,
1.8444852394287));
#17312=CARTESIAN_POINT('Ctrl Pts',(-14.8632730729469,-17.311848309036,1.83414667860658));
#17313=CARTESIAN_POINT('Ctrl Pts',(-14.4203422351862,-17.0896519219109,
1.81477087642983));
#17314=CARTESIAN_POINT('Ctrl Pts',(-14.219554067097,-16.9328779450836,1.80494338296207));
#17315=CARTESIAN_POINT('Ctrl Pts',(-13.8924269064666,-16.5521679595822,
1.78336560084335));
#17316=CARTESIAN_POINT('Ctrl Pts',(-13.7685238999814,-16.3326704187886,
1.77234014372881));
#17317=CARTESIAN_POINT('Ctrl Pts',(-13.615111347141,-15.8665290015337,1.75132541995281));
#17318=CARTESIAN_POINT('Ctrl Pts',(-13.5839053729158,-15.6253250129745,
1.74199046187692));
#17319=CARTESIAN_POINT('Ctrl Pts',(-13.6137650496087,-15.132767229072,1.72267736511237));
#17320=CARTESIAN_POINT('Ctrl Pts',(-13.6789651478017,-14.886362035283,1.71191650743335));
#17321=CARTESIAN_POINT('Ctrl Pts',(-13.899100443672,-14.43837788376,1.69013027367801));
#17322=CARTESIAN_POINT('Ctrl Pts',(-14.0499413576698,-14.2401343662606,
1.67932080826729));
#17323=CARTESIAN_POINT('Ctrl Pts',(-14.4160367346151,-13.9147211425423,
1.65898555861985));
#17324=CARTESIAN_POINT('Ctrl Pts',(-14.6268766935179,-13.7895204893169,
1.65019437036221));
#17325=CARTESIAN_POINT('Ctrl Pts',(-15.0942338092302,-13.6215167249473,
1.62975005208956));
#17326=CARTESIAN_POINT('Ctrl Pts',(-15.3476308678393,-13.5842452796376,
1.61866531636737));
#17327=CARTESIAN_POINT('Ctrl Pts',(-15.8444702391433,-13.6105884798816,
1.59693131062353));
#17328=CARTESIAN_POINT('Ctrl Pts',(-16.08336246302,-13.6701795096518,1.5864810821075));
#17329=CARTESIAN_POINT('Ctrl Pts',(-16.5309276996222,-13.8787046238777,
1.56690255032262));
#17330=CARTESIAN_POINT('Ctrl Pts',(-16.7343891762498,-14.0276855562089,
1.55744475601725));
#17331=CARTESIAN_POINT('Ctrl Pts',(-17.0726975821131,-14.3962002472928,
1.53608441974962));
#17332=CARTESIAN_POINT('Ctrl Pts',(-17.2040353110832,-14.6122988907963,
1.52502511181075));
#17333=CARTESIAN_POINT('Ctrl Pts',(-17.3660722950728,-15.0568360880483,
1.50464020377303));
#17334=CARTESIAN_POINT('Ctrl Pts',(-17.405,-15.2776473825378,1.49542357897272));
#17335=CARTESIAN_POINT('Ctrl Pts',(-17.405,-15.5,1.48699999999984));
#17336=CARTESIAN_POINT('Origin',(15.5,-15.5,-1.713));
#17337=CARTESIAN_POINT('',(13.595,-15.5,10.5495));
#17338=CARTESIAN_POINT('',(13.595,-15.5,10.612));
#17339=CARTESIAN_POINT('',(13.595,-15.5,-1.713));
#17340=CARTESIAN_POINT('',(16.8346987578547,-14.140733938563,10.7369999999983));
#17341=CARTESIAN_POINT('Ctrl Pts',(13.595,-15.5,10.5495));
#17342=CARTESIAN_POINT('Ctrl Pts',(13.595,-15.2823467000937,10.5590211417282));
#17343=CARTESIAN_POINT('Ctrl Pts',(13.6323041951647,-15.0660657837748,10.5684822491787));
#17344=CARTESIAN_POINT('Ctrl Pts',(13.7873649268709,-14.6308616850732,10.587520048772));
#17345=CARTESIAN_POINT('Ctrl Pts',(13.9125858088488,-14.4189647250675,10.5963406221173));
#17346=CARTESIAN_POINT('Ctrl Pts',(14.2422054289987,-14.0470719665195,10.6169620282376));
#17347=CARTESIAN_POINT('Ctrl Pts',(14.4460836501414,-13.8930475031147,10.6280545895014));
#17348=CARTESIAN_POINT('Ctrl Pts',(14.8934335791397,-13.6778143228103,10.6497095760738));
#17349=CARTESIAN_POINT('Ctrl Pts',(15.1310246903917,-13.6152821794268,10.6600781679263));
#17350=CARTESIAN_POINT('Ctrl Pts',(15.6249820475859,-13.5825299192131,10.6795075533079));
#17351=CARTESIAN_POINT('Ctrl Pts',(15.8768366076506,-13.6157681297062,10.6892302773471));
#17352=CARTESIAN_POINT('Ctrl Pts',(16.2498388977282,-13.742994250647,10.7061437733815));
#17353=CARTESIAN_POINT('Ctrl Pts',(16.3791092039297,-13.8039772459343,10.7123748699156));
#17354=CARTESIAN_POINT('Ctrl Pts',(16.6212238560751,-13.9533744742352,10.7248147672707));
#17355=CARTESIAN_POINT('Ctrl Pts',(16.733361069962,-14.0412278227297,10.7309845113732));
#17356=CARTESIAN_POINT('Ctrl Pts',(16.8346987578564,-14.1407339385622,10.7369999999993));
#17357=CARTESIAN_POINT('',(15.5,-13.595,10.737));
#17358=CARTESIAN_POINT('Origin',(15.5,-15.5,10.737));
#17359=CARTESIAN_POINT('Ctrl Pts',(15.5000000000012,-13.595,10.7370000000001));
#17360=CARTESIAN_POINT('Ctrl Pts',(15.2556996093285,-13.5949999999998,10.7277449543099));
#17361=CARTESIAN_POINT('Ctrl Pts',(15.0136080866584,-13.6419929658385,10.7175457464537));
#17362=CARTESIAN_POINT('Ctrl Pts',(14.554139443356,-13.8274550958886,10.6960828163414));
#17363=CARTESIAN_POINT('Ctrl Pts',(14.3421784047168,-13.9665356718971,10.6850109033022));
#17364=CARTESIAN_POINT('Ctrl Pts',(13.9869783327278,-14.3163501723868,10.6639033120506));
#17365=CARTESIAN_POINT('Ctrl Pts',(13.8461983203702,-14.5226600964613,10.6547532766204));
#17366=CARTESIAN_POINT('Ctrl Pts',(13.6524557631648,-14.9751135388291,10.6349609125623));
#17367=CARTESIAN_POINT('Ctrl Pts',(13.6003769945158,-15.2165551523544,10.6243991621894));
#17368=CARTESIAN_POINT('Ctrl Pts',(13.595131497578,-15.4741482639885,10.6131308720917));
#17369=CARTESIAN_POINT('Ctrl Pts',(13.595,-15.487077060846,10.6125653079245));
#17370=CARTESIAN_POINT('Ctrl Pts',(13.595,-15.5,10.612));
#17371=CARTESIAN_POINT('Origin',(15.5,-15.5,-1.713));
#17372=CARTESIAN_POINT('',(13.595,-15.5,10.0495));
#17373=CARTESIAN_POINT('',(13.595,-15.5,10.112));
#17374=CARTESIAN_POINT('',(13.595,-15.5,-1.713));
#17375=CARTESIAN_POINT('Ctrl Pts',(13.595,-15.5,10.0495));
#17376=CARTESIAN_POINT('Ctrl Pts',(13.595,-15.4885854639047,10.0499993235387));
#17377=CARTESIAN_POINT('Ctrl Pts',(13.5951025916268,-15.4771662931107,10.05049884982));
#17378=CARTESIAN_POINT('Ctrl Pts',(13.5997094823034,-15.2210165043723,10.0617040024332));
#17379=CARTESIAN_POINT('Ctrl Pts',(13.6512365443426,-14.9793981148592,10.072273485789));
#17380=CARTESIAN_POINT('Ctrl Pts',(13.8439031047659,-14.5265938173909,10.0920811978392));
#17381=CARTESIAN_POINT('Ctrl Pts',(13.9840951254248,-14.3200776670448,10.1012125562281));
#17382=CARTESIAN_POINT('Ctrl Pts',(14.3385164397248,-13.9692567662194,10.1223126573759));
#17383=CARTESIAN_POINT('Ctrl Pts',(14.5504233063801,-13.8295157144395,10.1333969642722));
#17384=CARTESIAN_POINT('Ctrl Pts',(15.0075282912686,-13.643915876073,10.1547733618354));
#17385=CARTESIAN_POINT('Ctrl Pts',(15.2470549408166,-13.5964192294268,10.164886418997));
#17386=CARTESIAN_POINT('Ctrl Pts',(15.7413437873917,-13.5935846520099,10.1836739949659));
#17387=CARTESIAN_POINT('Ctrl Pts',(15.9914666160098,-13.6422633525157,10.1941524169219));
#17388=CARTESIAN_POINT('Ctrl Pts',(16.454548301879,-13.8328030202801,10.2158632803459));
#17389=CARTESIAN_POINT('Ctrl Pts',(16.6635495836274,-13.9713189092327,10.2268107153369));
#17390=CARTESIAN_POINT('Ctrl Pts',(17.0116345047798,-14.315834058712,10.2475328482822));
#17391=CARTESIAN_POINT('Ctrl Pts',(17.14934504374,-14.5166690611182,10.2564846483428));
#17392=CARTESIAN_POINT('Ctrl Pts',(17.3469105138776,-14.9692567735138,10.2762828859804));
#17393=CARTESIAN_POINT('Ctrl Pts',(17.4009094163838,-15.2184123682085,10.287182080849));
#17394=CARTESIAN_POINT('Ctrl Pts',(17.4085380460922,-15.716338685697,10.3089636345449));
#17395=CARTESIAN_POINT('Ctrl Pts',(17.3647938906909,-15.9603021616113,10.3196357026077));
#17396=CARTESIAN_POINT('Ctrl Pts',(17.1871822359435,-16.4179451539634,10.3396550811008));
#17397=CARTESIAN_POINT('Ctrl Pts',(17.055093772971,-16.6273392867399,10.3485778184913));
#17398=CARTESIAN_POINT('Ctrl Pts',(16.713976725445,-16.9896048648143,10.3694242234719));
#17399=CARTESIAN_POINT('Ctrl Pts',(16.5062763678168,-17.1370893814211,10.3805185386244));
#17400=CARTESIAN_POINT('Ctrl Pts',(16.0541901813914,-17.3387032194885,10.4020550671098));
#17401=CARTESIAN_POINT('Ctrl Pts',(15.8155896670134,-17.3943024572225,10.4123102607089));
#17402=CARTESIAN_POINT('Ctrl Pts',(15.3189724577376,-17.413337548513,10.4315403860297));
#17403=CARTESIAN_POINT('Ctrl Pts',(15.0655514661997,-17.3721441088755,10.4416772271422));
#17404=CARTESIAN_POINT('Ctrl Pts',(14.5946111909685,-17.1945017469419,10.4634037110872));
#17405=CARTESIAN_POINT('Ctrl Pts',(14.3810461747161,-17.0617330829786,10.4743983331963));
#17406=CARTESIAN_POINT('Ctrl Pts',(14.0229544734009,-16.7269854446001,10.4952859241593));
#17407=CARTESIAN_POINT('Ctrl Pts',(13.8796963628073,-16.5304158725953,10.5044249399564));
#17408=CARTESIAN_POINT('Ctrl Pts',(13.6692420751003,-16.0840200856592,10.523952314713));
#17409=CARTESIAN_POINT('Ctrl Pts',(13.608054017622,-15.8365612745352,10.5347772845785));
#17410=CARTESIAN_POINT('Ctrl Pts',(13.5956225641649,-15.5562603941975,10.5470389153894));
#17411=CARTESIAN_POINT('Ctrl Pts',(13.595,-15.5281187444259,10.5482699586865));
#17412=CARTESIAN_POINT('Ctrl Pts',(13.595,-15.5,10.5495));
#17413=CARTESIAN_POINT('Ctrl Pts',(13.595,-15.5,10.612));
#17414=CARTESIAN_POINT('Ctrl Pts',(13.595,-15.7412909591996,10.60144483993));
#17415=CARTESIAN_POINT('Ctrl Pts',(13.6408457688845,-15.9805397719341,10.5909790126015));
#17416=CARTESIAN_POINT('Ctrl Pts',(13.8197845796609,-16.4297661061609,10.5713278168785));
#17417=CARTESIAN_POINT('Ctrl Pts',(13.9513442543879,-16.6354551426844,10.5625007719194));
#17418=CARTESIAN_POINT('Ctrl Pts',(14.2882893247519,-16.9906652611646,10.5419667364927));
#17419=CARTESIAN_POINT('Ctrl Pts',(14.4920727561511,-17.1353594156637,10.5310818412297));
#17420=CARTESIAN_POINT('Ctrl Pts',(14.9478948820757,-17.3406183841806,10.5093240536131));
#17421=CARTESIAN_POINT('Ctrl Pts',(15.1963067151894,-17.3974961759311,10.4986692043588));
#17422=CARTESIAN_POINT('Ctrl Pts',(15.6898143706627,-17.4108176576472,10.4796818505767));
#17423=CARTESIAN_POINT('Ctrl Pts',(15.9301253696938,-17.3714395343302,10.4699711404288));
#17424=CARTESIAN_POINT('Ctrl Pts',(16.3918716927025,-17.2018652329606,10.4487694257956));
#17425=CARTESIAN_POINT('Ctrl Pts',(16.6077003531134,-17.0699625826955,10.4377079897539));
#17426=CARTESIAN_POINT('Ctrl Pts',(16.9752781837248,-16.7308092166127,10.4163646641975));
#17427=CARTESIAN_POINT('Ctrl Pts',(17.1236678774154,-16.5271438579512,10.4069319272946));
#17428=CARTESIAN_POINT('Ctrl Pts',(17.3311410686046,-16.0792265773098,10.387337995508));
#17429=CARTESIAN_POINT('Ctrl Pts',(17.3902018446824,-15.840145597041,10.376879509932));
#17430=CARTESIAN_POINT('Ctrl Pts',(17.4153996480397,-15.343131166637,10.3551378463097));
#17431=CARTESIAN_POINT('Ctrl Pts',(17.3775197193691,-15.0897602206549,10.3440542528722));
#17432=CARTESIAN_POINT('Ctrl Pts',(17.2083963180158,-14.622830943006,10.3236286501754));
#17433=CARTESIAN_POINT('Ctrl Pts',(17.0827455582927,-14.4123598146853,10.3148380476183));
#17434=CARTESIAN_POINT('Ctrl Pts',(16.7565163753647,-14.0470286545255,10.2944886014262));
#17435=CARTESIAN_POINT('Ctrl Pts',(16.5578765661879,-13.8966142348298,10.2836734513476));
#17436=CARTESIAN_POINT('Ctrl Pts',(16.1093241222814,-13.6775176070575,10.261888406499));
#17437=CARTESIAN_POINT('Ctrl Pts',(15.8627681320143,-13.6129016625927,10.2511346128306));
#17438=CARTESIAN_POINT('Ctrl Pts',(15.3701374357996,-13.5842067572065,10.2318442300529));
#17439=CARTESIAN_POINT('Ctrl Pts',(15.1289999089402,-13.615985222063,10.2224860842217));
#17440=CARTESIAN_POINT('Ctrl Pts',(14.6631596610225,-13.7705267597449,10.2014580764508));
#17441=CARTESIAN_POINT('Ctrl Pts',(14.4439092045079,-13.8949918882011,10.1904296849652));
#17442=CARTESIAN_POINT('Ctrl Pts',(14.0641127575733,-14.2229686951434,10.1688679275381));
#17443=CARTESIAN_POINT('Ctrl Pts',(13.9079289550465,-14.4239586314856,10.1590709260069));
#17444=CARTESIAN_POINT('Ctrl Pts',(13.6867555065337,-14.8672400535419,10.1396797876843));
#17445=CARTESIAN_POINT('Ctrl Pts',(13.6208440607317,-15.1037768687542,10.1293325954178));
#17446=CARTESIAN_POINT('Ctrl Pts',(13.597065752003,-15.3974989140194,10.1164838620291));
#17447=CARTESIAN_POINT('Ctrl Pts',(13.595,-15.4487792632927,10.1142406271526));
#17448=CARTESIAN_POINT('Ctrl Pts',(13.595,-15.5,10.112));
#17449=CARTESIAN_POINT('Origin',(15.5,-15.5,-1.713));
#17450=CARTESIAN_POINT('',(13.595,-15.5,9.54949999999996));
#17451=CARTESIAN_POINT('',(13.595,-15.5,9.612));
#17452=CARTESIAN_POINT('',(13.595,-15.5,-1.713));
#17453=CARTESIAN_POINT('Ctrl Pts',(13.595,-15.5,9.54949999999995));
#17454=CARTESIAN_POINT('Ctrl Pts',(13.595,-15.4502744854574,9.55167521935877));
#17455=CARTESIAN_POINT('Ctrl Pts',(13.5969469079297,-15.4004916147963,9.553852947734));
#17456=CARTESIAN_POINT('Ctrl Pts',(13.6199184623743,-15.1081582486334,9.56664093400535));
#17457=CARTESIAN_POINT('Ctrl Pts',(13.6852966251491,-14.8714150898636,9.5769971526742));
#17458=CARTESIAN_POINT('Ctrl Pts',(13.9053946919737,-14.4277657801821,9.59640438406885));
#17459=CARTESIAN_POINT('Ctrl Pts',(14.0609593043538,-14.2265640689728,9.60616982353457));
#17460=CARTESIAN_POINT('Ctrl Pts',(14.439795526841,-13.8976963553052,9.62771469008669));
#17461=CARTESIAN_POINT('Ctrl Pts',(14.65878494751,-13.7726412812994,9.63874609596868));
#17462=CARTESIAN_POINT('Ctrl Pts',(15.1243079177073,-13.6169138584148,9.65978802202635));
#17463=CARTESIAN_POINT('Ctrl Pts',(15.3653763046083,-13.5845343459454,9.6691710250572));
#17464=CARTESIAN_POINT('Ctrl Pts',(15.8580824961113,-13.6120073228381,9.68843754154408));
#17465=CARTESIAN_POINT('Ctrl Pts',(16.1047951463693,-13.676010096271,9.69918385866022));
#17466=CARTESIAN_POINT('Ctrl Pts',(16.5539411468359,-13.894015560723,9.72096752351754));
#17467=CARTESIAN_POINT('Ctrl Pts',(16.7529957164446,-14.0439814927899,9.73178857688824));
#17468=CARTESIAN_POINT('Ctrl Pts',(17.0800802835538,-14.4085105467076,9.75215288446747));
#17469=CARTESIAN_POINT('Ctrl Pts',(17.2062028388546,-14.6185957461662,9.76094338347164));
#17470=CARTESIAN_POINT('Ctrl Pts',(17.3764987911599,-15.0850757309887,9.78134933206405));
#17471=CARTESIAN_POINT('Ctrl Pts',(17.4150163189817,-15.3384178102987,9.79243166274253));
#17472=CARTESIAN_POINT('Ctrl Pts',(17.3910192245,-15.8356128863494,9.81418122862402));
#17473=CARTESIAN_POINT('Ctrl Pts',(17.3325145603624,-16.074890375008,9.82464831036762));
#17474=CARTESIAN_POINT('Ctrl Pts',(17.1261431374813,-16.5231756890091,9.84425834160127));
#17475=CARTESIAN_POINT('Ctrl Pts',(16.9783714265357,-16.7270543597511,9.85366535294237));
#17476=CARTESIAN_POINT('Ctrl Pts',(16.6117745768507,-17.0670904080252,9.8749908213987));
#17477=CARTESIAN_POINT('Ctrl Pts',(16.3962299527202,-17.1995836267748,9.88605441411614));
#17478=CARTESIAN_POINT('Ctrl Pts',(15.9348178116792,-17.3703597238175,9.90726975463571));
#17479=CARTESIAN_POINT('Ctrl Pts',(15.6945683061102,-17.4103438385966,9.91701211657193));
#17480=CARTESIAN_POINT('Ctrl Pts',(15.2009978140301,-17.3982405944492,9.93597520523219));
#17481=CARTESIAN_POINT('Ctrl Pts',(14.9524496570676,-17.3419779720927,9.94662176381363));
#17482=CARTESIAN_POINT('Ctrl Pts',(14.4960700533142,-17.1378253197796,9.96837647320892));
#17483=CARTESIAN_POINT('Ctrl Pts',(14.2918860957013,-16.9935915259762,9.97926647282571));
#17484=CARTESIAN_POINT('Ctrl Pts',(13.9540961430899,-16.6391862209806,9.9998149125721));
#17485=CARTESIAN_POINT('Ctrl Pts',(13.8220704882375,-16.4338694301794,10.0086483188896));
#17486=CARTESIAN_POINT('Ctrl Pts',(13.6414552862163,-15.9836817917745,10.0283415664139));
#17487=CARTESIAN_POINT('Ctrl Pts',(13.595,-15.7428901843941,10.0388748825724));
#17488=CARTESIAN_POINT('Ctrl Pts',(13.595,-15.5,10.0495));
#17489=CARTESIAN_POINT('Ctrl Pts',(13.595,-15.5,10.112));
#17490=CARTESIAN_POINT('Ctrl Pts',(13.595,-15.7008367103392,10.1032144921112));
#17491=CARTESIAN_POINT('Ctrl Pts',(13.6267629324258,-15.900756920881,10.0944690760771));
#17492=CARTESIAN_POINT('Ctrl Pts',(13.7653182344057,-16.3243321971831,10.0759399738766));
#17493=CARTESIAN_POINT('Ctrl Pts',(13.8851281171556,-16.5396306949641,10.0671051936536));
#17494=CARTESIAN_POINT('Ctrl Pts',(14.200786992495,-16.9147965477635,10.0469410846696));
#17495=CARTESIAN_POINT('Ctrl Pts',(14.3942454641661,-17.0706361452585,10.0362035628064));
#17496=CARTESIAN_POINT('Ctrl Pts',(14.835280621152,-17.3030209097119,10.0144126602632));
#17497=CARTESIAN_POINT('Ctrl Pts',(15.0797818291005,-17.3751462450849,10.0035724623181));
#17498=CARTESIAN_POINT('Ctrl Pts',(15.5713993833167,-17.418869326979,9.98399176101256));
#17499=CARTESIAN_POINT('Ctrl Pts',(15.8134360435395,-17.3944470517877,9.97489501092434));
#17500=CARTESIAN_POINT('Ctrl Pts',(16.2830697953039,-17.2543658920727,9.95403957175722));
#17501=CARTESIAN_POINT('Ctrl Pts',(16.5053789616836,-17.137134027351,9.94305351235477));
#17502=CARTESIAN_POINT('Ctrl Pts',(16.8968287771957,-16.8201505199817,9.9212907285304));
#17503=CARTESIAN_POINT('Ctrl Pts',(17.0606228992972,-16.6217591407651,9.91107082855505));
#17504=CARTESIAN_POINT('Ctrl Pts',(17.2948368693994,-16.1829939416919,9.89187725029288));
#17505=CARTESIAN_POINT('Ctrl Pts',(17.3671514122205,-15.949046830156,9.88164334340155));
#17506=CARTESIAN_POINT('Ctrl Pts',(17.4211345562518,-15.4572525691451,9.86013003364604));
#17507=CARTESIAN_POINT('Ctrl Pts',(17.3986235514731,-15.2036525256751,9.84903641844612));
#17508=CARTESIAN_POINT('Ctrl Pts',(17.2580021132843,-14.7261927064949,9.82815016213902));
#17509=CARTESIAN_POINT('Ctrl Pts',(17.1437161358039,-14.5062482392129,9.81920140200463));
#17510=CARTESIAN_POINT('Ctrl Pts',(16.8380073730827,-14.1219539327206,9.79921458188554));
#17511=CARTESIAN_POINT('Ctrl Pts',(16.649512387961,-13.9612078910303,9.78855778107861));
#17512=CARTESIAN_POINT('Ctrl Pts',(16.2158461956214,-13.7166562727637,9.76677992681519));
#17513=CARTESIAN_POINT('Ctrl Pts',(15.9734738382061,-13.6375845413723,9.75586844455832));
#17514=CARTESIAN_POINT('Ctrl Pts',(15.4829480248446,-13.5798368529878,9.73602235270462));
#17515=CARTESIAN_POINT('Ctrl Pts',(15.23999153869,-13.5974435708591,9.7270964252791));
#17516=CARTESIAN_POINT('Ctrl Pts',(14.7669894001789,-13.7242335415259,9.70640408698826));
#17517=CARTESIAN_POINT('Ctrl Pts',(14.5420740146174,-13.8347603326945,9.69546594905376));
#17518=CARTESIAN_POINT('Ctrl Pts',(14.1440292603168,-14.1383602326029,9.67374605320853));
#17519=CARTESIAN_POINT('Ctrl Pts',(13.9758112521117,-14.3297413092978,9.66319241866602));
#17520=CARTESIAN_POINT('Ctrl Pts',(13.7289315632306,-14.7578028599957,9.64446706649201));
#17521=CARTESIAN_POINT('Ctrl Pts',(13.6491027494895,-14.9884388844074,9.63437800155712));
#17522=CARTESIAN_POINT('Ctrl Pts',(13.6015031498374,-15.3181544373058,9.61995474902438));
#17523=CARTESIAN_POINT('Ctrl Pts',(13.595,-15.4091197940947,9.61597551206935));
#17524=CARTESIAN_POINT('Ctrl Pts',(13.595,-15.5,9.612));
#17525=CARTESIAN_POINT('Origin',(15.5,-15.5,-1.713));
#17526=CARTESIAN_POINT('',(13.595,-15.5,9.04949999999995));
#17527=CARTESIAN_POINT('',(13.595,-15.5,9.11199999999999));
#17528=CARTESIAN_POINT('',(13.595,-15.5,-1.713));
#17529=CARTESIAN_POINT('Ctrl Pts',(13.595,-15.5,9.04949999999995));
#17530=CARTESIAN_POINT('Ctrl Pts',(13.595,-15.410571107507,9.05341202504338));
#17531=CARTESIAN_POINT('Ctrl Pts',(13.6012971006541,-15.3210561673908,9.05732781419969));
#17532=CARTESIAN_POINT('Ctrl Pts',(13.6479436729555,-14.9926259880107,9.07169483866952));
#17533=CARTESIAN_POINT('Ctrl Pts',(13.7272713627419,-14.761759744373,9.0817939744367));
#17534=CARTESIAN_POINT('Ctrl Pts',(13.9732357126391,-14.3331017483525,9.10054541783218));
#17535=CARTESIAN_POINT('Ctrl Pts',(14.1410360274765,-14.1413467593241,9.11106733583993));
#17536=CARTESIAN_POINT('Ctrl Pts',(14.5384579830271,-13.8368377733064,9.13278352142774));
#17537=CARTESIAN_POINT('Ctrl Pts',(14.7631831589794,-13.7258021200914,9.14372558345101));
#17538=CARTESIAN_POINT('Ctrl Pts',(15.2359343291776,-13.5980067128105,9.16443040526644));
#17539=CARTESIAN_POINT('Ctrl Pts',(15.4788180628624,-13.5798822975231,9.17336688771192));
#17540=CARTESIAN_POINT('Ctrl Pts',(15.9694321495217,-13.6365619282601,9.19319296285935));
#17541=CARTESIAN_POINT('Ctrl Pts',(16.2119737247838,-13.7151069957101,9.20409933641036));
#17542=CARTESIAN_POINT('Ctrl Pts',(16.6462128309944,-13.9587404009295,9.22587881147182));
#17543=CARTESIAN_POINT('Ctrl Pts',(16.8350899823954,-14.119118253725,9.23654203709323));
#17544=CARTESIAN_POINT('Ctrl Pts',(17.1415594948502,-14.5027190331107,9.2565425083515));
#17545=CARTESIAN_POINT('Ctrl Pts',(17.2562689319036,-14.72230470962,9.26548008353523));
#17546=CARTESIAN_POINT('Ctrl Pts',(17.3979598892063,-15.1993833986608,9.28634966748277));
#17547=CARTESIAN_POINT('Ctrl Pts',(17.4210424631524,-15.4529910108418,9.29744361377241));
#17548=CARTESIAN_POINT('Ctrl Pts',(17.3681244205606,-15.9450092692229,9.31896672218804));
#17549=CARTESIAN_POINT('Ctrl Pts',(17.2962975705816,-16.17916100399,9.32920958022685));
#17550=CARTESIAN_POINT('Ctrl Pts',(17.0630855458631,-16.6182768382877,9.34841849686281));
#17551=CARTESIAN_POINT('Ctrl Pts',(16.8998828532734,-16.8168700849708,9.35860327774385));
#17552=CARTESIAN_POINT('Ctrl Pts',(16.5093288066214,-17.1347108439304,9.38035087640664));
#17553=CARTESIAN_POINT('Ctrl Pts',(16.2872475205707,-17.2525035314174,9.39134056928365));
#17554=CARTESIAN_POINT('Ctrl Pts',(15.8179017431069,-17.3937009619574,9.41220951424044));
#17555=CARTESIAN_POINT('Ctrl Pts',(15.5759382291941,-17.4186930865504,9.42132366671565));
#17556=CARTESIAN_POINT('Ctrl Pts',(15.0842361807923,-17.3761386070571,9.44088200900592));
#17557=CARTESIAN_POINT('Ctrl Pts',(14.8395667426201,-17.3045949272268,9.45171585803926));
#17558=CARTESIAN_POINT('Ctrl Pts',(14.3979327965919,-17.0732344339334,9.47350704190107));
#17559=CARTESIAN_POINT('Ctrl Pts',(14.20406620879,-16.9178105839672,9.48425093144459));
#17560=CARTESIAN_POINT('Ctrl Pts',(13.8875820471894,-16.5434075363857,9.50442962119228));
#17561=CARTESIAN_POINT('Ctrl Pts',(13.7673152099352,-16.3284898256387,9.51325810036557));
#17562=CARTESIAN_POINT('Ctrl Pts',(13.6272628027254,-15.9038712930308,9.53183283932479));
#17563=CARTESIAN_POINT('Ctrl Pts',(13.595,-15.7024108270756,9.54064563311126));
#17564=CARTESIAN_POINT('Ctrl Pts',(13.595,-15.5,9.54949999999996));
#17565=CARTESIAN_POINT('Ctrl Pts',(13.595,-15.5,9.612));
#17566=CARTESIAN_POINT('Ctrl Pts',(13.595,-15.6592363994984,9.60503427823716));
#17567=CARTESIAN_POINT('Ctrl Pts',(13.6149664418887,-15.8182113811384,9.59807999207632));
#17568=CARTESIAN_POINT('Ctrl Pts',(13.7162061731805,-16.213048823518,9.58080801296959));
#17569=CARTESIAN_POINT('Ctrl Pts',(13.82389619804,-16.438630035475,9.57163400936754));
#17570=CARTESIAN_POINT('Ctrl Pts',(14.1178117380362,-16.8335843974178,9.55186080266696));
#17571=CARTESIAN_POINT('Ctrl Pts',(14.3003316472966,-16.9998901349052,9.54130875774747));
#17572=CARTESIAN_POINT('Ctrl Pts',(14.7265604220024,-17.2594103896354,9.51948526369304));
#17573=CARTESIAN_POINT('Ctrl Pts',(14.9681598682303,-17.3468610247554,9.50841979669683));
#17574=CARTESIAN_POINT('Ctrl Pts',(15.4592480622578,-17.419886963939,9.48821822971879));
#17575=CARTESIAN_POINT('Ctrl Pts',(15.7032719165713,-17.4095316129779,9.47939838857678));
#17576=CARTESIAN_POINT('Ctrl Pts',(16.179705827867,-17.2967441184858,9.45888230731463));
#17577=CARTESIAN_POINT('Ctrl Pts',(16.4071510785082,-17.1933275469165,9.44800384489947));
#17578=CARTESIAN_POINT('Ctrl Pts',(16.8136626439144,-16.9024937973762,9.42624241806902));
#17579=CARTESIAN_POINT('Ctrl Pts',(16.9877023586233,-16.7163326475971,9.41557735292926));
#17580=CARTESIAN_POINT('Ctrl Pts',(17.2472648561672,-16.2964293272925,9.39655988237394));
#17581=CARTESIAN_POINT('Ctrl Pts',(17.3340082850086,-16.0689342103612,9.38688776073332));
#17582=CARTESIAN_POINT('Ctrl Pts',(17.4195245794063,-15.584650961036,9.36570301666835));
#17583=CARTESIAN_POINT('Ctrl Pts',(17.4140187813701,-15.3318500259603,9.35464435809111));
#17584=CARTESIAN_POINT('Ctrl Pts',(17.3056516691084,-14.8434366460597,9.33327894339729));
#17585=CARTESIAN_POINT('Ctrl Pts',(17.2040806530936,-14.612561851177,9.32381356348501));
#17586=CARTESIAN_POINT('Ctrl Pts',(16.9209888558443,-14.207971510667,9.30423964142568));
#17587=CARTESIAN_POINT('Ctrl Pts',(16.7440258956182,-14.036809199301,9.2937918909984));
#17588=CARTESIAN_POINT('Ctrl Pts',(16.3271388577635,-13.7653056439892,9.27206019620634));
#17589=CARTESIAN_POINT('Ctrl Pts',(16.0891392566732,-13.6707238628737,9.26097513097483));
#17590=CARTESIAN_POINT('Ctrl Pts',(15.6004510343452,-13.5821870637115,9.24052522657206));
#17591=CARTESIAN_POINT('Ctrl Pts',(15.3552296432451,-13.5850223738718,9.23173377105869));
#17592=CARTESIAN_POINT('Ctrl Pts',(14.8753994325026,-13.6834655640153,9.2114027672495));
#17593=CARTESIAN_POINT('Ctrl Pts',(14.6455947298484,-13.779562778925,9.20059501056258));
#17594=CARTESIAN_POINT('Ctrl Pts',(14.2307765791858,-14.0571584130691,9.17880844566771));
#17595=CARTESIAN_POINT('Ctrl Pts',(14.0509806590752,-14.2378250741837,9.1680454900741));
#17596=CARTESIAN_POINT('Ctrl Pts',(13.7785522306151,-14.6492698322716,9.1487256161107));
#17597=CARTESIAN_POINT('Ctrl Pts',(13.6848174176791,-14.8736934308153,9.13939748771596));
#17598=CARTESIAN_POINT('Ctrl Pts',(13.6084807912089,-15.2383437374753,9.12344603073171));
#17599=CARTESIAN_POINT('Ctrl Pts',(13.595,-15.3691547988651,9.11772376207938));
#17600=CARTESIAN_POINT('Ctrl Pts',(13.595,-15.5,9.11199999999999));
#17601=CARTESIAN_POINT('Origin',(15.5,-15.5,-1.713));
#17602=CARTESIAN_POINT('',(13.595,-15.5,8.54949999999994));
#17603=CARTESIAN_POINT('',(13.595,-15.5,8.61199999999998));
#17604=CARTESIAN_POINT('',(13.595,-15.5,-1.713));
#17605=CARTESIAN_POINT('Ctrl Pts',(13.595,-15.5,8.54949999999994));
#17606=CARTESIAN_POINT('Ctrl Pts',(13.595,-15.3706312184885,8.55515917679397));
#17607=CARTESIAN_POINT('Ctrl Pts',(13.6081782572954,-15.2412882250917,8.56081722549889));
#17608=CARTESIAN_POINT('Ctrl Pts',(13.6833684033628,-14.8779059502326,8.57671321302554));
#17609=CARTESIAN_POINT('Ctrl Pts',(13.77658581932,-14.6532588833752,8.58606387124224));
#17610=CARTESIAN_POINT('Ctrl Pts',(14.0480634340968,-14.2411825017125,8.60536153973686));
#17611=CARTESIAN_POINT('Ctrl Pts',(14.2274385998401,-14.0601021103429,8.6161176047424));
#17612=CARTESIAN_POINT('Ctrl Pts',(14.6416556152634,-13.7815167346891,8.63790304419398));
#17613=CARTESIAN_POINT('Ctrl Pts',(14.8712932594593,-13.6848751833049,8.64871637793111));
#17614=CARTESIAN_POINT('Ctrl Pts',(15.3508753640126,-13.5853670120839,8.66906127606558));
#17615=CARTESIAN_POINT('Ctrl Pts',(15.5960042721982,-13.5819698294477,8.67785201458072));
#17616=CARTESIAN_POINT('Ctrl Pts',(16.0848780449043,-13.6693485876092,8.69828361937024));
#17617=CARTESIAN_POINT('Ctrl Pts',(16.3231535648926,-13.7634022146335,8.70936758555232));
#17618=CARTESIAN_POINT('Ctrl Pts',(16.7407498898442,-14.034021388476,8.73110680746206));
#17619=CARTESIAN_POINT('Ctrl Pts',(16.9181324415661,-14.2048270363753,8.74156265260331));
#17620=CARTESIAN_POINT('Ctrl Pts',(17.2020374331519,-14.6086982647906,8.76115165300497));
#17621=CARTESIAN_POINT('Ctrl Pts',(17.3040707483591,-14.8391714882777,8.77059236606621));
#17622=CARTESIAN_POINT('Ctrl Pts',(17.4136129180806,-15.3272046045457,8.7919411463054));
#17623=CARTESIAN_POINT('Ctrl Pts',(17.4197296533386,-15.5800536124631,8.8030019078066));
#17624=CARTESIAN_POINT('Ctrl Pts',(17.3353425167868,-16.0646292820051,8.82419944365709));
#17625=CARTESIAN_POINT('Ctrl Pts',(17.2491193178985,-16.2923574232655,8.83390056640762));
#17626=CARTESIAN_POINT('Ctrl Pts',(16.9905152523131,-16.7128834009353,8.85289534677308));
#17627=CARTESIAN_POINT('Ctrl Pts',(16.8169095940015,-16.8994448139881,8.86355272283891));
#17628=CARTESIAN_POINT('Ctrl Pts',(16.4110314361869,-17.1912511569425,8.88531142655658));
#17629=CARTESIAN_POINT('Ctrl Pts',(16.1837704005117,-17.2952088423174,8.89619474557987));
#17630=CARTESIAN_POINT('Ctrl Pts',(15.7075929037513,-17.4090592639519,8.91672436149072));
#17631=CARTESIAN_POINT('Ctrl Pts',(15.463653614066,-17.4199679649402,8.92554955866493));
#17632=CARTESIAN_POINT('Ctrl Pts',(14.9723958892026,-17.3480839035569,8.94573257267319));
#17633=CARTESIAN_POINT('Ctrl Pts',(14.7305396939158,-17.2611629600836,8.95679618076234));
#17634=CARTESIAN_POINT('Ctrl Pts',(14.3036369416927,-17.0025363920969,8.97862566074327));
#17635=CARTESIAN_POINT('Ctrl Pts',(14.1207134528123,-16.8365948553763,8.98918502892699));
#17636=CARTESIAN_POINT('Ctrl Pts',(13.8260068563253,-16.4423502430572,9.00897268008097));
#17637=CARTESIAN_POINT('Ctrl Pts',(13.7178723046654,-16.2171514711361,9.01812854456953));
#17638=CARTESIAN_POINT('Ctrl Pts',(13.6153487921593,-15.82122928745,9.03544797517697));
#17639=CARTESIAN_POINT('Ctrl Pts',(13.595,-15.6607536629728,9.04246790625661));
#17640=CARTESIAN_POINT('Ctrl Pts',(13.595,-15.5,9.04949999999995));
#17641=CARTESIAN_POINT('Ctrl Pts',(13.595,-15.5,9.11199999999999));
#17642=CARTESIAN_POINT('Ctrl Pts',(13.595,-15.6176025375141,9.10685553204224));
#17643=CARTESIAN_POINT('Ctrl Pts',(13.6058899738159,-15.7352326539994,9.1017098576554));
#17644=CARTESIAN_POINT('Ctrl Pts',(13.6742308708525,-16.0993980787507,9.08577961160329));
#17645=CARTESIAN_POINT('Ctrl Pts',(13.7695912343068,-16.335684931158,9.0759429345776));
#17646=CARTESIAN_POINT('Ctrl Pts',(14.0418391735161,-16.7497899605815,9.05657171208437));
#17647=CARTESIAN_POINT('Ctrl Pts',(14.213179571274,-16.9255805889196,9.04623573433626));
#17648=CARTESIAN_POINT('Ctrl Pts',(14.6205032004331,-17.2086275779359,9.02461385748055));
#17649=CARTESIAN_POINT('Ctrl Pts',(14.8547437993334,-17.3101319062483,9.01351978602818));
#17650=CARTESIAN_POINT('Ctrl Pts',(15.3408779598977,-17.4139985700453,8.99283134050786));
#17651=CARTESIAN_POINT('Ctrl Pts',(15.5873625676778,-17.4186132169735,8.98398811922745));
#17652=CARTESIAN_POINT('Ctrl Pts',(16.0704000423377,-17.3341792674494,8.96384202566675));
#17653=CARTESIAN_POINT('Ctrl Pts',(16.302280786376,-17.2452513854976,8.95311243004288));
#17654=CARTESIAN_POINT('Ctrl Pts',(16.7247704093841,-16.9807684807294,8.93132204514592));
#17655=CARTESIAN_POINT('Ctrl Pts',(16.9099992050158,-16.8056264225291,8.92047410675442));
#17656=CARTESIAN_POINT('Ctrl Pts',(17.1948681402976,-16.4025463604327,8.90086589302953));
#17657=CARTESIAN_POINT('Ctrl Pts',(17.2953896066004,-16.1809976105482,8.89178992172133));
#17658=CARTESIAN_POINT('Ctrl Pts',(17.4102594727264,-15.7046233105122,8.8709511509411));
#17659=CARTESIAN_POINT('Ctrl Pts',(17.4206259784906,-15.4535861600049,8.85996964829425));
#17660=CARTESIAN_POINT('Ctrl Pts',(17.3433017380162,-14.9556633660658,8.83818824873435));
#17661=CARTESIAN_POINT('Ctrl Pts',(17.2539668478584,-14.714110896276,8.82792455362117));
#17662=CARTESIAN_POINT('Ctrl Pts',(16.9920824638983,-14.2910418118942,8.80874987857501));
#17663=CARTESIAN_POINT('Ctrl Pts',(16.8261540972266,-14.1110498671306,8.79852703723084));
#17664=CARTESIAN_POINT('Ctrl Pts',(16.4281347961935,-13.8174079753212,8.77702590985569));
#17665=CARTESIAN_POINT('Ctrl Pts',(16.1976160092304,-13.7095001629511,8.76593277635856));
#17666=CARTESIAN_POINT('Ctrl Pts',(15.7140661012773,-13.5911788993635,8.74502607749248));
#17667=CARTESIAN_POINT('Ctrl Pts',(15.4663234134166,-13.5795094336733,8.73606301415881));
#17668=CARTESIAN_POINT('Ctrl Pts',(14.9803906031063,-13.6508785509999,8.71609299154619));
#17669=CARTESIAN_POINT('Ctrl Pts',(14.7467775836836,-13.7331143078645,8.70544414255637));
#17670=CARTESIAN_POINT('Ctrl Pts',(14.3175348174729,-13.9852300737107,8.68366841977192));
#17671=CARTESIAN_POINT('Ctrl Pts',(14.1274155894136,-14.1550903952042,8.67275073639511));
#17672=CARTESIAN_POINT('Ctrl Pts',(13.831060640224,-14.5502736758525,8.6528801084485));
#17673=CARTESIAN_POINT('Ctrl Pts',(13.7242349538834,-14.7692436797465,8.64396659318698));
#17674=CARTESIAN_POINT('Ctrl Pts',(13.6171517742805,-15.1649283516214,8.62665755242255));
#17675=CARTESIAN_POINT('Ctrl Pts',(13.595,-15.3322765292482,8.61933698472228));
#17676=CARTESIAN_POINT('Ctrl Pts',(13.595,-15.5,8.61199999999998));
#17677=CARTESIAN_POINT('Origin',(15.5,-15.5,-1.713));
#17678=CARTESIAN_POINT('',(13.595,-15.5,8.04949999999993));
#17679=CARTESIAN_POINT('',(13.595,-15.5,8.11199999999998));
#17680=CARTESIAN_POINT('',(13.595,-15.5,-1.713));
#17681=CARTESIAN_POINT('Ctrl Pts',(13.595,-15.5,8.04949999999993));
#17682=CARTESIAN_POINT('Ctrl Pts',(13.595,-15.3311510627383,8.05688621772792));
#17683=CARTESIAN_POINT('Ctrl Pts',(13.617450090195,-15.162692391182,8.06425536346524));
#17684=CARTESIAN_POINT('Ctrl Pts',(13.7255350044953,-14.7660823182981,8.08160488546367));
#17685=CARTESIAN_POINT('Ctrl Pts',(13.8327659814356,-14.5472751736397,8.09051029742115));
#17686=CARTESIAN_POINT('Ctrl Pts',(14.1298564730975,-14.1526035520423,8.11039759942469));
#17687=CARTESIAN_POINT('Ctrl Pts',(14.3202845677445,-13.9830872969252,8.12131945835369));
#17688=CARTESIAN_POINT('Ctrl Pts',(14.749948695651,-13.7317717547783,8.14309364124675));
#17689=CARTESIAN_POINT('Ctrl Pts',(14.9836665076678,-13.6499667726971,8.15373703816555));
#17690=CARTESIAN_POINT('Ctrl Pts',(15.4697825617727,-13.5794388007601,8.17369560500767));
#17691=CARTESIAN_POINT('Ctrl Pts',(15.7176088369337,-13.5915663013557,8.18266876340979));
#17692=CARTESIAN_POINT('Ctrl Pts',(16.200985293846,-13.7108233055556,8.20358935804573));
#17693=CARTESIAN_POINT('Ctrl Pts',(16.431257343107,-13.8191413162432,8.21468211612908));
#17694=CARTESIAN_POINT('Ctrl Pts',(16.8286650382414,-14.1134590723776,8.23617485618652));
#17695=CARTESIAN_POINT('Ctrl Pts',(16.9942395381288,-14.2937174227158,8.24639011857894));
#17696=CARTESIAN_POINT('Ctrl Pts',(17.2539964803157,-14.7150120255227,8.26544538595191));
#17697=CARTESIAN_POINT('Ctrl Pts',(17.3424675768812,-14.9540462123252,8.2756175071007));
#17698=CARTESIAN_POINT('Ctrl Pts',(17.4205245726411,-15.4492943382567,8.29728190456052));
#17699=CARTESIAN_POINT('Ctrl Pts',(17.4107131831776,-15.7004100784271,8.30826684507541));
#17700=CARTESIAN_POINT('Ctrl Pts',(17.2968718994881,-16.177071234859,8.32911816425442));
#17701=CARTESIAN_POINT('Ctrl Pts',(17.1968422883955,-16.3988248467073,8.33820970670972));
#17702=CARTESIAN_POINT('Ctrl Pts',(16.912872666671,-16.8025159955848,8.35779721680401));
#17703=CARTESIAN_POINT('Ctrl Pts',(16.7280319823578,-16.978064308801,8.36863933775223));
#17704=CARTESIAN_POINT('Ctrl Pts',(16.3060846545402,-17.24350511329,8.39043012984293));
#17705=CARTESIAN_POINT('Ctrl Pts',(16.0743470808187,-17.3329541050855,8.40116569947336));
#17706=CARTESIAN_POINT('Ctrl Pts',(15.5915390081312,-17.418405563219,8.42132535761712));
#17707=CARTESIAN_POINT('Ctrl Pts',(15.3451490992139,-17.4143358562908,8.43016215598123));
#17708=CARTESIAN_POINT('Ctrl Pts',(14.858822116526,-17.3115886025642,8.45083342231618));
#17709=CARTESIAN_POINT('Ctrl Pts',(14.6243004008481,-17.210585306207,8.46192718485752));
#17710=CARTESIAN_POINT('Ctrl Pts',(14.2162676588325,-16.9283707280214,8.48355771894564));
#17711=CARTESIAN_POINT('Ctrl Pts',(14.0445125088107,-16.7529121267539,8.49390214693266));
#17712=CARTESIAN_POINT('Ctrl Pts',(13.7714676912101,-16.3395015877221,8.51328836818941));
#17713=CARTESIAN_POINT('Ctrl Pts',(13.675647834441,-16.1036159659264,8.52309510210279));
#17714=CARTESIAN_POINT('Ctrl Pts',(13.6061757673627,-15.7382931073913,8.53907597955402));
#17715=CARTESIAN_POINT('Ctrl Pts',(13.595,-15.6191356188194,8.54428846811807));
#17716=CARTESIAN_POINT('Ctrl Pts',(13.595,-15.5,8.54949999999994));
#17717=CARTESIAN_POINT('Ctrl Pts',(13.595,-15.5,8.61199999999998));
#17718=CARTESIAN_POINT('Ctrl Pts',(13.595,-15.5794309395666,8.6085253307276));
#17719=CARTESIAN_POINT('Ctrl Pts',(13.5999678000312,-15.6589460501022,8.60504697943564));
#17720=CARTESIAN_POINT('Ctrl Pts',(13.641465784413,-15.9883922555288,8.59063550938198));
#17721=CARTESIAN_POINT('Ctrl Pts',(13.7224139007472,-16.2299939283492,8.58006675729009));
#17722=CARTESIAN_POINT('Ctrl Pts',(13.9685057180156,-16.6584443948786,8.56132439217507));
#17723=CARTESIAN_POINT('Ctrl Pts',(14.1277562475251,-16.8433063610855,8.55127142472815));
#17724=CARTESIAN_POINT('Ctrl Pts',(14.5142748007372,-17.1493795222357,8.52993409022724));
#17725=CARTESIAN_POINT('Ctrl Pts',(14.7400863745338,-17.2648350536812,8.51885419849063));
#17726=CARTESIAN_POINT('Ctrl Pts',(15.2202790765396,-17.4005804876757,8.49769357750874));
#17727=CARTESIAN_POINT('Ctrl Pts',(15.4696163825964,-17.4208116915508,8.48849688671508));
#17728=CARTESIAN_POINT('Ctrl Pts',(15.9588807925257,-17.3650172090941,8.46874130275205));
#17729=CARTESIAN_POINT('Ctrl Pts',(16.1943024582505,-17.2907505462864,8.45819823737484));
#17730=CARTESIAN_POINT('Ctrl Pts',(16.6326967446266,-17.0526412272871,8.43638217226655));
#17731=CARTESIAN_POINT('Ctrl Pts',(16.8296315264493,-16.8877291948126,8.42531451959006));
#17732=CARTESIAN_POINT('Ctrl Pts',(17.1395177580603,-16.4998220609018,8.40509042003568));
#17733=CARTESIAN_POINT('Ctrl Pts',(17.2531967787472,-16.2835605643862,8.39627649013066));
#17734=CARTESIAN_POINT('Ctrl Pts',(17.3950116373512,-15.8149399315971,8.37577689989492));
#17735=CARTESIAN_POINT('Ctrl Pts',(17.4198540512094,-15.5663949154174,8.36490441449773));
#17736=CARTESIAN_POINT('Ctrl Pts',(17.3726494328954,-15.0688566698042,8.34313983682436));
#17737=CARTESIAN_POINT('Ctrl Pts',(17.2991348321892,-14.824841396726,8.33246550291892));
#17738=CARTESIAN_POINT('Ctrl Pts',(17.066507698286,-14.3894725032585,8.31342049445577));
#17739=CARTESIAN_POINT('Ctrl Pts',(16.9134234150931,-14.2001966532814,8.30378297945824));
#17740=CARTESIAN_POINT('Ctrl Pts',(16.5377733451185,-13.8829872164622,8.28261380964455));
#17741=CARTESIAN_POINT('Ctrl Pts',(16.3165112992051,-13.7607430290753,8.27155778836951));
#17742=CARTESIAN_POINT('Ctrl Pts',(15.8396647684048,-13.6089185591677,8.25017224837243));
#17743=CARTESIAN_POINT('Ctrl Pts',(15.5887938715175,-13.5807136919527,8.24067632994134));
#17744=CARTESIAN_POINT('Ctrl Pts',(15.0966010032285,-13.6222926016751,8.22112073141286));
#17745=CARTESIAN_POINT('Ctrl Pts',(14.8597701187552,-13.6893089311827,8.21068286058571));
#17746=CARTESIAN_POINT('Ctrl Pts',(14.4157022868252,-13.9133101184512,8.18896043639108));
#17747=CARTESIAN_POINT('Ctrl Pts',(14.2144065933613,-14.0715222440947,8.17787411762319));
#17748=CARTESIAN_POINT('Ctrl Pts',(13.8922847111168,-14.4495722712142,8.15740208145966));
#17749=CARTESIAN_POINT('Ctrl Pts',(13.7714830508635,-14.6631148846274,8.14860914765412));
#17750=CARTESIAN_POINT('Ctrl Pts',(13.6283784023255,-15.0893069497315,8.12996557525237));
#17751=CARTESIAN_POINT('Ctrl Pts',(13.595,-15.2941185117879,8.12100618933559));
#17752=CARTESIAN_POINT('Ctrl Pts',(13.595,-15.5,8.11199999999998));
#17753=CARTESIAN_POINT('Origin',(15.5,-15.5,-1.713));
#17754=CARTESIAN_POINT('',(13.595,-15.5,7.54949999999993));
#17755=CARTESIAN_POINT('',(13.595,-15.5,7.61199999999997));
#17756=CARTESIAN_POINT('',(13.595,-15.5,-1.713));
#17757=CARTESIAN_POINT('Ctrl Pts',(13.595,-15.5,7.54949999999993));
#17758=CARTESIAN_POINT('Ctrl Pts',(13.595,-15.2929493792634,7.55855733249059));
#17759=CARTESIAN_POINT('Ctrl Pts',(13.6287585544377,-15.0869966833337,7.56756663677444));
#17760=CARTESIAN_POINT('Ctrl Pts',(13.7730330635226,-14.659900583067,7.58624975577124));
#17761=CARTESIAN_POINT('Ctrl Pts',(13.8942712821964,-14.4465216732759,7.59504406396131));
#17762=CARTESIAN_POINT('Ctrl Pts',(14.2171369312795,-14.0690784754299,7.61553100416422));
#17763=CARTESIAN_POINT('Ctrl Pts',(14.4186919319085,-13.9112790359548,7.62661812011093));
#17764=CARTESIAN_POINT('Ctrl Pts',(14.863092069992,-13.6881435985439,7.6483341974395));
#17765=CARTESIAN_POINT('Ctrl Pts',(15.1000019202232,-13.6215707720726,7.65876535937924));
#17766=CARTESIAN_POINT('Ctrl Pts',(15.5923708701065,-13.5808635018622,7.67830856382976));
#17767=CARTESIAN_POINT('Ctrl Pts',(15.8433379208265,-13.6095625320068,7.68782548676811));
#17768=CARTESIAN_POINT('Ctrl Pts',(16.3199700807978,-13.7623781380245,7.70922458395993));
#17769=CARTESIAN_POINT('Ctrl Pts',(16.5409454194786,-13.8850350400053,7.72027877065713));
#17770=CARTESIAN_POINT('Ctrl Pts',(16.915923850466,-14.2029253271881,7.741437387923));
#17771=CARTESIAN_POINT('Ctrl Pts',(17.0686294557123,-14.3924762194996,7.75105189061667));
#17772=CARTESIAN_POINT('Ctrl Pts',(17.3004182538365,-14.8282704095303,7.7701155034789));
#17773=CARTESIAN_POINT('Ctrl Pts',(17.373468436966,-15.0724279299405,7.78079605992729));
#17774=CARTESIAN_POINT('Ctrl Pts',(17.4197196437091,-15.5700126415031,7.80256267023187));
#17775=CARTESIAN_POINT('Ctrl Pts',(17.394416640621,-15.8184641689756,7.81343106600931));
#17776=CARTESIAN_POINT('Ctrl Pts',(17.251739357461,-16.2868291909747,7.8339194746707));
#17777=CARTESIAN_POINT('Ctrl Pts',(17.1376299104146,-16.502923705768,7.84272977902298));
#17778=CARTESIAN_POINT('Ctrl Pts',(16.8269990788688,-16.8902375863567,7.86296911111449));
#17779=CARTESIAN_POINT('Ctrl Pts',(16.6297938822244,-17.0547467440568,7.87403819636831));
#17780=CARTESIAN_POINT('Ctrl Pts',(16.1910433456394,-17.2920048615472,7.8958491399095));
#17781=CARTESIAN_POINT('Ctrl Pts',(15.9555300502227,-17.3658328375752,7.90638608150065));
#17782=CARTESIAN_POINT('Ctrl Pts',(15.4660857345857,-17.4207687430086,7.92612970196418));
#17783=CARTESIAN_POINT('Ctrl Pts',(15.2166577830259,-17.4000604106139,7.93534214140658));
#17784=CARTESIAN_POINT('Ctrl Pts',(14.736659339645,-17.2633485083323,7.95651654197027));
#17785=CARTESIAN_POINT('Ctrl Pts',(14.5111157371733,-17.1474800469075,7.96759531362881));
#17786=CARTESIAN_POINT('Ctrl Pts',(14.1252489758112,-16.840732545736,7.98892270507244));
#17787=CARTESIAN_POINT('Ctrl Pts',(13.9663704305421,-16.6556076801852,7.99894848293143));
#17788=CARTESIAN_POINT('Ctrl Pts',(13.7210808802104,-16.2267404176834,8.01770908059117));
#17789=CARTESIAN_POINT('Ctrl Pts',(13.6405741651424,-15.9849881593637,8.02828441997523));
#17790=CARTESIAN_POINT('Ctrl Pts',(13.5998236036108,-15.6566231870054,8.0426485919944));
#17791=CARTESIAN_POINT('Ctrl Pts',(13.595,-15.5782696639076,8.0460761301877));
#17792=CARTESIAN_POINT('Ctrl Pts',(13.595,-15.5,8.04949999999993));
#17793=CARTESIAN_POINT('Ctrl Pts',(13.595,-15.5,8.11199999999998));
#17794=CARTESIAN_POINT('Ctrl Pts',(13.595,-15.5401785671646,8.1102424073856));
#17795=CARTESIAN_POINT('Ctrl Pts',(13.5962710960814,-15.5803978824981,8.1084830322617));
#17796=CARTESIAN_POINT('Ctrl Pts',(13.6147984492805,-15.8724739282841,8.0957063023498));
#17797=CARTESIAN_POINT('Ctrl Pts',(13.6806733388295,-16.1187040113957,8.08493508261613));
#17798=CARTESIAN_POINT('Ctrl Pts',(13.8995422577313,-16.5609698965807,8.06558836847855));
#17799=CARTESIAN_POINT('Ctrl Pts',(14.0464846665982,-16.7547659878573,8.05628688580874));
#17800=CARTESIAN_POINT('Ctrl Pts',(14.4111890709962,-17.0829706259866,8.03529189026432));
#17801=CARTESIAN_POINT('Ctrl Pts',(14.6277011118655,-17.2118407447284,8.02427089345816));
#17802=CARTESIAN_POINT('Ctrl Pts',(15.1009405077996,-17.3797824410656,8.00266948544771));
#17803=CARTESIAN_POINT('Ctrl Pts',(15.3533937102224,-17.4160659498373,7.99279605189069));
#17804=CARTESIAN_POINT('Ctrl Pts',(15.8483877185811,-17.3885984573049,7.9734429839893));
#17805=CARTESIAN_POINT('Ctrl Pts',(16.086392355055,-17.3287429746659,7.96311727083424));
#17806=CARTESIAN_POINT('Ctrl Pts',(16.5356193755658,-17.1187588694243,7.94150598192568));
#17807=CARTESIAN_POINT('Ctrl Pts',(16.7409977273652,-16.9672499532929,7.93041161061722));
#17808=CARTESIAN_POINT('Ctrl Pts',(17.0750695532519,-16.5990575021999,7.909702471796));
#17809=CARTESIAN_POINT('Ctrl Pts',(17.2029358204013,-16.3881325397119,7.90085094224463));
#17810=CARTESIAN_POINT('Ctrl Pts',(17.3725337765339,-15.9279676166023,7.88072124307099));
#17811=CARTESIAN_POINT('Ctrl Pts',(17.412090442216,-15.6828552255489,7.86999891625325));
#17812=CARTESIAN_POINT('Ctrl Pts',(17.3956137144998,-15.1847415035945,7.8482091646367));
#17813=CARTESIAN_POINT('Ctrl Pts',(17.3372094330798,-14.9365988780476,7.8373542816294));
#17814=CARTESIAN_POINT('Ctrl Pts',(17.1317475349455,-14.4877852505327,7.81772113956837));
#17815=CARTESIAN_POINT('Ctrl Pts',(16.9906514017321,-14.2895661627728,7.80866338860339));
#17816=CARTESIAN_POINT('Ctrl Pts',(16.6364533234906,-13.9509993026596,7.78783976814033));
#17817=CARTESIAN_POINT('Ctrl Pts',(16.4246495253351,-13.8159724508042,7.77686247611286));
#17818=CARTESIAN_POINT('Ctrl Pts',(15.9577517677181,-13.6336642077804,7.75518708501145));
#17819=CARTESIAN_POINT('Ctrl Pts',(15.706738432325,-13.5895132845942,7.74495206001905));
#17820=CARTESIAN_POINT('Ctrl Pts',(15.2120813267271,-13.6013388582683,7.72595387950955));
#17821=CARTESIAN_POINT('Ctrl Pts',(14.9730376353124,-13.6533547357279,7.71576027285558));
#17822=CARTESIAN_POINT('Ctrl Pts',(14.5186634602065,-13.8478992469824,7.69429168868705));
#17823=CARTESIAN_POINT('Ctrl Pts',(14.3090682860259,-13.9919724974815,7.68320020265902));
#17824=CARTESIAN_POINT('Ctrl Pts',(13.9620507431484,-14.349204207856,7.66224036613768));
#17825=CARTESIAN_POINT('Ctrl Pts',(13.8263901549087,-14.5573208660807,7.6532370574768));
#17826=CARTESIAN_POINT('Ctrl Pts',(13.6422128223145,-15.0125264805873,7.63332430093671));
#17827=CARTESIAN_POINT('Ctrl Pts',(13.595,-15.2551322722671,7.62271162413527));
#17828=CARTESIAN_POINT('Ctrl Pts',(13.595,-15.5,7.61199999999997));
#17829=CARTESIAN_POINT('Origin',(15.5,-15.5,-1.713));
#17830=CARTESIAN_POINT('',(13.595,-15.5,7.04949999999992));
#17831=CARTESIAN_POINT('',(13.595,-15.5,7.11199999999996));
#17832=CARTESIAN_POINT('',(13.595,-15.5,-1.713));
#17833=CARTESIAN_POINT('Ctrl Pts',(13.595,-15.5,7.04949999999992));
#17834=CARTESIAN_POINT('Ctrl Pts',(13.595,-15.4991343357693,7.0495378680765));
#17835=CARTESIAN_POINT('Ctrl Pts',(13.5950005900588,-15.4982686422646,7.04957573743363));
#17836=CARTESIAN_POINT('Ctrl Pts',(13.5953359924214,-15.2522458300719,7.06033789019796));
#17837=CARTESIAN_POINT('Ctrl Pts',(13.6429915679965,-15.0094264327662,7.07095991107749));
#17838=CARTESIAN_POINT('Ctrl Pts',(13.8281413575464,-14.5541898043714,7.09087402430561));
#17839=CARTESIAN_POINT('Ctrl Pts',(13.9642588322537,-14.3462354806215,7.09988894990294));
#17840=CARTESIAN_POINT('Ctrl Pts',(14.3120270236143,-13.9896488844362,7.12086311378916));
#17841=CARTESIAN_POINT('Ctrl Pts',(14.5218599384075,-13.8460122470201,7.13195405663558));
#17842=CARTESIAN_POINT('Ctrl Pts',(14.9765181285096,-13.6523708761749,7.15341364666574));
#17843=CARTESIAN_POINT('Ctrl Pts',(15.2156145109008,-13.6008120471849,7.16359925277241));
#17844=CARTESIAN_POINT('Ctrl Pts',(15.7102416863387,-13.5898965411343,7.18257639417033));
#17845=CARTESIAN_POINT('Ctrl Pts',(15.9611684979088,-13.6345061488357,7.19283493915264));
#17846=CARTESIAN_POINT('Ctrl Pts',(16.4276866352902,-13.8176501538517,7.21451422877673));
#17847=CARTESIAN_POINT('Ctrl Pts',(16.639209586072,-13.9530323355161,7.22548865308526));
#17848=CARTESIAN_POINT('Ctrl Pts',(16.9927905859397,-14.2922022696668,7.2463020868235));
#17849=CARTESIAN_POINT('Ctrl Pts',(17.1335445138208,-14.4906839465111,7.25534794166705));
#17850=CARTESIAN_POINT('Ctrl Pts',(17.3382125741074,-14.939879781951,7.27499780323484));
#17851=CARTESIAN_POINT('Ctrl Pts',(17.3961740690682,-15.1881280415524,7.28585730715441));
#17852=CARTESIAN_POINT('Ctrl Pts',(17.411759261701,-15.6862300439605,7.3076465461049));
#17853=CARTESIAN_POINT('Ctrl Pts',(17.3717796671033,-15.931229923178,7.31836395114503));
#17854=CARTESIAN_POINT('Ctrl Pts',(17.2013748154031,-16.3911426119783,7.33848261644689));
#17855=CARTESIAN_POINT('Ctrl Pts',(17.0730862086873,-16.6019133458283,7.34734007234671));
#17856=CARTESIAN_POINT('Ctrl Pts',(16.738306266743,-16.9695140895441,7.36806309536767));
#17857=CARTESIAN_POINT('Ctrl Pts',(16.5326916408181,-17.1206209283353,7.37915762331326));
#17858=CARTESIAN_POINT('Ctrl Pts',(16.0831710552844,-17.3297672625767,7.40076170965258));
#17859=CARTESIAN_POINT('Ctrl Pts',(15.8451032740296,-17.3891960800257,7.41108048284215));
#17860=CARTESIAN_POINT('Ctrl Pts',(15.349945156537,-17.415819935853,7.43042131558722));
#17861=CARTESIAN_POINT('Ctrl Pts',(15.0973957888155,-17.3790480412991,7.4403198361288));
#17862=CARTESIAN_POINT('Ctrl Pts',(14.624381465431,-17.2101381010058,7.46193389520805));
#17863=CARTESIAN_POINT('Ctrl Pts',(14.4081606488506,-17.0808758006958,7.47295243720896));
#17864=CARTESIAN_POINT('Ctrl Pts',(14.0441154296759,-16.7520156512514,7.49393679777999));
#17865=CARTESIAN_POINT('Ctrl Pts',(13.8975410797082,-16.557944605115,7.50322070843755));
#17866=CARTESIAN_POINT('Ctrl Pts',(13.6795074139451,-16.1152657431494,7.52258548805109));
#17867=CARTESIAN_POINT('Ctrl Pts',(13.6140973678417,-15.8689094193862,7.53336223012298));
#17868=CARTESIAN_POINT('Ctrl Pts',(13.5961963787309,-15.5779984871332,7.54608799268872));
#17869=CARTESIAN_POINT('Ctrl Pts',(13.595,-15.5389797868994,7.54779484746714));
#17870=CARTESIAN_POINT('Ctrl Pts',(13.595,-15.5,7.54949999999993));
#17871=CARTESIAN_POINT('Ctrl Pts',(13.595,-15.5,7.61199999999997));
#17872=CARTESIAN_POINT('Ctrl Pts',(13.595,-15.5003277274783,7.61198566371483));
#17873=CARTESIAN_POINT('Ctrl Pts',(13.5950000845712,-15.5006554590083,7.6119713272525));
#17874=CARTESIAN_POINT('Ctrl Pts',(13.5951318731733,-15.756003956838,7.60080122673501));
#17875=CARTESIAN_POINT('Ctrl Pts',(13.6464713038349,-16.0084388450233,7.58975858070765));
#17876=CARTESIAN_POINT('Ctrl Pts',(13.8402272920192,-16.4656697349393,7.56975722944273));
#17877=CARTESIAN_POINT('Ctrl Pts',(13.9758927039181,-16.6681042598835,7.56085667132801));
#17878=CARTESIAN_POINT('Ctrl Pts',(14.3202774206731,-17.0161921226041,7.54019657313268));
#17879=CARTESIAN_POINT('Ctrl Pts',(14.5275609955708,-17.1567860835421,7.52926875939176));
#17880=CARTESIAN_POINT('Ctrl Pts',(14.98821042329,-17.3522284718803,7.50754280572542));
#17881=CARTESIAN_POINT('Ctrl Pts',(15.2377713581851,-17.4036653753014,7.49696342859849));
#17882=CARTESIAN_POINT('Ctrl Pts',(15.7318010893369,-17.4062280475813,7.47819161610757));
#17883=CARTESIAN_POINT('Ctrl Pts',(15.9715890158941,-17.3614766858768,7.46818242672917));
#17884=CARTESIAN_POINT('Ctrl Pts',(16.430331989696,-17.1812346610907,7.44686116332088));
#17885=CARTESIAN_POINT('Ctrl Pts',(16.6435859613336,-17.0441123582632,7.43578310084013));
#17886=CARTESIAN_POINT('Ctrl Pts',(17.0024361354668,-16.6971786416951,7.41460023884381));
#17887=CARTESIAN_POINT('Ctrl Pts',(17.1453663198282,-16.4916203149371,7.40537796653269));
#17888=CARTESIAN_POINT('Ctrl Pts',(17.343025031331,-16.0404494919582,7.38564171005943));
#17889=CARTESIAN_POINT('Ctrl Pts',(17.3971063213366,-15.7996614304134,7.37510854901198));
#17890=CARTESIAN_POINT('Ctrl Pts',(17.4115724937508,-15.3011360430778,7.35330078928601));
#17891=CARTESIAN_POINT('Ctrl Pts',(17.3680035532163,-15.0480770644475,7.34223084271425));
#17892=CARTESIAN_POINT('Ctrl Pts',(17.1884401117818,-14.5851921801101,7.32198216010981));
#17893=CARTESIAN_POINT('Ctrl Pts',(17.0585725890897,-14.378145289724,7.3131739326621));
#17894=CARTESIAN_POINT('Ctrl Pts',(16.7246962104993,-14.0200205218403,7.29269240118683));
#17895=CARTESIAN_POINT('Ctrl Pts',(16.5223738539402,-13.8736657419208,7.28182653546096));
#17896=CARTESIAN_POINT('Ctrl Pts',(16.0685961246215,-13.6644071382625,7.26005871642812));
#17897=CARTESIAN_POINT('Ctrl Pts',(15.8206918399668,-13.6053010700133,7.24937435762049));
#17898=CARTESIAN_POINT('Ctrl Pts',(15.3274201195724,-13.5875624482055,7.2302993291107));
#17899=CARTESIAN_POINT('Ctrl Pts',(15.0868812502939,-13.6247482194238,7.22069879957406));
#17900=CARTESIAN_POINT('Ctrl Pts',(14.6239355064353,-13.7899780527012,7.19954666959181));
#17901=CARTESIAN_POINT('Ctrl Pts',(14.4070929248025,-13.9197406682961,7.18849362969182));
#17902=CARTESIAN_POINT('Ctrl Pts',(14.0359738459738,-14.255689902187,7.16708622955883));
#17903=CARTESIAN_POINT('Ctrl Pts',(13.885343874168,-14.4585836779553,7.15755626955576));
#17904=CARTESIAN_POINT('Ctrl Pts',(13.6738959314522,-14.905167345095,7.1380206760676));
#17905=CARTESIAN_POINT('Ctrl Pts',(13.6128351904539,-15.1435292900942,7.12759364435285));
#17906=CARTESIAN_POINT('Ctrl Pts',(13.5961178635103,-15.4246035725244,7.11529818142939));
#17907=CARTESIAN_POINT('Ctrl Pts',(13.595,-15.4623209809862,7.11364825105044));
#17908=CARTESIAN_POINT('Ctrl Pts',(13.595,-15.5,7.11199999999997));
#17909=CARTESIAN_POINT('Origin',(15.5,-15.5,-1.713));
#17910=CARTESIAN_POINT('',(13.595,-15.5,6.54949999999991));
#17911=CARTESIAN_POINT('',(13.595,-15.5,6.61199999999996));
#17912=CARTESIAN_POINT('',(13.595,-15.5,-1.713));
#17913=CARTESIAN_POINT('Ctrl Pts',(13.595,-15.5,6.54949999999991));
#17914=CARTESIAN_POINT('Ctrl Pts',(13.595,-15.4610626456773,6.55120329633949));
#17915=CARTESIAN_POINT('Ctrl Pts',(13.5961937741644,-15.4220849065524,6.55290835929331));
#17916=CARTESIAN_POINT('Ctrl Pts',(13.6135439126654,-15.1398288859061,6.5652555168019));
#17917=CARTESIAN_POINT('Ctrl Pts',(13.6750573440076,-14.901632385016,6.57567531124154));
#17918=CARTESIAN_POINT('Ctrl Pts',(13.8874077255788,-14.455352793198,6.5951976030971));
#17919=CARTESIAN_POINT('Ctrl Pts',(14.0385487102697,-14.2526346764271,6.60475060010868));
#17920=CARTESIAN_POINT('Ctrl Pts',(14.4104722647551,-13.9174172546469,6.62617247050852));
#17921=CARTESIAN_POINT('Ctrl Pts',(14.6275426754921,-13.7881425696087,6.6372234693111));
#17922=CARTESIAN_POINT('Ctrl Pts',(15.0907593985093,-13.6239010437341,6.6583642485118));
#17923=CARTESIAN_POINT('Ctrl Pts',(15.3313513363661,-13.5872144057403,6.66794064636249));
#17924=CARTESIAN_POINT('Ctrl Pts',(15.8245674377791,-13.6059607746345,6.68703560952199));
#17925=CARTESIAN_POINT('Ctrl Pts',(16.0723530201276,-13.6655746954185,6.69772657931191));
#17926=CARTESIAN_POINT('Ctrl Pts',(16.5256592868876,-13.8757431795112,6.71949643866254));
#17927=CARTESIAN_POINT('Ctrl Pts',(16.7276463839847,-14.0224749216709,6.73035784847893));
#17928=CARTESIAN_POINT('Ctrl Pts',(17.0608214992481,-14.3812638928176,6.75082734101175));
#17929=CARTESIAN_POINT('Ctrl Pts',(17.1903023731798,-14.5886223743785,6.75963221235241));
#17930=CARTESIAN_POINT('Ctrl Pts',(17.368912415714,-15.0518806845181,6.77989723029377));
#17931=CARTESIAN_POINT('Ctrl Pts',(17.4119607652391,-15.304973303584,6.79096864845063));
#17932=CARTESIAN_POINT('Ctrl Pts',(17.3965108544052,-15.8033698669453,6.81277077283214));
#17933=CARTESIAN_POINT('Ctrl Pts',(17.3419722590831,-16.0440060481921,6.82329728994705));
#17934=CARTESIAN_POINT('Ctrl Pts',(17.1434168441495,-16.4948819322832,6.84302064445673));
#17935=CARTESIAN_POINT('Ctrl Pts',(16.9999920718481,-16.70026790681,6.85226039867485));
#17936=CARTESIAN_POINT('Ctrl Pts',(16.6403455757613,-17.0464984224452,6.87345804783543));
#17937=CARTESIAN_POINT('Ctrl Pts',(16.4268522650442,-17.1831477172723,6.88453483165137));
#17938=CARTESIAN_POINT('Ctrl Pts',(15.9678323975632,-17.3624186317035,6.90584534448146));
#17939=CARTESIAN_POINT('Ctrl Pts',(15.7279989456845,-17.4066813297663,6.91582574173733));
#17940=CARTESIAN_POINT('Ctrl Pts',(15.2340134689555,-17.403144337622,6.93461718828239));
#17941=CARTESIAN_POINT('Ctrl Pts',(14.9845514966635,-17.3512140199344,6.94520360841043));
#17942=CARTESIAN_POINT('Ctrl Pts',(14.5243302645298,-17.1548784572058,6.96693287611617));
#17943=CARTESIAN_POINT('Ctrl Pts',(14.3173601839665,-17.0139100171481,6.97785700418355));
#17944=CARTESIAN_POINT('Ctrl Pts',(13.9736471620034,-16.6651757950803,6.99850579332026));
#17945=CARTESIAN_POINT('Ctrl Pts',(13.8383527355207,-16.462449567229,7.00739809417185));
#17946=CARTESIAN_POINT('Ctrl Pts',(13.6458350057992,-16.0056519828164,7.02738049069033));
#17947=CARTESIAN_POINT('Ctrl Pts',(13.595,-15.7540869989855,7.03838508315891));
#17948=CARTESIAN_POINT('Ctrl Pts',(13.595,-15.5,7.04949999999992));
#17949=CARTESIAN_POINT('Ctrl Pts',(13.595,-15.5,7.11199999999997));
#17950=CARTESIAN_POINT('Ctrl Pts',(13.595,-15.7151084711071,7.10259018061645));
#17951=CARTESIAN_POINT('Ctrl Pts',(13.6314375584287,-15.9289657393821,7.09323509451523));
#17952=CARTESIAN_POINT('Ctrl Pts',(13.7837888964782,-16.3618713020821,7.0742978433035));
#17953=CARTESIAN_POINT('Ctrl Pts',(13.9077406040965,-16.5737379336832,7.06550254240705));
#17954=CARTESIAN_POINT('Ctrl Pts',(14.2308903575243,-16.9419485720183,7.04520677622757));
#17955=CARTESIAN_POINT('Ctrl Pts',(14.4280313004595,-17.0939658080948,7.03441335178549));
#17956=CARTESIAN_POINT('Ctrl Pts',(14.8744284026619,-17.3169710492469,7.0126244694032));
#17957=CARTESIAN_POINT('Ctrl Pts',(15.1204083881536,-17.3837876812905,7.00184436300425));
#17958=CARTESIAN_POINT('Ctrl Pts',(15.6127593154075,-17.4168741618687,6.98246852525851));
#17959=CARTESIAN_POINT('Ctrl Pts',(15.8541502591357,-17.3872519912577,6.97319522635436));
#17960=CARTESIAN_POINT('Ctrl Pts',(16.3211196205183,-17.236959840026,6.95221738709966));
#17961=CARTESIAN_POINT('Ctrl Pts',(16.5412928197739,-17.1146128808544,6.94120036770448));
#17962=CARTESIAN_POINT('Ctrl Pts',(16.9245245713851,-16.7898416281419,6.9195785803559));
#17963=CARTESIAN_POINT('Ctrl Pts',(17.082933253164,-16.5896119800978,6.90966456605852));
#17964=CARTESIAN_POINT('Ctrl Pts',(17.3079526732748,-16.1476518931442,6.89033122892145));
#17965=CARTESIAN_POINT('Ctrl Pts',(17.375764904958,-15.9118621302026,6.88001671610686));
#17966=CARTESIAN_POINT('Ctrl Pts',(17.4199326181634,-15.4180941903735,6.85841706869526));
#17967=CARTESIAN_POINT('Ctrl Pts',(17.3921628352553,-15.164471498879,6.84732246276811));
#17968=CARTESIAN_POINT('Ctrl Pts',(17.2417314993585,-14.6905493102034,6.82659095845158));
#17969=CARTESIAN_POINT('Ctrl Pts',(17.1235538851641,-14.4738860201229,6.81772974273954));
#17970=CARTESIAN_POINT('Ctrl Pts',(16.8108405892163,-14.0960047381003,6.7976178311296));
#17971=CARTESIAN_POINT('Ctrl Pts',(16.6188433475139,-13.9386922264281,6.78690345035065));
#17972=CARTESIAN_POINT('Ctrl Pts',(16.1799611386208,-13.7026704139082,6.7651145593432));
#17973=CARTESIAN_POINT('Ctrl Pts',(15.9360709048723,-13.6284758145378,6.75425224797636));
#17974=CARTESIAN_POINT('Ctrl Pts',(15.4447624444838,-13.5805885181933,6.73459217553703));
#17975=CARTESIAN_POINT('Ctrl Pts',(15.2024607337532,-13.6029827990872,6.72555345744808));
#17976=CARTESIAN_POINT('Ctrl Pts',(14.7318101012877,-13.7390972895958,6.70474625494253));
#17977=CARTESIAN_POINT('Ctrl Pts',(14.5087023988878,-13.854333231983,6.69377359924472));
#17978=CARTESIAN_POINT('Ctrl Pts',(14.1165104476134,-14.1663212633333,6.67209196282133));
#17979=CARTESIAN_POINT('Ctrl Pts',(13.9521980321027,-14.3611392816342,6.66181892906235));
#17980=CARTESIAN_POINT('Ctrl Pts',(13.7138657210454,-14.7946622708063,6.64285466881861));
#17981=CARTESIAN_POINT('Ctrl Pts',(13.6387111132089,-15.0273931336094,6.63267396615881));
#17982=CARTESIAN_POINT('Ctrl Pts',(13.5997187869975,-15.345083827799,6.61877673544186));
#17983=CARTESIAN_POINT('Ctrl Pts',(13.595,-15.4225853386876,6.61538646812386));
#17984=CARTESIAN_POINT('Ctrl Pts',(13.595,-15.5,6.61199999999996));
#17985=CARTESIAN_POINT('Origin',(15.5,-15.5,-1.713));
#17986=CARTESIAN_POINT('',(13.595,-15.5000000000007,6.04949999999984));
#17987=CARTESIAN_POINT('',(13.595,-15.5,6.11199999999995));
#17988=CARTESIAN_POINT('',(13.595,-15.5,-1.713));
#17989=CARTESIAN_POINT('Ctrl Pts',(13.595,-15.5000000000014,6.04949999999984));
#17990=CARTESIAN_POINT('Ctrl Pts',(13.5949999999999,-15.4212996333131,6.05294271070362));
#17991=CARTESIAN_POINT('Ctrl Pts',(13.5998768365782,-15.3425152813848,6.05638909525989));
#17992=CARTESIAN_POINT('Ctrl Pts',(13.6396656510538,-15.0236734792597,6.07033668065492));
#17993=CARTESIAN_POINT('Ctrl Pts',(13.7152677517337,-14.791138118477,6.08050883121264));
#17994=CARTESIAN_POINT('Ctrl Pts',(13.9544193128816,-14.3581281491297,6.09945064964428));
#17995=CARTESIAN_POINT('Ctrl Pts',(14.1191066045505,-14.1636342658724,6.1097490860317));
#17996=CARTESIAN_POINT('Ctrl Pts',(14.5118631593489,-13.8524405146268,6.13143473911924));
#17997=CARTESIAN_POINT('Ctrl Pts',(14.7351471528063,-13.7376518540051,6.14240429033984));
#17998=CARTESIAN_POINT('Ctrl Pts',(15.2060239795073,-13.6024250338468,6.16320064659774));
#17999=CARTESIAN_POINT('Ctrl Pts',(15.4483861027075,-13.5804852546147,6.17222719514705));
#18000=CARTESIAN_POINT('Ctrl Pts',(15.9396234792267,-13.6293069089211,6.19190501117974));
#18001=CARTESIAN_POINT('Ctrl Pts',(16.1833741630851,-13.7039650529646,6.20277217462826));
#18002=CARTESIAN_POINT('Ctrl Pts',(16.6217691980785,-13.9408001486887,6.2245603979467));
#18003=CARTESIAN_POINT('Ctrl Pts',(16.8134370968083,-14.0984413002525,6.23526949003646));
#18004=CARTESIAN_POINT('Ctrl Pts',(17.1254884498018,-14.4769312778602,6.25536963823337));
#18005=CARTESIAN_POINT('Ctrl Pts',(17.2432989432679,-14.6939024955189,6.2642376419736));
#18006=CARTESIAN_POINT('Ctrl Pts',(17.3928068238889,-15.1681616774429,6.28498388790203));
#18007=CARTESIAN_POINT('Ctrl Pts',(17.4200800648353,-15.4217867335681,6.29607859726884));
#18008=CARTESIAN_POINT('Ctrl Pts',(17.3749840443236,-15.9153766743346,6.31767045819477));
#18009=CARTESIAN_POINT('Ctrl Pts',(17.3067452371384,-16.150996284795,6.32797752776871));
#18010=CARTESIAN_POINT('Ctrl Pts',(17.0808598623415,-16.5926576436372,6.34729779718439));
#18011=CARTESIAN_POINT('Ctrl Pts',(16.9219479764644,-16.7927154491698,6.357239048736));
#18012=CARTESIAN_POINT('Ctrl Pts',(16.5379425112565,-17.1167607502192,6.37887426914662));
#18013=CARTESIAN_POINT('Ctrl Pts',(16.3175639018305,-17.2386290144578,6.38988860013231));
#18014=CARTESIAN_POINT('Ctrl Pts',(15.8503415097167,-17.3879626090542,6.41085505936614));
#18015=CARTESIAN_POINT('Ctrl Pts',(15.608892168395,-17.4170977909834,6.42011013650055));
#18016=CARTESIAN_POINT('Ctrl Pts',(15.1166063757536,-17.3830178532379,6.43950523585411));
#18017=CARTESIAN_POINT('Ctrl Pts',(14.870759502855,-17.3157040667844,6.4502911733256));
#18018=CARTESIAN_POINT('Ctrl Pts',(14.4248547550533,-17.0918174858598,6.47208068031278));
#18019=CARTESIAN_POINT('Ctrl Pts',(14.2280546533922,-16.9394396391344,6.48286907973836));
#18020=CARTESIAN_POINT('Ctrl Pts',(13.9056026551441,-16.5705783121195,6.50315264428303));
#18021=CARTESIAN_POINT('Ctrl Pts',(13.7820360793138,-16.3583941382296,6.51194995020858));
#18022=CARTESIAN_POINT('Ctrl Pts',(13.630989180424,-15.9263442702941,6.53084976945334));
#18023=CARTESIAN_POINT('Ctrl Pts',(13.595,-15.7137808200968,6.54014825808841));
#18024=CARTESIAN_POINT('Ctrl Pts',(13.595,-15.5,6.54949999999991));
#18025=CARTESIAN_POINT('Ctrl Pts',(13.595,-15.5,6.61199999999996));
#18026=CARTESIAN_POINT('Ctrl Pts',(13.595,-15.6733284920729,6.60441782624349));
#18027=CARTESIAN_POINT('Ctrl Pts',(13.6186572328438,-15.8462216114541,6.59685469766167));
#18028=CARTESIAN_POINT('Ctrl Pts',(13.7320473190416,-16.2510329369089,6.57914641570826));
#18029=CARTESIAN_POINT('Ctrl Pts',(13.8438568570137,-16.4730835714652,6.57012424533666));
#18030=CARTESIAN_POINT('Ctrl Pts',(14.1451247601535,-16.8614120171819,6.55021742642492));
#18031=CARTESIAN_POINT('Ctrl Pts',(14.3313806311313,-17.0242843089789,6.53959894603257));
#18032=CARTESIAN_POINT('Ctrl Pts',(14.7638243009585,-17.275405367102,6.51772371712454));
#18033=CARTESIAN_POINT('Ctrl Pts',(15.0077751382723,-17.3578889533404,6.50667781093437));
#18034=CARTESIAN_POINT('Ctrl Pts',(15.5004085561524,-17.4202581848602,6.48665079123196));
#18035=CARTESIAN_POINT('Ctrl Pts',(15.7436629817923,-17.4047379468316,6.47776337013216));
#18036=CARTESIAN_POINT('Ctrl Pts',(16.2176685098711,-17.2819927315602,6.45712148752121));
#18037=CARTESIAN_POINT('Ctrl Pts',(16.443337539286,-17.1735154737238,6.44619962657462));
#18038=CARTESIAN_POINT('Ctrl Pts',(16.8438200723545,-16.8736189807942,6.42446838012343));
#18039=CARTESIAN_POINT('Ctrl Pts',(17.0137541208759,-16.6837468325642,6.41387768558701));
#18040=CARTESIAN_POINT('Ctrl Pts',(17.2643108649679,-16.258032038322,6.39507427777451));
#18041=CARTESIAN_POINT('Ctrl Pts',(17.3461668124714,-16.0283235145553,6.38511126485366));
#18042=CARTESIAN_POINT('Ctrl Pts',(17.4210201547905,-15.5413152243351,6.36380731515024));
#18043=CARTESIAN_POINT('Ctrl Pts',(17.4097474835946,-15.2881182828737,6.35273133345901));
#18044=CARTESIAN_POINT('Ctrl Pts',(17.2903402726451,-14.803334467194,6.33152469235316));
#18045=CARTESIAN_POINT('Ctrl Pts',(17.1844249027143,-14.5762233150762,6.32227412134972));
#18046=CARTESIAN_POINT('Ctrl Pts',(16.893661371229,-14.1784483926715,6.3025586328999));
#18047=CARTESIAN_POINT('Ctrl Pts',(16.7127531792213,-14.01070398294,6.29203617905489));
#18048=CARTESIAN_POINT('Ctrl Pts',(16.2892221203122,-13.7476468776041,6.27023752599387));
#18049=CARTESIAN_POINT('Ctrl Pts',(16.0486544659216,-13.6580970861074,6.25916523396503));
#18050=CARTESIAN_POINT('Ctrl Pts',(15.5582496795982,-13.5805324739975,6.23889028605827));
#18051=CARTESIAN_POINT('Ctrl Pts',(15.3138847564439,-13.5886882666418,6.23008728511492));
#18052=CARTESIAN_POINT('Ctrl Pts',(14.8364404563567,-13.6972603894447,6.20962512613989));
#18053=CARTESIAN_POINT('Ctrl Pts',(14.6082773598722,-13.7985291079087,6.19876644735625));
#18054=CARTESIAN_POINT('Ctrl Pts',(14.1992779535143,-14.0854940002442,6.17699539214162));
#18055=CARTESIAN_POINT('Ctrl Pts',(14.0235269280418,-14.2700582652036,6.16630042340671));
#18056=CARTESIAN_POINT('Ctrl Pts',(13.7601702895471,-14.6874866951327,6.14719334754687));
#18057=CARTESIAN_POINT('Ctrl Pts',(13.6713668820483,-14.914065163743,6.13763144515555));
#18058=CARTESIAN_POINT('Ctrl Pts',(13.6057278858963,-15.2665198483617,6.12221347994914));
#18059=CARTESIAN_POINT('Ctrl Pts',(13.595,-15.3832758813928,6.11710604193377));
#18060=CARTESIAN_POINT('Ctrl Pts',(13.595,-15.5,6.11199999999995));
#18061=CARTESIAN_POINT('Origin',(15.5,-15.5,-1.713));
#18062=CARTESIAN_POINT('',(13.595,-15.5,5.5494999999999));
#18063=CARTESIAN_POINT('',(13.595,-15.5,5.61199999999994));
#18064=CARTESIAN_POINT('',(13.595,-15.5,-1.713));
#18065=CARTESIAN_POINT('Ctrl Pts',(13.595,-15.5,5.5494999999999));
#18066=CARTESIAN_POINT('Ctrl Pts',(13.595,-15.3804229784334,5.55473084083833));
#18067=CARTESIAN_POINT('Ctrl Pts',(13.6062587391732,-15.2608257903983,5.55996256384943));
#18068=CARTESIAN_POINT('Ctrl Pts',(13.6760576354803,-14.8951700410971,5.57595800345141));
#18069=CARTESIAN_POINT('Ctrl Pts',(13.7720096984448,-14.659399845156,5.58575619329743));
#18070=CARTESIAN_POINT('Ctrl Pts',(14.0452839613624,-14.2461894092018,5.6051467301244));
#18071=CARTESIAN_POINT('Ctrl Pts',(14.2171584892425,-14.0708266465022,5.61549358440075));
#18072=CARTESIAN_POINT('Ctrl Pts',(14.6253952287875,-13.7888522129699,5.63712659419822));
#18073=CARTESIAN_POINT('Ctrl Pts',(14.8599977473058,-13.6879934063342,5.6482202575467));
#18074=CARTESIAN_POINT('Ctrl Pts',(15.3463800940963,-13.5855686749737,5.66888656699346));
#18075=CARTESIAN_POINT('Ctrl Pts',(15.5927427947672,-13.5816559429033,5.67772159176443));
#18076=CARTESIAN_POINT('Ctrl Pts',(16.0754846316176,-13.667400719653,5.69788515618075));
#18077=CARTESIAN_POINT('Ctrl Pts',(16.3071807117551,-13.7569999255946,5.70862243939717));
#18078=CARTESIAN_POINT('Ctrl Pts',(16.7289712752251,-14.0227167140848,5.73041332904226));
#18079=CARTESIAN_POINT('Ctrl Pts',(16.9136998866891,-14.1983819978148,5.74125376264675));
#18080=CARTESIAN_POINT('Ctrl Pts',(17.1974101361019,-14.6022492014921,5.76083529742995));
#18081=CARTESIAN_POINT('Ctrl Pts',(17.2972979319089,-14.8240619808842,5.76993140773759));
#18082=CARTESIAN_POINT('Ctrl Pts',(17.410842370381,-15.3008057952467,5.79078634274907));
#18083=CARTESIAN_POINT('Ctrl Pts',(17.4204935309802,-15.5519439892812,5.80177226549774));
#18084=CARTESIAN_POINT('Ctrl Pts',(17.342110451467,-16.0471583288573,5.82343518498926));
#18085=CARTESIAN_POINT('Ctrl Pts',(17.2534824024277,-16.286136426886,5.83359920856734));
#18086=CARTESIAN_POINT('Ctrl Pts',(16.9934395803382,-16.7072759792659,5.85266191487493));
#18087=CARTESIAN_POINT('Ctrl Pts',(16.8277337075192,-16.8874355430668,5.86287999349777));
#18088=CARTESIAN_POINT('Ctrl Pts',(16.4300989084042,-17.181502621719,5.88437585424967));
#18089=CARTESIAN_POINT('Ctrl Pts',(16.1997352103395,-17.2896684655832,5.89546875611168));
#18090=CARTESIAN_POINT('Ctrl Pts',(15.7162942946846,-17.4085782046526,5.91638419721932));
#18091=CARTESIAN_POINT('Ctrl Pts',(15.468499068742,-17.4205357017102,5.92535357637161));
#18092=CARTESIAN_POINT('Ctrl Pts',(14.982450960336,-17.3496956343957,5.94531639540041));
#18093=CARTESIAN_POINT('Ctrl Pts',(14.7487719351981,-17.2677308223166,5.95596181876614));
#18094=CARTESIAN_POINT('Ctrl Pts',(14.3192639573802,-17.0161183157408,5.97773658137359));
#18095=CARTESIAN_POINT('Ctrl Pts',(14.1289503778061,-16.8464743447295,5.9886568954638));
#18096=CARTESIAN_POINT('Ctrl Pts',(13.8321327423216,-16.4516128328056,6.00853801394947));
#18097=CARTESIAN_POINT('Ctrl Pts',(13.7250521360265,-16.2327453046096,6.01744639962329));
#18098=CARTESIAN_POINT('Ctrl Pts',(13.617339209274,-15.8364783055986,6.03478091401572));
#18099=CARTESIAN_POINT('Ctrl Pts',(13.5950000000001,-15.6684314912174,6.04213204325374));
#18100=CARTESIAN_POINT('Ctrl Pts',(13.595,-15.5000000000014,6.04949999999984));
#18101=CARTESIAN_POINT('Ctrl Pts',(13.595,-15.5,6.11199999999995));
#18102=CARTESIAN_POINT('Ctrl Pts',(13.595,-15.6322811156622,6.10621342451166));
#18103=CARTESIAN_POINT('Ctrl Pts',(13.6087783153306,-15.7645212428739,6.10042864204396));
#18104=CARTESIAN_POINT('Ctrl Pts',(13.6882026227428,-16.1396868723561,6.08401719718472));
#18105=CARTESIAN_POINT('Ctrl Pts',(13.7879432930104,-16.3721536353157,6.07445003434073));
#18106=CARTESIAN_POINT('Ctrl Pts',(14.0727367572805,-16.7867289243291,6.05459325308234));
#18107=CARTESIAN_POINT('Ctrl Pts',(14.2556056457461,-16.964313169297,6.043781300895));
#18108=CARTESIAN_POINT('Ctrl Pts',(14.6747839923046,-17.2345693802169,6.02199008469658));
#18109=CARTESIAN_POINT('Ctrl Pts',(14.9057817799496,-17.3266442004838,6.01122510821138));
#18110=CARTESIAN_POINT('Ctrl Pts',(15.3874249059554,-17.417224156811,5.99099741088668));
#18111=CARTESIAN_POINT('Ctrl Pts',(15.6333450122464,-17.4158917348987,5.98218660102253));
#18112=CARTESIAN_POINT('Ctrl Pts',(16.1206259002119,-17.318772490929,5.96160229438465));
#18113=CARTESIAN_POINT('Ctrl Pts',(16.3565452350119,-17.2202990011103,5.95051091721535));
#18114=CARTESIAN_POINT('Ctrl Pts',(16.7681176293856,-16.9422948126497,5.92883837814036));
#18115=CARTESIAN_POINT('Ctrl Pts',(16.9419481430325,-16.7685197996487,5.91845215122558));
#18116=CARTESIAN_POINT('Ctrl Pts',(17.2189872203211,-16.3586015615324,5.89899099646484));
#18117=CARTESIAN_POINT('Ctrl Pts',(17.3171025973776,-16.1247187974314,5.88932803138367));
#18118=CARTESIAN_POINT('Ctrl Pts',(17.4166878372089,-15.6335097383612,5.86784032101315));
#18119=CARTESIAN_POINT('Ctrl Pts',(17.4176502390534,-15.3811120576987,5.85679930261146));
#18120=CARTESIAN_POINT('Ctrl Pts',(17.3237377628468,-14.8990312316065,5.83571090251993));
#18121=CARTESIAN_POINT('Ctrl Pts',(17.2331048196069,-14.6732587208355,5.82624068948459));
#18122=CARTESIAN_POINT('Ctrl Pts',(16.9663803747131,-14.2580406281809,5.80705437314968));
#18123=CARTESIAN_POINT('Ctrl Pts',(16.7891198766685,-14.0749102807301,5.79633358276825));
#18124=CARTESIAN_POINT('Ctrl Pts',(16.3779387565676,-13.7914042355473,5.77455552860573));
#18125=CARTESIAN_POINT('Ctrl Pts',(16.1491538474421,-13.6920495639437,5.76371515769118));
#18126=CARTESIAN_POINT('Ctrl Pts',(15.6708189064625,-13.5872293846082,5.74330132129251));
#18127=CARTESIAN_POINT('Ctrl Pts',(15.426142783217,-13.5810384099919,5.73450737397273));
#18128=CARTESIAN_POINT('Ctrl Pts',(14.9363614071728,-13.6626564055833,5.71416738658206));
#18129=CARTESIAN_POINT('Ctrl Pts',(14.6967303705424,-13.7540722981582,5.70308976140513));
#18130=CARTESIAN_POINT('Ctrl Pts',(14.2756337788508,-14.0202670563068,5.68131470782129));
#18131=CARTESIAN_POINT('Ctrl Pts',(14.0961750870679,-14.1892841101539,5.67081933105237));
#18132=CARTESIAN_POINT('Ctrl Pts',(13.8082370891342,-14.5895773327889,5.65115580383265));
#18133=CARTESIAN_POINT('Ctrl Pts',(13.7039174596371,-14.8180681428012,5.64183078990369));
#18134=CARTESIAN_POINT('Ctrl Pts',(13.6121927841121,-15.20462306897,5.62492112559185));
#18135=CARTESIAN_POINT('Ctrl Pts',(13.595,-15.3522360348498,5.61846386549207));
#18136=CARTESIAN_POINT('Ctrl Pts',(13.595,-15.5,5.61199999999994));
#18137=CARTESIAN_POINT('Origin',(15.5,-15.5,-1.713));
#18138=CARTESIAN_POINT('',(13.595,-15.5,5.04949999999989));
#18139=CARTESIAN_POINT('',(13.595,-15.5,5.11199999999994));
#18140=CARTESIAN_POINT('',(13.595,-15.5,-1.713));
#18141=CARTESIAN_POINT('Ctrl Pts',(13.595,-15.5,5.04949999999989));
#18142=CARTESIAN_POINT('Ctrl Pts',(13.595,-15.3388115089796,5.05655111509265));
#18143=CARTESIAN_POINT('Ctrl Pts',(13.6154590374407,-15.1779059102152,5.06358985519597));
#18144=CARTESIAN_POINT('Ctrl Pts',(13.7183515548725,-14.7816733255799,5.08092286414765));
#18145=CARTESIAN_POINT('Ctrl Pts',(13.8266134541381,-14.5565840536403,5.09007360954104));
#18146=CARTESIAN_POINT('Ctrl Pts',(14.1215467805684,-14.1625430065832,5.10986539767052));
#18147=CARTESIAN_POINT('Ctrl Pts',(14.304585872829,-13.9967060878679,5.1204268571255));
#18148=CARTESIAN_POINT('Ctrl Pts',(14.7316815678331,-13.7383361116675,5.14225803428301));
#18149=CARTESIAN_POINT('Ctrl Pts',(14.9736111872449,-13.6515671979833,5.15332109872661));
#18150=CARTESIAN_POINT('Ctrl Pts',(15.4649173561457,-13.580010626106,5.17349878504518));
#18151=CARTESIAN_POINT('Ctrl Pts',(15.7088324857421,-13.5910780271475,5.18232560154669));
#18152=CARTESIAN_POINT('Ctrl Pts',(16.1849362774886,-13.7052334734392,5.20285909680639));
#18153=CARTESIAN_POINT('Ctrl Pts',(16.4121442114176,-13.8093464029553,5.21374379967087));
#18154=CARTESIAN_POINT('Ctrl Pts',(16.8178401514487,-14.1014316240207,5.23550169996886));
#18155=CARTESIAN_POINT('Ctrl Pts',(16.9913210625043,-14.2881077192111,5.24615685848334));
#18156=CARTESIAN_POINT('Ctrl Pts',(17.2496499625203,-14.7088122754508,5.26514512042844));
#18157=CARTESIAN_POINT('Ctrl Pts',(17.3357238111982,-14.9366074284007,5.27485465566038));
#18158=CARTESIAN_POINT('Ctrl Pts',(17.4197865213486,-15.4212669482105,5.29605585950158));
#18159=CARTESIAN_POINT('Ctrl Pts',(17.4134942607844,-15.674129498803,5.30711721342076));
#18160=CARTESIAN_POINT('Ctrl Pts',(17.303614738454,-16.1620531754266,5.32846120627395));
#18161=CARTESIAN_POINT('Ctrl Pts',(17.2014486992905,-16.3924111516025,5.3378949159657));
#18162=CARTESIAN_POINT('Ctrl Pts',(16.9173100980276,-16.7960756528741,5.35748824481634));
#18163=CARTESIAN_POINT('Ctrl Pts',(16.7398070669348,-16.9667785935818,5.36794640774411));
#18164=CARTESIAN_POINT('Ctrl Pts',(16.3220071965648,-17.2371432267537,5.38968777336196));
#18165=CARTESIAN_POINT('Ctrl Pts',(16.0836525717957,-17.3310448981499,5.40077141272581));
#18166=CARTESIAN_POINT('Ctrl Pts',(15.5947256536311,-17.4180907622543,5.42119774972392));
#18167=CARTESIAN_POINT('Ctrl Pts',(15.3496232410368,-17.4145320800743,5.42998836628871));
#18168=CARTESIAN_POINT('Ctrl Pts',(14.8701126178109,-17.3147175905374,5.45033725630913));
#18169=CARTESIAN_POINT('Ctrl Pts',(14.6405232658285,-17.2179194954329,5.46115218451594));
#18170=CARTESIAN_POINT('Ctrl Pts',(14.2264796200393,-16.9390496379886,5.4829372783152));
#18171=CARTESIAN_POINT('Ctrl Pts',(14.0472256745101,-16.7578504143529,5.49369135016012));
#18172=CARTESIAN_POINT('Ctrl Pts',(13.7760216724758,-16.3455924692783,5.51298262434675));
#18173=CARTESIAN_POINT('Ctrl Pts',(13.6829531189867,-16.1208809938508,5.52233985153742));
#18174=CARTESIAN_POINT('Ctrl Pts',(13.6080918026188,-15.7578640712236,5.53821985690169));
#18175=CARTESIAN_POINT('Ctrl Pts',(13.595,-15.6289437604014,5.54385941555539));
#18176=CARTESIAN_POINT('Ctrl Pts',(13.595,-15.5,5.5494999999999));
#18177=CARTESIAN_POINT('Ctrl Pts',(13.595,-15.5,5.61199999999994));
#18178=CARTESIAN_POINT('Ctrl Pts',(13.595,-15.6018657066951,5.60754393234049));
#18179=CARTESIAN_POINT('Ctrl Pts',(13.6031704055488,-15.7038031752657,5.60308472549142));
#18180=CARTESIAN_POINT('Ctrl Pts',(13.6581997788096,-16.0432791052309,5.5882345098324));
#18181=CARTESIAN_POINT('Ctrl Pts',(13.7418506174913,-16.2721685073446,5.57838310477812));
#18182=CARTESIAN_POINT('Ctrl Pts',(13.9957147777142,-16.6957591219942,5.55950085984424));
#18183=CARTESIAN_POINT('Ctrl Pts',(14.1671636173094,-16.8842814200629,5.54888230343246));
#18184=CARTESIAN_POINT('Ctrl Pts',(14.5698803024982,-17.1808694560447,5.52713878208984));
#18185=CARTESIAN_POINT('Ctrl Pts',(14.7962133781878,-17.2874944048164,5.5162322786931));
#18186=CARTESIAN_POINT('Ctrl Pts',(15.2711157138763,-17.4065903198754,5.49563623999878));
#18187=CARTESIAN_POINT('Ctrl Pts',(15.5146461896474,-17.420222559271,5.4867780974336));
#18188=CARTESIAN_POINT('Ctrl Pts',(16.0067243777368,-17.3539584279855,5.46668692170409));
#18189=CARTESIAN_POINT('Ctrl Pts',(16.2498274691176,-17.2696533893205,5.45563329212373));
#18190=CARTESIAN_POINT('Ctrl Pts',(16.6800192677288,-17.0154474103198,5.43377589861552));
#18191=CARTESIAN_POINT('Ctrl Pts',(16.8649176699945,-16.8513113361359,5.42318120261494));
#18192=CARTESIAN_POINT('Ctrl Pts',(17.16350620977,-16.4605606452633,5.4033229083822));
#18193=CARTESIAN_POINT('Ctrl Pts',(17.2738175281523,-16.2372296372666,5.39424976540973));
#18194=CARTESIAN_POINT('Ctrl Pts',(17.4043803380836,-15.756240748363,5.37320913159943));
#18195=CARTESIAN_POINT('Ctrl Pts',(17.4215384742162,-15.5027722235257,5.36212126962054));
#18196=CARTESIAN_POINT('Ctrl Pts',(17.357600920214,-15.0131883429537,5.34070465192272));
#18197=CARTESIAN_POINT('Ctrl Pts',(17.2807387247273,-14.7812092050215,5.33055683311553));
#18198=CARTESIAN_POINT('Ctrl Pts',(17.0392813406235,-14.3496550077741,5.311678696753));
#18199=CARTESIAN_POINT('Ctrl Pts',(16.8735395704595,-14.1560794282237,5.30130708115627));
#18200=CARTESIAN_POINT('Ctrl Pts',(16.4791980485955,-13.847132194246,5.27961051979625));
#18201=CARTESIAN_POINT('Ctrl Pts',(16.2554212933711,-13.7336070322138,5.26864993642719));
#18202=CARTESIAN_POINT('Ctrl Pts',(15.7839087786619,-13.6008853677485,5.24788429127527));
#18203=CARTESIAN_POINT('Ctrl Pts',(15.5413739862863,-13.5802296539214,5.23889046790109));
#18204=CARTESIAN_POINT('Ctrl Pts',(15.0503410554409,-13.6316931270879,5.2191626144982));
#18205=CARTESIAN_POINT('Ctrl Pts',(14.8069898013851,-13.7076603642555,5.20828195016578));
#18206=CARTESIAN_POINT('Ctrl Pts',(14.3699802854607,-13.9467893376302,5.18649604337778));
#18207=CARTESIAN_POINT('Ctrl Pts',(14.1792464667997,-14.1053559943617,5.17580209496627));
#18208=CARTESIAN_POINT('Ctrl Pts',(13.8690687315096,-14.4855658574476,5.15573530887737));
#18209=CARTESIAN_POINT('Ctrl Pts',(13.7522980475817,-14.7034110952668,5.14684640878099));
#18210=CARTESIAN_POINT('Ctrl Pts',(13.6235390607378,-15.1199647574862,5.12862446380201));
#18211=CARTESIAN_POINT('Ctrl Pts',(13.595,-15.3096276017258,5.1203277514555));
#18212=CARTESIAN_POINT('Ctrl Pts',(13.595,-15.5,5.11199999999994));
#18213=CARTESIAN_POINT('Origin',(15.5,-15.5,-1.713));
#18214=CARTESIAN_POINT('',(13.595,-15.5,4.54949999999989));
#18215=CARTESIAN_POINT('',(13.595,-15.5,4.61199999999993));
#18216=CARTESIAN_POINT('',(13.595,-15.5,-1.713));
#18217=CARTESIAN_POINT('Ctrl Pts',(13.595,-15.5,4.54949999999989));
#18218=CARTESIAN_POINT('Ctrl Pts',(13.595,-15.2971397602935,4.55837402623377));
#18219=CARTESIAN_POINT('Ctrl Pts',(13.6274062319185,-15.0952396842029,4.56720605055957));
#18220=CARTESIAN_POINT('Ctrl Pts',(13.7678871857877,-14.6703239363409,4.58579379106097));
#18221=CARTESIAN_POINT('Ctrl Pts',(13.8882844780646,-14.4555148301993,4.59462055989613));
#18222=CARTESIAN_POINT('Ctrl Pts',(14.2050042984144,-14.0813297617617,4.61480340961284));
#18223=CARTESIAN_POINT('Ctrl Pts',(14.3989873176053,-13.926024873821,4.62554910805958));
#18224=CARTESIAN_POINT('Ctrl Pts',(14.8407918880583,-13.6949572788758,4.64734034948534));
#18225=CARTESIAN_POINT('Ctrl Pts',(15.0855091254695,-13.6235798401537,4.65817237326937));
#18226=CARTESIAN_POINT('Ctrl Pts',(15.5772351323095,-13.5813592039928,4.67772432128798));
#18227=CARTESIAN_POINT('Ctrl Pts',(15.8191778495975,-13.606514183194,4.68684353533109));
#18228=CARTESIAN_POINT('Ctrl Pts',(16.2884411473533,-13.7480307581005,4.70771633604734));
#18229=CARTESIAN_POINT('Ctrl Pts',(16.5104570271441,-13.8659837151826,4.71870705654094));
#18230=CARTESIAN_POINT('Ctrl Pts',(16.9007548492801,-14.1840692972141,4.7404503032613));
#18231=CARTESIAN_POINT('Ctrl Pts',(17.0637885719494,-14.3827202135971,4.75062511870481));
#18232=CARTESIAN_POINT('Ctrl Pts',(17.2967139942101,-14.8219362333497,4.76983841790658));
#18233=CARTESIAN_POINT('Ctrl Pts',(17.3684012078891,-15.0561463292249,4.78008382892474));
#18234=CARTESIAN_POINT('Ctrl Pts',(17.4210143756365,-15.5482282622774,4.80160972275907));
#18235=CARTESIAN_POINT('Ctrl Pts',(17.3977682372132,-15.8018378108878,4.8127037537569));
#18236=CARTESIAN_POINT('Ctrl Pts',(17.2557713716644,-16.2788072810669,4.83356855997647));
#18237=CARTESIAN_POINT('Ctrl Pts',(17.1409407810477,-16.4982903817682,4.84250300911577));
#18238=CARTESIAN_POINT('Ctrl Pts',(16.8342535452258,-16.8816925438905,4.86250738436947));
#18239=CARTESIAN_POINT('Ctrl Pts',(16.6452670974676,-17.041964810415,4.87317244114951));
#18240=CARTESIAN_POINT('Ctrl Pts',(16.2108643087021,-17.2853350570797,4.89495236126665));
#18241=CARTESIAN_POINT('Ctrl Pts',(15.9682744977844,-17.3637292576169,4.90585726236999));
#18242=CARTESIAN_POINT('Ctrl Pts',(15.4776352951499,-17.4201030864084,4.92567760042641));
#18243=CARTESIAN_POINT('Ctrl Pts',(15.2347723103959,-17.4018304096479,4.93461717900942));
#18244=CARTESIAN_POINT('Ctrl Pts',(14.7620931614237,-17.2737469265487,4.95532557325259));
#18245=CARTESIAN_POINT('Ctrl Pts',(14.5374226942709,-17.1625655212275,4.96626875062334));
#18246=CARTESIAN_POINT('Ctrl Pts',(14.1401795508119,-16.8577962651154,4.98798385481279));
#18247=CARTESIAN_POINT('Ctrl Pts',(13.9724990658054,-16.6659342866535,4.99849675036491));
#18248=CARTESIAN_POINT('Ctrl Pts',(13.7267972620337,-16.2371057275703,5.01725565496171));
#18249=CARTESIAN_POINT('Ctrl Pts',(13.6476132850042,-16.006173713243,5.02735766783692));
#18250=CARTESIAN_POINT('Ctrl Pts',(13.6012386706273,-15.6781123337951,5.04170855932633));
#18251=CARTESIAN_POINT('Ctrl Pts',(13.595,-15.5890130318589,5.04560616658524));
#18252=CARTESIAN_POINT('Ctrl Pts',(13.595,-15.5,5.04949999999989));
#18253=CARTESIAN_POINT('Ctrl Pts',(13.595,-15.5,5.11199999999994));
#18254=CARTESIAN_POINT('Ctrl Pts',(13.595,-15.5611707631063,5.10932411359984));
#18255=CARTESIAN_POINT('Ctrl Pts',(13.5979462709872,-15.6224147859416,5.10664502248724));
#18256=CARTESIAN_POINT('Ctrl Pts',(13.6272636334491,-15.9253242853065,5.09339438821931));
#18257=CARTESIAN_POINT('Ctrl Pts',(13.6967086552716,-16.1604577698354,5.08310858399669));
#18258=CARTESIAN_POINT('Ctrl Pts',(13.9250484322185,-16.6012699913425,5.06382545969629));
#18259=CARTESIAN_POINT('Ctrl Pts',(14.0853910786963,-16.8008393480576,5.05380523133158));
#18260=CARTESIAN_POINT('Ctrl Pts',(14.4715898770798,-17.1228186274331,5.0321321075346));
#18261=CARTESIAN_POINT('Ctrl Pts',(14.6925459349015,-17.2433266240215,5.02112565270137));
#18262=CARTESIAN_POINT('Ctrl Pts',(15.1604831200914,-17.3899398186166,5.00019161564768));
#18263=CARTESIAN_POINT('Ctrl Pts',(15.4021006853459,-17.4176916792359,4.99098640127391));
#18264=CARTESIAN_POINT('Ctrl Pts',(15.894197495309,-17.3807866060864,4.97153666920373));
#18265=CARTESIAN_POINT('Ctrl Pts',(16.1396601805575,-17.3120604793286,4.96073439516675));
#18266=CARTESIAN_POINT('Ctrl Pts',(16.5841552313493,-17.0856734720978,4.938943602977));
#18267=CARTESIAN_POINT('Ctrl Pts',(16.7799825417739,-16.9322741671381,4.92816971504776));
#18268=CARTESIAN_POINT('Ctrl Pts',(17.1004482091901,-16.5615636385129,4.90792095418443));
#18269=CARTESIAN_POINT('Ctrl Pts',(17.2229176548675,-16.348473177732,4.89911606201802));
#18270=CARTESIAN_POINT('Ctrl Pts',(17.3841085989977,-15.8785374579043,4.87855894391533));
#18271=CARTESIAN_POINT('Ctrl Pts',(17.417685068939,-15.6250119572512,4.86746858955605));
#18272=CARTESIAN_POINT('Ctrl Pts',(17.3843966400302,-15.1292914917116,4.84578352982115));
#18273=CARTESIAN_POINT('Ctrl Pts',(17.3215954113712,-14.8915711092175,4.83538456295789));
#18274=CARTESIAN_POINT('Ctrl Pts',(17.1066720877883,-14.4461610901709,4.8159003101562));
#18275=CARTESIAN_POINT('Ctrl Pts',(16.9540693082927,-14.2439448462617,4.80627967554572));
#18276=CARTESIAN_POINT('Ctrl Pts',(16.5798512566287,-13.9108227723273,4.78481671070483));
#18277=CARTESIAN_POINT('Ctrl Pts',(16.3621361692523,-13.7829433415911,4.7737718064256));
#18278=CARTESIAN_POINT('Ctrl Pts',(15.8981495645829,-13.6215234816301,4.75266357735125));
#18279=CARTESIAN_POINT('Ctrl Pts',(15.6574035720047,-13.5862627923587,4.74315415992228));
#18280=CARTESIAN_POINT('Ctrl Pts',(15.164350304509,-13.6078922913303,4.72400230495482));
#18281=CARTESIAN_POINT('Ctrl Pts',(14.9169102804823,-13.6689580320699,4.71329267166129));
#18282=CARTESIAN_POINT('Ctrl Pts',(14.4649631449192,-13.8817241688144,4.69151748491861));
#18283=CARTESIAN_POINT('Ctrl Pts',(14.2639391179947,-14.0295304408853,4.68066905752914));
#18284=CARTESIAN_POINT('Ctrl Pts',(13.932772664396,-14.3902181328522,4.66023413155884));
#18285=CARTESIAN_POINT('Ctrl Pts',(13.8043992661642,-14.5984718038406,4.65143692896586));
#18286=CARTESIAN_POINT('Ctrl Pts',(13.6367795651532,-15.0410028370471,4.63207861605219));
#18287=CARTESIAN_POINT('Ctrl Pts',(13.595,-15.2696606056661,4.62207608899091));
#18288=CARTESIAN_POINT('Ctrl Pts',(13.595,-15.5,4.61199999999993));
#18289=CARTESIAN_POINT('Origin',(15.5,-15.5,-1.713));
#18290=CARTESIAN_POINT('',(13.595,-15.5,4.04949999999988));
#18291=CARTESIAN_POINT('',(13.595,-15.5,4.11199999999992));
#18292=CARTESIAN_POINT('',(13.595,-15.5,-1.713));
#18293=CARTESIAN_POINT('Ctrl Pts',(13.595,-15.5,4.04949999999988));
#18294=CARTESIAN_POINT('Ctrl Pts',(13.595,-15.2566554804107,4.0601449921079));
#18295=CARTESIAN_POINT('Ctrl Pts',(13.6416291796205,-15.0154257502269,4.07069747374311));
#18296=CARTESIAN_POINT('Ctrl Pts',(13.8227217236572,-14.5649657826882,4.09040263417788));
#18297=CARTESIAN_POINT('Ctrl Pts',(13.9548797991019,-14.3597546423013,4.09923794107462));
#18298=CARTESIAN_POINT('Ctrl Pts',(14.292909829855,-14.0055782155994,4.11979046982463));
#18299=CARTESIAN_POINT('Ctrl Pts',(14.49720746026,-13.8614754836012,4.1306819091887));
#18300=CARTESIAN_POINT('Ctrl Pts',(14.9537450464085,-13.6576375985826,4.15243571889545));
#18301=CARTESIAN_POINT('Ctrl Pts',(15.2023316701596,-13.6015499101801,4.16307990854595));
#18302=CARTESIAN_POINT('Ctrl Pts',(15.6959198510094,-13.5897930012685,4.18203609218897));
#18303=CARTESIAN_POINT('Ctrl Pts',(15.9361519808382,-13.6299495035781,4.19178755236659));
#18304=CARTESIAN_POINT('Ctrl Pts',(16.3974688465401,-13.8010675464048,4.21300676261618));
#18305=CARTESIAN_POINT('Ctrl Pts',(16.6129323732134,-13.9337286843887,4.22407095582179));
#18306=CARTESIAN_POINT('Ctrl Pts',(16.9792499981077,-14.2740155925913,4.24539133303587));
#18307=CARTESIAN_POINT('Ctrl Pts',(17.1268460120532,-14.4779549496283,4.25479111765629));
#18308=CARTESIAN_POINT('Ctrl Pts',(17.3329037707492,-14.9263449102112,4.27440572660567));
#18309=CARTESIAN_POINT('Ctrl Pts',(17.3912499783115,-15.165678119567,4.28487524582508));
#18310=CARTESIAN_POINT('Ctrl Pts',(17.4149050488048,-15.6629241163841,4.30662703921166));
#18311=CARTESIAN_POINT('Ctrl Pts',(17.3762059499559,-15.9162576936056,4.31770899797026));
#18312=CARTESIAN_POINT('Ctrl Pts',(17.2055762083363,-16.3826095479846,4.3381093415564));
#18313=CARTESIAN_POINT('Ctrl Pts',(17.0793192680661,-16.5925849475532,4.34689990669029));
#18314=CARTESIAN_POINT('Ctrl Pts',(16.7519910378125,-16.9568853337845,4.3672684436934));
#18315=CARTESIAN_POINT('Ctrl Pts',(16.5528184484167,-17.1067232510974,4.37809116813831));
#18316=CARTESIAN_POINT('Ctrl Pts',(16.1035037812404,-17.3244174572891,4.39987441482088));
#18317=CARTESIAN_POINT('Ctrl Pts',(15.8567467722634,-17.3882454163308,4.41061858883035));
#18318=CARTESIAN_POINT('Ctrl Pts',(15.3640192511005,-17.4153701521319,4.42987829654564));
#18319=CARTESIAN_POINT('Ctrl Pts',(15.1229704593036,-17.3828192570121,4.43926848345183));
#18320=CARTESIAN_POINT('Ctrl Pts',(14.6575381615535,-17.2267535835976,4.46031437279132));
#18321=CARTESIAN_POINT('Ctrl Pts',(14.4386234773176,-17.1015303353839,4.47134662571857));
#18322=CARTESIAN_POINT('Ctrl Pts',(14.0600612599842,-16.7724088007001,4.49288666353421));
#18323=CARTESIAN_POINT('Ctrl Pts',(13.9046731226827,-16.5711467140639,4.50264318836092));
#18324=CARTESIAN_POINT('Ctrl Pts',(13.6848819544518,-16.1273925403157,4.52205500698508));
#18325=CARTESIAN_POINT('Ctrl Pts',(13.6196561257824,-15.8905906989304,4.53241379269747));
#18326=CARTESIAN_POINT('Ctrl Pts',(13.5969136295473,-15.5986541054857,4.54518442233197));
#18327=CARTESIAN_POINT('Ctrl Pts',(13.595,-15.5492987001803,4.54734345143557));
#18328=CARTESIAN_POINT('Ctrl Pts',(13.595,-15.5,4.54949999999988));
#18329=CARTESIAN_POINT('Ctrl Pts',(13.595,-15.5,4.61199999999993));
#18330=CARTESIAN_POINT('Ctrl Pts',(13.595,-15.5232640386944,4.61098232551636));
#18331=CARTESIAN_POINT('Ctrl Pts',(13.5954261508269,-15.5465452312985,4.60996390064311));
#18332=CARTESIAN_POINT('Ctrl Pts',(13.6052367897315,-15.8139970169025,4.59826434746708));
#18333=CARTESIAN_POINT('Ctrl Pts',(13.6610845605679,-16.0541929504136,4.5877570887833));
#18334=CARTESIAN_POINT('Ctrl Pts',(13.8622121225949,-16.5042202298844,4.56807085608553));
#18335=CARTESIAN_POINT('Ctrl Pts',(14.0070602801722,-16.7091112186004,4.55877900762857));
#18336=CARTESIAN_POINT('Ctrl Pts',(14.3689922543407,-17.0533161570304,4.53753907966327));
#18337=CARTESIAN_POINT('Ctrl Pts',(14.5831675755589,-17.188604275571,4.52646623065589));
#18338=CARTESIAN_POINT('Ctrl Pts',(15.0429789041739,-17.3650856346105,4.50518674810786));
#18339=CARTESIAN_POINT('Ctrl Pts',(15.2829454294141,-17.4079441568564,4.49528726380417));
#18340=CARTESIAN_POINT('Ctrl Pts',(15.7768001897292,-17.4016027587752,4.47643943059099));
#18341=CARTESIAN_POINT('Ctrl Pts',(16.025971640107,-17.3482529436014,4.46583296893254));
#18342=CARTESIAN_POINT('Ctrl Pts',(16.484950380057,-17.1493510893542,4.44409464103588));
#18343=CARTESIAN_POINT('Ctrl Pts',(16.6910142239839,-17.0073082566105,4.43318134532223));
#18344=CARTESIAN_POINT('Ctrl Pts',(17.0327916159658,-16.656715134371,4.4125652269926));
#18345=CARTESIAN_POINT('Ctrl Pts',(17.1670173530641,-16.453145959696,4.40369492387121));
#18346=CARTESIAN_POINT('Ctrl Pts',(17.3572681428002,-15.9945022723093,4.38363177044223));
#18347=CARTESIAN_POINT('Ctrl Pts',(17.4066852004337,-15.7418916985545,4.37258143913187));
#18348=CARTESIAN_POINT('Ctrl Pts',(17.4032935450824,-15.2420497972705,4.35071608911945));
#18349=CARTESIAN_POINT('Ctrl Pts',(17.3543721336288,-14.9996155181024,4.3401109150526));
#18350=CARTESIAN_POINT('Ctrl Pts',(17.1667709809438,-14.5451685249118,4.32023134404688));
#18351=CARTESIAN_POINT('Ctrl Pts',(17.0293310383393,-14.3376828194855,4.31118114347071));
#18352=CARTESIAN_POINT('Ctrl Pts',(16.6793953047937,-13.9829651227589,4.29016574175129));
#18353=CARTESIAN_POINT('Ctrl Pts',(16.468880140008,-13.840592555518,4.27907660070989));
#18354=CARTESIAN_POINT('Ctrl Pts',(16.0134108536659,-13.6495638134254,4.25764342732135));
#18355=CARTESIAN_POINT('Ctrl Pts',(15.7741670261507,-13.5993262037908,4.24748113348303));
#18356=CARTESIAN_POINT('Ctrl Pts',(15.279635668209,-13.591040510831,4.22856514199461));
#18357=CARTESIAN_POINT('Ctrl Pts',(15.0289634893632,-13.6369750738018,4.21823722129387));
#18358=CARTESIAN_POINT('Ctrl Pts',(14.5635507617894,-13.8225308635711,4.1965470576802));
#18359=CARTESIAN_POINT('Ctrl Pts',(14.3528429333689,-13.9589370809773,4.18558111538397));
#18360=CARTESIAN_POINT('Ctrl Pts',(14.0010471827939,-14.2998483865189,4.16479722607023));
#18361=CARTESIAN_POINT('Ctrl Pts',(13.8612826681553,-14.499091586802,4.15578427004365));
#18362=CARTESIAN_POINT('Ctrl Pts',(13.6589153177444,-14.9493916272471,4.13608610554475));
#18363=CARTESIAN_POINT('Ctrl Pts',(13.6022372644996,-15.1979412367233,4.12521341921595));
#18364=CARTESIAN_POINT('Ctrl Pts',(13.5952160880688,-15.4668590274496,4.11344973633204));
#18365=CARTESIAN_POINT('Ctrl Pts',(13.595,-15.4834339841796,4.11272467260799));
#18366=CARTESIAN_POINT('Ctrl Pts',(13.595,-15.5,4.11199999999992));
#18367=CARTESIAN_POINT('Origin',(15.5,-15.5,-1.713));
#18368=CARTESIAN_POINT('',(13.595,-15.5,3.54949999999988));
#18369=CARTESIAN_POINT('',(13.595,-15.5,3.61199999999992));
#18370=CARTESIAN_POINT('',(13.595,-15.5,-1.713));
#18371=CARTESIAN_POINT('Ctrl Pts',(13.595,-15.5,3.54949999999987));
#18372=CARTESIAN_POINT('Ctrl Pts',(13.595,-15.4714306338019,3.55074975355185));
#18373=CARTESIAN_POINT('Ctrl Pts',(13.5956426779202,-15.4428377365097,3.55200053646039));
#18374=CARTESIAN_POINT('Ctrl Pts',(13.6082936904735,-15.1620947970368,3.56428150494126));
#18375=CARTESIAN_POINT('Ctrl Pts',(13.6696572782828,-14.9146802469339,3.57510453862906));
#18376=CARTESIAN_POINT('Ctrl Pts',(13.880426471005,-14.4684377853199,3.59462520624122));
#18377=CARTESIAN_POINT('Ctrl Pts',(14.0238215350029,-14.2719721542518,3.60376972316979));
#18378=CARTESIAN_POINT('Ctrl Pts',(14.3821595775149,-13.9374669693537,3.62466134348506));
#18379=CARTESIAN_POINT('Ctrl Pts',(14.5958353841015,-13.8048421102622,3.6356570174231));
#18380=CARTESIAN_POINT('Ctrl Pts',(15.0668629636705,-13.6275606276633,3.65737891554599));
#18381=CARTESIAN_POINT('Ctrl Pts',(15.3202477975265,-13.5865505315346,3.66750548084134));
#18382=CARTESIAN_POINT('Ctrl Pts',(15.816805451799,-13.6058985466812,3.68674019434164));
#18383=CARTESIAN_POINT('Ctrl Pts',(16.0553852487261,-13.6616553849759,3.69699805016475));
#18384=CARTESIAN_POINT('Ctrl Pts',(16.5073683092457,-13.8635796722318,3.71853746206844));
#18385=CARTESIAN_POINT('Ctrl Pts',(16.714984071283,-14.0112137363233,3.72963184335436));
#18386=CARTESIAN_POINT('Ctrl Pts',(17.05584097305,-14.373699760751,3.75047321466667));
#18387=CARTESIAN_POINT('Ctrl Pts',(17.187772715427,-14.5831502941422,3.75939283876362));
#18388=CARTESIAN_POINT('Ctrl Pts',(17.3650890119976,-15.0408869006376,3.77941631236359));
#18389=CARTESIAN_POINT('Ctrl Pts',(17.4086793510686,-15.2848939598667,3.79009028695804));
#18390=CARTESIAN_POINT('Ctrl Pts',(17.4007248859629,-15.7828299846122,3.81187226529337));
#18391=CARTESIAN_POINT('Ctrl Pts',(17.3465633227248,-16.0319496742149,3.82276988951046));
#18392=CARTESIAN_POINT('Ctrl Pts',(17.1487063266573,-16.4843991573608,3.84256208037425));
#18393=CARTESIAN_POINT('Ctrl Pts',(17.0108715057099,-16.6851374249942,3.85151730562961));
#18394=CARTESIAN_POINT('Ctrl Pts',(16.6625618840933,-17.0294349516063,3.87224319119429));
#18395=CARTESIAN_POINT('Ctrl Pts',(16.4534568032229,-17.1678238226488,3.88319178032881));
#18396=CARTESIAN_POINT('Ctrl Pts',(15.990232707778,-17.3580628314253,3.90490146268614));
#18397=CARTESIAN_POINT('Ctrl Pts',(15.7400758586494,-17.406575753888,3.91537053064848));
#18398=CARTESIAN_POINT('Ctrl Pts',(15.2457706807686,-17.4034117022829,3.93416593165765));
#18399=CARTESIAN_POINT('Ctrl Pts',(15.0062602511874,-17.3557492987601,3.94428199982258));
#18400=CARTESIAN_POINT('Ctrl Pts',(14.5492523840756,-17.1698208151633,3.9656619064038));
#18401=CARTESIAN_POINT('Ctrl Pts',(14.3374287724992,-17.0299202761496,3.97674654762224));
#18402=CARTESIAN_POINT('Ctrl Pts',(13.9832783004022,-16.6788629497716,3.99784155938021));
#18403=CARTESIAN_POINT('Ctrl Pts',(13.8432530482872,-16.4722882519258,4.0069677055148));
#18404=CARTESIAN_POINT('Ctrl Pts',(13.650892065042,-16.0193844357471,4.02677977096443));
#18405=CARTESIAN_POINT('Ctrl Pts',(13.5995218004781,-15.7777160633025,4.03735144080016));
#18406=CARTESIAN_POINT('Ctrl Pts',(13.5950950344528,-15.5219764732979,4.04853864946178));
#18407=CARTESIAN_POINT('Ctrl Pts',(13.595,-15.5109860814884,4.04901941900738));
#18408=CARTESIAN_POINT('Ctrl Pts',(13.595,-15.5,4.04949999999988));
#18409=CARTESIAN_POINT('Ctrl Pts',(13.595,-15.5,4.11199999999992));
#18410=CARTESIAN_POINT('Ctrl Pts',(13.595,-15.7289515329785,4.10198462235432));
#18411=CARTESIAN_POINT('Ctrl Pts',(13.6362767838862,-15.9561952829852,4.09204395087554));
#18412=CARTESIAN_POINT('Ctrl Pts',(13.8031781282484,-16.399850271514,4.07263647106237));
#18413=CARTESIAN_POINT('Ctrl Pts',(13.9326934273677,-16.6101744716854,4.06376028309602));
#18414=CARTESIAN_POINT('Ctrl Pts',(14.2695258573257,-16.9760551325534,4.04299712598332));
#18415=CARTESIAN_POINT('Ctrl Pts',(14.4758216995285,-17.1259934829378,4.031902348414));
#18416=CARTESIAN_POINT('Ctrl Pts',(14.9261854058435,-17.3327070455456,4.01031953161981));
#18417=CARTESIAN_POINT('Ctrl Pts',(15.1644321192768,-17.3908977234114,4.00002106070406));
#18418=CARTESIAN_POINT('Ctrl Pts',(15.6600647053582,-17.4150713967616,3.98071584429264));
#18419=CARTESIAN_POINT('Ctrl Pts',(15.91289423843,-17.3768775258912,3.97074286366531));
#18420=CARTESIAN_POINT('Ctrl Pts',(16.3852486918124,-17.2051526017849,3.9490922329447));
#18421=CARTESIAN_POINT('Ctrl Pts',(16.6006191253838,-17.0747539459622,3.93808105207819));
#18422=CARTESIAN_POINT('Ctrl Pts',(16.9627468340224,-16.7439911348198,3.9171277187157));
#18423=CARTESIAN_POINT('Ctrl Pts',(17.1082515721606,-16.5491183901532,3.90789319292009));
#18424=CARTESIAN_POINT('Ctrl Pts',(17.3238511193209,-16.1052398174181,3.88847593252048));
#18425=CARTESIAN_POINT('Ctrl Pts',(17.3879059803852,-15.8585209725764,3.87768333213371));
#18426=CARTESIAN_POINT('Ctrl Pts',(17.4158038721806,-15.360398937719,3.8558932168731));
#18427=CARTESIAN_POINT('Ctrl Pts',(17.3816850354908,-15.1139096327732,3.84511065760162));
#18428=CARTESIAN_POINT('Ctrl Pts',(17.2224165141855,-14.6505493382599,3.82484117840156));
#18429=CARTESIAN_POINT('Ctrl Pts',(17.0999032647057,-14.4376467115784,3.81604112977348));
#18430=CARTESIAN_POINT('Ctrl Pts',(16.7748696009735,-14.061977534995,3.79551085863747));
#18431=CARTESIAN_POINT('Ctrl Pts',(16.5725626027766,-13.9053845439179,3.78442164186843));
#18432=CARTESIAN_POINT('Ctrl Pts',(16.1272021809119,-13.6847779241333,3.76272449623994));
#18433=CARTESIAN_POINT('Ctrl Pts',(15.8900665879685,-13.6194996239372,3.7523130965143));
#18434=CARTESIAN_POINT('Ctrl Pts',(15.3971856556628,-13.5813381708641,3.73280617897475));
#18435=CARTESIAN_POINT('Ctrl Pts',(15.1459364906506,-13.6114840999463,3.72322615732184));
#18436=CARTESIAN_POINT('Ctrl Pts',(14.6699367047473,-13.7671979148179,3.70178762651588));
#18437=CARTESIAN_POINT('Ctrl Pts',(14.4498038355065,-13.8910577433524,3.6907390450969));
#18438=CARTESIAN_POINT('Ctrl Pts',(14.0767904715835,-14.2109353139354,3.66961140579681));
#18439=CARTESIAN_POINT('Ctrl Pts',(13.9251913483846,-14.401292583377,3.66006244167204));
#18440=CARTESIAN_POINT('Ctrl Pts',(13.6958596666349,-14.8383295596045,3.64094446370933));
#18441=CARTESIAN_POINT('Ctrl Pts',(13.6241715837739,-15.0828985570044,3.63024590739263));
#18442=CARTESIAN_POINT('Ctrl Pts',(13.5974013523169,-15.3894873060977,3.61683432606746));
#18443=CARTESIAN_POINT('Ctrl Pts',(13.595,-15.4447751296727,3.61441578610347));
#18444=CARTESIAN_POINT('Ctrl Pts',(13.595,-15.5,3.61199999999992));
#18445=CARTESIAN_POINT('Origin',(15.5,-15.5,-1.713));
#18446=CARTESIAN_POINT('',(13.595,-15.5,3.04949999999987));
#18447=CARTESIAN_POINT('',(13.595,-15.5,3.11199999999991));
#18448=CARTESIAN_POINT('',(13.595,-15.5,-1.713));
#18449=CARTESIAN_POINT('Ctrl Pts',(13.595,-15.5,3.04949999999986));
#18450=CARTESIAN_POINT('Ctrl Pts',(13.595,-15.4321105957089,3.05246979021382));
#18451=CARTESIAN_POINT('Ctrl Pts',(13.5986290164635,-15.3641437215775,3.05544296930955));
#18452=CARTESIAN_POINT('Ctrl Pts',(13.6328808295919,-15.0455144947905,3.06938125569569));
#18453=CARTESIAN_POINT('Ctrl Pts',(13.7094288974123,-14.8024529166051,3.08001387066443));
#18454=CARTESIAN_POINT('Ctrl Pts',(13.947539576482,-14.3698817602423,3.09893649342746));
#18455=CARTESIAN_POINT('Ctrl Pts',(14.1031156679202,-14.1824041143387,3.10873274825438));
#18456=CARTESIAN_POINT('Ctrl Pts',(14.4831736554388,-13.869683883395,3.12997071796454));
#18457=CARTESIAN_POINT('Ctrl Pts',(14.7063014598291,-13.7501680402349,3.14103774633167));
#18458=CARTESIAN_POINT('Ctrl Pts',(15.1845327630667,-13.6048554585229,3.1623333171254));
#18459=CARTESIAN_POINT('Ctrl Pts',(15.4347763272853,-13.5798893549735,3.17169857042788));
#18460=CARTESIAN_POINT('Ctrl Pts',(15.9257996252396,-13.6272081761908,3.19133540596976));
#18461=CARTESIAN_POINT('Ctrl Pts',(16.1620890876457,-13.6971483687584,3.20181671714098));
#18462=CARTESIAN_POINT('Ctrl Pts',(16.6039237010221,-13.926849213995,3.223579202796));
#18463=CARTESIAN_POINT('Ctrl Pts',(16.8034884338474,-14.0877738251061,3.2346592742694));
#18464=CARTESIAN_POINT('Ctrl Pts',(17.1206937121615,-14.4698128490763,3.25503229881968));
#18465=CARTESIAN_POINT('Ctrl Pts',(17.2386202282881,-14.6844418676755,3.26382379123663));
#18466=CARTESIAN_POINT('Ctrl Pts',(17.3888917629425,-15.1505366019541,3.28421288722432));
#18467=CARTESIAN_POINT('Ctrl Pts',(17.4182411410945,-15.398128473592,3.29504367775966));
#18468=CARTESIAN_POINT('Ctrl Pts',(17.3803891247896,-15.8960433325684,3.31682473020833));
#18469=CARTESIAN_POINT('Ctrl Pts',(17.3114425366699,-16.1414147811316,3.32755838937558));
#18470=CARTESIAN_POINT('Ctrl Pts',(17.0870494462786,-16.5809326899874,3.34678489457488));
#18471=CARTESIAN_POINT('Ctrl Pts',(16.9376592234311,-16.7729119854775,3.35621069918009));
#18472=CARTESIAN_POINT('Ctrl Pts',(16.5685797137467,-17.096747035341,3.37727586787364));
#18473=CARTESIAN_POINT('Ctrl Pts',(16.3501494254049,-17.2229943740628,3.38831216918689));
#18474=CARTESIAN_POINT('Ctrl Pts',(15.875438963893,-17.3845028077707,3.40982859683191));
#18475=CARTESIAN_POINT('Ctrl Pts',(15.6236218003128,-17.4175504251718,3.41954222081694));
#18476=CARTESIAN_POINT('Ctrl Pts',(15.1297300926185,-17.3844660181691,3.43897638394394));
#18477=CARTESIAN_POINT('Ctrl Pts',(14.8921660094684,-17.3217654308467,3.44934763611788));
#18478=CARTESIAN_POINT('Ctrl Pts',(14.4449362538756,-17.1062023062259,3.47100528668579));
#18479=CARTESIAN_POINT('Ctrl Pts',(14.2411534699628,-16.9520199343099,3.48209768623437));
#18480=CARTESIAN_POINT('Ctrl Pts',(13.9118146101572,-16.5798949736209,3.50271353485158));
#18481=CARTESIAN_POINT('Ctrl Pts',(13.7867599790489,-16.3679365738482,3.51153252082878));
#18482=CARTESIAN_POINT('Ctrl Pts',(13.6321534490399,-15.9330658290354,3.53055573801219));
#18483=CARTESIAN_POINT('Ctrl Pts',(13.595,-15.7172130300017,3.53999811767259));
#18484=CARTESIAN_POINT('Ctrl Pts',(13.595,-15.5,3.54949999999988));
#18485=CARTESIAN_POINT('Ctrl Pts',(13.595,-15.5,3.61199999999992));
#18486=CARTESIAN_POINT('Ctrl Pts',(13.595,-15.6912263683259,3.60363489202415));
#18487=CARTESIAN_POINT('Ctrl Pts',(13.6237955742172,-15.8816979151119,3.59530280336343));
#18488=CARTESIAN_POINT('Ctrl Pts',(13.7525672066139,-16.2963954817282,3.57716205241783));
#18489=CARTESIAN_POINT('Ctrl Pts',(13.8679408263096,-16.5120016187347,3.56836062535117));
#18490=CARTESIAN_POINT('Ctrl Pts',(14.1807548240299,-16.8975712486844,3.54807673717706));
#18491=CARTESIAN_POINT('Ctrl Pts',(14.378749169732,-17.0608955312897,3.53700367180145));
#18492=CARTESIAN_POINT('Ctrl Pts',(14.8185361132323,-17.2956523714065,3.51520817375324));
#18493=CARTESIAN_POINT('Ctrl Pts',(15.0543137168578,-17.3681921867867,3.504689394135));
#18494=CARTESIAN_POINT('Ctrl Pts',(15.5442842580433,-17.420605965555,3.4849810028333));
#18495=CARTESIAN_POINT('Ctrl Pts',(15.7939800289263,-17.3984927944794,3.4757205697281));
#18496=CARTESIAN_POINT('Ctrl Pts',(16.2734020976102,-17.2589383174709,3.45450583092146));
#18497=CARTESIAN_POINT('Ctrl Pts',(16.4981534303578,-17.1418589191606,3.44343058757723));
#18498=CARTESIAN_POINT('Ctrl Pts',(16.8821020250365,-16.8331318042905,3.42213256508492));
#18499=CARTESIAN_POINT('Ctrl Pts',(17.039887556192,-16.6472320007423,3.4121851268916));
#18500=CARTESIAN_POINT('Ctrl Pts',(17.2828123298839,-16.2171395290268,3.39337093302828));
#18501=CARTESIAN_POINT('Ctrl Pts',(17.3620167587507,-15.974948381623,3.38277639464667));
#18502=CARTESIAN_POINT('Ctrl Pts',(17.4209499111993,-15.4781318962858,3.36104339003874));
#18503=CARTESIAN_POINT('Ctrl Pts',(17.4017949090046,-15.2285052132451,3.35012358763101));
#18504=CARTESIAN_POINT('Ctrl Pts',(17.2705998510944,-14.756774399514,3.32948794398572));
#18505=CARTESIAN_POINT('Ctrl Pts',(17.1621720414811,-14.5384461715233,3.32060482498444));
#18506=CARTESIAN_POINT('Ctrl Pts',(16.8614197732683,-14.143328147286,3.30056903685509));
#18507=CARTESIAN_POINT('Ctrl Pts',(16.6678535046653,-13.9735260229966,3.28952203912671));
#18508=CARTESIAN_POINT('Ctrl Pts',(16.2339422406164,-13.7250547244282,3.267649168307));
#18509=CARTESIAN_POINT('Ctrl Pts',(15.9997053097084,-13.6454347321454,3.25703389583053));
#18510=CARTESIAN_POINT('Ctrl Pts',(15.5126654428033,-13.5791741921149,3.23713366978456));
#18511=CARTESIAN_POINT('Ctrl Pts',(15.2644104975039,-13.5936329492472,3.22810485701442));
#18512=CARTESIAN_POINT('Ctrl Pts',(14.7819276091953,-13.7176467043136,3.20711407330051));
#18513=CARTESIAN_POINT('Ctrl Pts',(14.5529205606612,-13.8280415224273,3.19602381386336));
#18514=CARTESIAN_POINT('Ctrl Pts',(14.1586389397585,-14.1257757598693,3.17457477542644));
#18515=CARTESIAN_POINT('Ctrl Pts',(13.9948696580682,-14.3073777317988,3.16439851364743));
#18516=CARTESIAN_POINT('Ctrl Pts',(13.7390376698131,-14.7307767400854,3.14544591062588));
#18517=CARTESIAN_POINT('Ctrl Pts',(13.6527198374731,-14.9705690984086,3.13515970698127));
#18518=CARTESIAN_POINT('Ctrl Pts',(13.6018721779538,-15.3130738890647,3.12017699522903));
#18519=CARTESIAN_POINT('Ctrl Pts',(13.595,-15.406576934727,3.11608674826207));
#18520=CARTESIAN_POINT('Ctrl Pts',(13.595,-15.5,3.11199999999991));
#18521=CARTESIAN_POINT('Origin',(15.5,-15.5,-1.713));
#18522=CARTESIAN_POINT('',(13.595,-15.5,2.54949999999986));
#18523=CARTESIAN_POINT('',(13.595,-15.5,2.6119999999999));
#18524=CARTESIAN_POINT('',(13.595,-15.5,-1.713));
#18525=CARTESIAN_POINT('Ctrl Pts',(13.595,-15.5,2.54949999999986));
#18526=CARTESIAN_POINT('Ctrl Pts',(13.595,-15.3940361834186,2.5541353375581));
#18527=CARTESIAN_POINT('Ctrl Pts',(13.6038410612059,-15.288011292421,2.55877334678806));
#18528=CARTESIAN_POINT('Ctrl Pts',(13.6637959758933,-14.9326929260908,2.57431658241056));
#18529=CARTESIAN_POINT('Ctrl Pts',(13.7556513218222,-14.6933434299402,2.58439405147275));
#18530=CARTESIAN_POINT('Ctrl Pts',(14.0218508967873,-14.2739914824746,2.60365090047229));
#18531=CARTESIAN_POINT('Ctrl Pts',(14.1900364862303,-14.0957225603647,2.61392156775413));
#18532=CARTESIAN_POINT('Ctrl Pts',(14.5919478068822,-13.8064400352437,2.63547479068998));
#18533=CARTESIAN_POINT('Ctrl Pts',(14.8240308016903,-13.7011730185504,2.64656942225763));
#18534=CARTESIAN_POINT('Ctrl Pts',(15.3086740652865,-13.5888469871871,2.66738641235951));
#18535=CARTESIAN_POINT('Ctrl Pts',(15.5558872301103,-13.5801080383882,2.67629150394634));
#18536=CARTESIAN_POINT('Ctrl Pts',(16.0406340441411,-13.6568795152485,2.69633475826763));
#18537=CARTESIAN_POINT('Ctrl Pts',(16.2735546088288,-13.7418824267643,2.70701789833068));
#18538=CARTESIAN_POINT('Ctrl Pts',(16.7000523184248,-13.9991266542888,2.72880179880874));
#18539=CARTESIAN_POINT('Ctrl Pts',(16.8881704153838,-14.1711854189613,2.73969175651716));
#18540=CARTESIAN_POINT('Ctrl Pts',(17.1797897502373,-14.5696454767515,2.75945465157896));
#18541=CARTESIAN_POINT('Ctrl Pts',(17.2840108819561,-14.7896704164612,2.76842696484944));
#18542=CARTESIAN_POINT('Ctrl Pts',(17.4065692980086,-15.263878896105,2.78917099283035));
#18543=CARTESIAN_POINT('Ctrl Pts',(17.4210805548441,-15.5142899744512,2.80012510824357));
#18544=CARTESIAN_POINT('Ctrl Pts',(17.3526145046678,-16.0104396109907,2.82182894186297));
#18545=CARTESIAN_POINT('Ctrl Pts',(17.2687722227482,-16.2510780878475,2.83225316559533));
#18546=CARTESIAN_POINT('Ctrl Pts',(17.0174591997819,-16.6768447431001,2.85108635850073));
#18547=CARTESIAN_POINT('Ctrl Pts',(16.8557719537965,-16.8599648202848,2.86121694909931));
#18548=CARTESIAN_POINT('Ctrl Pts',(16.4651080959497,-17.1615752395479,2.88261371352921));
#18549=CARTESIAN_POINT('Ctrl Pts',(16.2375728975395,-17.2743330486224,2.89369989754563));
#18550=CARTESIAN_POINT('Ctrl Pts',(15.7561389183535,-17.4037991586832,2.91477019987504));
#18551=CARTESIAN_POINT('Ctrl Pts',(15.5073852023538,-17.4209364189226,2.92387165431679));
#18552=CARTESIAN_POINT('Ctrl Pts',(15.0193020385475,-17.3595502717834,2.94370479047538));
#18553=CARTESIAN_POINT('Ctrl Pts',(14.7844977321494,-17.2824246763799,2.95428699922258));
#18554=CARTESIAN_POINT('Ctrl Pts',(14.3484663173313,-17.0387757372993,2.97613471364169));
#18555=CARTESIAN_POINT('Ctrl Pts',(14.1533146606275,-16.8712461198078,2.98719206714309));
#18556=CARTESIAN_POINT('Ctrl Pts',(13.8482952604552,-16.4794816922368,3.00731616001192));
#18557=CARTESIAN_POINT('Ctrl Pts',(13.7374206757829,-16.2621233443958,3.01616127102353));
#18558=CARTESIAN_POINT('Ctrl Pts',(13.6202078713138,-15.8572987167627,3.0338701348745));
#18559=CARTESIAN_POINT('Ctrl Pts',(13.595,-15.6789183932981,3.04167329863075));
#18560=CARTESIAN_POINT('Ctrl Pts',(13.595,-15.5,3.04949999999987));
#18561=CARTESIAN_POINT('Ctrl Pts',(13.595,-15.5,3.11199999999991));
#18562=CARTESIAN_POINT('Ctrl Pts',(13.595,-15.6541792241808,3.10525550200425));
#18563=CARTESIAN_POINT('Ctrl Pts',(13.613718234728,-15.8081406136927,3.09852053308432));
#18564=CARTESIAN_POINT('Ctrl Pts',(13.7090394672623,-16.1925812119671,3.08170335905656));
#18565=CARTESIAN_POINT('Ctrl Pts',(13.8110165548982,-16.4135268313214,3.07267100412813));
#18566=CARTESIAN_POINT('Ctrl Pts',(14.0985444841908,-16.8147940837865,3.05300170765842));
#18567=CARTESIAN_POINT('Ctrl Pts',(14.284916456441,-16.9887287487779,3.04213686973113));
#18568=CARTESIAN_POINT('Ctrl Pts',(14.7089980877039,-17.2503705018038,3.02034831581753));
#18569=CARTESIAN_POINT('Ctrl Pts',(14.9412957771862,-17.3377551330109,3.00963667907495));
#18570=CARTESIAN_POINT('Ctrl Pts',(15.425009209639,-17.4191761013693,2.9895308783385));
#18571=CARTESIAN_POINT('Ctrl Pts',(15.6717770752374,-17.4129441093406,2.98066617426629));
#18572=CARTESIAN_POINT('Ctrl Pts',(16.1573332309325,-17.3057573161853,2.95992700705835));
#18573=CARTESIAN_POINT('Ctrl Pts',(16.390733983597,-17.202771203951,2.9488323422645));
#18574=CARTESIAN_POINT('Ctrl Pts',(16.7959446123815,-16.9172652580428,2.92723673109367));
#18575=CARTESIAN_POINT('Ctrl Pts',(16.9660511030679,-16.7404954349544,2.91692608131995));
#18576=CARTESIAN_POINT('Ctrl Pts',(17.2359307593028,-16.3243308173734,2.89759953070515));
#18577=CARTESIAN_POINT('Ctrl Pts',(17.329922430845,-16.086848361495,2.88767140688958));
#18578=CARTESIAN_POINT('Ctrl Pts',(17.419039281697,-15.5924146793421,2.86604263689164));
#18579=CARTESIAN_POINT('Ctrl Pts',(17.4146395404487,-15.3405974098753,2.85502700830604));
#18580=CARTESIAN_POINT('Ctrl Pts',(17.3108147227307,-14.8611790687817,2.83405507737456));
#18581=CARTESIAN_POINT('Ctrl Pts',(17.2155386186557,-14.6374175395723,2.82479128585809));
#18582=CARTESIAN_POINT('Ctrl Pts',(16.9402795018166,-14.2278595428682,2.80540544219412));
#18583=CARTESIAN_POINT('Ctrl Pts',(16.7592354923017,-14.0484317997801,2.79462230208097));
#18584=CARTESIAN_POINT('Ctrl Pts',(16.3426399863644,-13.7737933372308,2.77283308412301));
#18585=CARTESIAN_POINT('Ctrl Pts',(16.1123449290347,-13.679319787484,2.76204226413672));
#18586=CARTESIAN_POINT('Ctrl Pts',(15.6317787700925,-13.5840519387568,2.74175283166924));
#18587=CARTESIAN_POINT('Ctrl Pts',(15.3862782785964,-13.5828955095755,2.73295653304968));
#18588=CARTESIAN_POINT('Ctrl Pts',(14.8981505326115,-13.6748912262251,2.7124522072999));
#18589=CARTESIAN_POINT('Ctrl Pts',(14.6609818552512,-13.7710462848872,2.70136420953493));
#18590=CARTESIAN_POINT('Ctrl Pts',(14.2462245208683,-14.0451812116636,2.67965564210842));
#18591=CARTESIAN_POINT('Ctrl Pts',(14.0705192229696,-14.2174030232141,2.66923236313488));
#18592=CARTESIAN_POINT('Ctrl Pts',(13.7898612961189,-14.6241409731265,2.64970367243574));
#18593=CARTESIAN_POINT('Ctrl Pts',(13.6896766603476,-14.8562213087964,2.64016179751552));
#18594=CARTESIAN_POINT('Ctrl Pts',(13.6090916105792,-15.2324968962277,2.62370179806533));
#18595=CARTESIAN_POINT('Ctrl Pts',(13.595,-15.366223536707,2.61785198877037));
#18596=CARTESIAN_POINT('Ctrl Pts',(13.595,-15.5,2.6119999999999));
#18597=CARTESIAN_POINT('Origin',(15.5,-15.5,-1.713));
#18598=CARTESIAN_POINT('',(13.595,-15.5,2.04949999999985));
#18599=CARTESIAN_POINT('',(13.595,-15.5,2.1119999999999));
#18600=CARTESIAN_POINT('',(13.595,-15.5,-1.713));
#18601=CARTESIAN_POINT('Ctrl Pts',(13.595,-15.5,2.04949999999985));
#18602=CARTESIAN_POINT('Ctrl Pts',(13.595,-15.3526486934652,2.05594581393401));
#18603=CARTESIAN_POINT('Ctrl Pts',(13.6120968804531,-15.2054448958345,2.06238517516013));
#18604=CARTESIAN_POINT('Ctrl Pts',(13.7034856401193,-14.8191904603802,2.07928169464633));
#18605=CARTESIAN_POINT('Ctrl Pts',(13.807683709322,-14.5905944092652,2.08861259389317));
#18606=CARTESIAN_POINT('Ctrl Pts',(14.0954068155114,-14.1901100509355,2.10827216075147));
#18607=CARTESIAN_POINT('Ctrl Pts',(14.2747550927947,-14.0209968668794,2.11876545717668));
#18608=CARTESIAN_POINT('Ctrl Pts',(14.6956659242681,-13.7545647545419,2.14053866491739));
#18609=CARTESIAN_POINT('Ctrl Pts',(14.9352252828671,-13.6630075465578,2.15161666554088));
#18610=CARTESIAN_POINT('Ctrl Pts',(15.4249588273584,-13.5810818633938,2.17196157071134));
#18611=CARTESIAN_POINT('Ctrl Pts',(15.6696588246589,-13.5871236646452,2.18075506056207));
#18612=CARTESIAN_POINT('Ctrl Pts',(16.1480609274808,-13.6916595237858,2.20116522258474));
#18613=CARTESIAN_POINT('Ctrl Pts',(16.3768922992146,-13.7908690686559,2.21200417943249));
#18614=CARTESIAN_POINT('Ctrl Pts',(16.7882374895011,-14.0741124315941,2.23378270375365));
#18615=CARTESIAN_POINT('Ctrl Pts',(16.9656118429198,-14.2571336410767,2.24450542032328));
#18616=CARTESIAN_POINT('Ctrl Pts',(17.232591142638,-14.6721839437799,2.26369772160026));
#18617=CARTESIAN_POINT('Ctrl Pts',(17.32336258372,-14.8978957552497,2.27316123163802));
#18618=CARTESIAN_POINT('Ctrl Pts',(17.4175725023467,-15.379897660735,2.29424617938454));
#18619=CARTESIAN_POINT('Ctrl Pts',(17.416771052051,-15.6322795723552,2.30528650797685));
#18620=CARTESIAN_POINT('Ctrl Pts',(17.3174983539088,-16.1235866145717,2.32677850457425));
#18621=CARTESIAN_POINT('Ctrl Pts',(17.2195060026385,-16.3575766402513,2.33644892562892));
#18622=CARTESIAN_POINT('Ctrl Pts',(16.9426815429992,-16.7676830021745,2.35590606453524));
#18623=CARTESIAN_POINT('Ctrl Pts',(16.7689623850692,-16.9415492968901,2.36629006940178));
#18624=CARTESIAN_POINT('Ctrl Pts',(16.3575795447531,-17.2197813255831,2.38796041081653));
#18625=CARTESIAN_POINT('Ctrl Pts',(16.1217348139336,-17.3183915250379,2.39905195184739));
#18626=CARTESIAN_POINT('Ctrl Pts',(15.6345046479807,-17.4158138950701,2.41964096699268));
#18627=CARTESIAN_POINT('Ctrl Pts',(15.3885595106893,-17.4172936498083,2.42845290769226));
#18628=CARTESIAN_POINT('Ctrl Pts',(14.9068531433475,-17.3269904646265,2.4486769472318));
#18629=CARTESIAN_POINT('Ctrl Pts',(14.6758146573805,-17.235057316894,2.45944036682785));
#18630=CARTESIAN_POINT('Ctrl Pts',(14.2564853609403,-16.9650604282408,2.48123162962728));
#18631=CARTESIAN_POINT('Ctrl Pts',(14.07350939839,-16.7875855524868,2.49204524597581));
#18632=CARTESIAN_POINT('Ctrl Pts',(13.7938372069924,-16.3809882663696,2.51153351655939));
#18633=CARTESIAN_POINT('Ctrl Pts',(13.6961550187377,-16.1582494665765,2.52070518518896));
#18634=CARTESIAN_POINT('Ctrl Pts',(13.6108922085804,-15.7840215340723,2.5370756109328));
#18635=CARTESIAN_POINT('Ctrl Pts',(13.595,-15.6420656569251,2.54328540433385));
#18636=CARTESIAN_POINT('Ctrl Pts',(13.595,-15.5,2.54949999999986));
#18637=CARTESIAN_POINT('Ctrl Pts',(13.595,-15.5,2.6119999999999));
#18638=CARTESIAN_POINT('Ctrl Pts',(13.595,-15.615287445997,2.60695680463695));
#18639=CARTESIAN_POINT('Ctrl Pts',(13.6054654128687,-15.7306118946473,2.6019119906104));
#18640=CARTESIAN_POINT('Ctrl Pts',(13.670049584727,-16.081817780845,2.58654865350639));
#18641=CARTESIAN_POINT('Ctrl Pts',(13.7583532889062,-16.3086177155276,2.57696069284612));
#18642=CARTESIAN_POINT('Ctrl Pts',(14.020789732391,-16.7266478553754,2.55787531678046));
#18643=CARTESIAN_POINT('Ctrl Pts',(14.1961267477515,-16.9116012234265,2.54718752178696));
#18644=CARTESIAN_POINT('Ctrl Pts',(14.6045256721147,-17.1995071556895,2.52541863248213));
#18645=CARTESIAN_POINT('Ctrl Pts',(14.8325163477983,-17.3012976294405,2.51455507369634));
#18646=CARTESIAN_POINT('Ctrl Pts',(15.3097162815879,-17.41089322416,2.49407978661385));
#18647=CARTESIAN_POINT('Ctrl Pts',(15.5539975592879,-17.4195838172506,2.48527334429313));
#18648=CARTESIAN_POINT('Ctrl Pts',(16.0445699132335,-17.3431226694445,2.46501618354009));
#18649=CARTESIAN_POINT('Ctrl Pts',(16.2853900758208,-17.2540823090537,2.45394546793468));
#18650=CARTESIAN_POINT('Ctrl Pts',(16.7095797727962,-16.9918828300599,2.43214062134231));
#18651=CARTESIAN_POINT('Ctrl Pts',(16.8908809222461,-16.8244868770546,2.4216109022845));
#18652=CARTESIAN_POINT('Ctrl Pts',(17.182411929644,-16.4273976284614,2.40188133611241));
#18653=CARTESIAN_POINT('Ctrl Pts',(17.2887599224322,-16.2006598902134,2.39265003894187));
#18654=CARTESIAN_POINT('Ctrl Pts',(17.4092659708329,-15.716244240958,2.37145950310392));
#18655=CARTESIAN_POINT('Ctrl Pts',(17.4211158419616,-15.4630147587218,2.36038209793174));
#18656=CARTESIAN_POINT('Ctrl Pts',(17.3473304857396,-14.9757380640176,2.33906640699979));
#18657=CARTESIAN_POINT('Ctrl Pts',(17.2659610749238,-14.7458062619205,2.32907219089834));
#18658=CARTESIAN_POINT('Ctrl Pts',(17.0163007825848,-14.3195177133891,2.31029019484638));
#18659=CARTESIAN_POINT('Ctrl Pts',(16.8467786602378,-14.1292823167842,2.29970716060499));
#18660=CARTESIAN_POINT('Ctrl Pts',(16.4469056037788,-13.8284931106128,2.27797947782861));
#18661=CARTESIAN_POINT('Ctrl Pts',(16.2214188791038,-13.7195150770427,2.26705357019215));
#18662=CARTESIAN_POINT('Ctrl Pts',(15.7476574275375,-13.5957822729623,2.24639933334043));
#18663=CARTESIAN_POINT('Ctrl Pts',(15.5044765268383,-13.5797520093936,2.23750309629325));
#18664=CARTESIAN_POINT('Ctrl Pts',(15.0116950071339,-13.6410692883709,2.21749347450548));
#18665=CARTESIAN_POINT('Ctrl Pts',(14.7675175251247,-13.7230597672649,2.20644976751076));
#18666=CARTESIAN_POINT('Ctrl Pts',(14.3344695720043,-13.9733447110082,2.18456993372551));
#18667=CARTESIAN_POINT('Ctrl Pts',(14.1478486714339,-14.1358739422802,2.17394512810839));
#18668=CARTESIAN_POINT('Ctrl Pts',(13.8458586534847,-14.5235480647069,2.15402526422184));
#18669=CARTESIAN_POINT('Ctrl Pts',(13.7336458769756,-14.7452548620724,2.14501597278763));
#18670=CARTESIAN_POINT('Ctrl Pts',(13.6190362478944,-15.1510323337707,2.12726542721903));
#18671=CARTESIAN_POINT('Ctrl Pts',(13.595,-15.3252887149695,2.11964266338706));
#18672=CARTESIAN_POINT('Ctrl Pts',(13.595,-15.5,2.1119999999999));
#18673=CARTESIAN_POINT('Origin',(15.5,-15.5,-1.713));
#18674=CARTESIAN_POINT('',(13.595,-15.5,1.54949999999985));
#18675=CARTESIAN_POINT('',(13.595,-15.5,1.61199999999989));
#18676=CARTESIAN_POINT('',(13.595,-15.5,-1.713));
#18677=CARTESIAN_POINT('Ctrl Pts',(13.595,-15.5,1.54949999999985));
#18678=CARTESIAN_POINT('Ctrl Pts',(13.595,-15.3100000278905,1.55781145984716));
#18679=CARTESIAN_POINT('Ctrl Pts',(13.6234274993569,-15.1207028088503,1.5660921780903));
#18680=CARTESIAN_POINT('Ctrl Pts',(13.7518428572065,-14.7044017556307,1.58430307280682));
#18681=CARTESIAN_POINT('Ctrl Pts',(13.8685053079182,-14.4864653856672,1.59319428948728));
#18682=CARTESIAN_POINT('Ctrl Pts',(14.1784881282718,-14.1060768557497,1.61325759929138));
#18683=CARTESIAN_POINT('Ctrl Pts',(14.3691246157502,-13.9474143171397,1.62394995757439));
#18684=CARTESIAN_POINT('Ctrl Pts',(14.8059894395499,-13.7080473986579,1.64573558726254));
#18685=CARTESIAN_POINT('Ctrl Pts',(15.0492987655172,-13.6319442278147,1.65661763637394));
#18686=CARTESIAN_POINT('Ctrl Pts',(15.5403101516429,-13.580206165741,1.67635067946095));
#18687=CARTESIAN_POINT('Ctrl Pts',(15.7828630482455,-13.6007284968042,1.68534124383068));
#18688=CARTESIAN_POINT('Ctrl Pts',(16.2544413111661,-13.7331901706492,1.70610369319571));
#18689=CARTESIAN_POINT('Ctrl Pts',(16.4782688030326,-13.8465841050468,1.71706332841971));
#18690=CARTESIAN_POINT('Ctrl Pts',(16.8727741026647,-14.1552977792804,1.73876098583554));
#18691=CARTESIAN_POINT('Ctrl Pts',(17.0386250139318,-14.3487777596965,1.74914032194625));
#18692=CARTESIAN_POINT('Ctrl Pts',(17.2803211699226,-14.7801802079204,1.76801182011877));
#18693=CARTESIAN_POINT('Ctrl Pts',(17.3573139006528,-15.0121012423612,1.77815709721592));
#18694=CARTESIAN_POINT('Ctrl Pts',(17.4215377922237,-15.5016183964856,1.79957079599651));
#18695=CARTESIAN_POINT('Ctrl Pts',(17.4045339268535,-15.7550815033061,1.81065842096679));
#18696=CARTESIAN_POINT('Ctrl Pts',(17.2742621948363,-16.2361710137032,1.83170345641724));
#18697=CARTESIAN_POINT('Ctrl Pts',(17.1640657129151,-16.4596003404794,1.84078070819265));
#18698=CARTESIAN_POINT('Ctrl Pts',(16.8656822982862,-16.8505361109838,1.86063527960074));
#18699=CARTESIAN_POINT('Ctrl Pts',(16.6808880142321,-17.0147683442417,1.87122813441674));
#18700=CARTESIAN_POINT('Ctrl Pts',(16.2508692359186,-17.2692093625704,1.89308411408813));
#18701=CARTESIAN_POINT('Ctrl Pts',(16.0078314830718,-17.3536533130298,1.90413830670727));
#18702=CARTESIAN_POINT('Ctrl Pts',(15.5157961733657,-17.4202150896715,1.92423436821581));
#18703=CARTESIAN_POINT('Ctrl Pts',(15.2722443557045,-17.4067271094536,1.93309049077355));
#18704=CARTESIAN_POINT('Ctrl Pts',(14.7972739297611,-17.2879096009912,1.95368301960753));
#18705=CARTESIAN_POINT('Ctrl Pts',(14.570890814878,-17.1814260816023,1.96458832530181));
#18706=CARTESIAN_POINT('Ctrl Pts',(14.1680048503673,-16.8850910700194,1.98633272538432));
#18707=CARTESIAN_POINT('Ctrl Pts',(13.9964409246613,-16.6966722393834,1.99695337863682));
#18708=CARTESIAN_POINT('Ctrl Pts',(13.7423247716212,-16.2732439435685,2.01584161975457));
#18709=CARTESIAN_POINT('Ctrl Pts',(13.6585371841348,-16.0444166518227,2.025684748389));
#18710=CARTESIAN_POINT('Ctrl Pts',(13.6032339797595,-15.7045935164027,2.04055015238812));
#18711=CARTESIAN_POINT('Ctrl Pts',(13.595,-15.6022612357987,2.04502663010489));
#18712=CARTESIAN_POINT('Ctrl Pts',(13.595,-15.5,2.04949999999985));
#18713=CARTESIAN_POINT('Ctrl Pts',(13.595,-15.5,2.1119999999999));
#18714=CARTESIAN_POINT('Ctrl Pts',(13.595,-15.5760950455545,2.10867125784966));
#18715=CARTESIAN_POINT('Ctrl Pts',(13.5995592844064,-15.6522763870644,2.10533874072324));
#18716=CARTESIAN_POINT('Ctrl Pts',(13.6377365927073,-15.9687770978132,2.09149356527491));
#18717=CARTESIAN_POINT('Ctrl Pts',(13.7124302046239,-16.201708256264,2.08130410077575));
#18718=CARTESIAN_POINT('Ctrl Pts',(13.9499183283314,-16.6357575783573,2.06231681634471));
#18719=CARTESIAN_POINT('Ctrl Pts',(14.1138443305959,-16.8309084290227,2.05206963293043));
#18720=CARTESIAN_POINT('Ctrl Pts',(14.5054536833703,-17.1437127897055,2.03039221262406));
#18721=CARTESIAN_POINT('Ctrl Pts',(14.7283790660537,-17.2594087386999,2.01941640251692));
#18722=CARTESIAN_POINT('Ctrl Pts',(15.1987964301296,-17.396436622578,1.99859805913941));
#18723=CARTESIAN_POINT('Ctrl Pts',(15.4410363979128,-17.4192983143245,1.9895465063196));
#18724=CARTESIAN_POINT('Ctrl Pts',(15.9324172665455,-17.3723715040461,1.96990469878203));
#18725=CARTESIAN_POINT('Ctrl Pts',(16.1764500136759,-17.2986537031364,1.95904741711863));
#18726=CARTESIAN_POINT('Ctrl Pts',(16.6158314577467,-17.0634689885345,1.93725792237594));
#18727=CARTESIAN_POINT('Ctrl Pts',(16.8081666912994,-16.9064950156484,1.92653814176603));
#18728=CARTESIAN_POINT('Ctrl Pts',(17.1215600504422,-16.5292396737189,1.90641415745458));
#18729=CARTESIAN_POINT('Ctrl Pts',(17.240114711357,-16.3128922721586,1.89755959195784));
#18730=CARTESIAN_POINT('Ctrl Pts',(17.391494001895,-15.8393168702794,1.87684325766741));
#18731=CARTESIAN_POINT('Ctrl Pts',(17.4197738124388,-15.585697583992,1.86574880069946));
#18732=CARTESIAN_POINT('Ctrl Pts',(17.3765599477362,-15.0917486228472,1.84414123459513));
#18733=CARTESIAN_POINT('Ctrl Pts',(17.3091861934115,-14.8557849173145,1.83381911274331));
#18734=CARTESIAN_POINT('Ctrl Pts',(17.0850557933772,-14.4135186118599,1.81447238022123));
#18735=CARTESIAN_POINT('Ctrl Pts',(16.9271628563678,-14.213112801465,1.80458598817505));
#18736=CARTESIAN_POINT('Ctrl Pts',(16.5447253469805,-13.887597868733,1.78297802383317));
#18737=CARTESIAN_POINT('Ctrl Pts',(16.3247639331751,-13.764760137355,1.7719582933915));
#18738=CARTESIAN_POINT('Ctrl Pts',(15.8580547995251,-13.6134845740593,1.75096880312173));
#18739=CARTESIAN_POINT('Ctrl Pts',(15.6167232944308,-13.5833630154329,1.74167645802588));
#18740=CARTESIAN_POINT('Ctrl Pts',(15.1243063238811,-13.6154313613421,1.72232038721637));
#18741=CARTESIAN_POINT('Ctrl Pts',(14.8781909936369,-13.6817382234719,1.71154630325674));
#18742=CARTESIAN_POINT('Ctrl Pts',(14.4312911303674,-13.9038391283785,1.68975815421944));
#18743=CARTESIAN_POINT('Ctrl Pts',(14.233801553833,-14.0554860364106,1.67895962209881));
#18744=CARTESIAN_POINT('Ctrl Pts',(13.9099371458213,-14.4230295546759,1.65865137346135));
#18745=CARTESIAN_POINT('Ctrl Pts',(13.7855910418598,-14.6345714678699,1.64985776605983));
#18746=CARTESIAN_POINT('Ctrl Pts',(13.6318995591178,-15.0683505290783,1.63088230406471));
#18747=CARTESIAN_POINT('Ctrl Pts',(13.595,-15.2835320441008,1.6214692894093));
#18748=CARTESIAN_POINT('Ctrl Pts',(13.595,-15.5,1.61199999999989));
#18749=CARTESIAN_POINT('Origin',(15.5,15.5,-1.713));
#18750=CARTESIAN_POINT('',(13.595,15.5,10.6744999999999));
#18751=CARTESIAN_POINT('',(13.5949999999998,15.5000000000002,10.737));
#18752=CARTESIAN_POINT('',(13.595,15.5,-1.713));
#18753=CARTESIAN_POINT('',(14.1407339385615,16.8346987578533,10.7369999999981));
#18754=CARTESIAN_POINT('Ctrl Pts',(13.595,15.5,10.6744999999999));
#18755=CARTESIAN_POINT('Ctrl Pts',(13.595,15.7209850684948,10.6828717709174));
#18756=CARTESIAN_POINT('Ctrl Pts',(13.6334494343469,15.9405414658973,10.6920303944907));
#18757=CARTESIAN_POINT('Ctrl Pts',(13.7553915464664,16.2771811332396,10.7074507601906));
#18758=CARTESIAN_POINT('Ctrl Pts',(13.8155629219042,16.4001887992413,10.7134268516752));
#18759=CARTESIAN_POINT('Ctrl Pts',(13.9608604619492,16.6307356506883,10.7253388464319));
#18760=CARTESIAN_POINT('Ctrl Pts',(14.0454618665887,16.7376730482912,10.7312404739585));
#18761=CARTESIAN_POINT('Ctrl Pts',(14.1407339385603,16.8346987578544,10.7369999999991));
#18762=CARTESIAN_POINT('Origin',(15.5,15.5,10.737));
#18763=CARTESIAN_POINT('Origin',(15.5,15.5,-1.713));
#18764=CARTESIAN_POINT('',(13.595,15.5,10.1744999999999));
#18765=CARTESIAN_POINT('',(13.595,15.5,10.2370000000001));
#18766=CARTESIAN_POINT('',(13.595,15.5,-1.713));
#18767=CARTESIAN_POINT('Ctrl Pts',(13.595,15.5,10.1744999999999));
#18768=CARTESIAN_POINT('Ctrl Pts',(13.595,15.5074209450671,10.1747811341621));
#18769=CARTESIAN_POINT('Ctrl Pts',(13.5950433625137,15.514843711189,10.1750632857494));
#18770=CARTESIAN_POINT('Ctrl Pts',(13.5980800374719,15.7746106576663,10.1849706834831));
#18771=CARTESIAN_POINT('Ctrl Pts',(13.6511424766741,16.0238416218886,10.1955731141929));
#18772=CARTESIAN_POINT('Ctrl Pts',(13.8495251796916,16.4830731774224,10.21730966471));
#18773=CARTESIAN_POINT('Ctrl Pts',(13.9913508552489,16.6893210098465,10.2282251809013));
#18774=CARTESIAN_POINT('Ctrl Pts',(14.3415677125539,17.0314906605524,10.248847929745));
#18775=CARTESIAN_POINT('Ctrl Pts',(14.5449657800694,17.1659329264404,10.2577224750685));
#18776=CARTESIAN_POINT('Ctrl Pts',(15.0033973280684,17.3567117327104,10.2777763485593));
#18777=CARTESIAN_POINT('Ctrl Pts',(15.2559823434613,17.4064182514367,10.2888255618311));
#18778=CARTESIAN_POINT('Ctrl Pts',(15.7558831752725,17.4035758694502,10.3106934897319));
#18779=CARTESIAN_POINT('Ctrl Pts',(15.998396076538,17.3549109351872,10.3213021030856));
#18780=CARTESIAN_POINT('Ctrl Pts',(16.4530034996812,17.1678069519007,10.3411886920245));
#18781=CARTESIAN_POINT('Ctrl Pts',(16.6605842725638,17.0306357150664,10.3502315276944));
#18782=CARTESIAN_POINT('Ctrl Pts',(17.0156818941415,16.6811397631114,10.3712385786));
#18783=CARTESIAN_POINT('Ctrl Pts',(17.1583113324512,16.4707625120934,10.3823281132857));
#18784=CARTESIAN_POINT('Ctrl Pts',(17.3498707313289,16.0154567071911,10.40376670003));
#18785=CARTESIAN_POINT('Ctrl Pts',(17.4003765835231,15.7762422294572,10.4139337490575));
#18786=CARTESIAN_POINT('Ctrl Pts',(17.4091960808239,15.2816903031459,10.4328621952661));
#18787=CARTESIAN_POINT('Ctrl Pts',(17.3635304005437,15.030965887023,10.4431758642524));
#18788=CARTESIAN_POINT('Ctrl Pts',(17.178463764648,14.5653277698759,10.4648638675931));
#18789=CARTESIAN_POINT('Ctrl Pts',(17.042265077244,14.3544540576283,10.4758315550602));
#18790=CARTESIAN_POINT('Ctrl Pts',(16.7017070840868,14.0022956793364,10.4966214543749));
#18791=CARTESIAN_POINT('Ctrl Pts',(16.5026187900325,13.8623302617467,10.5056409103224));
#18792=CARTESIAN_POINT('Ctrl Pts',(16.0525428529262,13.6594950881445,10.5253292715256));
#18793=CARTESIAN_POINT('Ctrl Pts',(15.8040539415988,13.6025560456482,10.5361993026423));
#18794=CARTESIAN_POINT('Ctrl Pts',(15.3059850971027,13.5890276321658,10.5579870911154));
#18795=CARTESIAN_POINT('Ctrl Pts',(15.0612475636335,13.6299820743873,10.5686930199636));
#18796=CARTESIAN_POINT('Ctrl Pts',(14.6019183707757,13.8022488761935,10.5887861605086));
#18797=CARTESIAN_POINT('Ctrl Pts',(14.3915034254768,13.931514419436,10.5976583521008));
#18798=CARTESIAN_POINT('Ctrl Pts',(14.025272378736,14.2679294749982,10.6184133611866));
#18799=CARTESIAN_POINT('Ctrl Pts',(13.8750960478184,14.4740872298914,10.6295081126469));
#18800=CARTESIAN_POINT('Ctrl Pts',(13.6678872424595,14.9242804268043,10.6510953019652));
#18801=CARTESIAN_POINT('Ctrl Pts',(13.6094446156002,15.1624912483007,10.6613979238507));
#18802=CARTESIAN_POINT('Ctrl Pts',(13.5957842176475,15.4368541821284,10.6720906390531));
#18803=CARTESIAN_POINT('Ctrl Pts',(13.595,15.468441018576,10.6733044234631));
#18804=CARTESIAN_POINT('Ctrl Pts',(13.595,15.5,10.6744999999999));
#18805=CARTESIAN_POINT('Ctrl Pts',(13.595,15.5000000000014,10.7370000000001));
#18806=CARTESIAN_POINT('Ctrl Pts',(13.5949999999998,15.2615050818091,10.7279648881091));
#18807=CARTESIAN_POINT('Ctrl Pts',(13.639785942239,15.0250626381517,10.7180279618685));
#18808=CARTESIAN_POINT('Ctrl Pts',(13.8168676826068,14.574636639808,10.6970909003079));
#18809=CARTESIAN_POINT('Ctrl Pts',(13.9499258686807,14.3657577230364,10.6862674733056));
#18810=CARTESIAN_POINT('Ctrl Pts',(14.2901813294418,14.0076280664949,10.6652579758955));
#18811=CARTESIAN_POINT('Ctrl Pts',(14.4950326130465,13.8626655490992,10.6559618279509));
#18812=CARTESIAN_POINT('Ctrl Pts',(14.9449917262885,13.6613318768111,10.6362785771528));
#18813=CARTESIAN_POINT('Ctrl Pts',(15.1851520886087,13.6053793669476,10.6257728745141));
#18814=CARTESIAN_POINT('Ctrl Pts',(15.68313769875,13.5868855646606,10.6039887270888));
#18815=CARTESIAN_POINT('Ctrl Pts',(15.9363279765729,13.6283219440909,10.5929130368953));
#18816=CARTESIAN_POINT('Ctrl Pts',(16.4007383128052,13.803977489042,10.5725976241117));
#18817=CARTESIAN_POINT('Ctrl Pts',(16.6090638072585,13.9322622441969,10.5638009107335));
#18818=CARTESIAN_POINT('Ctrl Pts',(16.9699032308363,14.2632679249879,10.5433687567462));
#18819=CARTESIAN_POINT('Ctrl Pts',(17.117795172942,14.4642146921968,10.5325213824564));
#18820=CARTESIAN_POINT('Ctrl Pts',(17.330768674431,14.9160524890345,10.5107458023516));
#18821=CARTESIAN_POINT('Ctrl Pts',(17.391950434512,15.1634645000593,10.5000346926933));
#18822=CARTESIAN_POINT('Ctrl Pts',(17.413810480885,15.6565045081774,10.4808782974484));
#18823=CARTESIAN_POINT('Ctrl Pts',(17.3786636876491,15.8972629623921,10.4713741043925));
#18824=CARTESIAN_POINT('Ctrl Pts',(17.2174690866306,16.3613107883679,10.4502684829413));
#18825=CARTESIAN_POINT('Ctrl Pts',(17.0897011795524,16.5790769712636,10.4392240822409));
#18826=CARTESIAN_POINT('Ctrl Pts',(16.7567467648068,16.9534780470537,10.4177578508231));
#18827=CARTESIAN_POINT('Ctrl Pts',(16.5545706118485,17.1061977053063,10.4081316978063));
#18828=CARTESIAN_POINT('Ctrl Pts',(16.1092301033711,17.3213262050678,10.388650485712));
#18829=CARTESIAN_POINT('Ctrl Pts',(15.8715479691291,17.3842299432809,10.3782531920006));
#18830=CARTESIAN_POINT('Ctrl Pts',(15.3758649154132,17.4177404610146,10.3565697688284));
#18831=CARTESIAN_POINT('Ctrl Pts',(15.1223361573197,17.3842822988696,10.345479271974));
#18832=CARTESIAN_POINT('Ctrl Pts',(14.6523183795208,17.2233098897233,10.3249185642837));
#18833=CARTESIAN_POINT('Ctrl Pts',(14.4391556307392,17.1009279013749,10.3161129504634));
#18834=CARTESIAN_POINT('Ctrl Pts',(14.0682979998266,16.7806204218859,10.2958669649115));
#18835=CARTESIAN_POINT('Ctrl Pts',(13.9148176649309,16.5848707484272,10.2850942458631));
#18836=CARTESIAN_POINT('Ctrl Pts',(13.6882320520984,16.1404884866467,10.2633033826038));
#18837=CARTESIAN_POINT('Ctrl Pts',(13.619393625544,15.8950567334125,10.2524998241403));
#18838=CARTESIAN_POINT('Ctrl Pts',(13.5967962139983,15.5955738319869,10.2406599944637));
#18839=CARTESIAN_POINT('Ctrl Pts',(13.595,15.5477624964957,10.2388094284915));
#18840=CARTESIAN_POINT('Ctrl Pts',(13.595,15.5000000000001,10.2370000000001));
#18841=CARTESIAN_POINT('Origin',(15.5,15.5,-1.713));
#18842=CARTESIAN_POINT('',(13.595,15.5,9.6744999999999));
#18843=CARTESIAN_POINT('',(13.595,15.5,9.73700000000006));
#18844=CARTESIAN_POINT('',(13.595,15.5,-1.713));
#18845=CARTESIAN_POINT('Ctrl Pts',(13.595,15.5000000000001,9.6744999999999));
#18846=CARTESIAN_POINT('Ctrl Pts',(13.595,15.5467420728766,9.67627077088952));
#18847=CARTESIAN_POINT('Ctrl Pts',(13.5967202853277,15.5935315793058,9.67808096528403));
#18848=CARTESIAN_POINT('Ctrl Pts',(13.6187597648754,15.8920261509568,9.68987114996099));
#18849=CARTESIAN_POINT('Ctrl Pts',(13.6872020874657,16.1375667551881,9.70067016843079));
#18850=CARTESIAN_POINT('Ctrl Pts',(13.9130870394511,16.582346386742,9.72246076055695));
#18851=CARTESIAN_POINT('Ctrl Pts',(14.0662814409298,16.7783697126165,9.73323759260773));
#18852=CARTESIAN_POINT('Ctrl Pts',(14.4366202357196,17.0992349697923,9.75349336081863));
#18853=CARTESIAN_POINT('Ctrl Pts',(14.6495282078216,17.2219253191499,9.76229650952821));
#18854=CARTESIAN_POINT('Ctrl Pts',(15.1192565164498,17.3836681050642,9.7828445545251));
#18855=CARTESIAN_POINT('Ctrl Pts',(15.3727735533347,17.4175433890708,9.79393453864082));
#18856=CARTESIAN_POINT('Ctrl Pts',(15.8685880727844,17.3848159770126,9.81562371272001));
#18857=CARTESIAN_POINT('Ctrl Pts',(16.1064048590934,17.3222737366833,9.82602689672305));
#18858=CARTESIAN_POINT('Ctrl Pts',(16.5519903024088,17.1078685429527,9.84551882337728));
#18859=CARTESIAN_POINT('Ctrl Pts',(16.7543077408873,16.955560712628,9.8551256043988));
#18860=CARTESIAN_POINT('Ctrl Pts',(17.0878528289383,16.5818048170048,9.87658031325489));
#18861=CARTESIAN_POINT('Ctrl Pts',(17.2160137186657,16.3642189675569,9.8876264776464));
#18862=CARTESIAN_POINT('Ctrl Pts',(17.3780022600017,15.900387077464,9.90874128388326));
#18863=CARTESIAN_POINT('Ctrl Pts',(17.4135504472185,15.6596724374698,9.91826397153366));
#18864=CARTESIAN_POINT('Ctrl Pts',(17.392502729278,15.1665858676451,9.93740436325299));
#18865=CARTESIAN_POINT('Ctrl Pts',(17.3317298104215,14.9190754039315,9.94811026039677));
#18866=CARTESIAN_POINT('Ctrl Pts',(17.1194871886625,14.4668527863303,9.9698844330078));
#18867=CARTESIAN_POINT('Ctrl Pts',(16.9718972706699,14.2656339594174,9.9807355080219));
#18868=CARTESIAN_POINT('Ctrl Pts',(16.6115925344041,13.9340618991594,10.0011774238356));
#18869=CARTESIAN_POINT('Ctrl Pts',(16.403519949665,13.805464868694,10.0099759427094));
#18870=CARTESIAN_POINT('Ctrl Pts',(15.9394099046984,13.6290372471708,10.0302782193921));
#18871=CARTESIAN_POINT('Ctrl Pts',(15.686244186523,13.5871798170603,10.0413528352353));
#18872=CARTESIAN_POINT('Ctrl Pts',(15.1881494751231,13.6048788651152,10.063141755244));
#18873=CARTESIAN_POINT('Ctrl Pts',(14.9478640205276,13.6604623627683,10.0736529299857));
#18874=CARTESIAN_POINT('Ctrl Pts',(14.4976649285535,13.8610700940611,10.0933466785409));
#18875=CARTESIAN_POINT('Ctrl Pts',(14.2926738275613,14.0056300238769,10.1026277657149));
#18876=CARTESIAN_POINT('Ctrl Pts',(13.9480585027388,14.3670999545861,10.1238591657634));
#18877=CARTESIAN_POINT('Ctrl Pts',(13.8124947693485,14.5811379852324,10.1349328419931));
#18878=CARTESIAN_POINT('Ctrl Pts',(13.6381189944803,15.033858197244,10.1558976316625));
#18879=CARTESIAN_POINT('Ctrl Pts',(13.595,15.2659883514768,10.1656347317408));
#18880=CARTESIAN_POINT('Ctrl Pts',(13.595,15.5,10.1744999999999));
#18881=CARTESIAN_POINT('Ctrl Pts',(13.595,15.5000000000001,10.2370000000001));
#18882=CARTESIAN_POINT('Ctrl Pts',(13.595,15.3073914717115,10.2297032424111));
#18883=CARTESIAN_POINT('Ctrl Pts',(13.6242072503768,15.1156254204738,10.2217995723699));
#18884=CARTESIAN_POINT('Ctrl Pts',(13.7563026575638,14.6933503455336,10.2029129299431));
#18885=CARTESIAN_POINT('Ctrl Pts',(13.876702471396,14.4723487585835,10.191907116492));
#18886=CARTESIAN_POINT('Ctrl Pts',(14.1985172362278,14.0859758557941,10.1702309952512));
#18887=CARTESIAN_POINT('Ctrl Pts',(14.3980477346431,13.9255193647073,10.1602043860612));
#18888=CARTESIAN_POINT('Ctrl Pts',(14.8387924057178,13.6969847837616,10.1409242167228));
#18889=CARTESIAN_POINT('Ctrl Pts',(15.0738870635064,13.6274442067412,10.1306401109577));
#18890=CARTESIAN_POINT('Ctrl Pts',(15.56692222814,13.5795131523613,10.1090725184541));
#18891=CARTESIAN_POINT('Ctrl Pts',(15.8205486951867,13.6052689140877,10.0979777473671));
#18892=CARTESIAN_POINT('Ctrl Pts',(16.295833937723,13.7519510936001,10.0771866168975));
#18893=CARTESIAN_POINT('Ctrl Pts',(16.5137486247078,13.8686392930067,10.0682959537461));
#18894=CARTESIAN_POINT('Ctrl Pts',(16.8940946558731,14.1786684817262,10.0482318168726));
#18895=CARTESIAN_POINT('Ctrl Pts',(17.0527343919501,14.3693281260121,10.0375390800631));
#18896=CARTESIAN_POINT('Ctrl Pts',(17.2920447174216,14.8062273800874,10.01575338384));
#18897=CARTESIAN_POINT('Ctrl Pts',(17.3681155553099,15.0495466867222,10.0048716638172));
#18898=CARTESIAN_POINT('Ctrl Pts',(17.4197882995062,15.5405632028496,9.98513985503588));
#18899=CARTESIAN_POINT('Ctrl Pts',(17.3992342413671,15.7831117902299,9.97614851785801));
#18900=CARTESIAN_POINT('Ctrl Pts',(17.2667107289173,16.2546744188013,9.95538530823236));
#18901=CARTESIAN_POINT('Ctrl Pts',(17.153285580449,16.4784898498698,9.9444254471957));
#18902=CARTESIAN_POINT('Ctrl Pts',(16.844516347237,16.8729562072233,9.9227280498636));
#18903=CARTESIAN_POINT('Ctrl Pts',(16.6510136236391,17.0387811643789,9.91235055221528));
#18904=CARTESIAN_POINT('Ctrl Pts',(16.2195750707347,17.2804205377355,9.89347747466042));
#18905=CARTESIAN_POINT('Ctrl Pts',(15.9876402100024,17.3573822248701,9.88333159273864));
#18906=CARTESIAN_POINT('Ctrl Pts',(15.4981071703884,17.4215380171854,9.86191719905476));
#18907=CARTESIAN_POINT('Ctrl Pts',(15.2446427666752,17.4044974603097,9.85082951735254));
#18908=CARTESIAN_POINT('Ctrl Pts',(14.7635771823721,17.2741564925379,9.8297855285379));
#18909=CARTESIAN_POINT('Ctrl Pts',(14.5401712432681,17.1639326964274,9.8207092566462));
#18910=CARTESIAN_POINT('Ctrl Pts',(14.1492794869322,16.8655004954172,9.8008537997105));
#18911=CARTESIAN_POINT('Ctrl Pts',(13.9850701162271,16.6806814457249,9.79026050673195));
#18912=CARTESIAN_POINT('Ctrl Pts',(13.7306849843362,16.2506215088065,9.76840419017609));
#18913=CARTESIAN_POINT('Ctrl Pts',(13.64627406536,16.0075682104305,9.75735013110541));
#18914=CARTESIAN_POINT('Ctrl Pts',(13.6007088250896,15.6703770935448,9.74357940961421));
#18915=CARTESIAN_POINT('Ctrl Pts',(13.595,15.5851515525511,9.74022587085224));
#18916=CARTESIAN_POINT('Ctrl Pts',(13.595,15.5,9.73700000000006));
#18917=CARTESIAN_POINT('Origin',(15.5,15.5,-1.713));
#18918=CARTESIAN_POINT('',(13.595,15.5,9.17449999999989));
#18919=CARTESIAN_POINT('',(13.595,15.5,9.23700000000004));
#18920=CARTESIAN_POINT('',(13.595,15.5,-1.713));
#18921=CARTESIAN_POINT('Ctrl Pts',(13.595,15.5,9.17449999999989));
#18922=CARTESIAN_POINT('Ctrl Pts',(13.595,15.5841182662493,9.17768672596201));
#18923=CARTESIAN_POINT('Ctrl Pts',(13.6005711245743,15.6683109452453,9.18099812408572));
#18924=CARTESIAN_POINT('Ctrl Pts',(13.6454546573156,16.0045874721858,9.1947192868765));
#18925=CARTESIAN_POINT('Ctrl Pts',(13.7294915060449,16.2478164334572,9.20577181897456));
#18926=CARTESIAN_POINT('Ctrl Pts',(13.9832436140053,16.6783417574239,9.22763192052782));
#18927=CARTESIAN_POINT('Ctrl Pts',(14.1471939492586,16.86344093734,9.2382301602327));
#18928=CARTESIAN_POINT('Ctrl Pts',(14.5375874579699,17.1624251842472,9.25809563300211));
#18929=CARTESIAN_POINT('Ctrl Pts',(14.7607289180441,17.2729579775885,9.26716093254761));
#18930=CARTESIAN_POINT('Ctrl Pts',(15.241523528774,17.4040821001499,9.28819306775017));
#18931=CARTESIAN_POINT('Ctrl Pts',(15.4950022472308,17.4215378340722,9.29928137564419));
#18932=CARTESIAN_POINT('Ctrl Pts',(15.9847143678794,17.3581527301986,9.32070360314416));
#18933=CARTESIAN_POINT('Ctrl Pts',(16.2168053712309,17.28154242915,9.33085631545177));
#18934=CARTESIAN_POINT('Ctrl Pts',(16.6486518981535,17.040545852793,9.34974723963913));
#18935=CARTESIAN_POINT('Ctrl Pts',(16.8424117059181,16.8750147420928,9.36010403130906));
#18936=CARTESIAN_POINT('Ctrl Pts',(17.1518091946145,16.4809894807787,9.38179845958465));
#18937=CARTESIAN_POINT('Ctrl Pts',(17.2655874061658,16.2573107967103,9.39276086240461));
#18938=CARTESIAN_POINT('Ctrl Pts',(17.3988105199629,15.7859252111179,9.41353266682281));
#18939=CARTESIAN_POINT('Ctrl Pts',(17.4197234276662,15.5434252388177,9.42253284891444));
#18940=CARTESIAN_POINT('Ctrl Pts',(17.3687893392891,15.0523509285774,9.44225069108431));
#18941=CARTESIAN_POINT('Ctrl Pts',(17.2930842421058,14.8089190591844,9.4531286758427));
#18942=CARTESIAN_POINT('Ctrl Pts',(17.0544142628338,14.3716309506468,9.4749150975576));
#18943=CARTESIAN_POINT('Ctrl Pts',(16.8960326259638,14.1807096144753,9.48561210305558));
#18944=CARTESIAN_POINT('Ctrl Pts',(16.5161672691566,13.8701561909454,9.5056855865382));
#18945=CARTESIAN_POINT('Ctrl Pts',(16.2984975738922,13.7531769261292,9.51457009738001));
#18946=CARTESIAN_POINT('Ctrl Pts',(15.8234778340686,13.6057615265908,9.53534961355776));
#18947=CARTESIAN_POINT('Ctrl Pts',(15.5698508909803,13.5796122840123,9.54644440546888));
#18948=CARTESIAN_POINT('Ctrl Pts',(15.0766703107743,13.6268085008889,9.56801835910867));
#18949=CARTESIAN_POINT('Ctrl Pts',(14.8414388165919,13.696011803256,9.57830845071767));
#18950=CARTESIAN_POINT('Ctrl Pts',(14.4004559035201,13.9238590409404,9.59759904184063));
#18951=CARTESIAN_POINT('Ctrl Pts',(14.2007883583779,14.0839140324855,9.60760321080475));
#18952=CARTESIAN_POINT('Ctrl Pts',(13.878393475411,14.4696726411921,9.62926874870289));
#18953=CARTESIAN_POINT('Ctrl Pts',(13.757612094652,14.6905133848896,9.64027681452144));
#18954=CARTESIAN_POINT('Ctrl Pts',(13.6245198828295,15.1135898960811,9.65921562083584));
#18955=CARTESIAN_POINT('Ctrl Pts',(13.595,15.3063635593616,9.66716430110702));
#18956=CARTESIAN_POINT('Ctrl Pts',(13.595,15.5000000000001,9.6744999999999));
#18957=CARTESIAN_POINT('Ctrl Pts',(13.595,15.5,9.73700000000006));
#18958=CARTESIAN_POINT('Ctrl Pts',(13.595,15.3443757211123,9.73110434912681));
#18959=CARTESIAN_POINT('Ctrl Pts',(13.6140670739429,15.1890304985196,9.72480222987521));
#18960=CARTESIAN_POINT('Ctrl Pts',(13.7121890711489,14.7970217199471,9.70780526752377));
#18961=CARTESIAN_POINT('Ctrl Pts',(13.8187062227913,14.5706504960066,9.69689967669088));
#18962=CARTESIAN_POINT('Ctrl Pts',(14.1151014095004,14.1678047697919,9.6751554848246));
#18963=CARTESIAN_POINT('Ctrl Pts',(14.3035448501051,13.996268204494,9.66453532981459));
#18964=CARTESIAN_POINT('Ctrl Pts',(14.7270117474889,13.7422119691238,9.64564851430658));
#18965=CARTESIAN_POINT('Ctrl Pts',(14.9558538037295,13.6584568971322,9.63580342065923));
#18966=CARTESIAN_POINT('Ctrl Pts',(15.4418092917676,13.5794459199939,9.61454552529446));
#18967=CARTESIAN_POINT('Ctrl Pts',(15.6948672237038,13.5884707586786,9.60347562450985));
#18968=CARTESIAN_POINT('Ctrl Pts',(16.1810763955832,13.7035882433432,9.5822066318642));
#18969=CARTESIAN_POINT('Ctrl Pts',(16.4096474213849,13.807815216395,9.57287713472466));
#18970=CARTESIAN_POINT('Ctrl Pts',(16.8100863417348,14.095589413607,9.55321662617198));
#18971=CARTESIAN_POINT('Ctrl Pts',(16.9791766790479,14.274963944393,9.54272283487236));
#18972=CARTESIAN_POINT('Ctrl Pts',(17.2455523762227,14.6959189485245,9.52094918762759));
#18973=CARTESIAN_POINT('Ctrl Pts',(17.3370759939428,14.9354953543987,9.50987127588242));
#18974=CARTESIAN_POINT('Ctrl Pts',(17.418928531162,15.4252402763329,9.48952753955791));
#18975=CARTESIAN_POINT('Ctrl Pts',(17.4128512668343,15.6699345949103,9.48073394388639));
#18976=CARTESIAN_POINT('Ctrl Pts',(17.3082478230082,16.1483207371468,9.46032290828238));
#18977=CARTESIAN_POINT('Ctrl Pts',(17.2090037796179,16.3771410728329,9.44948361496211));
#18978=CARTESIAN_POINT('Ctrl Pts',(16.9256979682556,16.7884472787197,9.42770520163259));
#18979=CARTESIAN_POINT('Ctrl Pts',(16.7426508099571,16.9657945748251,9.41698294253947));
#18980=CARTESIAN_POINT('Ctrl Pts',(16.3275606187935,17.2327132985125,9.39779206366632));
#18981=CARTESIAN_POINT('Ctrl Pts',(16.1018343834856,17.3234518195672,9.38832696340719));
#18982=CARTESIAN_POINT('Ctrl Pts',(15.6198137161474,17.4175910477827,9.36724119493223));
#18983=CARTESIAN_POINT('Ctrl Pts',(15.3674280476353,17.4167513457427,9.35620070199646));
#18984=CARTESIAN_POINT('Ctrl Pts',(14.8761442854853,17.3174043597842,9.33470972377469));
#18985=CARTESIAN_POINT('Ctrl Pts',(14.6421797559789,17.2193827662245,9.32504107753166));
#18986=CARTESIAN_POINT('Ctrl Pts',(14.2321180998651,16.9425072991653,9.30558298408394));
#18987=CARTESIAN_POINT('Ctrl Pts',(14.0582734913165,16.7687616740425,9.29519845086315));
#18988=CARTESIAN_POINT('Ctrl Pts',(13.7800955960699,16.3573337764091,9.27352758652369));
#18989=CARTESIAN_POINT('Ctrl Pts',(13.6815178799167,16.1214713095999,9.26243608406818));
#18990=CARTESIAN_POINT('Ctrl Pts',(13.6073102174294,15.7500590608669,9.24674245878719));
#18991=CARTESIAN_POINT('Ctrl Pts',(13.595,15.6250436923898,9.24173713972851));
#18992=CARTESIAN_POINT('Ctrl Pts',(13.595,15.5,9.23700000000004));
#18993=CARTESIAN_POINT('Origin',(15.5,15.5,-1.713));
#18994=CARTESIAN_POINT('',(13.595,15.5,8.67449999999988));
#18995=CARTESIAN_POINT('',(13.595,15.5,8.73700000000004));
#18996=CARTESIAN_POINT('',(13.595,15.5,-1.713));
#18997=CARTESIAN_POINT('Ctrl Pts',(13.595,15.5,8.67449999999988));
#18998=CARTESIAN_POINT('Ctrl Pts',(13.595,15.6239845320393,8.67919701462902));
#18999=CARTESIAN_POINT('Ctrl Pts',(13.6071025749427,15.7479460830675,8.68415786938632));
#19000=CARTESIAN_POINT('Ctrl Pts',(13.6804921932185,16.1184792978077,8.699800300972));
#19001=CARTESIAN_POINT('Ctrl Pts',(13.7787009766107,16.3545427883822,8.71089134959139));
#19002=CARTESIAN_POINT('Ctrl Pts',(14.0562639047011,16.7664816532921,8.73256812062653));
#19003=CARTESIAN_POINT('Ctrl Pts',(14.2298620747682,16.9405275247559,8.74295863817442));
#19004=CARTESIAN_POINT('Ctrl Pts',(14.6394162455077,17.2179817661285,8.76242755798135));
#19005=CARTESIAN_POINT('Ctrl Pts',(14.8730916348169,17.3163350292274,8.77207618699962));
#19006=CARTESIAN_POINT('Ctrl Pts',(15.3641109252586,17.4165246373014,8.79355559603034));
#19007=CARTESIAN_POINT('Ctrl Pts',(15.6165388243955,17.4177984219125,8.80459793632506));
#19008=CARTESIAN_POINT('Ctrl Pts',(16.0987721583091,17.3244613816136,8.82569300779987));
#19009=CARTESIAN_POINT('Ctrl Pts',(16.3246621616815,17.2340962369326,8.83517627677367));
#19010=CARTESIAN_POINT('Ctrl Pts',(16.7402045072762,16.9678646173124,8.85435101512362));
#19011=CARTESIAN_POINT('Ctrl Pts',(16.9235456499428,16.7908244365945,8.86506806959983));
#19012=CARTESIAN_POINT('Ctrl Pts',(17.2075592835694,16.3799609992319,8.88684519081839));
#19013=CARTESIAN_POINT('Ctrl Pts',(17.3071944815201,16.1512661741415,8.89768828474744));
#19014=CARTESIAN_POINT('Ctrl Pts',(17.4125643059193,15.6730612014238,8.91810921942767));
#19015=CARTESIAN_POINT('Ctrl Pts',(17.419043547601,15.4284311150773,8.92690414254867));
#19016=CARTESIAN_POINT('Ctrl Pts',(17.3380201613409,14.9385575085308,8.94723461853481));
#19017=CARTESIAN_POINT('Ctrl Pts',(17.2468774984138,14.6987881849774,8.95831150640485));
#19018=CARTESIAN_POINT('Ctrl Pts',(16.9811417597461,14.2773329934121,8.98009010534563));
#19019=CARTESIAN_POINT('Ctrl Pts',(16.8123106690072,14.0976610775107,8.99058949243603));
#19020=CARTESIAN_POINT('Ctrl Pts',(16.4123868281412,13.8093079629692,9.01026066666552));
#19021=CARTESIAN_POINT('Ctrl Pts',(16.1840991925207,13.7047535905898,9.01957440102707));
#19022=CARTESIAN_POINT('Ctrl Pts',(15.6981649699483,13.5888041447591,9.04083136614396));
#19023=CARTESIAN_POINT('Ctrl Pts',(15.4450785930213,13.57934404525,9.05190251124137));
#19024=CARTESIAN_POINT('Ctrl Pts',(14.9589183093013,13.6575501242183,9.07316936529735));
#19025=CARTESIAN_POINT('Ctrl Pts',(14.7299088508642,13.7409368965763,9.08303684340075));
#19026=CARTESIAN_POINT('Ctrl Pts',(14.3060049856638,13.9943144509653,9.1019075053189));
#19027=CARTESIAN_POINT('Ctrl Pts',(14.1172831377335,14.1655409239974,9.11252200223102));
#19028=CARTESIAN_POINT('Ctrl Pts',(13.8202068842977,14.5679303467204,9.13426380402496));
#19029=CARTESIAN_POINT('Ctrl Pts',(13.713308951115,14.7941665723081,9.14517260915209));
#19030=CARTESIAN_POINT('Ctrl Pts',(13.6143140137655,15.1870326885528,9.16222114395649));
#19031=CARTESIAN_POINT('Ctrl Pts',(13.595,15.3433711822066,9.16856629329937));
#19032=CARTESIAN_POINT('Ctrl Pts',(13.595,15.5,9.17449999999989));
#19033=CARTESIAN_POINT('Ctrl Pts',(13.595,15.5,9.23700000000004));
#19034=CARTESIAN_POINT('Ctrl Pts',(13.595,15.3824179949987,9.23254553791084));
#19035=CARTESIAN_POINT('Ctrl Pts',(13.6058849666647,15.2648292060637,9.2278527399341));
#19036=CARTESIAN_POINT('Ctrl Pts',(13.6730917558932,14.9065985535113,9.2128116095693));
#19037=CARTESIAN_POINT('Ctrl Pts',(13.7650585684708,14.6755697303343,9.20204781971074));
#19038=CARTESIAN_POINT('Ctrl Pts',(14.0351170833788,14.2562762872752,9.18025656727049));
#19039=CARTESIAN_POINT('Ctrl Pts',(14.2126179528575,14.0733257609175,9.16944334600184));
#19040=CARTESIAN_POINT('Ctrl Pts',(14.6192545459505,13.7937119274237,9.14995642650917));
#19041=CARTESIAN_POINT('Ctrl Pts',(14.8420067964181,13.6960615850448,9.14078360470611));
#19042=CARTESIAN_POINT('Ctrl Pts',(15.3200515847365,13.587216811041,9.11987175919784));
#19043=CARTESIAN_POINT('Ctrl Pts',(15.5715317297405,13.5801037207342,9.10887087796406));
#19044=CARTESIAN_POINT('Ctrl Pts',(16.0675652845523,13.6638775132778,9.08717212228549));
#19045=CARTESIAN_POINT('Ctrl Pts',(16.3068900679662,13.7557611321738,9.07709668135702));
#19046=CARTESIAN_POINT('Ctrl Pts',(16.7262000522004,14.0220092773353,9.05783891016115));
#19047=CARTESIAN_POINT('Ctrl Pts',(16.9044493669819,14.1902202450991,9.04756771030684));
#19048=CARTESIAN_POINT('Ctrl Pts',(17.1936824006456,14.5921752325474,9.02601391559381));
#19049=CARTESIAN_POINT('Ctrl Pts',(17.2989194857813,14.8242757180613,9.0149192760814));
#19050=CARTESIAN_POINT('Ctrl Pts',(17.4111778468184,15.3089311471049,8.99410330520862));
#19051=CARTESIAN_POINT('Ctrl Pts',(17.4198837561645,15.5561383958149,8.98519880145138));
#19052=CARTESIAN_POINT('Ctrl Pts',(17.3430511693906,16.0408717039469,8.96515472217364));
#19053=CARTESIAN_POINT('Ctrl Pts',(17.2580169539502,16.2737842435358,8.95447120144469));
#19054=CARTESIAN_POINT('Ctrl Pts',(17.0007148280792,16.7002505185199,8.93268722546357));
#19055=CARTESIAN_POINT('Ctrl Pts',(16.8286313095095,16.8883458080266,8.92179759036604));
#19056=CARTESIAN_POINT('Ctrl Pts',(16.4301342785154,17.1799114619574,8.90203592025793));
#19057=CARTESIAN_POINT('Ctrl Pts',(16.2100973155903,17.2841031152121,8.89306287469785));
#19058=CARTESIAN_POINT('Ctrl Pts',(15.73587152622,17.4066006102442,8.87231808951107));
#19059=CARTESIAN_POINT('Ctrl Pts',(15.4854552195119,17.421079061893,8.86136374538563));
#19060=CARTESIAN_POINT('Ctrl Pts',(14.9893112781569,17.3525458909645,8.83966016089943));
#19061=CARTESIAN_POINT('Ctrl Pts',(14.7486837279404,17.2686711336872,8.82923779513071));
#19062=CARTESIAN_POINT('Ctrl Pts',(14.322947778983,17.0172987846112,8.81040302633861));
#19063=CARTESIAN_POINT('Ctrl Pts',(14.1398474340529,16.8555841798672,8.80027183087332));
#19064=CARTESIAN_POINT('Ctrl Pts',(13.8382875093919,16.464872698706,8.77887436671905));
#19065=CARTESIAN_POINT('Ctrl Pts',(13.7255605297403,16.2373180714138,8.76778812097058));
#19066=CARTESIAN_POINT('Ctrl Pts',(13.6168584404567,15.8328625954923,8.75008821889316));
#19067=CARTESIAN_POINT('Ctrl Pts',(13.595,15.6666266500849,8.74331246333868));
#19068=CARTESIAN_POINT('Ctrl Pts',(13.595,15.4999999999999,8.73700000000004));
#19069=CARTESIAN_POINT('Origin',(15.5,15.5,-1.713));
#19070=CARTESIAN_POINT('',(13.595,15.5,8.17449999999987));
#19071=CARTESIAN_POINT('',(13.595,15.5,8.23700000000003));
#19072=CARTESIAN_POINT('',(13.595,15.5,-1.713));
#19073=CARTESIAN_POINT('Ctrl Pts',(13.595,15.4999999999999,8.17449999999987));
#19074=CARTESIAN_POINT('Ctrl Pts',(13.595,15.6655706799604,8.18077245909731));
#19075=CARTESIAN_POINT('Ctrl Pts',(13.6165822658861,15.8307639689365,8.18750267422103));
#19076=CARTESIAN_POINT('Ctrl Pts',(13.7243523871219,16.234417933857,8.20515182770209));
#19077=CARTESIAN_POINT('Ctrl Pts',(13.8367284095049,16.4621933127477,8.21623876014598));
#19078=CARTESIAN_POINT('Ctrl Pts',(14.1377133670211,16.8534461367269,8.23764415663007));
#19079=CARTESIAN_POINT('Ctrl Pts',(14.3205889440629,17.0154718238113,8.24778222091711));
#19080=CARTESIAN_POINT('Ctrl Pts',(14.7459749943083,17.2675188424774,8.26663489573058));
#19081=CARTESIAN_POINT('Ctrl Pts',(14.9864779484859,17.3517629615954,8.27703621821872));
#19082=CARTESIAN_POINT('Ctrl Pts',(15.4825564974726,17.421059699816,8.29873694214642));
#19083=CARTESIAN_POINT('Ctrl Pts',(15.7330319879065,17.4069545259146,8.3096938752363));
#19084=CARTESIAN_POINT('Ctrl Pts',(16.2074545486742,17.28515014628,8.3304472680958));
#19085=CARTESIAN_POINT('Ctrl Pts',(16.4276283590798,17.1812936902314,8.33942874595681));
#19086=CARTESIAN_POINT('Ctrl Pts',(16.8265456288579,16.890338562991,8.35917647852205));
#19087=CARTESIAN_POINT('Ctrl Pts',(16.9989104159136,16.7025028612466,8.37006243140816));
#19088=CARTESIAN_POINT('Ctrl Pts',(17.2568706598939,16.2763945983601,8.39184723903779));
#19089=CARTESIAN_POINT('Ctrl Pts',(17.3422608012701,16.0435736064316,8.4025350764933));
#19090=CARTESIAN_POINT('Ctrl Pts',(17.4197882054961,15.5589940023013,8.42258853009988));
#19091=CARTESIAN_POINT('Ctrl Pts',(17.4114577837839,15.3118539019019,8.43148645707275));
#19092=CARTESIAN_POINT('Ctrl Pts',(17.2999686011362,14.8270604670506,8.45229083246616));
#19093=CARTESIAN_POINT('Ctrl Pts',(17.1950719271862,14.5947614328546,8.46338554820822));
#19094=CARTESIAN_POINT('Ctrl Pts',(16.9064018859139,14.1923105216186,8.48494581651717));
#19095=CARTESIAN_POINT('Ctrl Pts',(16.7283756870393,14.0238112481951,8.49522305845685));
#19096=CARTESIAN_POINT('Ctrl Pts',(16.3095426905112,13.7570112404865,8.514491303543));
#19097=CARTESIAN_POINT('Ctrl Pts',(16.0704985648374,13.664806527007,8.52454380731241));
#19098=CARTESIAN_POINT('Ctrl Pts',(15.5747065379353,13.5802193514064,8.54623199746559));
#19099=CARTESIAN_POINT('Ctrl Pts',(15.323173313475,13.5869204313355,8.55723520063533));
#19100=CARTESIAN_POINT('Ctrl Pts',(14.8449188118345,13.6950026924642,8.57815621995466));
#19101=CARTESIAN_POINT('Ctrl Pts',(14.6220136440858,13.7922913682329,8.58734226249266));
#19102=CARTESIAN_POINT('Ctrl Pts',(14.2149308751917,14.0712423419691,8.60681382916423));
#19103=CARTESIAN_POINT('Ctrl Pts',(14.0371350730656,14.2539037389004,8.61762254793483));
#19104=CARTESIAN_POINT('Ctrl Pts',(13.7663770367188,14.6727893773774,8.63941365127579));
#19105=CARTESIAN_POINT('Ctrl Pts',(13.6740279732215,14.9037081281676,8.65018163185947));
#19106=CARTESIAN_POINT('Ctrl Pts',(13.6060693707565,15.2628498531252,8.66527372103727));
#19107=CARTESIAN_POINT('Ctrl Pts',(13.595,15.3814261510959,8.67000796301933));
#19108=CARTESIAN_POINT('Ctrl Pts',(13.595,15.5,8.67449999999988));
#19109=CARTESIAN_POINT('Ctrl Pts',(13.595,15.4999999999999,8.73700000000004));
#19110=CARTESIAN_POINT('Ctrl Pts',(13.595,15.4206038404396,8.73399216574185));
#19111=CARTESIAN_POINT('Ctrl Pts',(13.5999632283935,15.3411272724663,8.73087272824994));
#19112=CARTESIAN_POINT('Ctrl Pts',(13.6405135877242,15.0190534423791,8.71778439498593));
#19113=CARTESIAN_POINT('Ctrl Pts',(13.7176717851386,14.7842563785789,8.70720174753657));
#19114=CARTESIAN_POINT('Ctrl Pts',(13.9613838186573,14.3482523216224,8.68535368952092));
#19115=CARTESIAN_POINT('Ctrl Pts',(14.1289432061782,14.1531212076419,8.67429646311949));
#19116=CARTESIAN_POINT('Ctrl Pts',(14.520751534431,13.8481574518962,8.65417351806977));
#19117=CARTESIAN_POINT('Ctrl Pts',(14.738122479254,13.7373148446311,8.64532797553569));
#19118=CARTESIAN_POINT('Ctrl Pts',(15.2084251123979,13.6012137520089,8.62475480698168));
#19119=CARTESIAN_POINT('Ctrl Pts',(15.4575681112309,13.5794278792961,8.61385616311321));
#19120=CARTESIAN_POINT('Ctrl Pts',(15.9547523726961,13.632945839073,8.5921070703107));
#19121=CARTESIAN_POINT('Ctrl Pts',(16.1978028064333,13.7095285676326,8.58147494285063));
#19122=CARTESIAN_POINT('Ctrl Pts',(16.6303417949376,13.9477019847125,8.56255372725551));
#19123=CARTESIAN_POINT('Ctrl Pts',(16.8177988743282,14.103306736907,8.5527555734894));
#19124=CARTESIAN_POINT('Ctrl Pts',(17.1304673813216,14.4834153029675,8.53151681898803));
#19125=CARTESIAN_POINT('Ctrl Pts',(17.2499517200763,14.706564354543,8.5204496747679));
#19126=CARTESIAN_POINT('Ctrl Pts',(17.395189508853,15.1848113261174,8.49915514628783));
#19127=CARTESIAN_POINT('Ctrl Pts',(17.4201184911673,15.4350477316951,8.4897913193337));
#19128=CARTESIAN_POINT('Ctrl Pts',(17.3727336093045,15.9260574676149,8.47015355267829));
#19129=CARTESIAN_POINT('Ctrl Pts',(17.3027597345931,16.1623404818524,8.4596717490839));
#19130=CARTESIAN_POINT('Ctrl Pts',(17.0729933111687,16.6041489389338,8.43790881998719));
#19131=CARTESIAN_POINT('Ctrl Pts',(16.9120375361652,16.8036935141921,8.42682883053564));
#19132=CARTESIAN_POINT('Ctrl Pts',(16.5299526739395,17.1208420183918,8.40645695422237));
#19133=CARTESIAN_POINT('Ctrl Pts',(16.3153110648192,17.2387354398894,8.39766540091083));
#19134=CARTESIAN_POINT('Ctrl Pts',(15.8491966228593,17.3889415479785,8.37727544281987));
#19135=CARTESIAN_POINT('Ctrl Pts',(15.6015970664843,17.4182561416708,8.36644431611931));
#19136=CARTESIAN_POINT('Ctrl Pts',(15.1036844451788,17.3803317435638,8.34466336155654));
#19137=CARTESIAN_POINT('Ctrl Pts',(14.8583231569413,17.3113496979315,8.333930146848));
#19138=CARTESIAN_POINT('Ctrl Pts',(14.4188371634068,17.0868927869893,8.3147050377695));
#19139=CARTESIAN_POINT('Ctrl Pts',(14.2268788412801,16.9374741445605,8.30527771422209));
#19140=CARTESIAN_POINT('Ctrl Pts',(13.9030946233503,16.56834393363,8.28421173657838));
#19141=CARTESIAN_POINT('Ctrl Pts',(13.7768778801302,16.3498915663607,8.27317526802272));
#19142=CARTESIAN_POINT('Ctrl Pts',(13.6291678335146,15.9155216662343,8.25348889919258));
#19143=CARTESIAN_POINT('Ctrl Pts',(13.595,15.7083210063564,8.24489200715868));
#19144=CARTESIAN_POINT('Ctrl Pts',(13.595,15.4999999999999,8.23700000000003));
#19145=CARTESIAN_POINT('Origin',(15.5,15.5,-1.713));
#19146=CARTESIAN_POINT('',(13.595,15.5,7.67449999999987));
#19147=CARTESIAN_POINT('',(13.595,15.5000000314704,7.73700000238446));
#19148=CARTESIAN_POINT('',(13.595,15.5,-1.713));
#19149=CARTESIAN_POINT('Ctrl Pts',(13.595,15.4999999999999,7.67449999999987));
#19150=CARTESIAN_POINT('Ctrl Pts',(13.595,15.7072119682429,7.68234999249621));
#19151=CARTESIAN_POINT('Ctrl Pts',(13.6288049256949,15.9133285386797,7.69089787740364));
#19152=CARTESIAN_POINT('Ctrl Pts',(13.7754232237215,16.3469484282891,7.71053195391287));
#19153=CARTESIAN_POINT('Ctrl Pts',(13.9012906536843,16.5656523838065,7.72157031333401));
#19154=CARTESIAN_POINT('Ctrl Pts',(14.2244947448307,16.9353609163451,7.74264551135446));
#19155=CARTESIAN_POINT('Ctrl Pts',(14.4162139638687,17.0851038136441,7.75209028713306));
#19156=CARTESIAN_POINT('Ctrl Pts',(14.8553358061007,17.3102883722132,7.7712994665833));
#19157=CARTESIAN_POINT('Ctrl Pts',(15.1005808635409,17.379674633204,7.78202759683005));
#19158=CARTESIAN_POINT('Ctrl Pts',(15.598467221476,17.4184244187749,7.80380740251403));
#19159=CARTESIAN_POINT('Ctrl Pts',(15.8461540690323,17.3895065864025,7.81464234772649));
#19160=CARTESIAN_POINT('Ctrl Pts',(16.3124930652495,17.2400465688875,7.83504212883837));
#19161=CARTESIAN_POINT('Ctrl Pts',(16.5272782908419,17.1225302803764,7.84383450149611));
#19162=CARTESIAN_POINT('Ctrl Pts',(16.9098853806253,16.8060290372117,7.86419327935274));
#19163=CARTESIAN_POINT('Ctrl Pts',(17.0711961872398,16.6067145422958,7.875272317815));
#19164=CARTESIAN_POINT('Ctrl Pts',(17.3017098565452,16.1652048743794,7.89704027158077));
#19165=CARTESIAN_POINT('Ctrl Pts',(17.3720675968037,15.9289956883797,7.90752767428474));
#19166=CARTESIAN_POINT('Ctrl Pts',(17.4202052599821,15.4381406590471,7.92717604508821));
#19167=CARTESIAN_POINT('Ctrl Pts',(17.3956990415148,15.1879857265255,7.93652374306273));
#19168=CARTESIAN_POINT('Ctrl Pts',(17.2513132939779,14.7095606372835,7.95780638325783));
#19169=CARTESIAN_POINT('Ctrl Pts',(17.1321881203751,14.4861698317101,7.96887483030069));
#19170=CARTESIAN_POINT('Ctrl Pts',(16.8201091168,14.1054851539516,7.99012251637059));
#19171=CARTESIAN_POINT('Ctrl Pts',(16.6328861955586,13.9495538297391,7.99994242364131));
#19172=CARTESIAN_POINT('Ctrl Pts',(16.2007137166297,13.7106660880922,8.0188476064466));
#19173=CARTESIAN_POINT('Ctrl Pts',(15.9577905429681,13.6336887948883,8.02947416697423));
#19174=CARTESIAN_POINT('Ctrl Pts',(15.4606577648512,13.5793570642748,8.05122100766174));
#19175=CARTESIAN_POINT('Ctrl Pts',(15.2114403555342,13.6007481227263,8.06212290658198));
#19176=CARTESIAN_POINT('Ctrl Pts',(14.7409222498438,13.7361122958494,8.08270550088162));
#19177=CARTESIAN_POINT('Ctrl Pts',(14.5234077996986,13.8465909841975,8.09155607566125));
#19178=CARTESIAN_POINT('Ctrl Pts',(14.1310999921285,14.1509212443981,8.11166594618874));
#19179=CARTESIAN_POINT('Ctrl Pts',(13.9632019341827,14.3458182397711,8.12272171075946));
#19180=CARTESIAN_POINT('Ctrl Pts',(13.7187719777927,14.7815102938362,8.1445736514962));
#19181=CARTESIAN_POINT('Ctrl Pts',(13.6412427536576,15.0162246109299,8.1551612793747));
#19182=CARTESIAN_POINT('Ctrl Pts',(13.6000829545093,15.3392233658662,8.1682979822067));
#19183=CARTESIAN_POINT('Ctrl Pts',(13.595,15.4196518696993,8.17145610140027));
#19184=CARTESIAN_POINT('Ctrl Pts',(13.595,15.4999999999999,8.17449999999987));
#19185=CARTESIAN_POINT('Ctrl Pts',(13.595,15.4999999999999,8.23700000000003));
#19186=CARTESIAN_POINT('Ctrl Pts',(13.595,15.4574945914102,8.23538973037462));
#19187=CARTESIAN_POINT('Ctrl Pts',(13.596422573169,15.4149448812192,8.23374666753423));
#19188=CARTESIAN_POINT('Ctrl Pts',(13.6155835759862,15.1294756706011,8.22251289282721));
#19189=CARTESIAN_POINT('Ctrl Pts',(13.6783172687067,14.8919169134681,8.21214111833337));
#19190=CARTESIAN_POINT('Ctrl Pts',(13.8939452341179,14.4447108048819,8.19048294539069));
#19191=CARTESIAN_POINT('Ctrl Pts',(14.0481586353087,14.2409467922808,8.17939057829159));
#19192=CARTESIAN_POINT('Ctrl Pts',(14.4203292232219,13.9116631203642,8.1587758224347));
#19193=CARTESIAN_POINT('Ctrl Pts',(14.6322997021123,13.786641160677,8.14995714338966));
#19194=CARTESIAN_POINT('Ctrl Pts',(15.0941629204617,13.6225082001164,8.12975315308563));
#19195=CARTESIAN_POINT('Ctrl Pts',(15.3400184947618,13.585823183673,8.11899831606461));
#19196=CARTESIAN_POINT('Ctrl Pts',(15.8381693806136,13.6083409191706,8.09720693873075));
#19197=CARTESIAN_POINT('Ctrl Pts',(16.0855752145909,13.669739009931,8.08638428632579));
#19198=CARTESIAN_POINT('Ctrl Pts',(16.5317875257589,13.8805701034552,8.06686493763077));
#19199=CARTESIAN_POINT('Ctrl Pts',(16.7282327266091,14.0239920966143,8.05771933408628));
#19200=CARTESIAN_POINT('Ctrl Pts',(17.0626902307113,14.3823785727111,8.03682692180615));
#19201=CARTESIAN_POINT('Ctrl Pts',(17.1952868030276,14.5960761529612,8.0258310416932));
#19202=CARTESIAN_POINT('Ctrl Pts',(17.3724973279344,15.067120882404,8.00411004587214));
#19203=CARTESIAN_POINT('Ctrl Pts',(17.4134713806441,15.3204986080025,7.9939854967544));
#19204=CARTESIAN_POINT('Ctrl Pts',(17.3940618301428,15.8170445447974,7.97474988123996));
#19205=CARTESIAN_POINT('Ctrl Pts',(17.3382739969744,16.0556202551099,7.96449150230556));
#19206=CARTESIAN_POINT('Ctrl Pts',(17.1362886591698,16.507583009347,7.94295152436876));
#19207=CARTESIAN_POINT('Ctrl Pts',(16.9886251887867,16.7151821216971,7.9318571306553));
#19208=CARTESIAN_POINT('Ctrl Pts',(16.6260958189486,17.0559878548847,7.9110167497448));
#19209=CARTESIAN_POINT('Ctrl Pts',(16.4166341910597,17.1878887790938,7.90209773364225));
#19210=CARTESIAN_POINT('Ctrl Pts',(15.9588791758701,17.3651469763034,7.88207345476258));
#19211=CARTESIAN_POINT('Ctrl Pts',(15.7148635545466,17.4087070536214,7.87139910562334));
#19212=CARTESIAN_POINT('Ctrl Pts',(15.216925645497,17.4006884912397,7.84961704486003));
#19213=CARTESIAN_POINT('Ctrl Pts',(14.9678130316258,17.346494933789,7.83871973016752));
#19214=CARTESIAN_POINT('Ctrl Pts',(14.5153907472423,17.1485805966075,7.81892872910089));
#19215=CARTESIAN_POINT('Ctrl Pts',(14.3146715051907,17.0107213240227,7.80997282577612));
#19216=CARTESIAN_POINT('Ctrl Pts',(13.9704168011547,16.6623674964646,7.7892462021458));
#19217=CARTESIAN_POINT('Ctrl Pts',(13.8320529297719,16.4532420018724,7.77829738645955));
#19218=CARTESIAN_POINT('Ctrl Pts',(13.6434492900726,15.9938293223661,7.75676786453815));
#19219=CARTESIAN_POINT('Ctrl Pts',(13.5950000041037,15.7480519480125,7.74639716931276));
#19220=CARTESIAN_POINT('Ctrl Pts',(13.595,15.5000000315158,7.73700000119396));
#19221=CARTESIAN_POINT('Origin',(15.5,15.5,-1.713));
#19222=CARTESIAN_POINT('',(13.595,15.5000000468491,7.17450000354951));
#19223=CARTESIAN_POINT('',(13.595,15.5,7.23700000000002));
#19224=CARTESIAN_POINT('',(13.595,15.5,-1.713));
#19225=CARTESIAN_POINT('Ctrl Pts',(13.595,15.5000000469168,7.17450000177725));
#19226=CARTESIAN_POINT('Ctrl Pts',(13.5950000060854,15.7470883071305,7.1838606629043));
#19227=CARTESIAN_POINT('Ctrl Pts',(13.6430734174731,15.9919359338936,7.1941879144583));
#19228=CARTESIAN_POINT('Ctrl Pts',(13.8306451460201,16.4507838931113,7.21567347235114));
#19229=CARTESIAN_POINT('Ctrl Pts',(13.9687228558569,16.6601426812252,7.22662486709875));
#19230=CARTESIAN_POINT('Ctrl Pts',(14.3124876181408,17.00900205961,7.24735992681755));
#19231=CARTESIAN_POINT('Ctrl Pts',(14.5129894026531,17.1471409984407,7.25632368340536));
#19232=CARTESIAN_POINT('Ctrl Pts',(14.9651005289506,17.3457108331891,7.27610107300719));
#19233=CARTESIAN_POINT('Ctrl Pts',(15.2141319420346,17.4002701330433,7.28699483560931));
#19234=CARTESIAN_POINT('Ctrl Pts',(15.7120908062108,17.4090216060289,7.30877781304487));
#19235=CARTESIAN_POINT('Ctrl Pts',(15.9562040613889,17.3658076341079,7.31945643313142));
#19236=CARTESIAN_POINT('Ctrl Pts',(16.4141694099564,17.1892137068839,7.33948991294629));
#19237=CARTESIAN_POINT('Ctrl Pts',(16.623757886392,17.0576649028473,7.34840208078488));
#19238=CARTESIAN_POINT('Ctrl Pts',(16.9867824147931,16.7174440987839,7.36923113255287));
#19239=CARTESIAN_POINT('Ctrl Pts',(17.1347818420411,16.5100355588719,7.38032565478166));
#19240=CARTESIAN_POINT('Ctrl Pts',(17.3374647859651,16.0583054532881,7.4018720773124));
#19241=CARTESIAN_POINT('Ctrl Pts',(17.3936068432643,15.8197767308892,7.41213642384694));
#19242=CARTESIAN_POINT('Ctrl Pts',(17.4137194975374,15.3233648227343,7.43138234030978));
#19243=CARTESIAN_POINT('Ctrl Pts',(17.3731570345151,15.0700682684394,7.44148395818749));
#19244=CARTESIAN_POINT('Ctrl Pts',(17.1967570875381,14.5988280085548,7.4631946322835));
#19245=CARTESIAN_POINT('Ctrl Pts',(17.0644839078362,14.3848819424175,7.47419285267569));
#19246=CARTESIAN_POINT('Ctrl Pts',(16.7305712796223,14.0259422626678,7.49509430478401));
#19247=CARTESIAN_POINT('Ctrl Pts',(16.5343592960234,13.8822126282349,7.50425243674433));
#19248=CARTESIAN_POINT('Ctrl Pts',(16.0884914737045,13.6706748179657,7.52375671593588));
#19249=CARTESIAN_POINT('Ctrl Pts',(15.8411855178205,13.6088828336564,7.53457499922039));
#19250=CARTESIAN_POINT('Ctrl Pts',(15.3430352235694,13.5855685820084,7.55636635067493));
#19251=CARTESIAN_POINT('Ctrl Pts',(15.0970841547928,13.6218741990355,7.56712536505709));
#19252=CARTESIAN_POINT('Ctrl Pts',(14.6349984075474,13.7852868598577,7.58733908978345));
#19253=CARTESIAN_POINT('Ctrl Pts',(14.4228899770894,13.9099360093728,7.59615438328633));
#19254=CARTESIAN_POINT('Ctrl Pts',(14.0501988550116,14.2385896315513,7.61675665567874));
#19255=CARTESIAN_POINT('Ctrl Pts',(13.8956314460231,14.4421390723225,7.62784863691793));
#19256=CARTESIAN_POINT('Ctrl Pts',(13.6792635784448,14.8890746339752,7.64951274383108));
#19257=CARTESIAN_POINT('Ctrl Pts',(13.6161520545551,15.1265722793911,7.65989046720001));
#19258=CARTESIAN_POINT('Ctrl Pts',(13.5964878424717,15.4130150531057,7.67117213057748));
#19259=CARTESIAN_POINT('Ctrl Pts',(13.595,15.4565304058035,7.67285320328655));
#19260=CARTESIAN_POINT('Ctrl Pts',(13.595,15.4999999999999,7.67449999999987));
#19261=CARTESIAN_POINT('Ctrl Pts',(13.595,15.5000000315158,7.73700000119396));
#19262=CARTESIAN_POINT('Ctrl Pts',(13.5949999999314,15.4958528079258,7.73684288828852));
#19263=CARTESIAN_POINT('Ctrl Pts',(13.5950135427448,15.4917049707995,7.73668545593254));
#19264=CARTESIAN_POINT('Ctrl Pts',(13.596621664402,15.2455180119549,7.72732376646322));
#19265=CARTESIAN_POINT('Ctrl Pts',(13.6443166811126,15.0060107870849,7.71720710638086));
#19266=CARTESIAN_POINT('Ctrl Pts',(13.8303098215743,14.5490220554584,7.69582651053382));
#19267=CARTESIAN_POINT('Ctrl Pts',(13.9702417349155,14.3372148383134,7.68474180417234));
#19268=CARTESIAN_POINT('Ctrl Pts',(14.3213455669013,13.9831176615365,7.6636477942646));
#19269=CARTESIAN_POINT('Ctrl Pts',(14.5279317852933,13.8431252163888,7.65452266905979));
#19270=CARTESIAN_POINT('Ctrl Pts',(14.9808551793442,13.6508243675268,7.63470974718525));
#19271=CARTESIAN_POINT('Ctrl Pts',(15.2225333764069,13.5994849650689,7.6241376475762));
#19272=CARTESIAN_POINT('Ctrl Pts',(15.7217895293589,13.5909093754666,7.60229792085037));
#19273=CARTESIAN_POINT('Ctrl Pts',(15.9746259000064,13.6375917998351,7.59123771216063));
#19274=CARTESIAN_POINT('Ctrl Pts',(16.4352634071348,13.8228499867134,7.57108734002026));
#19275=CARTESIAN_POINT('Ctrl Pts',(16.6404537600255,13.9550341255943,7.56225165420826));
#19276=CARTESIAN_POINT('Ctrl Pts',(16.9945851294045,14.2931114083031,7.54169832087678));
#19277=CARTESIAN_POINT('Ctrl Pts',(17.1386620530399,14.4974314044083,7.53080659870066));
#19278=CARTESIAN_POINT('Ctrl Pts',(17.3424379649764,14.9540000621413,7.5090529673736));
#19279=CARTESIAN_POINT('Ctrl Pts',(17.3984912162882,15.2025942427762,7.49840924465625));
#19280=CARTESIAN_POINT('Ctrl Pts',(17.4101799511541,15.6961858964362,7.47945442057061));
#19281=CARTESIAN_POINT('Ctrl Pts',(17.369989509654,15.9364146114939,7.46970116424717));
#19282=CARTESIAN_POINT('Ctrl Pts',(17.1988041419557,16.3977127086814,7.44848119247419));
#19283=CARTESIAN_POINT('Ctrl Pts',(17.0661099487767,16.6131602536261,7.43741688172641));
#19284=CARTESIAN_POINT('Ctrl Pts',(16.7257736644268,16.9794228970614,7.41609750745491));
#19285=CARTESIAN_POINT('Ctrl Pts',(16.5218223593459,17.1269843255975,7.40669914082883));
#19286=CARTESIAN_POINT('Ctrl Pts',(16.0734117987848,17.3329803183507,7.38708363074307));
#19287=CARTESIAN_POINT('Ctrl Pts',(15.8340676287476,17.3912953159661,7.37661363205379));
#19288=CARTESIAN_POINT('Ctrl Pts',(15.3368116312762,17.414883025994,7.3548614011933));
#19289=CARTESIAN_POINT('Ctrl Pts',(15.0834797431034,17.3761481699676,7.34377951632137));
#19290=CARTESIAN_POINT('Ctrl Pts',(14.6171531313432,17.2054527007769,7.3233802769618));
#19291=CARTESIAN_POINT('Ctrl Pts',(14.4071993495888,17.0791692941371,7.31458969380564));
#19292=CARTESIAN_POINT('Ctrl Pts',(14.0429440084805,16.7517930749219,7.29422032403357));
#19293=CARTESIAN_POINT('Ctrl Pts',(13.8931313169624,16.5525972484919,7.28339727102502));
#19294=CARTESIAN_POINT('Ctrl Pts',(13.6754984349704,16.103249384372,7.26161410801274));
#19295=CARTESIAN_POINT('Ctrl Pts',(13.6117049129581,15.8564836530191,7.2508703567817));
#19296=CARTESIAN_POINT('Ctrl Pts',(13.5959534549509,15.5696266820693,7.23965858280537));
#19297=CARTESIAN_POINT('Ctrl Pts',(13.595,15.5347980724284,7.23831828585853));
#19298=CARTESIAN_POINT('Ctrl Pts',(13.595,15.5,7.23700000000002));
#19299=CARTESIAN_POINT('Origin',(15.5,15.5,-1.713));
#19300=CARTESIAN_POINT('',(13.595,15.5,6.67449999999986));
#19301=CARTESIAN_POINT('',(13.595,15.5,6.73700000000002));
#19302=CARTESIAN_POINT('',(13.595,15.5,-1.713));
#19303=CARTESIAN_POINT('Ctrl Pts',(13.595,15.5,6.67449999999986));
#19304=CARTESIAN_POINT('Ctrl Pts',(13.595,15.5337860699612,6.67577994728247));
#19305=CARTESIAN_POINT('Ctrl Pts',(13.5958988051172,15.5676012636805,6.67708065679041));
#19306=CARTESIAN_POINT('Ctrl Pts',(13.6111380804091,15.8534666090834,6.68824366155095));
#19307=CARTESIAN_POINT('Ctrl Pts',(13.6745367085023,16.1003319863785,6.69898255053165));
#19308=CARTESIAN_POINT('Ctrl Pts',(13.8914661703111,16.5500598413007,6.72076472367497));
#19309=CARTESIAN_POINT('Ctrl Pts',(14.0409894081154,16.7495218496875,6.73159152967911));
#19310=CARTESIAN_POINT('Ctrl Pts',(14.4047282234883,17.0774481133631,6.75197043967901));
#19311=CARTESIAN_POINT('Ctrl Pts',(14.614434389684,17.2040348641911,6.76076134688004));
#19312=CARTESIAN_POINT('Ctrl Pts',(15.0804714953236,17.3754834245413,6.78114792192992));
#19313=CARTESIAN_POINT('Ctrl Pts',(15.3337836813351,17.4146280576722,6.79222894494007));
#19314=CARTESIAN_POINT('Ctrl Pts',(15.8311536453238,17.3918124142706,6.81398616121256));
#19315=CARTESIAN_POINT('Ctrl Pts',(16.0706231306758,17.3338551940679,6.82446164176166));
#19316=CARTESIAN_POINT('Ctrl Pts',(16.5192695723309,17.1285669310391,6.84408747035551));
#19317=CARTESIAN_POINT('Ctrl Pts',(16.723357731448,16.9814015000744,6.85346970837494));
#19318=CARTESIAN_POINT('Ctrl Pts',(17.0642592513022,16.6157687823903,6.87477758159879));
#19319=CARTESIAN_POINT('Ctrl Pts',(17.1973319398078,16.4005046466869,6.88584322264411));
#19320=CARTESIAN_POINT('Ctrl Pts',(17.3692884929086,15.9394217717019,6.90707190853817));
#19321=CARTESIAN_POINT('Ctrl Pts',(17.4098676563665,15.699232024322,6.91684585203433));
#19322=CARTESIAN_POINT('Ctrl Pts',(17.3989594809284,15.2056008222122,6.93578510176519));
#19323=CARTESIAN_POINT('Ctrl Pts',(17.3433005725257,14.9569204724809,6.94642346372892));
#19324=CARTESIAN_POINT('Ctrl Pts',(17.1402345257407,14.4999966777563,6.96817502266233));
#19325=CARTESIAN_POINT('Ctrl Pts',(16.9964533203441,14.295420842877,6.97906996897484));
#19326=CARTESIAN_POINT('Ctrl Pts',(16.6428379287255,13.9568026893442,6.99963250698671));
#19327=CARTESIAN_POINT('Ctrl Pts',(16.4378853679788,13.8243202013929,7.00847264357042));
#19328=CARTESIAN_POINT('Ctrl Pts',(15.9775384842111,13.6383308597002,7.02861030252789));
#19329=CARTESIAN_POINT('Ctrl Pts',(15.7247333891731,13.5912482315457,7.03966914308073));
#19330=CARTESIAN_POINT('Ctrl Pts',(15.2253882367842,13.5990657619463,7.06151276304523));
#19331=CARTESIAN_POINT('Ctrl Pts',(14.9835978859395,13.6500518687448,7.07208976876896));
#19332=CARTESIAN_POINT('Ctrl Pts',(14.5304506110992,13.8416645991434,7.09191248420376));
#19333=CARTESIAN_POINT('Ctrl Pts',(14.3237325854823,13.9812818988211,7.10102603895217));
#19334=CARTESIAN_POINT('Ctrl Pts',(13.972097067769,14.334769301076,7.12210857740915));
#19335=CARTESIAN_POINT('Ctrl Pts',(13.8318063975557,14.5463886664587,7.13319401404347));
#19336=CARTESIAN_POINT('Ctrl Pts',(13.6450737883124,15.0031578759162,7.1545824673977));
#19337=CARTESIAN_POINT('Ctrl Pts',(13.5970057201001,15.2426281300911,7.16470588636848));
#19338=CARTESIAN_POINT('Ctrl Pts',(13.5950204734553,15.4898007705079,7.17411316585421));
#19339=CARTESIAN_POINT('Ctrl Pts',(13.5949999998744,15.4949008690299,7.17430682515208));
#19340=CARTESIAN_POINT('Ctrl Pts',(13.595,15.5000000469168,7.17450000177725));
#19341=CARTESIAN_POINT('Ctrl Pts',(13.595,15.5,7.23700000000002));
#19342=CARTESIAN_POINT('Ctrl Pts',(13.595,15.2942576541637,7.22920568249658));
#19343=CARTESIAN_POINT('Ctrl Pts',(13.628327246639,15.0896374680993,7.22072493435236));
#19344=CARTESIAN_POINT('Ctrl Pts',(13.7733657429176,14.6572925777788,7.20117371360197));
#19345=CARTESIAN_POINT('Ctrl Pts',(13.8986221191241,14.4383926325365,7.19014129446066));
#19346=CARTESIAN_POINT('Ctrl Pts',(14.2277936453813,14.059884404928,7.16860220855603));
#19347=CARTESIAN_POINT('Ctrl Pts',(14.429067625472,13.9045310289345,7.15884743545613));
#19348=CARTESIAN_POINT('Ctrl Pts',(14.8728424555568,13.6848003334792,7.13943471323016));
#19349=CARTESIAN_POINT('Ctrl Pts',(15.1096558493003,13.6196045289078,7.12907542216525));
#19350=CARTESIAN_POINT('Ctrl Pts',(15.6044749214628,13.581123133793,7.10742979346171));
#19351=CARTESIAN_POINT('Ctrl Pts',(15.8580627362377,13.6119307905017,7.09633671320034));
#19352=CARTESIAN_POINT('Ctrl Pts',(16.3299097903082,13.7679999989471,7.07569598467581));
#19353=CARTESIAN_POINT('Ctrl Pts',(16.5446974999677,13.8884229991925,7.06686954824442));
#19354=CARTESIAN_POINT('Ctrl Pts',(16.9188396017716,14.2051892618886,7.04668587888927));
#19355=CARTESIAN_POINT('Ctrl Pts',(17.0741210324274,14.3991952212007,7.03593982444579));
#19356=CARTESIAN_POINT('Ctrl Pts',(17.3051308825832,14.8410333985517,7.01414857286987));
#19357=CARTESIAN_POINT('Ctrl Pts',(17.3764755515413,15.0857600434564,7.00331690944251));
#19358=CARTESIAN_POINT('Ctrl Pts',(17.418630387735,15.5774907630638,6.98376622208042));
#19359=CARTESIAN_POINT('Ctrl Pts',(17.3934433069012,15.8194293865979,6.97464600568416));
#19360=CARTESIAN_POINT('Ctrl Pts',(17.2518638159962,16.2886764165972,6.95377244513816));
#19361=CARTESIAN_POINT('Ctrl Pts',(17.1338792671752,16.5106793888636,6.94278152264873));
#19362=CARTESIAN_POINT('Ctrl Pts',(16.8157454348218,16.9009266926162,6.9210391344167));
#19363=CARTESIAN_POINT('Ctrl Pts',(16.6170831517666,17.0639271109788,6.91086627960484));
#19364=CARTESIAN_POINT('Ctrl Pts',(16.1778473847405,17.2967960249788,6.89165211656785));
#19365=CARTESIAN_POINT('Ctrl Pts',(15.9436257910071,17.3684557001225,6.88140620258127));
#19366=CARTESIAN_POINT('Ctrl Pts',(15.4515313244385,17.4210087460935,6.85987976047418));
#19367=CARTESIAN_POINT('Ctrl Pts',(15.1979214060386,17.3977303546936,6.8487857133001));
#19368=CARTESIAN_POINT('Ctrl Pts',(14.720973480494,17.2556731756669,6.82792184954051));
#19369=CARTESIAN_POINT('Ctrl Pts',(14.5015106013679,17.140818696364,6.81898801289335));
#19370=CARTESIAN_POINT('Ctrl Pts',(14.1181476122605,16.834088526908,6.79898286794978));
#19371=CARTESIAN_POINT('Ctrl Pts',(13.9578961778042,16.6450805307376,6.78831745047689));
#19372=CARTESIAN_POINT('Ctrl Pts',(13.7145778437055,16.2106454797413,6.76653744358683));
#19373=CARTESIAN_POINT('Ctrl Pts',(13.6362134003717,15.9680461672624,6.75563283338496));
#19374=CARTESIAN_POINT('Ctrl Pts',(13.5991327778437,15.644972943146,6.74258253020773));
#19375=CARTESIAN_POINT('Ctrl Pts',(13.595,15.5724496349748,6.73974467298265));
#19376=CARTESIAN_POINT('Ctrl Pts',(13.595,15.5000000000001,6.73700000000002));
#19377=CARTESIAN_POINT('Origin',(15.5,15.5,-1.713));
#19378=CARTESIAN_POINT('',(13.595,15.5,6.17449999999985));
#19379=CARTESIAN_POINT('',(13.595,15.5,6.237));
#19380=CARTESIAN_POINT('',(13.595,15.5,-1.713));
#19381=CARTESIAN_POINT('Ctrl Pts',(13.595,15.5000000000001,6.17449999999985));
#19382=CARTESIAN_POINT('Ctrl Pts',(13.595,15.5715577417839,6.1772108846115));
#19383=CARTESIAN_POINT('Ctrl Pts',(13.5990316560547,15.643188728214,6.18001272546772));
#19384=CARTESIAN_POINT('Ctrl Pts',(13.6355563128653,15.9654212002569,6.19301901746765));
#19385=CARTESIAN_POINT('Ctrl Pts',(13.7135786375042,16.2081294563647,6.20392027196532));
#19386=CARTESIAN_POINT('Ctrl Pts',(13.9562999717204,16.6429348882667,6.22570125257942));
#19387=CARTESIAN_POINT('Ctrl Pts',(14.1163117558812,16.8321904053189,6.23637080540767));
#19388=CARTESIAN_POINT('Ctrl Pts',(14.4992244320732,17.139413936818,6.2563847914538));
#19389=CARTESIAN_POINT('Ctrl Pts',(14.7184550745985,17.2545428804559,6.26531168305308));
#19390=CARTESIAN_POINT('Ctrl Pts',(15.19515525073,17.397292910129,6.2861647091306));
#19391=CARTESIAN_POINT('Ctrl Pts',(15.4487691333913,17.4209419080911,6.29725892971948));
#19392=CARTESIAN_POINT('Ctrl Pts',(15.941007088933,17.3690797945405,6.31879164868458));
#19393=CARTESIAN_POINT('Ctrl Pts',(16.1753605576116,17.2977366465769,6.32904333147894));
#19394=CARTESIAN_POINT('Ctrl Pts',(16.6148230416808,17.0655168979927,6.3482674121469));
#19395=CARTESIAN_POINT('Ctrl Pts',(16.8136158148582,16.9028988231385,6.35841784285429));
#19396=CARTESIAN_POINT('Ctrl Pts',(17.1323034625999,16.5132318636455,6.38015035859392));
#19397=CARTESIAN_POINT('Ctrl Pts',(17.2506507476386,16.2913774471692,6.3911435870773));
#19398=CARTESIAN_POINT('Ctrl Pts',(17.3929528169657,15.8223174322594,6.41202586719434));
#19399=CARTESIAN_POINT('Ctrl Pts',(17.4185084978342,15.5804256811536,6.42115770201604));
#19400=CARTESIAN_POINT('Ctrl Pts',(17.3771090366558,15.0886410810562,6.44069390881674));
#19401=CARTESIAN_POINT('Ctrl Pts',(17.3061406522188,14.8438067616542,6.45152142117628));
#19402=CARTESIAN_POINT('Ctrl Pts',(17.0757940579712,14.4015833220502,6.47331276106997));
#19403=CARTESIAN_POINT('Ctrl Pts',(16.920782151046,14.2073142095694,6.48406288968071));
#19404=CARTESIAN_POINT('Ctrl Pts',(16.5471333786859,13.890014926918,6.50425596166491));
#19405=CARTESIAN_POINT('Ctrl Pts',(16.3325910784869,13.769296908048,6.51307869297957));
#19406=CARTESIAN_POINT('Ctrl Pts',(15.8610184152089,13.6124883201033,6.53370741840729));
#19407=CARTESIAN_POINT('Ctrl Pts',(15.6074377895398,13.5812814714514,6.54480018418459));
#19408=CARTESIAN_POINT('Ctrl Pts',(15.1124854292573,13.6190147779313,6.5664516435145));
#19409=CARTESIAN_POINT('Ctrl Pts',(14.8755397433854,13.6838659268469,6.57681672163662));
#19410=CARTESIAN_POINT('Ctrl Pts',(14.4315280685365,13.9029027899722,6.59623980452585));
#19411=CARTESIAN_POINT('Ctrl Pts',(14.2301177041952,14.0578576203021,6.60597459366607));
#19412=CARTESIAN_POINT('Ctrl Pts',(13.9003731317584,14.4357464363045,6.62750274767666));
#19413=CARTESIAN_POINT('Ctrl Pts',(13.7747368954394,14.6544769786506,6.63853705758105));
#19414=CARTESIAN_POINT('Ctrl Pts',(13.6286625233942,15.0875972864192,6.65814031110006));
#19415=CARTESIAN_POINT('Ctrl Pts',(13.595,15.2932256254231,6.66666658524766));
#19416=CARTESIAN_POINT('Ctrl Pts',(13.595,15.5,6.67449999999986));
#19417=CARTESIAN_POINT('Ctrl Pts',(13.595,15.5000000000001,6.73700000000002));
#19418=CARTESIAN_POINT('Ctrl Pts',(13.595,15.3319584802696,6.73063393591528));
#19419=CARTESIAN_POINT('Ctrl Pts',(13.6172311655285,15.1643504197289,6.72379804697953));
#19420=CARTESIAN_POINT('Ctrl Pts',(13.7263421054778,14.7618781860687,6.70616433531536));
#19421=CARTESIAN_POINT('Ctrl Pts',(13.8375522583477,14.5372185214291,6.69522093841164));
#19422=CARTESIAN_POINT('Ctrl Pts',(14.1423728428836,14.1400106685456,6.67350604849701));
#19423=CARTESIAN_POINT('Ctrl Pts',(14.3342559177248,13.9723538283477,6.66299492923329));
#19424=CARTESIAN_POINT('Ctrl Pts',(14.7631181034437,13.726703827452,6.644234553655));
#19425=CARTESIAN_POINT('Ctrl Pts',(14.9940630811368,13.6475482050451,6.6341319737034));
#19426=CARTESIAN_POINT('Ctrl Pts',(15.4824475728478,13.5785748586731,6.6127678227099));
#19427=CARTESIAN_POINT('Ctrl Pts',(15.7358073629665,13.5930174114947,6.60168471728038));
#19428=CARTESIAN_POINT('Ctrl Pts',(16.2185584714547,13.718446186762,6.58056699599917));
#19429=CARTESIAN_POINT('Ctrl Pts',(16.4436261482446,13.826733204793,6.57141725624811));
#19430=CARTESIAN_POINT('Ctrl Pts',(16.8376270305051,14.1217112584022,6.55162465217484));
#19431=CARTESIAN_POINT('Ctrl Pts',(17.0034432989467,14.3047731521569,6.54106278057916));
#19432=CARTESIAN_POINT('Ctrl Pts',(17.2617626336329,14.7319068969529,6.51923126959273));
#19433=CARTESIAN_POINT('Ctrl Pts',(17.3485015451824,14.97385099212,6.50816831296608));
#19434=CARTESIAN_POINT('Ctrl Pts',(17.4199935020024,15.465166709918,6.48799167817601));
#19435=CARTESIAN_POINT('Ctrl Pts',(17.4088947887542,15.7090770775306,6.47916453779018));
#19436=CARTESIAN_POINT('Ctrl Pts',(17.2946791504231,16.1851663182313,6.45863027724424));
#19437=CARTESIAN_POINT('Ctrl Pts',(17.1905355878056,16.4123637607824,6.4477453018185));
#19438=CARTESIAN_POINT('Ctrl Pts',(16.8983953461694,16.8180237191349,6.42598756122144));
#19439=CARTESIAN_POINT('Ctrl Pts',(16.7116966296892,16.9914800033301,6.41533284088903));
#19440=CARTESIAN_POINT('Ctrl Pts',(16.2909568390832,17.2497545968349,6.39634586562964));
#19441=CARTESIAN_POINT('Ctrl Pts',(16.0631484549132,17.3357989702144,6.38663466556925));
#19442=CARTESIAN_POINT('Ctrl Pts',(15.5784723919421,17.4197976388017,6.36543273805523));
#19443=CARTESIAN_POINT('Ctrl Pts',(15.3256071822455,17.4134707300782,6.3543712678148));
#19444=CARTESIAN_POINT('Ctrl Pts',(14.8377051185746,17.3035246283544,6.33302822041015));
#19445=CARTESIAN_POINT('Ctrl Pts',(14.6073698852201,17.2013323949424,6.32359588875386));
#19446=CARTESIAN_POINT('Ctrl Pts',(14.2037461977663,16.9171476811232,6.30400170567155));
#19447=CARTESIAN_POINT('Ctrl Pts',(14.0330635436095,16.7396208715381,6.29354308563515));
#19448=CARTESIAN_POINT('Ctrl Pts',(13.7627491799401,16.3217808344018,6.27180129785241));
#19449=CARTESIAN_POINT('Ctrl Pts',(13.6688775154418,16.0834106034676,6.26071772358537));
#19450=CARTESIAN_POINT('Ctrl Pts',(13.6048088999498,15.7232646950227,6.24567267487459));
#19451=CARTESIAN_POINT('Ctrl Pts',(13.595,15.6116185684224,6.24122854399773));
#19452=CARTESIAN_POINT('Ctrl Pts',(13.595,15.5,6.23700000000001));
#19453=CARTESIAN_POINT('Origin',(15.5,15.5,-1.713));
#19454=CARTESIAN_POINT('',(13.595,15.5,5.67449999999984));
#19455=CARTESIAN_POINT('',(13.595,15.5,5.73700000000001));
#19456=CARTESIAN_POINT('',(13.595,15.5,-1.713));
#19457=CARTESIAN_POINT('Ctrl Pts',(13.595,15.5,5.67449999999984));
#19458=CARTESIAN_POINT('Ctrl Pts',(13.595,15.6185870823364,5.67899253831409));
#19459=CARTESIAN_POINT('Ctrl Pts',(13.6060718415959,15.7371765549238,5.68372733344444));
#19460=CARTESIAN_POINT('Ctrl Pts',(13.6740404949213,16.0963304252555,5.69882010257118));
#19461=CARTESIAN_POINT('Ctrl Pts',(13.7663946575648,16.3272477032882,5.70958813889097));
#19462=CARTESIAN_POINT('Ctrl Pts',(14.0371620226424,16.7461278929931,5.73137923985182));
#19463=CARTESIAN_POINT('Ctrl Pts',(14.2149617564259,16.9287854291272,5.74218789835473));
#19464=CARTESIAN_POINT('Ctrl Pts',(14.6220504754878,17.2077275576028,5.76165926007725));
#19465=CARTESIAN_POINT('Ctrl Pts',(14.84495768549,17.3050114079439,5.77084548055492));
#19466=CARTESIAN_POINT('Ctrl Pts',(15.3232149840341,17.4130834901566,5.79176662222354));
#19467=CARTESIAN_POINT('Ctrl Pts',(15.5747489125264,17.4197790697252,5.80276985619085));
#19468=CARTESIAN_POINT('Ctrl Pts',(16.070537711592,17.3351810404709,5.82445790514388));
#19469=CARTESIAN_POINT('Ctrl Pts',(16.309578092675,17.2429720428253,5.83451010407533));
#19470=CARTESIAN_POINT('Ctrl Pts',(16.7284047199156,16.9761646688132,5.85377848891489));
#19471=CARTESIAN_POINT('Ctrl Pts',(16.9064279364666,16.8076615476523,5.86405581139163));
#19472=CARTESIAN_POINT('Ctrl Pts',(17.1950904546403,16.4052040196009,5.88561616582402));
#19473=CARTESIAN_POINT('Ctrl Pts',(17.2999825807302,16.1729023374491,5.89671088240892));
#19474=CARTESIAN_POINT('Ctrl Pts',(17.4114614926336,15.6881070632203,5.91751510284064));
#19475=CARTESIAN_POINT('Ctrl Pts',(17.4197869012108,15.440967858228,5.92641294329876));
#19476=CARTESIAN_POINT('Ctrl Pts',(17.3422502165789,14.9563903088349,5.94646652204742));
#19477=CARTESIAN_POINT('Ctrl Pts',(17.2568553212246,14.7235705434374,5.95715441701744));
#19478=CARTESIAN_POINT('Ctrl Pts',(16.9988862893144,14.2974670698628,5.97893923542126));
#19479=CARTESIAN_POINT('Ctrl Pts',(16.8265177477385,14.1096348386612,5.98982513894961));
#19480=CARTESIAN_POINT('Ctrl Pts',(16.4275948667997,13.8186878681828,6.00957268523384));
#19481=CARTESIAN_POINT('Ctrl Pts',(16.2074192267811,13.7148358895865,6.01855427704374));
#19482=CARTESIAN_POINT('Ctrl Pts',(15.7329940381332,13.5930407731274,6.03930778485859));
#19483=CARTESIAN_POINT('Ctrl Pts',(15.4825177602965,13.5789405886467,6.05026475235153));
#19484=CARTESIAN_POINT('Ctrl Pts',(14.9967865899441,13.6468020229089,6.07151283504417));
#19485=CARTESIAN_POINT('Ctrl Pts',(14.7656927933891,13.725631450455,6.08162192504857));
#19486=CARTESIAN_POINT('Ctrl Pts',(14.3364443687422,13.970685449457,6.10039919646789));
#19487=CARTESIAN_POINT('Ctrl Pts',(14.1443188999266,14.1380702221899,6.11088997219073));
#19488=CARTESIAN_POINT('Ctrl Pts',(13.8389083728738,14.5348718312672,6.13260237539498));
#19489=CARTESIAN_POINT('Ctrl Pts',(13.7273677282824,14.7594070229154,6.14354828538213));
#19490=CARTESIAN_POINT('Ctrl Pts',(13.617463969655,15.1626075070602,6.16122692673826));
#19491=CARTESIAN_POINT('Ctrl Pts',(13.595,15.331080930445,6.16810069092643));
#19492=CARTESIAN_POINT('Ctrl Pts',(13.595,15.5000000000001,6.17449999999985));
#19493=CARTESIAN_POINT('Ctrl Pts',(13.595,15.5,6.23700000000001));
#19494=CARTESIAN_POINT('Ctrl Pts',(13.595,15.36977425128,6.23206654389246));
#19495=CARTESIAN_POINT('Ctrl Pts',(13.6083515816957,15.2396084108537,6.22684332799736));
#19496=CARTESIAN_POINT('Ctrl Pts',(13.6853629128828,14.8698795142821,6.21115215203331));
#19497=CARTESIAN_POINT('Ctrl Pts',(13.7821919173308,14.6402997106635,6.20033690949815));
#19498=CARTESIAN_POINT('Ctrl Pts',(14.0611179371588,14.2262903224373,6.17855188510953));
#19499=CARTESIAN_POINT('Ctrl Pts',(14.2423406160885,14.04706032314,6.16779820742024));
#19500=CARTESIAN_POINT('Ctrl Pts',(14.6546344062719,13.7759103546784,6.14850819622096));
#19501=CARTESIAN_POINT('Ctrl Pts',(14.8793586066212,13.6828711974297,6.13914966725177));
#19502=CARTESIAN_POINT('Ctrl Pts',(15.3600638250521,13.5838064298187,6.11812144247349));
#19503=CARTESIAN_POINT('Ctrl Pts',(15.6121739396263,13.5819811503158,6.10709300351574));
#19504=CARTESIAN_POINT('Ctrl Pts',(16.1050697123474,13.6761386719974,6.08553150864603));
#19505=CARTESIAN_POINT('Ctrl Pts',(16.340817115604,13.7721168422437,6.07573500226256));
#19506=CARTESIAN_POINT('Ctrl Pts',(16.7615603791949,14.0504456667631,6.05598821904094));
#19507=CARTESIAN_POINT('Ctrl Pts',(16.9423029071645,14.2301645816036,6.04522652131986));
#19508=CARTESIAN_POINT('Ctrl Pts',(17.2200799494863,14.644872787505,6.02344015375077));
#19509=CARTESIAN_POINT('Ctrl Pts',(17.3162769006898,14.8746469811613,6.01263137140422));
#19510=CARTESIAN_POINT('Ctrl Pts',(17.4149152048833,15.3544317846958,5.99229782020969));
#19511=CARTESIAN_POINT('Ctrl Pts',(17.4178535000102,15.5996361896873,5.98350653012241));
#19512=CARTESIAN_POINT('Ctrl Pts',(17.3295289414075,16.0883584972103,5.96305997662234));
#19513=CARTESIAN_POINT('Ctrl Pts',(17.2350439049634,16.3264087530365,5.95197510841829));
#19514=CARTESIAN_POINT('Ctrl Pts',(16.9637023080458,16.7434259265959,5.93024202597844));
#19515=CARTESIAN_POINT('Ctrl Pts',(16.7926052916268,16.9204658432537,5.91979278829171));
#19516=CARTESIAN_POINT('Ctrl Pts',(16.3881467431463,17.2037067413353,5.90021610030532));
#19517=CARTESIAN_POINT('Ctrl Pts',(16.1573456231628,17.3053625544976,5.89075527660389));
#19518=CARTESIAN_POINT('Ctrl Pts',(15.6690018842731,17.4139452013283,5.86939290832352));
#19519=CARTESIAN_POINT('Ctrl Pts',(15.4161920266675,17.4195630080999,5.8583338594344));
#19520=CARTESIAN_POINT('Ctrl Pts',(14.9318550990572,17.3342537273976,5.83714676723799));
#19521=CARTESIAN_POINT('Ctrl Pts',(14.7043172849098,17.2476057238062,5.82746936111434));
#19522=CARTESIAN_POINT('Ctrl Pts',(14.2842996795786,16.9882190243175,5.80845605079822));
#19523=CARTESIAN_POINT('Ctrl Pts',(14.0980650179494,16.8142588725985,5.79779239194216));
#19524=CARTESIAN_POINT('Ctrl Pts',(13.8070527298312,16.4078633395944,5.77603145582555));
#19525=CARTESIAN_POINT('Ctrl Pts',(13.7035368615051,16.1804517914393,5.76515209834613));
#19526=CARTESIAN_POINT('Ctrl Pts',(13.6121804111135,15.7952504451143,5.74856100575271));
#19527=CARTESIAN_POINT('Ctrl Pts',(13.595,15.6477240375953,5.74259635911231));
#19528=CARTESIAN_POINT('Ctrl Pts',(13.595,15.5,5.737));
#19529=CARTESIAN_POINT('Origin',(15.5,15.5,-1.713));
#19530=CARTESIAN_POINT('',(13.595,15.5,5.17449999999983));
#19531=CARTESIAN_POINT('',(13.595,15.5,5.23699999999999));
#19532=CARTESIAN_POINT('',(13.595,15.5,-1.713));
#19533=CARTESIAN_POINT('Ctrl Pts',(13.595,15.5,5.17449999999983));
#19534=CARTESIAN_POINT('Ctrl Pts',(13.595,15.6566421856364,5.18043421312606));
#19535=CARTESIAN_POINT('Ctrl Pts',(13.6143173106204,15.8129938957689,5.18677993526994));
#19536=CARTESIAN_POINT('Ctrl Pts',(13.7133238837561,16.2058714082875,5.20382915631037));
#19537=CARTESIAN_POINT('Ctrl Pts',(13.8202268828639,16.4321058332676,5.21473800402677));
#19538=CARTESIAN_POINT('Ctrl Pts',(14.1173121943619,16.8344891762869,5.23647977361834));
#19539=CARTESIAN_POINT('Ctrl Pts',(14.3060377434444,17.0057115198797,5.24709419504389));
#19540=CARTESIAN_POINT('Ctrl Pts',(14.7299474211406,17.2590800413806,5.26596464189374));
#19541=CARTESIAN_POINT('Ctrl Pts',(14.9589591096765,17.3424619118548,5.2758324194957));
#19542=CARTESIAN_POINT('Ctrl Pts',(15.4451221171311,17.4206572734562,5.29709939270021));
#19543=CARTESIAN_POINT('Ctrl Pts',(15.6982088678367,17.4111913786412,5.30817055414842));
#19544=CARTESIAN_POINT('Ctrl Pts',(16.1841394261652,17.2952308599276,5.32942735897471));
#19545=CARTESIAN_POINT('Ctrl Pts',(16.4124232908667,17.1906721299216,5.33874088501521));
#19546=CARTESIAN_POINT('Ctrl Pts',(16.8123402712279,16.9023113076282,5.35841220118947));
#19547=CARTESIAN_POINT('Ctrl Pts',(16.9811679057763,16.7226354335115,5.36891166263772));
#19548=CARTESIAN_POINT('Ctrl Pts',(17.2468951151508,16.3011735866021,5.39069032715379));
#19549=CARTESIAN_POINT('Ctrl Pts',(17.3380327017994,16.0614016975905,5.40176720118363));
#19550=CARTESIAN_POINT('Ctrl Pts',(17.4190450446205,15.5715263806302,5.42209750042186));
#19551=CARTESIAN_POINT('Ctrl Pts',(17.4125604492154,15.3268971480608,5.43089244281013));
#19552=CARTESIAN_POINT('Ctrl Pts',(17.3071804140669,14.8486945914045,5.45131350929278));
#19553=CARTESIAN_POINT('Ctrl Pts',(17.2075400051757,14.6200014430832,5.46215665367438));
#19554=CARTESIAN_POINT('Ctrl Pts',(16.9235169449159,14.2091439135888,5.48393375726179));
#19555=CARTESIAN_POINT('Ctrl Pts',(16.740171888673,14.0321078283592,5.49465074218377));
#19556=CARTESIAN_POINT('Ctrl Pts',(16.3246235208931,13.7658853657224,5.5138252653505));
#19557=CARTESIAN_POINT('Ctrl Pts',(16.0987313329976,13.675525196633,5.5233087780841));
#19558=CARTESIAN_POINT('Ctrl Pts',(15.6164951667096,13.5821988514804,5.54440397345977));
#19559=CARTESIAN_POINT('Ctrl Pts',(15.3640667095275,13.583478423546,5.55544633816588));
#19560=CARTESIAN_POINT('Ctrl Pts',(14.8730509487618,13.6836792610265,5.57692559279253));
#19561=CARTESIAN_POINT('Ctrl Pts',(14.6393794120696,13.7820369440063,5.58657395646151));
#19562=CARTESIAN_POINT('Ctrl Pts',(14.2298320094521,14.0594989012133,5.60604302053995));
#19563=CARTESIAN_POINT('Ctrl Pts',(14.0562371293134,14.233548774446,5.61643361773215));
#19564=CARTESIAN_POINT('Ctrl Pts',(13.7786824085209,14.6454944475955,5.63811046717757));
#19565=CARTESIAN_POINT('Ctrl Pts',(13.6804785478273,14.8815606152973,5.64920150954635));
#19566=CARTESIAN_POINT('Ctrl Pts',(13.6070998178414,15.2520820958729,5.66484325844481));
#19567=CARTESIAN_POINT('Ctrl Pts',(13.595,15.3760295924857,5.66980352046244));
#19568=CARTESIAN_POINT('Ctrl Pts',(13.595,15.5,5.67449999999984));
#19569=CARTESIAN_POINT('Ctrl Pts',(13.595,15.5,5.73700000000001));
#19570=CARTESIAN_POINT('Ctrl Pts',(13.595,15.4066866192903,5.73346492746249));
#19571=CARTESIAN_POINT('Ctrl Pts',(13.6018555842158,15.3133058701765,5.72977735558749));
#19572=CARTESIAN_POINT('Ctrl Pts',(13.6529137828576,14.9689371987211,5.71561457706302));
#19573=CARTESIAN_POINT('Ctrl Pts',(13.7402672426745,14.7272905418752,5.70454944698966));
#19574=CARTESIAN_POINT('Ctrl Pts',(13.9996235813187,14.3009379189473,5.68272484630075));
#19575=CARTESIAN_POINT('Ctrl Pts',(14.1658625390628,14.1183438769257,5.67217145356922));
#19576=CARTESIAN_POINT('Ctrl Pts',(14.5606866342577,13.8242830841638,5.65239559335981));
#19577=CARTESIAN_POINT('Ctrl Pts',(14.7861975769119,13.7165114108178,5.64322495289096));
#19578=CARTESIAN_POINT('Ctrl Pts',(15.2693933527132,13.5923905631024,5.62208777984625));
#19579=CARTESIAN_POINT('Ctrl Pts',(15.5227209974273,13.5786379454799,5.61100608060241));
#19580=CARTESIAN_POINT('Ctrl Pts',(16.0107923698647,13.6488891805299,5.58965562686497));
#19581=CARTESIAN_POINT('Ctrl Pts',(16.2414707537612,13.7286260121631,5.57956470893425));
#19582=CARTESIAN_POINT('Ctrl Pts',(16.6696419804527,13.9753377070707,5.56083455903523));
#19583=CARTESIAN_POINT('Ctrl Pts',(16.86109178745,14.1434790644713,5.55028677590578));
#19584=CARTESIAN_POINT('Ctrl Pts',(17.1648587298731,14.5414095863163,5.52856755403043));
#19585=CARTESIAN_POINT('Ctrl Pts',(17.2754789966671,14.7662901237697,5.5176286917536));
#19586=CARTESIAN_POINT('Ctrl Pts',(17.4024536246495,15.2392462161482,5.49693405899484));
#19587=CARTESIAN_POINT('Ctrl Pts',(17.4201554501318,15.4821893016267,5.48800622232349));
#19588=CARTESIAN_POINT('Ctrl Pts',(17.3626040078135,15.9727313988826,5.46816380591895));
#19589=CARTESIAN_POINT('Ctrl Pts',(17.2836290157076,16.2151349357133,5.45725325837236));
#19590=CARTESIAN_POINT('Ctrl Pts',(17.0392460050135,16.6489065389848,5.43547509856397));
#19591=CARTESIAN_POINT('Ctrl Pts',(16.8785675462961,16.8374717941287,5.42481711384901));
#19592=CARTESIAN_POINT('Ctrl Pts',(16.4944006491489,17.1433203750861,5.40482778360432));
#19593=CARTESIAN_POINT('Ctrl Pts',(16.2745221682787,17.2576841962038,5.39588110972356));
#19594=CARTESIAN_POINT('Ctrl Pts',(15.797132339406,17.3985022762211,5.37499791510973));
#19595=CARTESIAN_POINT('Ctrl Pts',(15.5435308112421,17.4211183361773,5.36390423496259));
#19596=CARTESIAN_POINT('Ctrl Pts',(15.0516952055145,17.3673309276156,5.34238911660183));
#19597=CARTESIAN_POINT('Ctrl Pts',(14.8177104042985,17.2951059930202,5.33215356099309));
#19598=CARTESIAN_POINT('Ctrl Pts',(14.3788806946875,17.0610762316894,5.31295716074765));
#19599=CARTESIAN_POINT('Ctrl Pts',(14.1804521716289,16.8973909286625,5.30274375017752));
#19600=CARTESIAN_POINT('Ctrl Pts',(13.8633108982278,16.506105803706,5.28098375476911));
#19601=CARTESIAN_POINT('Ctrl Pts',(13.7459758639615,16.2838384426846,5.26999702256394));
#19602=CARTESIAN_POINT('Ctrl Pts',(13.6217634454933,15.8680622081078,5.25152900022502));
#19603=CARTESIAN_POINT('Ctrl Pts',(13.595,15.6843757766305,5.24398486904657));
#19604=CARTESIAN_POINT('Ctrl Pts',(13.595,15.4999999999999,5.23699999999999));
#19605=CARTESIAN_POINT('Origin',(15.5,15.5,-1.713));
#19606=CARTESIAN_POINT('',(13.595,15.4999999999999,4.67449999999982));
#19607=CARTESIAN_POINT('',(13.595,15.5,4.73699999999999));
#19608=CARTESIAN_POINT('',(13.595,15.5,-1.713));
#19609=CARTESIAN_POINT('Ctrl Pts',(13.595,15.4999999999999,4.67449999999982));
#19610=CARTESIAN_POINT('Ctrl Pts',(13.595,15.693650091279,4.68183621603188));
#19611=CARTESIAN_POINT('Ctrl Pts',(13.6245240457925,15.8864371338263,4.6897854942148));
#19612=CARTESIAN_POINT('Ctrl Pts',(13.7576295137902,16.309524273011,4.70872499310137));
#19613=CARTESIAN_POINT('Ctrl Pts',(13.8784159600935,16.5303628765405,4.71973308863698));
#19614=CARTESIAN_POINT('Ctrl Pts',(14.2008185419825,16.9161133260124,4.74139848582457));
#19615=CARTESIAN_POINT('Ctrl Pts',(14.4004879063477,17.076162988088,4.75140235810768));
#19616=CARTESIAN_POINT('Ctrl Pts',(14.8414739820042,17.3040010959973,4.77069308757649));
#19617=CARTESIAN_POINT('Ctrl Pts',(15.0767072907508,17.3731999162084,4.7809832585628));
#19618=CARTESIAN_POINT('Ctrl Pts',(15.5698897955118,17.420386369048,4.80255729639139));
#19619=CARTESIAN_POINT('Ctrl Pts',(15.8235167409559,17.3942318988719,4.81365208840559));
#19620=CARTESIAN_POINT('Ctrl Pts',(16.298532950826,17.246806760591,4.83443145016721));
#19621=CARTESIAN_POINT('Ctrl Pts',(16.5161993929083,17.1298236291038,4.84331588057563));
#19622=CARTESIAN_POINT('Ctrl Pts',(16.8960583609061,16.8192632403375,4.86338948819069));
#19623=CARTESIAN_POINT('Ctrl Pts',(17.0544365648767,16.6283384286404,4.87408655026979));
#19624=CARTESIAN_POINT('Ctrl Pts',(17.2930980298608,16.1910451586717,4.89587298129296));
#19625=CARTESIAN_POINT('Ctrl Pts',(17.3687982653089,15.9476117971498,4.90675091624183));
#19626=CARTESIAN_POINT('Ctrl Pts',(17.4197225373191,15.4565367215639,4.92646857269976));
#19627=CARTESIAN_POINT('Ctrl Pts',(17.39880485994,15.2140373938938,4.93546887364174));
#19628=CARTESIAN_POINT('Ctrl Pts',(17.2655724451835,14.7426541640862,4.95624079224673));
#19629=CARTESIAN_POINT('Ctrl Pts',(17.15178954068,14.5189773017227,4.96720322869893));
#19630=CARTESIAN_POINT('Ctrl Pts',(16.8423837032947,14.1249579111728,4.98889761717191));
#19631=CARTESIAN_POINT('Ctrl Pts',(16.6486204803811,13.9594307097668,4.99925413471649));
#19632=CARTESIAN_POINT('Ctrl Pts',(16.2167685356687,13.7184426840639,5.0181452959025));
#19633=CARTESIAN_POINT('Ctrl Pts',(15.9846754599108,13.6418370567856,5.02829809886653));
#19634=CARTESIAN_POINT('Ctrl Pts',(15.4949609663296,13.5784622021334,5.04972043016928));
#19635=CARTESIAN_POINT('Ctrl Pts',(15.2414820619885,13.5959234565942,5.06080874619469));
#19636=CARTESIAN_POINT('Ctrl Pts',(14.7606910573368,13.7270579892792,5.08184072365098));
#19637=CARTESIAN_POINT('Ctrl Pts',(14.5375531120099,13.8375948904197,5.09090587872771));
#19638=CARTESIAN_POINT('Ctrl Pts',(14.1471662310465,14.1365864779329,5.11077148462383));
#19639=CARTESIAN_POINT('Ctrl Pts',(13.983219344328,14.3216893814352,5.1213697899653));
#19640=CARTESIAN_POINT('Ctrl Pts',(13.7294756616269,14.7522208894023,5.14322994151294));
#19641=CARTESIAN_POINT('Ctrl Pts',(13.645443790657,14.9954521834583,5.15428245311104));
#19642=CARTESIAN_POINT('Ctrl Pts',(13.6005693043702,15.3317165368294,5.16800295685337));
#19643=CARTESIAN_POINT('Ctrl Pts',(13.595,15.4158954773162,5.17131379469724));
#19644=CARTESIAN_POINT('Ctrl Pts',(13.595,15.4999999999999,5.17449999999983));
#19645=CARTESIAN_POINT('Ctrl Pts',(13.595,15.4999999999999,5.23699999999999));
#19646=CARTESIAN_POINT('Ctrl Pts',(13.595,15.4440288618566,5.23487959634685));
#19647=CARTESIAN_POINT('Ctrl Pts',(13.5974666521958,15.3879982888102,5.23270298979645));
#19648=CARTESIAN_POINT('Ctrl Pts',(13.6246703649183,15.0806012568895,5.22046259193762));
#19649=CARTESIAN_POINT('Ctrl Pts',(13.696688705695,14.8360689879445,5.2096235574958));
#19650=CARTESIAN_POINT('Ctrl Pts',(13.9288851203419,14.3949234747567,5.18783259386893));
#19651=CARTESIAN_POINT('Ctrl Pts',(14.0846482983729,14.2013898445396,5.17709389617555));
#19652=CARTESIAN_POINT('Ctrl Pts',(14.4596738194808,13.8855790715094,5.15692710209035));
#19653=CARTESIAN_POINT('Ctrl Pts',(14.6749021791709,13.7656850727794,5.14809351797152));
#19654=CARTESIAN_POINT('Ctrl Pts',(15.1472402509199,13.6109424793995,5.12743131010844));
#19655=CARTESIAN_POINT('Ctrl Pts',(15.4008394411745,13.58085061349,5.11633773223203));
#19656=CARTESIAN_POINT('Ctrl Pts',(15.8954167028646,13.6206728956279,5.09470268141442));
#19657=CARTESIAN_POINT('Ctrl Pts',(16.1319915940397,13.6864862114627,5.08435382353274));
#19658=CARTESIAN_POINT('Ctrl Pts',(16.5753408034579,13.9074616597123,5.06495971988364));
#19659=CARTESIAN_POINT('Ctrl Pts',(16.7763697576834,14.0635313609246,5.05516856755623));
#19660=CARTESIAN_POINT('Ctrl Pts',(17.1045107759233,14.443150998749,5.03360991667034));
#19661=CARTESIAN_POINT('Ctrl Pts',(17.2290846024511,14.6623534917871,5.02258096475398));
#19662=CARTESIAN_POINT('Ctrl Pts',(17.3838445618186,15.1281353737474,5.00155039073458));
#19663=CARTESIAN_POINT('Ctrl Pts',(17.4157337528869,15.3692601144926,4.99218770509971));
#19664=CARTESIAN_POINT('Ctrl Pts',(17.3872640267862,15.8619047995735,4.97290171755076));
#19665=CARTESIAN_POINT('Ctrl Pts',(17.3227610517695,16.1084897777251,4.9621492966068));
#19666=CARTESIAN_POINT('Ctrl Pts',(17.1038653885543,16.5571518054196,4.94036449584985));
#19667=CARTESIAN_POINT('Ctrl Pts',(16.9535335352168,16.7558681228355,4.92954825325593));
#19668=CARTESIAN_POINT('Ctrl Pts',(16.5883501587876,17.0822549849342,4.90919606593078));
#19669=CARTESIAN_POINT('Ctrl Pts',(16.3779502270845,17.2079927184403,4.90040552174481));
#19670=CARTESIAN_POINT('Ctrl Pts',(15.9111037107944,17.3773323556364,4.87998353940493));
#19671=CARTESIAN_POINT('Ctrl Pts',(15.6577379712513,17.415329839683,4.86890017372065));
#19672=CARTESIAN_POINT('Ctrl Pts',(15.1606900201998,17.3903533744672,4.84715704375341));
#19673=CARTESIAN_POINT('Ctrl Pts',(14.921572710822,17.3313950924429,4.83669696897749));
#19674=CARTESIAN_POINT('Ctrl Pts',(14.4735875094848,17.1241250736244,4.81710006603188));
#19675=CARTESIAN_POINT('Ctrl Pts',(14.2698827973726,16.9758494372357,4.80767211301389));
#19676=CARTESIAN_POINT('Ctrl Pts',(13.9305664816617,16.6084525263448,4.78633207732014));
#19677=CARTESIAN_POINT('Ctrl Pts',(13.7985548407317,16.3926761471158,4.77527023801942));
#19678=CARTESIAN_POINT('Ctrl Pts',(13.6345793555488,15.9468176951894,4.75479287631985));
#19679=CARTESIAN_POINT('Ctrl Pts',(13.595,15.7242052404364,4.74549376351178));
#19680=CARTESIAN_POINT('Ctrl Pts',(13.595,15.5,4.73699999999999));
#19681=CARTESIAN_POINT('Origin',(15.5,15.5,-1.713));
#19682=CARTESIAN_POINT('',(13.595,15.5,4.17449999999982));
#19683=CARTESIAN_POINT('',(13.595,15.5,4.23699999999999));
#19684=CARTESIAN_POINT('',(13.595,15.5,-1.713));
#19685=CARTESIAN_POINT('Ctrl Pts',(13.595,15.5,4.17449999999982));
#19686=CARTESIAN_POINT('Ctrl Pts',(13.595,15.734025771486,4.18336580329146));
#19687=CARTESIAN_POINT('Ctrl Pts',(13.6381242017143,15.9661696128238,4.19310353578431));
#19688=CARTESIAN_POINT('Ctrl Pts',(13.812515122304,16.4188995454661,4.21406902498013));
#19689=CARTESIAN_POINT('Ctrl Pts',(13.9480839527807,16.6329350332865,4.22514271636255));
#19690=CARTESIAN_POINT('Ctrl Pts',(14.2927068659157,16.9943964157289,4.24637395854319));
#19691=CARTESIAN_POINT('Ctrl Pts',(14.4976998188631,17.1389510152929,4.25565484771903));
#19692=CARTESIAN_POINT('Ctrl Pts',(14.9479020883219,17.3395491284113,4.27534873527192));
#19693=CARTESIAN_POINT('Ctrl Pts',(15.1881891966758,17.3951277348535,4.28585998235654));
#19694=CARTESIAN_POINT('Ctrl Pts',(15.6862853454185,17.4128162501582,4.3076489652412));
#19695=CARTESIAN_POINT('Ctrl Pts',(15.9394507336502,17.3709532407305,4.31872356665118));
#19696=CARTESIAN_POINT('Ctrl Pts',(16.4035567965287,17.1945153901765,4.33902566913932));
#19697=CARTESIAN_POINT('Ctrl Pts',(16.6116260315229,17.0659142210648,4.34782421348068));
#19698=CARTESIAN_POINT('Ctrl Pts',(16.9719236784538,16.7343346544246,4.36826625860546));
#19699=CARTESIAN_POINT('Ctrl Pts',(17.1195095894967,16.5331122239924,4.3791173824938));
#19700=CARTESIAN_POINT('Ctrl Pts',(17.3317425178926,16.0808845130844,4.40089153604325));
#19701=CARTESIAN_POINT('Ctrl Pts',(17.3925100159836,15.8333727489235,4.41159736388861));
#19702=CARTESIAN_POINT('Ctrl Pts',(17.4135469652281,15.3402855648001,4.43073754334417));
#19703=CARTESIAN_POINT('Ctrl Pts',(17.3779934553216,15.0995715038687,4.44026047779474));
#19704=CARTESIAN_POINT('Ctrl Pts',(17.2159943844446,14.635742480553,4.46137540573186));
#19705=CARTESIAN_POINT('Ctrl Pts',(17.0878282845223,14.41815902733,4.47242159330383));
#19706=CARTESIAN_POINT('Ctrl Pts',(16.7542753674769,14.0444116901943,4.49387614916905));
#19707=CARTESIAN_POINT('Ctrl Pts',(16.5519560555435,13.8921093194543,4.50348267473561));
#19708=CARTESIAN_POINT('Ctrl Pts',(16.1063673649305,13.6777137212781,4.52297474344133));
#19709=CARTESIAN_POINT('Ctrl Pts',(15.8685487957529,13.6151762789497,4.5333780054351));
#19710=CARTESIAN_POINT('Ctrl Pts',(15.3727325401662,13.5824592590899,4.55506725546075));
#19711=CARTESIAN_POINT('Ctrl Pts',(15.1192156632405,13.6163400777149,4.56615723257909));
#19712=CARTESIAN_POINT('Ctrl Pts',(14.6494911983603,13.778093083205,4.58670510943296));
#19713=CARTESIAN_POINT('Ctrl Pts',(14.4365866050679,13.9007875242667,4.59550822692166));
#19714=CARTESIAN_POINT('Ctrl Pts',(14.0662546981211,14.2216601832908,4.61576412489049));
#19715=CARTESIAN_POINT('Ctrl Pts',(13.9130640951453,14.4176871387399,4.62654101136175));
#19716=CARTESIAN_POINT('Ctrl Pts',(13.6871884480189,14.8624720373025,4.64833159950425));
#19717=CARTESIAN_POINT('Ctrl Pts',(13.6187513842615,15.1080140819445,4.65913055751981));
#19718=CARTESIAN_POINT('Ctrl Pts',(13.5967192885175,15.4064955285285,4.67092008346784));
#19719=CARTESIAN_POINT('Ctrl Pts',(13.595,15.4532714716672,4.67272974223003));
#19720=CARTESIAN_POINT('Ctrl Pts',(13.595,15.4999999999999,4.67449999999982));
#19721=CARTESIAN_POINT('Ctrl Pts',(13.595,15.5,4.73699999999999));
#19722=CARTESIAN_POINT('Ctrl Pts',(13.595,15.4831619553197,4.7363621096044));
#19723=CARTESIAN_POINT('Ctrl Pts',(13.5952232431582,15.4663152912995,4.7357190098412));
#19724=CARTESIAN_POINT('Ctrl Pts',(13.6023655458863,15.1971724622401,4.72536661795248));
#19725=CARTESIAN_POINT('Ctrl Pts',(13.6591298149792,14.9487353487148,4.71471329397599));
#19726=CARTESIAN_POINT('Ctrl Pts',(13.8641846941326,14.492810121388,4.69295606437544));
#19727=CARTESIAN_POINT('Ctrl Pts',(14.0087939561605,14.2889526851148,4.68207022231169));
#19728=CARTESIAN_POINT('Ctrl Pts',(14.3638555614543,13.9518516272429,4.66153352579343));
#19729=CARTESIAN_POINT('Ctrl Pts',(14.5694758198165,13.8202059240749,4.65270534471494));
#19730=CARTESIAN_POINT('Ctrl Pts',(15.0306371499171,13.6362685867437,4.63253205818381));
#19731=CARTESIAN_POINT('Ctrl Pts',(15.2835284644135,13.5903088851982,4.62146944600111));
#19732=CARTESIAN_POINT('Ctrl Pts',(15.7826210477588,13.6002529304787,4.59963687455116));
#19733=CARTESIAN_POINT('Ctrl Pts',(16.0240954015147,13.6522298508273,4.58907369197216));
#19734=CARTESIAN_POINT('Ctrl Pts',(16.4766136948028,13.8457736790557,4.56927849104091));
#19735=CARTESIAN_POINT('Ctrl Pts',(16.6829617157418,13.9864450034406,4.56013194309592));
#19736=CARTESIAN_POINT('Ctrl Pts',(17.0331029063219,14.3416440342871,4.5390172458342));
#19737=CARTESIAN_POINT('Ctrl Pts',(17.1723855710743,14.5537894077969,4.52793392933678));
#19738=CARTESIAN_POINT('Ctrl Pts',(17.3570411132624,15.0111720821459,4.50656766571775));
#19739=CARTESIAN_POINT('Ctrl Pts',(17.4040616127429,15.250744692468,4.4964632818013));
#19740=CARTESIAN_POINT('Ctrl Pts',(17.4059498803602,15.7449854401353,4.47769822594508));
#19741=CARTESIAN_POINT('Ctrl Pts',(17.3567950913128,15.9950099762399,4.46719275289177));
#19742=CARTESIAN_POINT('Ctrl Pts',(17.1653922803363,16.4576815526093,4.44547854710732));
#19743=CARTESIAN_POINT('Ctrl Pts',(17.0265119247938,16.6663842353441,4.43453445249414));
#19744=CARTESIAN_POINT('Ctrl Pts',(16.6813718542421,17.0138234716047,4.41382311215519));
#19745=CARTESIAN_POINT('Ctrl Pts',(16.4802586289945,17.1511769420762,4.40488095489924));
#19746=CARTESIAN_POINT('Ctrl Pts',(16.0272739253252,17.3479041534575,4.38506535106421));
#19747=CARTESIAN_POINT('Ctrl Pts',(15.7780157251603,17.4014353388329,4.37416166776742));
#19748=CARTESIAN_POINT('Ctrl Pts',(15.2801185049117,17.4081274237639,4.35238138691667));
#19749=CARTESIAN_POINT('Ctrl Pts',(15.0362808427617,17.3639413217721,4.34171482251817));
#19750=CARTESIAN_POINT('Ctrl Pts',(14.5789072455624,17.1854806004968,4.32170722858996));
#19751=CARTESIAN_POINT('Ctrl Pts',(14.3696752470818,17.0529411363222,4.31277533237892));
#19752=CARTESIAN_POINT('Ctrl Pts',(14.0080442480033,16.7110760491522,4.29191446843773));
#19753=CARTESIAN_POINT('Ctrl Pts',(13.8609901516845,16.5031329336648,4.28082037094368));
#19754=CARTESIAN_POINT('Ctrl Pts',(13.6602695809877,16.0507512667193,4.25929218629232));
#19755=CARTESIAN_POINT('Ctrl Pts',(13.6051237015921,15.8120917324614,4.24904467276561));
#19756=CARTESIAN_POINT('Ctrl Pts',(13.5954220493531,15.5463200269535,4.23876401333006));
#19757=CARTESIAN_POINT('Ctrl Pts',(13.595,15.5231518125555,4.23787708039442));
#19758=CARTESIAN_POINT('Ctrl Pts',(13.595,15.5,4.23699999999999));
#19759=CARTESIAN_POINT('Origin',(15.5,15.5,-1.713));
#19760=CARTESIAN_POINT('',(13.595,15.5,3.67449999999982));
#19761=CARTESIAN_POINT('',(13.595,15.5000000000001,3.73699999999998));
#19762=CARTESIAN_POINT('',(13.595,15.5,-1.713));
#19763=CARTESIAN_POINT('Ctrl Pts',(13.595,15.5000000000001,3.67449999999982));
#19764=CARTESIAN_POINT('Ctrl Pts',(13.595,15.5315708493142,3.67569602613827));
#19765=CARTESIAN_POINT('Ctrl Pts',(13.5957848075677,15.5631695708928,3.67691027370593));
#19766=CARTESIAN_POINT('Ctrl Pts',(13.6094509573792,15.8375445965614,3.68760357280036));
#19767=CARTESIAN_POINT('Ctrl Pts',(13.6678982376643,16.0757547526509,3.69790627125859));
#19768=CARTESIAN_POINT('Ctrl Pts',(13.8751161890635,16.5259447952251,3.71949354112295));
#19769=CARTESIAN_POINT('Ctrl Pts',(14.0252969144295,16.7320999971229,3.73058829198247));
#19770=CARTESIAN_POINT('Ctrl Pts',(14.3915344309247,17.0685073425307,3.75134315048599));
#19771=CARTESIAN_POINT('Ctrl Pts',(14.601951052826,17.1977682735184,3.76021526915221));
#19772=CARTESIAN_POINT('Ctrl Pts',(15.0612830005563,17.3700262996204,3.7803085302078));
#19773=CARTESIAN_POINT('Ctrl Pts',(15.3060217793934,17.4109761507869,3.79101451353403));
#19774=CARTESIAN_POINT('Ctrl Pts',(15.804090800173,17.3974380449954,3.81280230971864));
#19775=CARTESIAN_POINT('Ctrl Pts',(16.0525785874332,17.340494181246,3.82367229166355));
#19776=CARTESIAN_POINT('Ctrl Pts',(16.5026503825806,17.1376503654255,3.84336047167876));
#19777=CARTESIAN_POINT('Ctrl Pts',(16.7017358152984,16.9976812351531,3.85238004861031));
#19778=CARTESIAN_POINT('Ctrl Pts',(17.0422872779096,16.6455161561091,3.8731700589377));
#19779=CARTESIAN_POINT('Ctrl Pts',(17.1784821282183,16.4346393801006,3.88413777854603));
#19780=CARTESIAN_POINT('Ctrl Pts',(17.3635397218247,15.9689971022106,3.90582574173643));
#19781=CARTESIAN_POINT('Ctrl Pts',(17.4092004324088,15.7182717232893,3.91613914814077));
#19782=CARTESIAN_POINT('Ctrl Pts',(17.4003710694834,15.2237194221972,3.93506782433103));
#19783=CARTESIAN_POINT('Ctrl Pts',(17.3498602599869,14.9845054896736,3.94523496113124));
#19784=CARTESIAN_POINT('Ctrl Pts',(17.1582910552894,14.5292027117347,3.96667364767794));
#19785=CARTESIAN_POINT('Ctrl Pts',(17.015656870939,14.3188280123367,3.97776318950503));
#19786=CARTESIAN_POINT('Ctrl Pts',(16.660552230454,13.9693401892086,3.99877008597855));
#19787=CARTESIAN_POINT('Ctrl Pts',(16.4529697003171,13.8321739172205,4.00781278651278));
#19788=CARTESIAN_POINT('Ctrl Pts',(15.9983593128666,13.6450791244421,4.0276995051239));
#19789=CARTESIAN_POINT('Ctrl Pts',(15.7558449606823,13.5964189325426,4.03830818194736));
#19790=CARTESIAN_POINT('Ctrl Pts',(15.2559430449784,13.5935867057772,4.06017615726248));
#19791=CARTESIAN_POINT('Ctrl Pts',(15.0033585050623,13.6432985756689,4.07122534973473));
#19792=CARTESIAN_POINT('Ctrl Pts',(14.5449308807844,13.8340871424297,4.09127905158412));
#19793=CARTESIAN_POINT('Ctrl Pts',(14.3415359755962,13.9685334120202,4.10015367637626));
#19794=CARTESIAN_POINT('Ctrl Pts',(13.9913260773587,14.3107103153903,4.12077654776842));
#19795=CARTESIAN_POINT('Ctrl Pts',(13.8495044196596,14.5169615480573,4.13169210489444));
#19796=CARTESIAN_POINT('Ctrl Pts',(13.6511313198597,14.9761977731424,4.15342862226806));
#19797=CARTESIAN_POINT('Ctrl Pts',(13.5980741954768,15.2254298346918,4.16403097830177));
#19798=CARTESIAN_POINT('Ctrl Pts',(13.5950432048621,15.4851832998888,4.17393774098282));
#19799=CARTESIAN_POINT('Ctrl Pts',(13.595,15.4925925572656,4.1742193773583));
#19800=CARTESIAN_POINT('Ctrl Pts',(13.595,15.5,4.17449999999982));
#19801=CARTESIAN_POINT('Ctrl Pts',(13.595,15.5,4.23699999999999));
#19802=CARTESIAN_POINT('Ctrl Pts',(13.595,15.2691971061883,4.22825629180628));
#19803=CARTESIAN_POINT('Ctrl Pts',(13.6369428485792,15.0400926775705,4.21865954291788));
#19804=CARTESIAN_POINT('Ctrl Pts',(13.8073918288257,14.5910901252192,4.19792148050212));
#19805=CARTESIAN_POINT('Ctrl Pts',(13.9405739255903,14.377844531064,4.18692991662784));
#19806=CARTESIAN_POINT('Ctrl Pts',(14.2760191032244,14.0204621113541,4.16605393923708));
#19807=CARTESIAN_POINT('Ctrl Pts',(14.4728882249431,13.8775982084076,4.15693052384329));
#19808=CARTESIAN_POINT('Ctrl Pts',(14.9197252436716,13.6680512453625,4.1373838476084));
#19809=CARTESIAN_POINT('Ctrl Pts',(15.1673108338374,13.6073689833216,4.1265533318531));
#19810=CARTESIAN_POINT('Ctrl Pts',(15.6654595231384,13.5862977508088,4.10476205060632));
#19811=CARTESIAN_POINT('Ctrl Pts',(15.911140189458,13.6236713128153,4.09401486485305));
#19812=CARTESIAN_POINT('Ctrl Pts',(16.372598461827,13.7891125043602,4.07382858872142));
#19813=CARTESIAN_POINT('Ctrl Pts',(16.584318487475,13.9148128026822,4.06500319942661));
#19814=CARTESIAN_POINT('Ctrl Pts',(16.9555414155677,14.2452414189295,4.04436579610842));
#19815=CARTESIAN_POINT('Ctrl Pts',(17.1091103920882,14.449394084336,4.03327280036245));
#19816=CARTESIAN_POINT('Ctrl Pts',(17.3233921437259,14.8970890954297,4.01162555064358));
#19817=CARTESIAN_POINT('Ctrl Pts',(17.3854386913095,15.1347574577275,4.00126465330248));
#19818=CARTESIAN_POINT('Ctrl Pts',(17.4172331534591,15.628903797461,3.98184905774384));
#19819=CARTESIAN_POINT('Ctrl Pts',(17.3834448089266,15.8808663522567,3.9720998454925));
#19820=CARTESIAN_POINT('Ctrl Pts',(17.2204610163731,16.3552431693938,3.95056378814853));
#19821=CARTESIAN_POINT('Ctrl Pts',(17.0936095846538,16.5732361235507,3.93953084186659));
#19822=CARTESIAN_POINT('Ctrl Pts',(16.7687702371492,16.9413129963823,3.91848169067809));
#19823=CARTESIAN_POINT('Ctrl Pts',(16.5763758116767,17.0901414674553,3.90908555606629));
#19824=CARTESIAN_POINT('Ctrl Pts',(16.1362270921317,17.3132715624607,3.88983145634868));
#19825=CARTESIAN_POINT('Ctrl Pts',(15.890655702729,17.381516306028,3.87908905086301));
#19826=CARTESIAN_POINT('Ctrl Pts',(15.3926987432721,17.4179362844291,3.85730615674856));
#19827=CARTESIAN_POINT('Ctrl Pts',(15.1452598980358,17.387899019869,3.84648206028155));
#19828=CARTESIAN_POINT('Ctrl Pts',(14.6795555871987,17.2363330912826,3.82611004318458));
#19829=CARTESIAN_POINT('Ctrl Pts',(14.4651755424473,17.1177510719111,3.81731939179786));
#19830=CARTESIAN_POINT('Ctrl Pts',(14.084044801387,16.7994221119836,3.79692366403812));
#19831=CARTESIAN_POINT('Ctrl Pts',(13.9237377365017,16.5994592092857,3.78584201548196));
#19832=CARTESIAN_POINT('Ctrl Pts',(13.6953359488009,16.1571086298419,3.76408839636438));
#19833=CARTESIAN_POINT('Ctrl Pts',(13.6260627817449,15.9206924627447,3.75361687448774));
#19834=CARTESIAN_POINT('Ctrl Pts',(13.597760005866,15.618479508341,3.74154883057672));
#19835=CARTESIAN_POINT('Ctrl Pts',(13.595,15.5592060680503,3.73924295533636));
#19836=CARTESIAN_POINT('Ctrl Pts',(13.595,15.5000000000001,3.73699999999998));
#19837=CARTESIAN_POINT('Origin',(15.5,15.5,-1.713));
#19838=CARTESIAN_POINT('',(13.595,15.5000000000001,3.17449999999981));
#19839=CARTESIAN_POINT('',(13.595,15.5,3.23699999999997));
#19840=CARTESIAN_POINT('',(13.595,15.5,-1.713));
#19841=CARTESIAN_POINT('Ctrl Pts',(13.595,15.5000000000001,3.17449999999981));
#19842=CARTESIAN_POINT('Ctrl Pts',(13.595,15.568249989465,3.177085574133));
#19843=CARTESIAN_POINT('Ctrl Pts',(13.5986675612602,15.6365760475214,3.17975424791452));
#19844=CARTESIAN_POINT('Ctrl Pts',(13.6322958131998,15.947741225573,3.19227791698431));
#19845=CARTESIAN_POINT('Ctrl Pts',(13.705104464663,16.1834642537271,3.20280050912647));
#19846=CARTESIAN_POINT('Ctrl Pts',(13.9403835379756,16.6230360937529,3.2245992806447));
#19847=CARTESIAN_POINT('Ctrl Pts',(14.1039553317352,16.8208663486228,3.23567154325336));
#19848=CARTESIAN_POINT('Ctrl Pts',(14.4898892604546,17.1332251253252,3.25594615393048));
#19849=CARTESIAN_POINT('Ctrl Pts',(14.7055970842692,17.2483348778709,3.26474921628444));
#19850=CARTESIAN_POINT('Ctrl Pts',(15.1733677361523,17.3930116831415,3.28521162450332));
#19851=CARTESIAN_POINT('Ctrl Pts',(15.4215992597164,17.4193817462098,3.29607039631279));
#19852=CARTESIAN_POINT('Ctrl Pts',(15.9192846661276,17.3753414100464,3.31784141146642));
#19853=CARTESIAN_POINT('Ctrl Pts',(16.1637685524579,17.3033692592156,3.32853624463924));
#19854=CARTESIAN_POINT('Ctrl Pts',(16.6005469044634,17.0735253401857,3.34764290920643));
#19855=CARTESIAN_POINT('Ctrl Pts',(16.7907360361107,16.9216959633891,3.35720530171909));
#19856=CARTESIAN_POINT('Ctrl Pts',(17.1102003271643,16.5482733681289,3.37833940492863));
#19857=CARTESIAN_POINT('Ctrl Pts',(17.2338102066998,16.3279646081025,3.38938918282134));
#19858=CARTESIAN_POINT('Ctrl Pts',(17.3889206611445,15.8518324907181,3.410819529997));
#19859=CARTESIAN_POINT('Ctrl Pts',(17.4187651327053,15.6006421711202,3.42038620983217));
#19860=CARTESIAN_POINT('Ctrl Pts',(17.3800740437233,15.1078674697106,3.43990068727113));
#19861=CARTESIAN_POINT('Ctrl Pts',(17.3145265316614,14.8707782405648,3.45031621882997));
#19862=CARTESIAN_POINT('Ctrl Pts',(17.093393792891,14.4256163350543,3.47201735130392));
#19863=CARTESIAN_POINT('Ctrl Pts',(16.9365496772127,14.2234651246719,3.48310615889079));
#19864=CARTESIAN_POINT('Ctrl Pts',(16.5605112283184,13.8988819668973,3.50362743993718));
#19865=CARTESIAN_POINT('Ctrl Pts',(16.3475097391379,13.7766339740126,3.51242608315226));
#19866=CARTESIAN_POINT('Ctrl Pts',(15.8839911682231,13.6178819280046,3.53270248607941));
#19867=CARTESIAN_POINT('Ctrl Pts',(15.637436117626,13.584036105808,3.54348792136362));
#19868=CARTESIAN_POINT('Ctrl Pts',(15.1393205736819,13.6125053812221,3.56527775268223));
#19869=CARTESIAN_POINT('Ctrl Pts',(14.8926763909184,13.6768418688357,3.57606708701133));
#19870=CARTESIAN_POINT('Ctrl Pts',(14.4490466142148,13.8929471500693,3.59547346394495));
#19871=CARTESIAN_POINT('Ctrl Pts',(14.2543404899168,14.0386737560065,3.60471802731944));
#19872=CARTESIAN_POINT('Ctrl Pts',(13.9239720590515,14.4011994334501,3.62567781129242));
#19873=CARTESIAN_POINT('Ctrl Pts',(13.7938087002647,14.6167467537565,3.63669054683468));
#19874=CARTESIAN_POINT('Ctrl Pts',(13.6334446299582,15.0594857800668,3.6569707427745));
#19875=CARTESIAN_POINT('Ctrl Pts',(13.595,15.2790287344985,3.66612875199322));
#19876=CARTESIAN_POINT('Ctrl Pts',(13.595,15.5000000000001,3.67449999999982));
#19877=CARTESIAN_POINT('Ctrl Pts',(13.595,15.5000000000001,3.73699999999998));
#19878=CARTESIAN_POINT('Ctrl Pts',(13.595,15.3107417523562,3.7298301640273));
#19879=CARTESIAN_POINT('Ctrl Pts',(13.6231998597127,15.1222187510603,3.72207138720419));
#19880=CARTESIAN_POINT('Ctrl Pts',(13.7525493543417,14.7010956562945,3.70328844558116));
#19881=CARTESIAN_POINT('Ctrl Pts',(13.8726887488314,14.4783897716366,3.69222376268828));
#19882=CARTESIAN_POINT('Ctrl Pts',(14.1864332416871,14.0993343465173,3.67100137099868));
#19883=CARTESIAN_POINT('Ctrl Pts',(14.3743188608229,13.9443260371385,3.66124239453956));
#19884=CARTESIAN_POINT('Ctrl Pts',(14.8075273411798,13.707459792369,3.64229189233668));
#19885=CARTESIAN_POINT('Ctrl Pts',(15.0508088855582,13.6315994557552,3.63164965504977));
#19886=CARTESIAN_POINT('Ctrl Pts',(15.5480838732381,13.5795702874817,3.60989659347145));
#19887=CARTESIAN_POINT('Ctrl Pts',(15.7970891607354,13.6020779774247,3.59900397372091));
#19888=CARTESIAN_POINT('Ctrl Pts',(16.266996803239,13.7395269848502,3.5784480838476));
#19889=CARTESIAN_POINT('Ctrl Pts',(16.4841055119923,13.8510363568198,3.56961118324191));
#19890=CARTESIAN_POINT('Ctrl Pts',(16.8749980751583,14.1571596683536,3.54946433958215));
#19891=CARTESIAN_POINT('Ctrl Pts',(17.0419363550534,14.3527181428317,3.53840450813985));
#19892=CARTESIAN_POINT('Ctrl Pts',(17.2843324468652,14.7892907094982,3.51656369539994));
#19893=CARTESIAN_POINT('Ctrl Pts',(17.3608108597669,15.0242378422134,3.5059902311861));
#19894=CARTESIAN_POINT('Ctrl Pts',(17.4209317256358,15.5125897526223,3.48617458843306));
#19895=CARTESIAN_POINT('Ctrl Pts',(17.4030963877,15.7614744775627,3.47705269701819));
#19896=CARTESIAN_POINT('Ctrl Pts',(17.2722116836178,16.2426311732042,3.45596187139847));
#19897=CARTESIAN_POINT('Ctrl Pts',(17.1588421845852,16.4697796343246,3.4448769594441));
#19898=CARTESIAN_POINT('Ctrl Pts',(16.8562303219055,16.8594962581601,3.42349417607325));
#19899=CARTESIAN_POINT('Ctrl Pts',(16.6727191440018,17.0206396007897,3.41337563638298));
#19900=CARTESIAN_POINT('Ctrl Pts',(16.2463442487807,17.2707735006488,3.39457380964476));
#19901=CARTESIAN_POINT('Ctrl Pts',(16.0054895868111,17.3539704573083,3.38411240537228));
#19902=CARTESIAN_POINT('Ctrl Pts',(15.5092285939096,17.4211032108309,3.36240370052097));
#19903=CARTESIAN_POINT('Ctrl Pts',(15.2589222384643,17.4059405573717,3.35145416616205));
#19904=CARTESIAN_POINT('Ctrl Pts',(14.7850580275298,17.2821722166527,3.3307251980547));
#19905=CARTESIAN_POINT('Ctrl Pts',(14.5652717116774,17.1773650722673,3.32176713122677));
#19906=CARTESIAN_POINT('Ctrl Pts',(14.167547187961,16.8846789705213,3.30197991069725));
#19907=CARTESIAN_POINT('Ctrl Pts',(13.9959811186205,16.6961082057814,3.29108358054212));
#19908=CARTESIAN_POINT('Ctrl Pts',(13.7398885692823,16.2689872877109,3.26930126032312));
#19909=CARTESIAN_POINT('Ctrl Pts',(13.6555080384971,16.0359080603258,3.25862572237898));
#19910=CARTESIAN_POINT('Ctrl Pts',(13.6025563404818,15.6959986001898,3.24459046094099));
#19911=CARTESIAN_POINT('Ctrl Pts',(13.595,15.5979667544917,3.2407113603725));
#19912=CARTESIAN_POINT('Ctrl Pts',(13.595,15.5,3.23699999999997));
#19913=CARTESIAN_POINT('Origin',(15.5,15.5,-1.713));
#19914=CARTESIAN_POINT('',(13.595,15.5,2.6744999999998));
#19915=CARTESIAN_POINT('',(13.595,15.5,2.73699999999996));
#19916=CARTESIAN_POINT('',(13.595,15.5,-1.713));
#19917=CARTESIAN_POINT('Ctrl Pts',(13.595,15.5,2.6744999999998));
#19918=CARTESIAN_POINT('Ctrl Pts',(13.595,15.6063456034545,2.67852878364688));
#19919=CARTESIAN_POINT('Ctrl Pts',(13.6039040754401,15.712737450423,2.68275407148365));
#19920=CARTESIAN_POINT('Ctrl Pts',(13.6628013387962,16.0605419293528,2.69721846982053));
#19921=CARTESIAN_POINT('Ctrl Pts',(13.7504283648582,16.2927748267109,2.70793295371105));
#19922=CARTESIAN_POINT('Ctrl Pts',(14.0125168018968,16.7166077868478,2.72972185699009));
#19923=CARTESIAN_POINT('Ctrl Pts',(14.1866415324471,16.9028008162696,2.74058407303392));
#19924=CARTESIAN_POINT('Ctrl Pts',(14.5881938303327,17.1899115237428,2.76024379811324));
#19925=CARTESIAN_POINT('Ctrl Pts',(14.809233833783,17.2916600718789,2.76928275738304));
#19926=CARTESIAN_POINT('Ctrl Pts',(15.2848913317403,17.4090895189284,2.79009017199187));
#19927=CARTESIAN_POINT('Ctrl Pts',(15.5357276212959,17.4208368072303,2.80106288807043));
#19928=CARTESIAN_POINT('Ctrl Pts',(16.0313680146098,17.3467242333267,2.82274444508332));
#19929=CARTESIAN_POINT('Ctrl Pts',(16.2710725586215,17.2601539276952,2.83301698439854));
#19930=CARTESIAN_POINT('Ctrl Pts',(16.6942270056888,17.0038614551219,2.85198168324288));
#19931=CARTESIAN_POINT('Ctrl Pts',(16.8756725561019,16.8398802310465,2.86216255292791));
#19932=CARTESIAN_POINT('Ctrl Pts',(17.1730083799238,16.4452310737242,2.88361680086033));
#19933=CARTESIAN_POINT('Ctrl Pts',(17.2831607273355,16.216074965942,2.89470740385587));
#19934=CARTESIAN_POINT('Ctrl Pts',(17.4066174506574,15.7334864081388,2.91569000719336));
#19935=CARTESIAN_POINT('Ctrl Pts',(17.420802952878,15.4852819804533,2.92471192923798));
#19936=CARTESIAN_POINT('Ctrl Pts',(17.35404340675,14.9983496347111,2.94461899635966));
#19937=CARTESIAN_POINT('Ctrl Pts',(17.2741679649323,14.7641723259516,2.95523759737822));
#19938=CARTESIAN_POINT('Ctrl Pts',(17.0252033879657,14.3304812783692,2.97711291466097));
#19939=CARTESIAN_POINT('Ctrl Pts',(16.8551691352643,14.1370789335407,2.98815877949576));
#19940=CARTESIAN_POINT('Ctrl Pts',(16.4597082538015,13.8367647917469,3.00818546876262));
#19941=CARTESIAN_POINT('Ctrl Pts',(16.2412799892886,13.7285875958632,3.01707305383682));
#19942=CARTESIAN_POINT('Ctrl Pts',(15.769401181861,13.5979038735229,3.03771517139708));
#19943=CARTESIAN_POINT('Ctrl Pts',(15.5197256729543,13.5790233888131,3.04863710966946));
#19944=CARTESIAN_POINT('Ctrl Pts',(15.0229509050475,13.6385205832759,3.07036828936789));
#19945=CARTESIAN_POINT('Ctrl Pts',(14.780850944374,13.7179975568388,3.08095883882865));
#19946=CARTESIAN_POINT('Ctrl Pts',(14.3510143352543,13.9614169703243,3.09976184010243));
#19947=CARTESIAN_POINT('Ctrl Pts',(14.1652766286123,14.1194307028667,3.10972544193732));
#19948=CARTESIAN_POINT('Ctrl Pts',(13.8569625944506,14.5037801398521,3.13102961487869));
#19949=CARTESIAN_POINT('Ctrl Pts',(13.7401357188322,14.7286974836181,3.14210562412025));
#19950=CARTESIAN_POINT('Ctrl Pts',(13.6202437330165,15.1424359669405,3.16040195089137));
#19951=CARTESIAN_POINT('Ctrl Pts',(13.595,15.3209351345322,3.16771632885281));
#19952=CARTESIAN_POINT('Ctrl Pts',(13.595,15.5000000000001,3.17449999999981));
#19953=CARTESIAN_POINT('Ctrl Pts',(13.595,15.5,3.23699999999997));
#19954=CARTESIAN_POINT('Ctrl Pts',(13.595,15.3537934880559,3.23146113064115));
#19955=CARTESIAN_POINT('Ctrl Pts',(13.6118292995507,15.2077601688887,3.22556072758023));
#19956=CARTESIAN_POINT('Ctrl Pts',(13.703020040462,14.8191615490059,3.20884455753866));
#19957=CARTESIAN_POINT('Ctrl Pts',(13.8088818890257,14.5874272503676,3.19775012561254));
#19958=CARTESIAN_POINT('Ctrl Pts',(14.0991475865153,14.186385786418,3.17620835201251));
#19959=CARTESIAN_POINT('Ctrl Pts',(14.2778058056202,14.0187054927708,3.16594831248646));
#19960=CARTESIAN_POINT('Ctrl Pts',(14.6979924612101,13.7534727151105,3.14670983255795));
#19961=CARTESIAN_POINT('Ctrl Pts',(14.9378342582387,13.6621805869591,3.13659167724224));
#19962=CARTESIAN_POINT('Ctrl Pts',(15.4343106839288,13.5799046605583,3.11487354838438));
#19963=CARTESIAN_POINT('Ctrl Pts',(15.6856914399172,13.587775485027,3.10387701487657));
#19964=CARTESIAN_POINT('Ctrl Pts',(16.1633494669556,13.6980228775345,3.08298208805948));
#19965=CARTESIAN_POINT('Ctrl Pts',(16.3858207901989,13.7963394742754,3.07383302272958));
#19966=CARTESIAN_POINT('Ctrl Pts',(16.7916343681647,14.0771739162689,3.05431786306173));
#19967=CARTESIAN_POINT('Ctrl Pts',(16.9685906134332,14.2606558327297,3.04349642284193));
#19968=CARTESIAN_POINT('Ctrl Pts',(17.2373587916645,14.6806975070553,3.02170504708823));
#19969=CARTESIAN_POINT('Ctrl Pts',(17.3286210834497,14.911927493209,3.01094904586258));
#19970=CARTESIAN_POINT('Ctrl Pts',(17.4176138080143,15.3939327184791,2.99074234716955));
#19971=CARTESIAN_POINT('Ctrl Pts',(17.415435860485,15.6399968762604,2.98192463162497));
#19972=CARTESIAN_POINT('Ctrl Pts',(17.3165773094733,16.1269857163728,2.96131334630555));
#19973=CARTESIAN_POINT('Ctrl Pts',(17.2173200906876,16.3624759378803,2.95022108368259));
#19974=CARTESIAN_POINT('Ctrl Pts',(16.9380102219418,16.7729589921194,2.92856125484767));
#19975=CARTESIAN_POINT('Ctrl Pts',(16.7637123739558,16.9461498976184,2.91818782318278));
#19976=CARTESIAN_POINT('Ctrl Pts',(16.3527147432174,17.2219567273831,2.89874974197185));
#19977=CARTESIAN_POINT('Ctrl Pts',(16.1182155734959,17.3193652589469,2.88904355089655));
#19978=CARTESIAN_POINT('Ctrl Pts',(15.626445026524,17.4171549396238,2.86753127850061));
#19979=CARTESIAN_POINT('Ctrl Pts',(15.3741392554428,17.4171933827677,2.85649428064055));
#19980=CARTESIAN_POINT('Ctrl Pts',(14.8925123198339,17.3215733653222,2.83542573577579));
#19981=CARTESIAN_POINT('Ctrl Pts',(14.6670879670194,17.2301446596474,2.82599357878335));
#19982=CARTESIAN_POINT('Ctrl Pts',(14.2528348239649,16.9619561037788,2.80677290188424));
#19983=CARTESIAN_POINT('Ctrl Pts',(14.0703326623383,16.7840422422845,2.79604109941036));
#19984=CARTESIAN_POINT('Ctrl Pts',(13.7883374842567,16.3719205442741,2.77426045859807));
#19985=CARTESIAN_POINT('Ctrl Pts',(13.6898170858119,16.1428698537008,2.76342826629651));
#19986=CARTESIAN_POINT('Ctrl Pts',(13.6092718154206,15.7691888526544,2.74751007403869));
#19987=CARTESIAN_POINT('Ctrl Pts',(13.595,15.6346391293541,2.74210065207189));
#19988=CARTESIAN_POINT('Ctrl Pts',(13.595,15.5,2.73699999999996));
#19989=CARTESIAN_POINT('Origin',(15.5,15.5,-1.713));
#19990=CARTESIAN_POINT('',(13.595,15.5,2.1744999999998));
#19991=CARTESIAN_POINT('',(13.595,15.5,2.23699999999995));
#19992=CARTESIAN_POINT('',(13.595,15.5,-1.713));
#19993=CARTESIAN_POINT('Ctrl Pts',(13.595,15.5,2.1744999999998));
#19994=CARTESIAN_POINT('Ctrl Pts',(13.595,15.6438717177873,2.17995041830644));
#19995=CARTESIAN_POINT('Ctrl Pts',(13.6112960890959,15.7875810170524,2.18575111596478));
#19996=CARTESIAN_POINT('Ctrl Pts',(13.6994181942645,16.1694219103305,2.20214415911293));
#19997=CARTESIAN_POINT('Ctrl Pts',(13.8014664402575,16.39732693886,2.21301011131559));
#19998=CARTESIAN_POINT('Ctrl Pts',(14.0898370033197,16.805428282584,2.23477788964081));
#19999=CARTESIAN_POINT('Ctrl Pts',(14.2749823259478,16.9805603547105,2.24546211907182));
#20000=CARTESIAN_POINT('Ctrl Pts',(14.6933096159863,17.2425418310181,2.26453675856539));
#20001=CARTESIAN_POINT('Ctrl Pts',(14.9202192490859,17.3305984944438,2.2741377624269));
#20002=CARTESIAN_POINT('Ctrl Pts',(15.4037619976461,17.4189587852763,2.29529011363254));
#20003=CARTESIAN_POINT('Ctrl Pts',(15.6564353891663,17.4149918847535,2.30634319287666));
#20004=CARTESIAN_POINT('Ctrl Pts',(16.1458020926397,17.3095906453332,2.32775031026398));
#20005=CARTESIAN_POINT('Ctrl Pts',(16.3776914452839,17.2091865162443,2.33727982413664));
#20006=CARTESIAN_POINT('Ctrl Pts',(16.7840902788011,16.9281437430753,2.35681567706199));
#20007=CARTESIAN_POINT('Ctrl Pts',(16.9561453578496,16.7522394033176,2.36724284969501));
#20008=CARTESIAN_POINT('Ctrl Pts',(17.2298657636766,16.3371446453742,2.38895513352139));
#20009=CARTESIAN_POINT('Ctrl Pts',(17.3257728014476,16.0998440762515,2.40004270307863));
#20010=CARTESIAN_POINT('Ctrl Pts',(17.4172222954957,15.6116271944855,2.42053845851129));
#20011=CARTESIAN_POINT('Ctrl Pts',(17.4158006733317,15.3661710612252,2.42933372371272));
#20012=CARTESIAN_POINT('Ctrl Pts',(17.320031940749,14.8857206145777,2.44962972801491));
#20013=CARTESIAN_POINT('Ctrl Pts',(17.2253022083536,14.6555021357188,2.46042325020695));
#20014=CARTESIAN_POINT('Ctrl Pts',(16.9501966716434,14.2391854988472,2.48221211949409));
#20015=CARTESIAN_POINT('Ctrl Pts',(16.7705729717939,14.0583377226447,2.49299211154719));
#20016=CARTESIAN_POINT('Ctrl Pts',(16.3607170029023,13.7835246991033,2.51236757279492));
#20017=CARTESIAN_POINT('Ctrl Pts',(16.1368514548924,13.6884915883818,2.52164123119447));
#20018=CARTESIAN_POINT('Ctrl Pts',(15.6572929705878,13.585182428074,2.5426192926251));
#20019=CARTESIAN_POINT('Ctrl Pts',(15.4054427164359,13.5810615146841,2.55363636411031));
#20020=CARTESIAN_POINT('Ctrl Pts',(14.9111746682304,13.67072563478,2.57525788852872));
#20021=CARTESIAN_POINT('Ctrl Pts',(14.6738807357029,13.7649330778004,2.58517137358941));
#20022=CARTESIAN_POINT('Ctrl Pts',(14.2580399017547,14.0351855492971,2.60450496600958));
#20023=CARTESIAN_POINT('Ctrl Pts',(14.0814234721209,14.205486405278,2.61481962403155));
#20024=CARTESIAN_POINT('Ctrl Pts',(13.7963031328522,14.6110302058985,2.63641942295186));
#20025=CARTESIAN_POINT('Ctrl Pts',(13.6935495615298,14.8445635980581,2.64751402644718));
#20026=CARTESIAN_POINT('Ctrl Pts',(13.6098017218543,15.2258696997939,2.66379113452061));
#20027=CARTESIAN_POINT('Ctrl Pts',(13.595,15.3628839986378,2.66930551441603));
#20028=CARTESIAN_POINT('Ctrl Pts',(13.595,15.5,2.6744999999998));
#20029=CARTESIAN_POINT('Ctrl Pts',(13.595,15.5,2.73699999999997));
#20030=CARTESIAN_POINT('Ctrl Pts',(13.595,15.3930282082835,2.73294749391445));
#20031=CARTESIAN_POINT('Ctrl Pts',(13.6040092351669,15.2860150896782,2.7286963698185));
#20032=CARTESIAN_POINT('Ctrl Pts',(13.6646854787885,14.9298303122742,2.71387558296442));
#20033=CARTESIAN_POINT('Ctrl Pts',(13.7569133947645,14.6906125998951,2.70279585532033));
#20034=CARTESIAN_POINT('Ctrl Pts',(14.0244715433773,14.2705861319543,2.68103152173303));
#20035=CARTESIAN_POINT('Ctrl Pts',(14.1940405065733,14.0917631521739,2.67054815669065));
#20036=CARTESIAN_POINT('Ctrl Pts',(14.5954328728501,13.8050617550424,2.65090743594019));
#20037=CARTESIAN_POINT('Ctrl Pts',(14.8245298971626,13.7014420434005,2.64154812348355));
#20038=CARTESIAN_POINT('Ctrl Pts',(15.3112471846211,13.5878678116446,2.6202569035597));
#20039=CARTESIAN_POINT('Ctrl Pts',(15.5642504683678,13.5796494726171,2.60918939333455));
#20040=CARTESIAN_POINT('Ctrl Pts',(16.0498253014062,13.6601516696882,2.58794814954459));
#20041=CARTESIAN_POINT('Ctrl Pts',(16.2783576488718,13.7445899106109,2.57814395918767));
#20042=CARTESIAN_POINT('Ctrl Pts',(16.7010127006999,13.9999050425915,2.55922720869861));
#20043=CARTESIAN_POINT('Ctrl Pts',(16.8889380307444,14.1720159053704,2.54859662932607));
#20044=CARTESIAN_POINT('Ctrl Pts',(17.1840673178039,14.5757054590094,2.52684815810019));
#20045=CARTESIAN_POINT('Ctrl Pts',(17.2898773392592,14.802325578808,2.51594860466704));
#20046=CARTESIAN_POINT('Ctrl Pts',(17.407369479363,15.2776195184105,2.495372808691));
#20047=CARTESIAN_POINT('Ctrl Pts',(17.4201702625757,15.5212734828779,2.4865258860317));
#20048=CARTESIAN_POINT('Ctrl Pts',(17.35219055494,16.0131036479769,2.4664065828322));
#20049=CARTESIAN_POINT('Ctrl Pts',(17.2670854108525,16.2558290618805,2.45534976101996));
#20050=CARTESIAN_POINT('Ctrl Pts',(17.011526099875,16.685021789749,2.43350061574692));
#20051=CARTESIAN_POINT('Ctrl Pts',(16.8468366025359,16.8693193346392,2.42291657793418));
#20052=CARTESIAN_POINT('Ctrl Pts',(16.4550191957345,17.1667248449986,2.40307976994657));
#20053=CARTESIAN_POINT('Ctrl Pts',(16.2311205707705,17.2763735831971,2.39398252715528));
#20054=CARTESIAN_POINT('Ctrl Pts',(15.7495521891942,17.4052566407165,2.37291654370927));
#20055=CARTESIAN_POINT('Ctrl Pts',(15.4961161692798,17.4215250171174,2.36183010364304));
#20056=CARTESIAN_POINT('Ctrl Pts',(15.0069194685944,17.3559364307211,2.34043042294816));
#20057=CARTESIAN_POINT('Ctrl Pts',(14.7752765137846,17.2783217792191,2.33029731031432));
#20058=CARTESIAN_POINT('Ctrl Pts',(14.3445994938058,17.035488255536,2.31145754566084));
#20059=CARTESIAN_POINT('Ctrl Pts',(14.1515761993843,16.8691175909564,2.30104106361459));
#20060=CARTESIAN_POINT('Ctrl Pts',(13.8439774695534,16.473833045966,2.27933827172479));
#20061=CARTESIAN_POINT('Ctrl Pts',(13.7312096376842,16.2497646250875,2.26838320345701));
#20062=CARTESIAN_POINT('Ctrl Pts',(13.6183400493023,15.8438701603391,2.2505376342567));
#20063=CARTESIAN_POINT('Ctrl Pts',(13.595,15.672181316349,2.24352289562618));
#20064=CARTESIAN_POINT('Ctrl Pts',(13.595,15.4999999999999,2.23699999999995));
#20065=CARTESIAN_POINT('Origin',(15.5,15.5,-1.713));
#20066=CARTESIAN_POINT('',(13.595,15.4999999999999,1.67449999999978));
#20067=CARTESIAN_POINT('',(13.595,15.5,1.73699999999994));
#20068=CARTESIAN_POINT('',(13.595,15.5,-1.713));
#20069=CARTESIAN_POINT('Ctrl Pts',(13.595,15.4999999999999,1.67449999999978));
#20070=CARTESIAN_POINT('Ctrl Pts',(13.595,15.6805943382424,1.68134161350361));
#20071=CARTESIAN_POINT('Ctrl Pts',(13.6206767895374,15.8605641359682,1.68872117656185));
#20072=CARTESIAN_POINT('Ctrl Pts',(13.7413289123729,16.2733083137167,1.70699646110305));
#20073=CARTESIAN_POINT('Ctrl Pts',(13.8572511397691,16.4961436352298,1.71797380856537));
#20074=CARTESIAN_POINT('Ctrl Pts',(14.1704568500251,16.8874656850136,1.73964912314549));
#20075=CARTESIAN_POINT('Ctrl Pts',(14.3657712252737,17.0512012839823,1.74988369314374));
#20076=CARTESIAN_POINT('Ctrl Pts',(14.8000789722952,17.2882735425523,1.76888228225231));
#20077=CARTESIAN_POINT('Ctrl Pts',(15.0331083699897,17.3627401021875,1.77907604418122));
#20078=CARTESIAN_POINT('Ctrl Pts',(15.5238841860569,17.4214287213786,1.80054480253939));
#20079=CARTESIAN_POINT('Ctrl Pts',(15.7774357888171,17.4014455462687,1.81163629872315));
#20080=CARTESIAN_POINT('Ctrl Pts',(16.2565712745634,17.2655644201264,1.83259585627988));
#20081=CARTESIAN_POINT('Ctrl Pts',(16.4781090057824,17.1531532245574,1.84159894199786));
#20082=CARTESIAN_POINT('Ctrl Pts',(16.865460791257,16.8508077335818,1.86152522234094));
#20083=CARTESIAN_POINT('Ctrl Pts',(17.027820762239,16.6640072719447,1.87215312832116));
#20084=CARTESIAN_POINT('Ctrl Pts',(17.277693383932,16.2306622638974,1.89403519728088));
#20085=CARTESIAN_POINT('Ctrl Pts',(17.3594407795806,15.9863735004033,1.90507780326818));
#20086=CARTESIAN_POINT('Ctrl Pts',(17.4202398674738,15.4935193143535,1.92507884392557));
#20087=CARTESIAN_POINT('Ctrl Pts',(17.4039583455681,15.2503744699176,1.93397956595357));
#20088=CARTESIAN_POINT('Ctrl Pts',(17.2797387468027,14.7767335439119,1.95463988413274));
#20089=CARTESIAN_POINT('Ctrl Pts',(17.1705139566369,14.5513370860411,1.96556776923869));
#20090=CARTESIAN_POINT('Ctrl Pts',(16.8692851398174,14.1517652070239,1.98729365752725));
#20091=CARTESIAN_POINT('Ctrl Pts',(16.6788710179229,13.9824464372533,1.99787289711194));
#20092=CARTESIAN_POINT('Ctrl Pts',(16.2522998301226,13.7332282337451,2.01664432708673));
#20093=CARTESIAN_POINT('Ctrl Pts',(16.022257718409,13.652098771619,2.02665408055944));
#20094=CARTESIAN_POINT('Ctrl Pts',(15.5348488553472,13.5788405414173,2.04797555313431));
#20095=CARTESIAN_POINT('Ctrl Pts',(15.2816037882842,13.5909752658634,2.05905364005744));
#20096=CARTESIAN_POINT('Ctrl Pts',(14.7973701563817,13.7120232043683,2.08023621363144));
#20097=CARTESIAN_POINT('Ctrl Pts',(14.5708164836265,13.8185845683307,2.08945814873325));
#20098=CARTESIAN_POINT('Ctrl Pts',(14.174065869201,14.1104943182623,2.10919465644389));
#20099=CARTESIAN_POINT('Ctrl Pts',(14.0068423137263,14.2919892661037,2.11972794661126));
#20100=CARTESIAN_POINT('Ctrl Pts',(13.7450669096734,14.7165035768415,2.14153581535119));
#20101=CARTESIAN_POINT('Ctrl Pts',(13.6562783501935,14.9574480480878,2.1526057327939));
#20102=CARTESIAN_POINT('Ctrl Pts',(13.6024563313451,15.3053056555503,2.1669611367478));
#20103=CARTESIAN_POINT('Ctrl Pts',(13.595,15.4026837338876,2.17081328264832));
#20104=CARTESIAN_POINT('Ctrl Pts',(13.595,15.5,2.1744999999998));
#20105=CARTESIAN_POINT('Ctrl Pts',(13.595,15.4999999999999,2.23699999999995));
#20106=CARTESIAN_POINT('Ctrl Pts',(13.595,15.431751208773,2.23441447126066));
#20107=CARTESIAN_POINT('Ctrl Pts',(13.5986674333316,15.3634311572752,2.2317460278289));
#20108=CARTESIAN_POINT('Ctrl Pts',(13.6331507396179,15.0443258754603,2.21890285487715));
#20109=CARTESIAN_POINT('Ctrl Pts',(13.7099023892996,14.8012177434886,2.20801424407246));
#20110=CARTESIAN_POINT('Ctrl Pts',(13.9504037976665,14.3650453166575,2.18623003120062));
#20111=CARTESIAN_POINT('Ctrl Pts',(14.109523173235,14.1748740307419,2.17554530449642));
#20112=CARTESIAN_POINT('Ctrl Pts',(14.4907642526035,13.8658220120849,2.15549860987993));
#20113=CARTESIAN_POINT('Ctrl Pts',(14.7091363539253,13.7496765856905,2.14659596002061));
#20114=CARTESIAN_POINT('Ctrl Pts',(15.1849155528709,13.6043623820501,2.12578322165901));
#20115=CARTESIAN_POINT('Ctrl Pts',(15.4385395576878,13.5793402113641,2.11468855828118));
#20116=CARTESIAN_POINT('Ctrl Pts',(15.9313006918732,13.6286407381194,2.0931329531112));
#20117=CARTESIAN_POINT('Ctrl Pts',(16.1661388964057,13.6988096067292,2.08286006577382));
#20118=CARTESIAN_POINT('Ctrl Pts',(16.6064383681386,13.928626421797,2.06359937147228));
#20119=CARTESIAN_POINT('Ctrl Pts',(16.8057127521754,14.0898333101884,2.05353034999365));
#20120=CARTESIAN_POINT('Ctrl Pts',(17.1264426786317,14.4773522669783,2.03183453965873));
#20121=CARTESIAN_POINT('Ctrl Pts',(17.2461296157387,14.6986524180764,2.02083300766985));
#20122=CARTESIAN_POINT('Ctrl Pts',(17.3911031791095,15.1670180712176,1.99991860103969));
#20123=CARTESIAN_POINT('Ctrl Pts',(17.4180203684862,15.4087388151163,1.99074211236779));
#20124=CARTESIAN_POINT('Ctrl Pts',(17.3794084666146,15.9007187389138,1.97125947618687));
#20125=CARTESIAN_POINT('Ctrl Pts',(17.3098301237469,16.1459452707687,1.96044750865836));
#20126=CARTESIAN_POINT('Ctrl Pts',(17.081936726472,16.589581810925,1.93865629201535));
#20127=CARTESIAN_POINT('Ctrl Pts',(16.9279232039071,16.7848188928723,1.92789132989771));
#20128=CARTESIAN_POINT('Ctrl Pts',(16.5560962147641,17.1040830769658,1.90766366635815));
#20129=CARTESIAN_POINT('Ctrl Pts',(16.3424560638699,17.2258881558211,1.89885284618849));
#20130=CARTESIAN_POINT('Ctrl Pts',(15.8718978195449,17.3854182082523,1.87826849604306));
#20131=CARTESIAN_POINT('Ctrl Pts',(15.6183489024308,17.4180958936047,1.86717711734167));
#20132=CARTESIAN_POINT('Ctrl Pts',(15.1229151224816,17.3831207028366,1.84550459853377));
#20133=CARTESIAN_POINT('Ctrl Pts',(14.8854864440878,17.319541139132,1.83511839212985));
#20134=CARTESIAN_POINT('Ctrl Pts',(14.4406052940417,17.1030585739811,1.81565727445506));
#20135=CARTESIAN_POINT('Ctrl Pts',(14.2386939916263,16.9495664214194,1.805994240649));
#20136=CARTESIAN_POINT('Ctrl Pts',(13.9068481615258,16.5739572903711,1.78450649067386));
#20137=CARTESIAN_POINT('Ctrl Pts',(13.7798172168087,16.3558550703986,1.77346547862325));
#20138=CARTESIAN_POINT('Ctrl Pts',(13.629909999065,15.9199032586047,1.75367112373648));
#20139=CARTESIAN_POINT('Ctrl Pts',(13.595,15.710569767174,1.74497719893441));
#20140=CARTESIAN_POINT('Ctrl Pts',(13.595,15.5,1.73699999999994));
#20141=CARTESIAN_POINT('Origin',(-15.5,15.5,-1.713));
#20142=CARTESIAN_POINT('',(-17.405,15.5,10.2995));
#20143=CARTESIAN_POINT('',(-17.405,15.5,10.362));
#20144=CARTESIAN_POINT('',(-17.405,15.5,-1.713));
#20145=CARTESIAN_POINT('',(-16.8346987578547,14.140733938563,10.7369999999983));
#20146=CARTESIAN_POINT('Ctrl Pts',(-17.405,15.5,10.2995));
#20147=CARTESIAN_POINT('Ctrl Pts',(-17.405,15.5040685861377,10.2996779783962));
#20148=CARTESIAN_POINT('Ctrl Pts',(-17.4049869658359,15.5081378012993,10.2998559843088));
#20149=CARTESIAN_POINT('Ctrl Pts',(-17.4033906330436,15.7572412627348,10.3107528986323));
#20150=CARTESIAN_POINT('Ctrl Pts',(-17.3545571787606,15.9997025387586,10.321359253664));
#20151=CARTESIAN_POINT('Ctrl Pts',(-17.1671265552,16.4542045755556,10.3412412325265));
#20152=CARTESIAN_POINT('Ctrl Pts',(-17.0297788069357,16.661722890711,10.3502888948547));
#20153=CARTESIAN_POINT('Ctrl Pts',(-16.6799939284003,17.0165709526528,10.3713014329842));
#20154=CARTESIAN_POINT('Ctrl Pts',(-16.4695260417865,17.1590316553049,10.3823907106664));
#20155=CARTESIAN_POINT('Ctrl Pts',(-16.0141127709042,17.3502424572529,10.4038257440338));
#20156=CARTESIAN_POINT('Ctrl Pts',(-15.7748789785151,17.4005720901235,10.4139896704593));
#20157=CARTESIAN_POINT('Ctrl Pts',(-15.2803405005136,17.4090409031514,10.4329099369341));
#20158=CARTESIAN_POINT('Ctrl Pts',(-15.0296503702655,17.3631985762762,10.4432329588745));
#20159=CARTESIAN_POINT('Ctrl Pts',(-14.5641602654383,17.1778105668438,10.4649223841023));
#20160=CARTESIAN_POINT('Ctrl Pts',(-14.353395506391,17.041475523071,10.4758889264227));
#20161=CARTESIAN_POINT('Ctrl Pts',(-14.001475342609,16.7006854117087,10.4966748781996));
#20162=CARTESIAN_POINT('Ctrl Pts',(-13.8616419045569,16.5014953707221,10.5056900537741));
#20163=CARTESIAN_POINT('Ctrl Pts',(-13.6591140212472,16.0512722065885,10.5253848553548));
#20164=CARTESIAN_POINT('Ctrl Pts',(-13.6023464090874,15.8027433923608,10.5362566320052));
#20165=CARTESIAN_POINT('Ctrl Pts',(-13.5891625890781,15.304680938602,10.5580441409185));
#20166=CARTESIAN_POINT('Ctrl Pts',(-13.6302802412451,15.0599877380409,10.5687481304444));
#20167=CARTESIAN_POINT('Ctrl Pts',(-13.8028590578393,14.6007565222116,10.5888369850301));
#20168=CARTESIAN_POINT('Ctrl Pts',(-13.9322886349895,14.3904011858836,10.5977117908643));
#20169=CARTESIAN_POINT('Ctrl Pts',(-14.2689778421792,14.0244002544545,10.6184721527331));
#20170=CARTESIAN_POINT('Ctrl Pts',(-14.4752263247542,13.8743802194899,10.629566922763));
#20171=CARTESIAN_POINT('Ctrl Pts',(-14.9255315746248,13.6674966826003,10.6511512427232));
#20172=CARTESIAN_POINT('Ctrl Pts',(-15.1637660001395,13.6092195380962,10.6614511393463));
#20173=CARTESIAN_POINT('Ctrl Pts',(-15.6593655361598,13.5848746537428,10.6807588484659));
#20174=CARTESIAN_POINT('Ctrl Pts',(-15.9121754512101,13.6229689888941,10.6907265488194));
#20175=CARTESIAN_POINT('Ctrl Pts',(-16.2782877509633,13.7559038448062,10.7075038882848));
#20176=CARTESIAN_POINT('Ctrl Pts',(-16.4010418909404,13.8160386819109,10.7134695760448));
#20177=CARTESIAN_POINT('Ctrl Pts',(-16.6311209277075,13.9611652333068,10.725360108259));
#20178=CARTESIAN_POINT('Ctrl Pts',(-16.7378480595021,14.0456337146558,10.7312508627682));
#20179=CARTESIAN_POINT('Ctrl Pts',(-16.8346987578564,14.1407339385622,10.7369999999993));
#20180=CARTESIAN_POINT('',(-15.5,13.595,10.737));
#20181=CARTESIAN_POINT('Origin',(-15.5,15.5,10.737));
#20182=CARTESIAN_POINT('Ctrl Pts',(-15.5000000000006,13.595,10.737));
#20183=CARTESIAN_POINT('Ctrl Pts',(-15.3699120138899,13.595,10.7320717628741));
#20184=CARTESIAN_POINT('Ctrl Pts',(-15.2401373096739,13.6083238613174,10.7268639710421));
#20185=CARTESIAN_POINT('Ctrl Pts',(-14.9809515435032,13.6621430987188,10.7158678609589));
#20186=CARTESIAN_POINT('Ctrl Pts',(-14.8524833192468,13.7033785949584,10.7100990729491));
#20187=CARTESIAN_POINT('Ctrl Pts',(-14.4988222300249,13.8597998187566,10.6932797335136));
#20188=CARTESIAN_POINT('Ctrl Pts',(-14.2907287000254,14.0065862685042,10.6821857917719));
#20189=CARTESIAN_POINT('Ctrl Pts',(-13.9483989836387,14.3678225922382,10.6613159583192));
#20190=CARTESIAN_POINT('Ctrl Pts',(-13.8155791216889,14.5769539155351,10.6523782189181));
#20191=CARTESIAN_POINT('Ctrl Pts',(-13.6365911873295,15.0341600256621,10.6323779516335));
#20192=CARTESIAN_POINT('Ctrl Pts',(-13.5921308386535,15.2779191745305,10.6217148217617));
#20193=CARTESIAN_POINT('Ctrl Pts',(-13.598241495346,15.7757974377006,10.5999353701795));
#20194=CARTESIAN_POINT('Ctrl Pts',(-13.6514821744474,16.0251188925287,10.589028919837));
#20195=CARTESIAN_POINT('Ctrl Pts',(-13.8476887277444,16.4783498191008,10.5692025450963));
#20196=CARTESIAN_POINT('Ctrl Pts',(-13.9848206347882,16.6796359062972,10.5602662234653));
#20197=CARTESIAN_POINT('Ctrl Pts',(-14.3318591399905,17.0251635041763,10.5395615882713));
#20198=CARTESIAN_POINT('Ctrl Pts',(-14.5403762591266,17.1642696671436,10.5286195846064));
#20199=CARTESIAN_POINT('Ctrl Pts',(-15.0027926478457,17.3562075644913,10.5069033427678));
#20200=CARTESIAN_POINT('Ctrl Pts',(-15.2527557847393,17.4056576180186,10.496380952772));
#20201=CARTESIAN_POINT('Ctrl Pts',(-15.7469658100237,17.4043563226145,10.477629899211));
#20202=CARTESIAN_POINT('Ctrl Pts',(-15.986566461954,17.3576312123841,10.467530913802));
#20203=CARTESIAN_POINT('Ctrl Pts',(-16.4441204477045,17.1735616671745,10.4461709773248));
#20204=CARTESIAN_POINT('Ctrl Pts',(-16.6564133010635,17.0345635599908,10.4350882976379));
#20205=CARTESIAN_POINT('Ctrl Pts',(-17.0120945880556,16.6848444658985,10.4139645628509));
#20206=CARTESIAN_POINT('Ctrl Pts',(-17.1530634482971,16.4786007112435,10.4048084300633));
#20207=CARTESIAN_POINT('Ctrl Pts',(-17.347151124169,16.0262599452583,10.3850209949808));
#20208=CARTESIAN_POINT('Ctrl Pts',(-17.3994067137205,15.7848752872053,10.3744617360984));
#20209=CARTESIAN_POINT('Ctrl Pts',(-17.4048584739919,15.526819595538,10.3631732106536));
#20210=CARTESIAN_POINT('Ctrl Pts',(-17.405,15.5134066598368,10.3625864680594));
#20211=CARTESIAN_POINT('Ctrl Pts',(-17.405,15.5,10.362));
#20212=CARTESIAN_POINT('Origin',(-15.5,15.5,-1.713));
#20213=CARTESIAN_POINT('',(-17.405,15.5,9.79949999999996));
#20214=CARTESIAN_POINT('',(-17.405,15.5,9.862));
#20215=CARTESIAN_POINT('',(-17.405,15.5,-1.713));
#20216=CARTESIAN_POINT('Ctrl Pts',(-17.405,15.5,9.79949999999996));
#20217=CARTESIAN_POINT('Ctrl Pts',(-17.405,15.5422757379386,9.80134933236823));
#20218=CARTESIAN_POINT('Ctrl Pts',(-17.40359275119,15.5845971736778,9.80320066376537));
#20219=CARTESIAN_POINT('Ctrl Pts',(-17.3845405641599,15.8699821476011,9.8156846958705));
#20220=CARTESIAN_POINT('Ctrl Pts',(-17.3218280438504,16.1077355872408,9.82608510880312));
#20221=CARTESIAN_POINT('Ctrl Pts',(-17.1070822286942,16.553205723457,9.84557199140226));
#20222=CARTESIAN_POINT('Ctrl Pts',(-16.9545805300396,16.755456643589,9.85518786661981));
#20223=CARTESIAN_POINT('Ctrl Pts',(-16.5805208159003,17.0887237001984,9.8766480041212));
#20224=CARTESIAN_POINT('Ctrl Pts',(-16.3628499713819,17.2166995848147,9.8876933419744));
#20225=CARTESIAN_POINT('Ctrl Pts',(-15.8989163528556,17.3783142982288,9.90880382561483));
#20226=CARTESIAN_POINT('Ctrl Pts',(-15.6581811203113,17.4136735025017,9.91831777690985));
#20227=CARTESIAN_POINT('Ctrl Pts',(-15.1651164143754,17.3922433860113,9.93746570426309));
#20228=CARTESIAN_POINT('Ctrl Pts',(-14.9176522095134,17.3312779904081,9.94817405884487));
#20229=CARTESIAN_POINT('Ctrl Pts',(-14.4656105936897,17.1186912299103,9.96994890150104));
#20230=CARTESIAN_POINT('Ctrl Pts',(-14.2645197804293,16.970959077615,9.98079823784833));
#20231=CARTESIAN_POINT('Ctrl Pts',(-13.9332143050592,16.6104026181867,10.0012355601492));
#20232=CARTESIAN_POINT('Ctrl Pts',(-13.8047642566147,16.4022110329364,10.0100332006589));
#20233=CARTESIAN_POINT('Ctrl Pts',(-13.628699972833,15.9379596044362,10.0303416620981));
#20234=CARTESIAN_POINT('Ctrl Pts',(-13.5870407057066,15.6847822439277,10.0414167872297));
#20235=CARTESIAN_POINT('Ctrl Pts',(-13.6051138243238,15.1867387248958,10.0632034678523));
#20236=CARTESIAN_POINT('Ctrl Pts',(-13.6608710205603,14.9465120725361,10.0737120703177));
#20237=CARTESIAN_POINT('Ctrl Pts',(-13.8618203853613,14.4964258783141,10.0934008802136));
#20238=CARTESIAN_POINT('Ctrl Pts',(-14.0065697067588,14.2915005667656,10.1026890264168));
#20239=CARTESIAN_POINT('Ctrl Pts',(-14.3683432847775,13.9471548902683,10.1239260319824));
#20240=CARTESIAN_POINT('Ctrl Pts',(-14.5824715741539,13.8117722617144,10.1349991663895));
#20241=CARTESIAN_POINT('Ctrl Pts',(-15.0422282039318,13.635097453793,10.156280807899));
#20242=CARTESIAN_POINT('Ctrl Pts',(-15.2821853899945,13.5921415314096,10.1661858171533));
#20243=CARTESIAN_POINT('Ctrl Pts',(-15.776049388456,13.5982881804018,10.1850297407394));
#20244=CARTESIAN_POINT('Ctrl Pts',(-16.0252412858902,13.651539455332,10.1956348217132));
#20245=CARTESIAN_POINT('Ctrl Pts',(-16.484306788393,13.8502633168274,10.2173725434068));
#20246=CARTESIAN_POINT('Ctrl Pts',(-16.6904337512215,13.992231707287,10.2282866020876));
#20247=CARTESIAN_POINT('Ctrl Pts',(-17.0323456700082,14.3426958132205,10.2489049949351));
#20248=CARTESIAN_POINT('Ctrl Pts',(-17.1666456642617,14.5462062897174,10.2577767405825));
#20249=CARTESIAN_POINT('Ctrl Pts',(-17.3555164898945,15.0010180770042,10.2776722693352));
#20250=CARTESIAN_POINT('Ctrl Pts',(-17.405,15.2493150318857,10.288533903407));
#20251=CARTESIAN_POINT('Ctrl Pts',(-17.405,15.5,10.2995));
#20252=CARTESIAN_POINT('Ctrl Pts',(-17.405,15.5,10.362));
#20253=CARTESIAN_POINT('Ctrl Pts',(-17.405,15.2592217904251,10.3514672699224));
#20254=CARTESIAN_POINT('Ctrl Pts',(-17.3593488079492,15.0204678429165,10.3410230902414));
#20255=CARTESIAN_POINT('Ctrl Pts',(-17.1809462278487,14.5715506218093,10.3213854165272));
#20256=CARTESIAN_POINT('Ctrl Pts',(-17.0495359155277,14.3657421139465,10.3125603028827));
#20257=CARTESIAN_POINT('Ctrl Pts',(-16.7128616771596,14.0102742229046,10.2920308895517));
#20258=CARTESIAN_POINT('Ctrl Pts',(-16.5092067974019,13.8654327846184,10.281147642893));
#20259=CARTESIAN_POINT('Ctrl Pts',(-16.0535638696873,13.6598196462403,10.2593888975018));
#20260=CARTESIAN_POINT('Ctrl Pts',(-15.8051960491987,13.602744809826,10.248731405803));
#20261=CARTESIAN_POINT('Ctrl Pts',(-15.3117087298555,13.5890330071187,10.2297362852278));
#20262=CARTESIAN_POINT('Ctrl Pts',(-15.0713779050357,13.6282170971557,10.2200356005496));
#20263=CARTESIAN_POINT('Ctrl Pts',(-14.6095248225641,13.7974066753042,10.1988382562227));
#20264=CARTESIAN_POINT('Ctrl Pts',(-14.3936055605611,13.9291201388172,10.1877775257845));
#20265=CARTESIAN_POINT('Ctrl Pts',(-14.0257138194173,14.2679906029282,10.1664284957877));
#20266=CARTESIAN_POINT('Ctrl Pts',(-13.8771261361364,14.4715876659088,10.1569874161896));
#20267=CARTESIAN_POINT('Ctrl Pts',(-13.6693004494634,14.9193870498654,10.1373986417383));
#20268=CARTESIAN_POINT('Ctrl Pts',(-13.6100619110029,15.1584049022711,10.1269429176611));
#20269=CARTESIAN_POINT('Ctrl Pts',(-13.5844801810218,15.6553609522086,10.105203807865));
#20270=CARTESIAN_POINT('Ctrl Pts',(-13.6221561794649,15.9087408059525,10.0941198247616));
#20271=CARTESIAN_POINT('Ctrl Pts',(-13.7909044092091,16.3758135735006,10.0736879451663));
#20272=CARTESIAN_POINT('Ctrl Pts',(-13.9164043028326,16.5864082562103,10.0648971992549));
#20273=CARTESIAN_POINT('Ctrl Pts',(-14.2423599818571,16.951995676498,10.0445525094611));
#20274=CARTESIAN_POINT('Ctrl Pts',(-14.4408670269628,17.1025531980931,10.0337392590372));
#20275=CARTESIAN_POINT('Ctrl Pts',(-14.8892292103314,17.3219982202937,10.0119538018197));
#20276=CARTESIAN_POINT('Ctrl Pts',(-15.1357348020651,17.3868100515806,10.0011976329544));
#20277=CARTESIAN_POINT('Ctrl Pts',(-15.6283411562131,17.4158954713742,9.98189963091358));
#20278=CARTESIAN_POINT('Ctrl Pts',(-15.8695009053101,17.384308993885,9.97254931435808));
#20279=CARTESIAN_POINT('Ctrl Pts',(-16.3354422641055,17.2301461277349,9.95152575851967));
#20280=CARTESIAN_POINT('Ctrl Pts',(-16.5547757501047,17.1058694878024,9.94049834422647));
#20281=CARTESIAN_POINT('Ctrl Pts',(-16.9348786729487,16.7781774979898,9.91893120590005));
#20282=CARTESIAN_POINT('Ctrl Pts',(-17.0912603497348,16.5772552192783,9.90912402534039));
#20283=CARTESIAN_POINT('Ctrl Pts',(-17.3127769926582,16.1340913484092,9.88973802923938));
#20284=CARTESIAN_POINT('Ctrl Pts',(-17.3788584645816,15.8976206198245,9.87939372790147));
#20285=CARTESIAN_POINT('Ctrl Pts',(-17.4028955886778,15.6034559308058,9.86652563126897));
#20286=CARTESIAN_POINT('Ctrl Pts',(-17.405,15.5516978034419,9.86426149621355));
#20287=CARTESIAN_POINT('Ctrl Pts',(-17.405,15.5,9.862));
#20288=CARTESIAN_POINT('Origin',(-15.5,15.5,-1.713));
#20289=CARTESIAN_POINT('',(-17.405,15.5,9.29949999999995));
#20290=CARTESIAN_POINT('',(-17.405,15.5,9.36199999999999));
#20291=CARTESIAN_POINT('',(-17.405,15.5,-1.713));
#20292=CARTESIAN_POINT('Ctrl Pts',(-17.405,15.5,9.29949999999995));
#20293=CARTESIAN_POINT('Ctrl Pts',(-17.405,15.5820677505046,9.30309001533261));
#20294=CARTESIAN_POINT('Ctrl Pts',(-17.3996969075475,15.6642233508363,9.30668387361483));
#20295=CARTESIAN_POINT('Ctrl Pts',(-17.3577900418683,15.9860939368977,9.32076395174525));
#20296=CARTESIAN_POINT('Ctrl Pts',(-17.2810140392098,16.2181113908634,9.33091344666938));
#20297=CARTESIAN_POINT('Ctrl Pts',(-17.0397143263387,16.6497656912777,9.34979596199811));
#20298=CARTESIAN_POINT('Ctrl Pts',(-16.8740446319471,16.8434043467781,9.36016249414648));
#20299=CARTESIAN_POINT('Ctrl Pts',(-16.4798112952846,17.1525057143526,9.38185832828277));
#20300=CARTESIAN_POINT('Ctrl Pts',(-16.2560680735181,17.2661174912732,9.39281953573834));
#20301=CARTESIAN_POINT('Ctrl Pts',(-15.7845989831092,17.3990107786923,9.41358728959235));
#20302=CARTESIAN_POINT('Ctrl Pts',(-15.5420761225529,17.4197545276094,9.4225832784414));
#20303=CARTESIAN_POINT('Ctrl Pts',(-15.0510290036265,17.3684722711093,9.44230770572467));
#20304=CARTESIAN_POINT('Ctrl Pts',(-14.8076501212771,17.29259475803,9.45318745425482));
#20305=CARTESIAN_POINT('Ctrl Pts',(-14.3705451850896,17.0536228676406,9.4749735401714));
#20306=CARTESIAN_POINT('Ctrl Pts',(-14.1797471571256,16.8951195212724,9.48566853633907));
#20307=CARTESIAN_POINT('Ctrl Pts',(-13.8694408043038,16.5150275804391,9.50573761573171));
#20308=CARTESIAN_POINT('Ctrl Pts',(-13.752598707486,16.297242456207,9.51462500191565));
#20309=CARTESIAN_POINT('Ctrl Pts',(-13.6055288142055,15.8220975418946,9.53540999379283));
#20310=CARTESIAN_POINT('Ctrl Pts',(-13.5795650113124,15.5684707496953,9.54650477910339));
#20311=CARTESIAN_POINT('Ctrl Pts',(-13.6271075672436,15.0753585645942,9.56807574083135));
#20312=CARTESIAN_POINT('Ctrl Pts',(-13.6964698442562,14.840191496141,9.57836301416701));
#20313=CARTESIAN_POINT('Ctrl Pts',(-13.9246409771947,14.3993208139103,9.5976486958044));
#20314=CARTESIAN_POINT('Ctrl Pts',(-14.0848851011449,14.1997178280672,9.60766341357319));
#20315=CARTESIAN_POINT('Ctrl Pts',(-14.4709331777304,13.8775961904101,9.62933394114247));
#20316=CARTESIAN_POINT('Ctrl Pts',(-14.6918497844256,13.7569945647325,9.64034094929446));
#20317=CARTESIAN_POINT('Ctrl Pts',(-15.159737967836,13.6101942820625,9.66127722201094));
#20318=CARTESIAN_POINT('Ctrl Pts',(-15.4013438456414,13.5823472271013,9.67048577767432));
#20319=CARTESIAN_POINT('Ctrl Pts',(-15.8934538493798,13.6190577395498,9.68993175409244));
#20320=CARTESIAN_POINT('Ctrl Pts',(-16.138943260469,13.6876866711395,9.70073291472929));
#20321=CARTESIAN_POINT('Ctrl Pts',(-16.5835358465521,13.9139017605907,9.72252364170252));
#20322=CARTESIAN_POINT('Ctrl Pts',(-16.7794303173594,14.0672309118011,9.7332985395059));
#20323=CARTESIAN_POINT('Ctrl Pts',(-17.1000328628224,14.4378141280377,9.75354970122975));
#20324=CARTESIAN_POINT('Ctrl Pts',(-17.2225779810542,14.6508420595766,9.76235398335849));
#20325=CARTESIAN_POINT('Ctrl Pts',(-17.3701864548766,15.080610356166,9.78115399633266));
#20326=CARTESIAN_POINT('Ctrl Pts',(-17.405,15.2897399857174,9.79030227409083));
#20327=CARTESIAN_POINT('Ctrl Pts',(-17.405,15.5,9.79949999999996));
#20328=CARTESIAN_POINT('Ctrl Pts',(-17.405,15.5,9.862));
#20329=CARTESIAN_POINT('Ctrl Pts',(-17.405,15.2996654395986,9.85323645842513));
#20330=CARTESIAN_POINT('Ctrl Pts',(-17.3733957080017,15.1002367309777,9.84451254291253));
#20331=CARTESIAN_POINT('Ctrl Pts',(-17.2353167025393,14.6769949840126,9.82599803079682));
#20332=CARTESIAN_POINT('Ctrl Pts',(-17.1156525983397,14.4615748866098,9.81716113898337));
#20333=CARTESIAN_POINT('Ctrl Pts',(-16.80025694917,14.0861659210485,9.79700168459996));
#20334=CARTESIAN_POINT('Ctrl Pts',(-16.6069287666911,13.9301940026155,9.78626620443764));
#20335=CARTESIAN_POINT('Ctrl Pts',(-16.1660850038395,13.6974830274193,9.76447541767791));
#20336=CARTESIAN_POINT('Ctrl Pts',(-15.9216377259792,13.6251723453872,9.75363320886213));
#20337=CARTESIAN_POINT('Ctrl Pts',(-15.4300473148473,13.5810767095709,9.73404538724335));
#20338=CARTESIAN_POINT('Ctrl Pts',(-15.1879872214084,13.605317384551,9.72495408202806));
#20339=CARTESIAN_POINT('Ctrl Pts',(-14.7182619044003,13.7450429607215,9.70410295143247));
#20340=CARTESIAN_POINT('Ctrl Pts',(-14.495880438928,13.8620960973241,9.69311806224912));
#20341=CARTESIAN_POINT('Ctrl Pts',(-14.1060014570964,14.177305655609,9.6714535879792));
#20342=CARTESIAN_POINT('Ctrl Pts',(-13.9432207050001,14.3734353392653,9.66128104377678));
#20343=CARTESIAN_POINT('Ctrl Pts',(-13.7082328973408,14.8090298803107,9.64222616446597));
#20344=CARTESIAN_POINT('Ctrl Pts',(-13.6349039528453,15.0425474193521,9.63201104902234));
#20345=CARTESIAN_POINT('Ctrl Pts',(-13.5787039095847,15.5338677316258,9.6105184719325));
#20346=CARTESIAN_POINT('Ctrl Pts',(-13.600024525759,15.7874480067464,9.59942572148978));
#20347=CARTESIAN_POINT('Ctrl Pts',(-13.7384157971629,16.265698939995,9.57850485826805));
#20348=CARTESIAN_POINT('Ctrl Pts',(-13.8518193442911,16.4863923752458,9.56953150176069));
#20349=CARTESIAN_POINT('Ctrl Pts',(-14.1559440668483,16.8721284426117,9.54957315664535));
#20350=CARTESIAN_POINT('Ctrl Pts',(-14.3436419591919,17.0336374285784,9.5389298654822));
#20351=CARTESIAN_POINT('Ctrl Pts',(-14.7761103255414,17.2800944931863,9.51715571308082));
#20352=CARTESIAN_POINT('Ctrl Pts',(-15.0181269721434,17.3602604306989,9.50623377376096));
#20353=CARTESIAN_POINT('Ctrl Pts',(-15.5084664054007,17.4202298003529,9.4863461495044));
#20354=CARTESIAN_POINT('Ctrl Pts',(-15.7515756341446,17.4036993399806,9.47744089150703));
#20355=CARTESIAN_POINT('Ctrl Pts',(-16.2250969623653,17.2789972666476,9.45677455134344));
#20356=CARTESIAN_POINT('Ctrl Pts',(-16.4504036897706,17.169527963874,9.44584471753051));
#20357=CARTESIAN_POINT('Ctrl Pts',(-16.8496765704376,16.867863712006,9.42412063250715));
#20358=CARTESIAN_POINT('Ctrl Pts',(-17.0187935914998,16.6772726628492,9.41354516614536));
#20359=CARTESIAN_POINT('Ctrl Pts',(-17.2675734884154,16.2504214554202,9.39478421625935));
#20360=CARTESIAN_POINT('Ctrl Pts',(-17.3484650463879,16.0202698478367,9.38475896097284));
#20361=CARTESIAN_POINT('Ctrl Pts',(-17.3980615102738,15.6878282291739,9.37021645796922));
#20362=CARTESIAN_POINT('Ctrl Pts',(-17.405,15.5938727688573,9.36610642033496));
#20363=CARTESIAN_POINT('Ctrl Pts',(-17.405,15.5,9.36199999999999));
#20364=CARTESIAN_POINT('Origin',(-15.5,15.5,-1.713));
#20365=CARTESIAN_POINT('',(-17.405,15.5,8.79949999999994));
#20366=CARTESIAN_POINT('',(-17.405,15.5,8.86199999999999));
#20367=CARTESIAN_POINT('',(-17.405,15.5,-1.713));
#20368=CARTESIAN_POINT('Ctrl Pts',(-17.405,15.5,8.79949999999994));
#20369=CARTESIAN_POINT('Ctrl Pts',(-17.405,15.6217129566144,8.80482427631728));
#20370=CARTESIAN_POINT('Ctrl Pts',(-17.3933354276504,15.7434379092509,8.81014907739487));
#20371=CARTESIAN_POINT('Ctrl Pts',(-17.3239854242046,16.100217949099,8.82575625324124));
#20372=CARTESIAN_POINT('Ctrl Pts',(-17.23344403582,16.3260306096801,8.83523091573828));
#20373=CARTESIAN_POINT('Ctrl Pts',(-16.9668880720112,16.7413595851955,8.85441327461609));
#20374=CARTESIAN_POINT('Ctrl Pts',(-16.7897028711993,16.9245620338575,8.86513278946336));
#20375=CARTESIAN_POINT('Ctrl Pts',(-16.3786302955034,17.2082416625364,8.88691052820751));
#20376=CARTESIAN_POINT('Ctrl Pts',(-16.1498761480714,17.3076922537381,8.89775183172885));
#20377=CARTESIAN_POINT('Ctrl Pts',(-15.6715856250916,17.4127003625554,8.91816809584514));
#20378=CARTESIAN_POINT('Ctrl Pts',(-15.4269252595872,17.4189899155349,8.92696236324586));
#20379=CARTESIAN_POINT('Ctrl Pts',(-14.9371123138399,17.337575254231,8.94729909923763));
#20380=CARTESIAN_POINT('Ctrl Pts',(-14.6974339538685,17.2462527758639,8.95837647402575));
#20381=CARTESIAN_POINT('Ctrl Pts',(-14.2762146774355,16.9802149363982,8.98015274321594));
#20382=CARTESIAN_POINT('Ctrl Pts',(-14.0966830482229,16.8112614467855,8.99064949284356));
#20383=CARTESIAN_POINT('Ctrl Pts',(-13.8086030715521,16.4110945374824,9.01031563600935));
#20384=CARTESIAN_POINT('Ctrl Pts',(-13.7042031430122,16.182673235973,9.01963677882861));
#20385=CARTESIAN_POINT('Ctrl Pts',(-13.5886461508703,15.69660922453,9.04089942149891));
#20386=CARTESIAN_POINT('Ctrl Pts',(-13.5793914148363,15.4435361769218,9.05196998351153));
#20387=CARTESIAN_POINT('Ctrl Pts',(-13.6579772676657,14.9574724633382,9.07323261315211));
#20388=CARTESIAN_POINT('Ctrl Pts',(-13.7415377755509,14.728542010486,9.0830895029216));
#20389=CARTESIAN_POINT('Ctrl Pts',(-13.9952354793971,14.3048442117511,9.10196778620158));
#20390=CARTESIAN_POINT('Ctrl Pts',(-14.1666082721507,14.116253615467,9.11258495550098));
#20391=CARTESIAN_POINT('Ctrl Pts',(-14.5692130647157,13.8194985153817,9.13432789198782));
#20392=CARTESIAN_POINT('Ctrl Pts',(-14.7955130433048,13.7127801672651,9.14523518439342));
#20393=CARTESIAN_POINT('Ctrl Pts',(-15.2703703828886,13.5935003764332,9.16583354024071));
#20394=CARTESIAN_POINT('Ctrl Pts',(-15.513886785152,13.5797728775705,9.17469303357404));
#20395=CARTESIAN_POINT('Ctrl Pts',(-16.0059932519448,13.6458404657106,9.19478098176649));
#20396=CARTESIAN_POINT('Ctrl Pts',(-16.2491394450304,13.730053755045,9.20583423744073));
#20397=CARTESIAN_POINT('Ctrl Pts',(-16.6794454210861,13.9841044758504,9.22769256058453));
#20398=CARTESIAN_POINT('Ctrl Pts',(-16.8644125458322,14.1481770209327,9.23828847053363));
#20399=CARTESIAN_POINT('Ctrl Pts',(-17.1631365063348,14.5388054967535,9.25814922190827));
#20400=CARTESIAN_POINT('Ctrl Pts',(-17.2735236272034,14.7620716191431,9.2672196683789));
#20401=CARTESIAN_POINT('Ctrl Pts',(-17.382654501544,15.1634597944469,9.28477820623121));
#20402=CARTESIAN_POINT('Ctrl Pts',(-17.405,15.3315448278493,9.29213100734244));
#20403=CARTESIAN_POINT('Ctrl Pts',(-17.405,15.5,9.29949999999995));
#20404=CARTESIAN_POINT('Ctrl Pts',(-17.405,15.5,9.36199999999999));
#20405=CARTESIAN_POINT('Ctrl Pts',(-17.405,15.3438909532137,9.35517108281774));
#20406=CARTESIAN_POINT('Ctrl Pts',(-17.3858102084349,15.1880105913564,9.34835216935078));
#20407=CARTESIAN_POINT('Ctrl Pts',(-17.2871979074516,14.7954169839361,9.33117834575409));
#20408=CARTESIAN_POINT('Ctrl Pts',(-17.1804249826959,14.5690457460954,9.32196559917841));
#20409=CARTESIAN_POINT('Ctrl Pts',(-16.8881395613673,14.1726311899945,9.30222220993619));
#20410=CARTESIAN_POINT('Ctrl Pts',(-16.7064524674602,14.0055789194889,9.29168538692149));
#20411=CARTESIAN_POINT('Ctrl Pts',(-16.2816164498491,13.7442247021789,9.26987454298673));
#20412=CARTESIAN_POINT('Ctrl Pts',(-16.0405488758122,13.6556861633548,9.25880543045145));
#20413=CARTESIAN_POINT('Ctrl Pts',(-15.5498125385308,13.5803107326153,9.23856580446651));
#20414=CARTESIAN_POINT('Ctrl Pts',(-15.3056131089065,13.5895274997495,9.22975556711626));
#20415=CARTESIAN_POINT('Ctrl Pts',(-14.8286544138276,13.7001309752404,9.20926737445485));
#20416=CARTESIAN_POINT('Ctrl Pts',(-14.6008347040115,13.8024350925033,9.19839905797125));
#20417=CARTESIAN_POINT('Ctrl Pts',(-14.1930293445707,14.0912666711002,9.17663240922349));
#20418=CARTESIAN_POINT('Ctrl Pts',(-14.0181009676516,14.2766023486454,9.16595173306307));
#20419=CARTESIAN_POINT('Ctrl Pts',(-13.7565713314147,14.6952245179651,9.14688776134465));
#20420=CARTESIAN_POINT('Ctrl Pts',(-13.6687599955847,14.9222432269351,9.13727369960923));
#20421=CARTESIAN_POINT('Ctrl Pts',(-13.580930297248,15.4059245590157,9.11611528613239));
#20422=CARTESIAN_POINT('Ctrl Pts',(-13.5851843147722,15.6586224483939,9.10506113524095));
#20423=CARTESIAN_POINT('Ctrl Pts',(-13.691139565932,16.1478117809865,9.08366177685982));
#20424=CARTESIAN_POINT('Ctrl Pts',(-13.7917616714532,16.3795115137555,9.07414444581643));
#20425=CARTESIAN_POINT('Ctrl Pts',(-14.0731868140641,16.785573240168,9.05460148055085));
#20426=CARTESIAN_POINT('Ctrl Pts',(-14.2492888490198,16.9574623633346,9.04417044828869));
#20427=CARTESIAN_POINT('Ctrl Pts',(-14.6647186105415,17.2307703373922,9.0224544940457));
#20428=CARTESIAN_POINT('Ctrl Pts',(-14.9021500355565,17.326430672079,9.01136736311557));
#20429=CARTESIAN_POINT('Ctrl Pts',(-15.3904552885232,17.4173371966627,8.99088013581188));
#20430=CARTESIAN_POINT('Ctrl Pts',(-15.6358674326582,17.4156519875527,8.98208579814301));
#20431=CARTESIAN_POINT('Ctrl Pts',(-16.1162026684393,17.3193851476517,8.96178326373925));
#20432=CARTESIAN_POINT('Ctrl Pts',(-16.346344706898,17.2244006751455,8.95098706566238));
#20433=CARTESIAN_POINT('Ctrl Pts',(-16.7623834649252,16.9488308762145,8.92919856903612));
#20434=CARTESIAN_POINT('Ctrl Pts',(-16.9430358563345,16.76901250103,8.91842172092558));
#20435=CARTESIAN_POINT('Ctrl Pts',(-17.2174051014579,16.3588603424316,8.89905659338433));
#20436=CARTESIAN_POINT('Ctrl Pts',(-17.3121965174972,16.1348911979066,8.8897730182812));
#20437=CARTESIAN_POINT('Ctrl Pts',(-17.3908915635191,15.7676602614367,8.87370867285382));
#20438=CARTESIAN_POINT('Ctrl Pts',(-17.405,15.6338562764287,8.86785548015872));
#20439=CARTESIAN_POINT('Ctrl Pts',(-17.405,15.5,8.86199999999999));
#20440=CARTESIAN_POINT('Origin',(-15.5,15.5,-1.713));
#20441=CARTESIAN_POINT('',(-17.405,15.5,8.29949999999994));
#20442=CARTESIAN_POINT('',(-17.405,15.5,8.36199999999998));
#20443=CARTESIAN_POINT('',(-17.405,15.5,-1.713));
#20444=CARTESIAN_POINT('Ctrl Pts',(-17.405,15.5,8.29949999999994));
#20445=CARTESIAN_POINT('Ctrl Pts',(-17.405,15.659889295304,8.30649428238419));
#20446=CARTESIAN_POINT('Ctrl Pts',(-17.3848694669146,15.8194993551224,8.31347634974275));
#20447=CARTESIAN_POINT('Ctrl Pts',(-17.2846557073979,16.2087039329203,8.3305019218249));
#20448=CARTESIAN_POINT('Ctrl Pts',(-17.1806408331997,16.4288130372242,8.33947939030711));
#20449=CARTESIAN_POINT('Ctrl Pts',(-16.8893971352298,16.8275317385818,8.35923371190873));
#20450=CARTESIAN_POINT('Ctrl Pts',(-16.7014386929281,16.9997636421122,8.37012140821907));
#20451=CARTESIAN_POINT('Ctrl Pts',(-16.2751610984012,17.2574129066877,8.39190582896325));
#20452=CARTESIAN_POINT('Ctrl Pts',(-16.0422967724175,17.3426348398669,8.40259162898628));
#20453=CARTESIAN_POINT('Ctrl Pts',(-15.557644496301,17.4198338786248,8.42264065359248));
#20454=CARTESIAN_POINT('Ctrl Pts',(-15.3104726891065,17.4113260431361,8.4315416642333));
#20455=CARTESIAN_POINT('Ctrl Pts',(-14.8257444026703,17.2994734054767,8.45235152113692));
#20456=CARTESIAN_POINT('Ctrl Pts',(-14.5935391277617,17.1944158351004,8.46344620408319));
#20457=CARTESIAN_POINT('Ctrl Pts',(-14.1913224566373,16.9054796646701,8.48500341931656));
#20458=CARTESIAN_POINT('Ctrl Pts',(-14.0229593781544,16.7273479814129,8.49527780884648));
#20459=CARTESIAN_POINT('Ctrl Pts',(-13.7564200897581,16.3082895945115,8.51454110667273));
#20460=CARTESIAN_POINT('Ctrl Pts',(-13.6643670389324,16.0691129066074,8.52460442228296));
#20461=CARTESIAN_POINT('Ctrl Pts',(-13.5801640706732,15.5732067014332,8.54629760711124));
#20462=CARTESIAN_POINT('Ctrl Pts',(-13.5870598138748,15.321698471096,8.55729971692476));
#20463=CARTESIAN_POINT('Ctrl Pts',(-13.6955023283534,14.8435430018443,8.57821640411864));
#20464=CARTESIAN_POINT('Ctrl Pts',(-13.7929618289516,14.620710097899,8.58739617365219));
#20465=CARTESIAN_POINT('Ctrl Pts',(-14.0722259123273,14.2138380182375,8.60687499387961));
#20466=CARTESIAN_POINT('Ctrl Pts',(-14.2550239314294,14.0361814582294,8.61768584288696));
#20467=CARTESIAN_POINT('Ctrl Pts',(-14.6741023301257,13.7657537432244,8.63947702385593));
#20468=CARTESIAN_POINT('Ctrl Pts',(-14.9050731475777,13.6735852101748,8.6502430283166));
#20469=CARTESIAN_POINT('Ctrl Pts',(-15.386674416427,13.5828221715784,8.67047314435406));
#20470=CARTESIAN_POINT('Ctrl Pts',(-15.6325779853084,13.58405715791,8.67928322319381));
#20471=CARTESIAN_POINT('Ctrl Pts',(-16.1198923784801,13.6809759238713,8.69986441423044));
#20472=CARTESIAN_POINT('Ctrl Pts',(-16.3558610117794,13.779358970167,8.71095568081319));
#20473=CARTESIAN_POINT('Ctrl Pts',(-16.7675587024543,14.0572124059979,8.73262966929611));
#20474=CARTESIAN_POINT('Ctrl Pts',(-16.9414628364907,14.2309270106159,8.74301736396836));
#20475=CARTESIAN_POINT('Ctrl Pts',(-17.2186438231263,14.6407208278419,8.76248117343841));
#20476=CARTESIAN_POINT('Ctrl Pts',(-17.3168405279419,14.8745326909115,8.77213922532401));
#20477=CARTESIAN_POINT('Ctrl Pts',(-17.392281680729,15.2458303944107,8.78838146957158));
#20478=CARTESIAN_POINT('Ctrl Pts',(-17.405,15.3729086573887,8.79394044870461));
#20479=CARTESIAN_POINT('Ctrl Pts',(-17.405,15.5,8.79949999999994));
#20480=CARTESIAN_POINT('Ctrl Pts',(-17.405,15.5,8.86199999999999));
#20481=CARTESIAN_POINT('Ctrl Pts',(-17.405,15.3855229224658,8.85699225382614));
#20482=CARTESIAN_POINT('Ctrl Pts',(-17.3946811986137,15.2710075985785,8.85198283458356));
#20483=CARTESIAN_POINT('Ctrl Pts',(-17.3286272675359,14.9092076691282,8.83615606601617));
#20484=CARTESIAN_POINT('Ctrl Pts',(-17.2342052023006,14.6721012428112,8.82625705957892));
#20485=CARTESIAN_POINT('Ctrl Pts',(-16.9635816997827,14.2565828049718,8.80691646259897));
#20486=CARTESIAN_POINT('Ctrl Pts',(-16.7930874537182,14.0801193134113,8.79659782331327));
#20487=CARTESIAN_POINT('Ctrl Pts',(-16.3872122755908,13.7953832855463,8.77499387628981));
#20488=CARTESIAN_POINT('Ctrl Pts',(-16.153547037711,13.6928614102057,8.76389934568372));
#20489=CARTESIAN_POINT('Ctrl Pts',(-15.6678085401293,13.5867163450376,8.74317605560998));
#20490=CARTESIAN_POINT('Ctrl Pts',(-15.421129930203,13.5809919918463,8.7343184829412));
#20491=CARTESIAN_POINT('Ctrl Pts',(-14.9376278753187,13.6633575294034,8.71420003013759));
#20492=CARTESIAN_POINT('Ctrl Pts',(-14.7054597718186,13.7512259923533,8.70348272011769));
#20493=CARTESIAN_POINT('Ctrl Pts',(-14.2818750115858,14.0137591886409,8.68169349172043));
#20494=CARTESIAN_POINT('Ctrl Pts',(-14.0958604448596,14.188073077006,8.67083389922518));
#20495=CARTESIAN_POINT('Ctrl Pts',(-13.8091654649599,14.5899091772312,8.65118371611744));
#20496=CARTESIAN_POINT('Ctrl Pts',(-13.7076445856252,14.8110433198424,8.642138087496));
#20497=CARTESIAN_POINT('Ctrl Pts',(-13.5906893278651,15.286833932135,8.62132484986291));
#20498=CARTESIAN_POINT('Ctrl Pts',(-13.5791977767196,15.5377080032355,8.61035048104836));
#20499=CARTESIAN_POINT('Ctrl Pts',(-13.6538319112419,16.0332982624169,8.58867111712966));
#20500=CARTESIAN_POINT('Ctrl Pts',(-13.7406537883804,16.2729150218738,8.57841211733937));
#20501=CARTESIAN_POINT('Ctrl Pts',(-13.9974050276377,16.6958252070472,8.55943538119602));
#20502=CARTESIAN_POINT('Ctrl Pts',(-14.1615973637091,16.8771145995509,8.54924992929767));
#20503=CARTESIAN_POINT('Ctrl Pts',(-14.5566124809955,17.1740528601567,8.52779051299181));
#20504=CARTESIAN_POINT('Ctrl Pts',(-14.7859169215418,17.2839633295296,8.51669958099706));
#20505=CARTESIAN_POINT('Ctrl Pts',(-15.2686105331722,17.4068648278051,8.49572514184335));
#20506=CARTESIAN_POINT('Ctrl Pts',(-15.516764690117,17.4207780307135,8.4867099898438));
#20507=CARTESIAN_POINT('Ctrl Pts',(-16.0035896898075,17.3535209067153,8.46679610625113));
#20508=CARTESIAN_POINT('Ctrl Pts',(-16.2377072623264,17.2733907321687,8.45617419669088));
#20509=CARTESIAN_POINT('Ctrl Pts',(-16.6711781378121,17.0239343677871,8.43429646387539));
#20510=CARTESIAN_POINT('Ctrl Pts',(-16.8644167285607,16.8536687488138,8.42325174217519));
#20511=CARTESIAN_POINT('Ctrl Pts',(-17.1642937602988,16.4578660758281,8.40323413657636));
#20512=CARTESIAN_POINT('Ctrl Pts',(-17.272221033532,16.2393379204675,8.39434199127156));
#20513=CARTESIAN_POINT('Ctrl Pts',(-17.3820334094121,15.8411433720287,8.37692315713163));
#20514=CARTESIAN_POINT('Ctrl Pts',(-17.405,15.6707800180835,8.36947069195464));
#20515=CARTESIAN_POINT('Ctrl Pts',(-17.405,15.5,8.36199999999998));
#20516=CARTESIAN_POINT('Origin',(-15.5,15.5,-1.713));
#20517=CARTESIAN_POINT('',(-17.405,15.5,7.79949999999993));
#20518=CARTESIAN_POINT('',(-17.405,15.5,7.86199999999997));
#20519=CARTESIAN_POINT('',(-17.405,15.5,-1.713));
#20520=CARTESIAN_POINT('Ctrl Pts',(-17.405,15.5,7.79949999999993));
#20521=CARTESIAN_POINT('Ctrl Pts',(-17.405,15.6975196488277,7.80814040458557));
#20522=CARTESIAN_POINT('Ctrl Pts',(-17.3742778394761,15.8941571127754,7.81674221840651));
#20523=CARTESIAN_POINT('Ctrl Pts',(-17.2394266701263,16.3138268615082,7.83510047513149));
#20524=CARTESIAN_POINT('Ctrl Pts',(-17.1217319567968,16.5285441088021,7.84389243139474));
#20525=CARTESIAN_POINT('Ctrl Pts',(-16.8049244234265,16.9109041573485,7.86425740935985));
#20526=CARTESIAN_POINT('Ctrl Pts',(-16.605500990129,17.0720470183816,7.87533690147979));
#20527=CARTESIAN_POINT('Ctrl Pts',(-16.1638497969511,17.3022071724644,7.89710248459199));
#20528=CARTESIAN_POINT('Ctrl Pts',(-15.9276056025431,17.3723832941734,7.90758724114091));
#20529=CARTESIAN_POINT('Ctrl Pts',(-15.436677343757,17.4201648145539,7.92723059650988));
#20530=CARTESIAN_POINT('Ctrl Pts',(-15.1864838895139,17.3954586412815,7.9365858965675));
#20531=CARTESIAN_POINT('Ctrl Pts',(-14.7081429702316,17.2506698475039,7.95787416361287));
#20532=CARTESIAN_POINT('Ctrl Pts',(-14.4848664556224,17.1313747146956,7.96894199826398));
#20533=CARTESIAN_POINT('Ctrl Pts',(-14.1044542813343,16.8190167941685,7.99018546139198));
#20534=CARTESIAN_POINT('Ctrl Pts',(-13.9486774532445,16.6316831386892,7.9999950508009));
#20535=CARTESIAN_POINT('Ctrl Pts',(-13.710127524274,16.1993372753248,8.01890781822715));
#20536=CARTESIAN_POINT('Ctrl Pts',(-13.6333368077763,15.9563538337873,8.0295370151448));
#20537=CARTESIAN_POINT('Ctrl Pts',(-13.5793899361072,15.4591965407512,8.05128492822599));
#20538=CARTESIAN_POINT('Ctrl Pts',(-13.6009677390036,15.2100142466142,8.06218529104914));
#20539=CARTESIAN_POINT('Ctrl Pts',(-13.7366804393283,14.7395980072616,8.08276342925354));
#20540=CARTESIAN_POINT('Ctrl Pts',(-13.8473311902744,14.5221514404535,8.09161159696003));
#20541=CARTESIAN_POINT('Ctrl Pts',(-14.1519610237373,14.1300797586998,8.1117276518772));
#20542=CARTESIAN_POINT('Ctrl Pts',(-14.3469687875577,13.9623417964605,8.12278411113019));
#20543=CARTESIAN_POINT('Ctrl Pts',(-14.7828085084972,13.7182512489598,8.144634222419));
#20544=CARTESIAN_POINT('Ctrl Pts',(-15.0175620224701,13.6408974478214,8.15521949832876));
#20545=CARTESIAN_POINT('Ctrl Pts',(-15.5055502329557,13.5790652088895,8.17505879432587));
#20546=CARTESIAN_POINT('Ctrl Pts',(-15.7542579090358,13.5959566304196,8.18415319875526));
#20547=CARTESIAN_POINT('Ctrl Pts',(-16.2357891521937,13.7249229177914,8.20521625356614));
#20548=CARTESIAN_POINT('Ctrl Pts',(-16.4634602409219,13.8374648979382,8.21630286496682));
#20549=CARTESIAN_POINT('Ctrl Pts',(-16.8544572608822,14.1387217742593,8.23770451808363));
#20550=CARTESIAN_POINT('Ctrl Pts',(-17.0163359296066,14.3217036695108,8.24783933816551));
#20551=CARTESIAN_POINT('Ctrl Pts',(-17.2680640740017,14.7472552555663,8.2666835534289));
#20552=CARTESIAN_POINT('Ctrl Pts',(-17.3521336084914,14.9878171755692,8.27709480208075));
#20553=CARTESIAN_POINT('Ctrl Pts',(-17.3989688038528,15.3248756230826,8.29183926610146));
#20554=CARTESIAN_POINT('Ctrl Pts',(-17.405,15.4124796446347,8.29567146301983));
#20555=CARTESIAN_POINT('Ctrl Pts',(-17.405,15.5,8.29949999999994));
#20556=CARTESIAN_POINT('Ctrl Pts',(-17.405,15.5,8.36199999999998));
#20557=CARTESIAN_POINT('Ctrl Pts',(-17.405,15.4237223563989,8.35866327018366));
#20558=CARTESIAN_POINT('Ctrl Pts',(-17.4004188007143,15.3473615926038,8.35532290431339));
#20559=CARTESIAN_POINT('Ctrl Pts',(-17.3609408206951,15.020855136578,8.34104003222127));
#20560=CARTESIAN_POINT('Ctrl Pts',(-17.2811919732465,14.7788464883823,8.33045347718208));
#20561=CARTESIAN_POINT('Ctrl Pts',(-17.0372789993401,14.3492654021155,8.31166165363585));
#20562=CARTESIAN_POINT('Ctrl Pts',(-16.8790373404125,14.1636894364016,8.30168180611397));
#20563=CARTESIAN_POINT('Ctrl Pts',(-16.4942877349889,13.8557881049619,8.28037149998481));
#20564=CARTESIAN_POINT('Ctrl Pts',(-16.2692048955806,13.739213606314,8.26929474118309));
#20565=CARTESIAN_POINT('Ctrl Pts',(-15.7895412841264,13.6008458658965,8.24809680841848));
#20566=CARTESIAN_POINT('Ctrl Pts',(-15.5399575414503,13.5793194731614,8.23885671519635));
#20567=CARTESIAN_POINT('Ctrl Pts',(-15.0502061650656,13.6327856423769,8.21913360854301));
#20568=CARTESIAN_POINT('Ctrl Pts',(-14.8145379663992,13.7058628640712,8.20860721931481));
#20569=CARTESIAN_POINT('Ctrl Pts',(-14.3751816447576,13.9416635369909,8.18680520390296));
#20570=CARTESIAN_POINT('Ctrl Pts',(-14.1775156357315,14.1054824757792,8.17573375794165));
#20571=CARTESIAN_POINT('Ctrl Pts',(-13.8656118399955,14.4917801955565,8.15546842677224));
#20572=CARTESIAN_POINT('Ctrl Pts',(-13.7507656728511,14.7075897292398,8.14666361639372));
#20573=CARTESIAN_POINT('Ctrl Pts',(-13.6066151074591,15.175517044435,8.12619435501161));
#20574=CARTESIAN_POINT('Ctrl Pts',(-13.5805257646738,15.4238069094281,8.11533303108365));
#20575=CARTESIAN_POINT('Ctrl Pts',(-13.6251480140868,15.921466768242,8.09356313349774));
#20576=CARTESIAN_POINT('Ctrl Pts',(-13.6974040568621,16.1658652264558,8.0828720373379));
#20577=CARTESIAN_POINT('Ctrl Pts',(-13.9277599983122,16.6023848199964,8.06377669203865));
#20578=CARTESIAN_POINT('Ctrl Pts',(-14.0798197501874,16.7924059014821,8.05420075343611));
#20579=CARTESIAN_POINT('Ctrl Pts',(-14.4536516307035,17.1114565550985,8.0330601921028));
#20580=CARTESIAN_POINT('Ctrl Pts',(-14.6741360716317,17.2348161556276,8.02200923290562));
#20581=CARTESIAN_POINT('Ctrl Pts',(-15.1504002019035,17.3893230647177,8.00058708547467));
#20582=CARTESIAN_POINT('Ctrl Pts',(-15.4015317171629,17.4188661114753,7.99103364348828));
#20583=CARTESIAN_POINT('Ctrl Pts',(-15.8941999682968,17.379645034335,7.97151160675642));
#20584=CARTESIAN_POINT('Ctrl Pts',(-16.1312424873964,17.3138280762805,7.96109195136076));
#20585=CARTESIAN_POINT('Ctrl Pts',(-16.5762050805964,17.0921688775659,7.93938685473773));
#20586=CARTESIAN_POINT('Ctrl Pts',(-16.7782000529196,16.9350735395531,7.92829847125238));
#20587=CARTESIAN_POINT('Ctrl Pts',(-17.1023321254605,16.5586656791824,7.90778619919696));
#20588=CARTESIAN_POINT('Ctrl Pts',(-17.2243146842095,16.3455651446033,7.89898885146997));
#20589=CARTESIAN_POINT('Ctrl Pts',(-17.370589418067,15.91693477667,7.88023861665224));
#20590=CARTESIAN_POINT('Ctrl Pts',(-17.405,15.7090406870887,7.87114438701173));
#20591=CARTESIAN_POINT('Ctrl Pts',(-17.405,15.5,7.86199999999997));
#20592=CARTESIAN_POINT('Origin',(-15.5,15.5,-1.713));
#20593=CARTESIAN_POINT('',(-17.405,15.5,7.29949999999993));
#20594=CARTESIAN_POINT('',(-17.405,15.5,7.36199999999997));
#20595=CARTESIAN_POINT('',(-17.405,15.5,-1.713));
#20596=CARTESIAN_POINT('Ctrl Pts',(-17.405,15.5,7.29949999999993));
#20597=CARTESIAN_POINT('Ctrl Pts',(-17.405,15.7346844862759,7.30976616300412));
#20598=CARTESIAN_POINT('Ctrl Pts',(-17.3616308313112,15.9674729947138,7.3199493873452));
#20599=CARTESIAN_POINT('Ctrl Pts',(-17.188586342212,16.4153375533469,7.33954101283222));
#20600=CARTESIAN_POINT('Ctrl Pts',(-17.0568707339665,16.624865920156,7.34845640218951));
#20601=CARTESIAN_POINT('Ctrl Pts',(-16.7163727742873,16.9876559067647,7.36929082372597));
#20602=CARTESIAN_POINT('Ctrl Pts',(-16.5088738801906,17.1354961938847,7.38038528816625));
#20603=CARTESIAN_POINT('Ctrl Pts',(-16.0570334202494,17.3378486587404,7.40192866302165));
#20604=CARTESIAN_POINT('Ctrl Pts',(-15.8184823713025,17.3938228957298,7.41219018476189));
#20605=CARTESIAN_POINT('Ctrl Pts',(-15.3220069380349,17.4136024760751,7.43143122272065));
#20606=CARTESIAN_POINT('Ctrl Pts',(-15.0686719423133,17.3728450906666,7.44154367935196));
#20607=CARTESIAN_POINT('Ctrl Pts',(-14.5975242118065,17.1960611997515,7.46325924580043));
#20608=CARTESIAN_POINT('Ctrl Pts',(-14.383695789403,17.0636347797371,7.47425636110489));
#20609=CARTESIAN_POINT('Ctrl Pts',(-14.0250181273177,16.7294640161342,7.49515353297442));
#20610=CARTESIAN_POINT('Ctrl Pts',(-13.8814342167352,16.5331416030756,7.50430570415231));
#20611=CARTESIAN_POINT('Ctrl Pts',(-13.6702310630037,16.0871105921573,7.52381712195276));
#20612=CARTESIAN_POINT('Ctrl Pts',(-13.6086255963041,15.8397572562305,7.53463747785507));
#20613=CARTESIAN_POINT('Ctrl Pts',(-13.5856885629066,15.3416065223655,7.55642884854033));
#20614=CARTESIAN_POINT('Ctrl Pts',(-13.6221738802065,15.0957006058977,7.56718588775589));
#20615=CARTESIAN_POINT('Ctrl Pts',(-13.785927657894,14.633720204913,7.58739500415943));
#20616=CARTESIAN_POINT('Ctrl Pts',(-13.9107533017096,14.4216771100387,7.59621187363859));
#20617=CARTESIAN_POINT('Ctrl Pts',(-14.239705269712,14.0492323911653,7.6168200591308));
#20618=CARTESIAN_POINT('Ctrl Pts',(-14.4433563780086,13.8948325603828,7.62791222661482));
#20619=CARTESIAN_POINT('Ctrl Pts',(-14.8904201844231,13.6788149766268,7.64957353043571));
#20620=CARTESIAN_POINT('Ctrl Pts',(-15.127946838379,13.615882339785,7.65994844009548));
#20621=CARTESIAN_POINT('Ctrl Pts',(-15.6217480265965,13.5823404443143,7.6793891803033));
#20622=CARTESIAN_POINT('Ctrl Pts',(-15.8735137276434,13.6151256989545,7.68909034235678));
#20623=CARTESIAN_POINT('Ctrl Pts',(-16.3483419251982,13.7761111850588,7.71059979225039));
#20624=CARTESIAN_POINT('Ctrl Pts',(-16.5669268548491,13.902144028833,7.72163726048528));
#20625=CARTESIAN_POINT('Ctrl Pts',(-16.9363616526307,14.2256227819054,7.74270809585085));
#20626=CARTESIAN_POINT('Ctrl Pts',(-17.0859510511762,14.417455145383,7.75214458203764));
#20627=CARTESIAN_POINT('Ctrl Pts',(-17.3107912676849,14.8567493754688,7.77136130251383));
#20628=CARTESIAN_POINT('Ctrl Pts',(-17.3799862553193,15.1020495253587,7.78209184275398));
#20629=CARTESIAN_POINT('Ctrl Pts',(-17.4031280242506,15.4024279056926,7.79523175440463));
#20630=CARTESIAN_POINT('Ctrl Pts',(-17.405,15.4512408323701,7.79736705303449));
#20631=CARTESIAN_POINT('Ctrl Pts',(-17.405,15.5,7.79949999999993));
#20632=CARTESIAN_POINT('Ctrl Pts',(-17.405,15.5,7.86199999999997));
#20633=CARTESIAN_POINT('Ctrl Pts',(-17.405,15.4630602155995,7.86038408642165));
#20634=CARTESIAN_POINT('Ctrl Pts',(-17.4039255679755,15.4260846266625,7.85876660659067));
#20635=CARTESIAN_POINT('Ctrl Pts',(-17.387080139803,15.1371592208085,7.84612769994789));
#20636=CARTESIAN_POINT('Ctrl Pts',(-17.3224616755698,14.8905901473679,7.83534165124095));
#20637=CARTESIAN_POINT('Ctrl Pts',(-17.105849975258,14.4472097491717,7.81594618325336));
#20638=CARTESIAN_POINT('Ctrl Pts',(-16.9599010103547,14.2526704430696,7.80669145159722));
#20639=CARTESIAN_POINT('Ctrl Pts',(-16.5969765988213,13.9226974163492,7.78572521041605));
#20640=CARTESIAN_POINT('Ctrl Pts',(-16.3812522583051,13.7927700947983,7.77471093133132));
#20641=CARTESIAN_POINT('Ctrl Pts',(-15.9086227031579,13.6222144824737,7.75307545418788));
#20642=CARTESIAN_POINT('Ctrl Pts',(-15.6559096497849,13.5846116642005,7.74313367827248));
#20643=CARTESIAN_POINT('Ctrl Pts',(-15.1604736749438,13.6098026607374,7.72381365909359));
#20644=CARTESIAN_POINT('Ctrl Pts',(-14.9223004500424,13.6685072296533,7.71350673224652));
#20645=CARTESIAN_POINT('Ctrl Pts',(-14.4722850980472,13.8762308132931,7.69191502101551));
#20646=CARTESIAN_POINT('Ctrl Pts',(-14.266271196293,14.0266544528219,7.68082031006991));
#20647=CARTESIAN_POINT('Ctrl Pts',(-13.93029022398,14.3932495833448,7.66007378240269));
#20648=CARTESIAN_POINT('Ctrl Pts',(-13.8012842680293,14.6037589371102,7.65120564579572));
#20649=CARTESIAN_POINT('Ctrl Pts',(-13.629511599771,15.0632431785232,7.63110572272428));
#20650=CARTESIAN_POINT('Ctrl Pts',(-13.5888157191007,15.3080507039922,7.62039673210884));
#20651=CARTESIAN_POINT('Ctrl Pts',(-13.6028899025254,15.8061291795299,7.59860852233028));
#20652=CARTESIAN_POINT('Ctrl Pts',(-13.6601003824371,16.0545546479973,7.58774126649181));
#20653=CARTESIAN_POINT('Ctrl Pts',(-13.8634221218517,16.5043972734192,7.56806311139898));
#20654=CARTESIAN_POINT('Ctrl Pts',(-14.0035966438283,16.7033244873628,7.55903679252281));
#20655=CARTESIAN_POINT('Ctrl Pts',(-14.3561323851029,17.0435145939322,7.53824064374894));
#20656=CARTESIAN_POINT('Ctrl Pts',(-14.5671785530695,17.1794970602246,7.52727115223642));
#20657=CARTESIAN_POINT('Ctrl Pts',(-15.0330507577244,17.3640542656091,7.50558542315329));
#20658=CARTESIAN_POINT('Ctrl Pts',(-15.2838292559505,17.4094400025414,7.49528649856399));
#20659=CARTESIAN_POINT('Ctrl Pts',(-15.7784019892638,17.4000648055593,7.47634510969437));
#20660=CARTESIAN_POINT('Ctrl Pts',(-16.0175856000629,17.3492797400771,7.46617312299874));
#20661=CARTESIAN_POINT('Ctrl Pts',(-16.4727205920939,17.1571681024677,7.44472892859563));
#20662=CARTESIAN_POINT('Ctrl Pts',(-16.6829539636631,17.0142714125952,7.43363899922387));
#20663=CARTESIAN_POINT('Ctrl Pts',(-17.0319919929381,16.6587785935647,7.41264065234048));
#20664=CARTESIAN_POINT('Ctrl Pts',(-17.1688836487448,16.451098825887,7.40360537296093));
#20665=CARTESIAN_POINT('Ctrl Pts',(-17.3554698481453,15.9963244729221,7.38371148175513));
#20666=CARTESIAN_POINT('Ctrl Pts',(-17.4038675341353,15.7537299678413,7.37309929868073));
#20667=CARTESIAN_POINT('Ctrl Pts',(-17.4049934554365,15.5057662871049,7.3622522435304));
#20668=CARTESIAN_POINT('Ctrl Pts',(-17.405,15.5028829839971,7.36212611478549));
#20669=CARTESIAN_POINT('Ctrl Pts',(-17.405,15.5,7.36199999999997));
#20670=CARTESIAN_POINT('Origin',(-15.5,15.5,-1.713));
#20671=CARTESIAN_POINT('',(-17.405,15.5,6.79949999999992));
#20672=CARTESIAN_POINT('',(-17.405,15.5,6.86199999999996));
#20673=CARTESIAN_POINT('',(-17.405,15.5,-1.713));
#20674=CARTESIAN_POINT('Ctrl Pts',(-17.405,15.5,6.79949999999992));
#20675=CARTESIAN_POINT('Ctrl Pts',(-17.405,15.529549846541,6.80079264420556));
#20676=CARTESIAN_POINT('Ctrl Pts',(-17.4043124534958,15.5591255898548,6.80208642125338));
#20677=CARTESIAN_POINT('Ctrl Pts',(-17.3915676693565,15.8325360994437,6.81404663602105));
#20678=CARTESIAN_POINT('Ctrl Pts',(-17.333440693878,16.0719462026126,6.82451951892433));
#20679=CARTESIAN_POINT('Ctrl Pts',(-17.1278167083024,16.520480786797,6.84414045436547));
#20680=CARTESIAN_POINT('Ctrl Pts',(-16.980463496419,16.724504038407,6.85353031591982));
#20681=CARTESIAN_POINT('Ctrl Pts',(-16.6145319788221,17.0651375512721,6.87484364692231));
#20682=CARTESIAN_POINT('Ctrl Pts',(-16.3991807744398,17.1980307541944,6.88590866071021));
#20683=CARTESIAN_POINT('Ctrl Pts',(-15.9379957669685,17.3696215386,6.90713321558848));
#20684=CARTESIAN_POINT('Ctrl Pts',(-15.6977875712375,17.4100163428367,6.91689732140571));
#20685=CARTESIAN_POINT('Ctrl Pts',(-15.2041750736869,17.3987380335797,6.93584395820067));
#20686=CARTESIAN_POINT('Ctrl Pts',(-14.9555355034449,17.3428921189607,6.94648486552899));
#20687=CARTESIAN_POINT('Ctrl Pts',(-14.4987799696637,17.1394893913568,6.96823741405812));
#20688=CARTESIAN_POINT('Ctrl Pts',(-14.294325396585,16.9955679076125,6.97913083470897));
#20689=CARTESIAN_POINT('Ctrl Pts',(-13.9559636865064,16.6417078228246,6.9996890096429));
#20690=CARTESIAN_POINT('Ctrl Pts',(-13.8236226580918,16.436642552474,7.0085270099529));
#20691=CARTESIAN_POINT('Ctrl Pts',(-13.6379799213828,15.9761578395865,7.0286706981807));
#20692=CARTESIAN_POINT('Ctrl Pts',(-13.5910870227694,15.7233378417343,7.03973019065018));
#20693=CARTESIAN_POINT('Ctrl Pts',(-13.5992639609071,15.224034742332,7.06157197102649));
#20694=CARTESIAN_POINT('Ctrl Pts',(-13.6504175832456,14.9822974973374,7.07214665365967));
#20695=CARTESIAN_POINT('Ctrl Pts',(-13.8423565232607,14.52925632131,7.09196472785161));
#20696=CARTESIAN_POINT('Ctrl Pts',(-13.9821516037496,14.3226007751505,7.10108374200246));
#20697=CARTESIAN_POINT('Ctrl Pts',(-14.3359280564568,13.971217198846,7.12217172028144));
#20698=CARTESIAN_POINT('Ctrl Pts',(-14.5476365321871,13.8310965413759,7.13325681419718));
#20699=CARTESIAN_POINT('Ctrl Pts',(-15.0045099354585,13.6447143929865,7.15464154944394));
#20700=CARTESIAN_POINT('Ctrl Pts',(-15.2439977845298,13.5968231411538,7.16476176760272));
#20701=CARTESIAN_POINT('Ctrl Pts',(-15.7383251588478,13.5932041716068,7.18356795958517));
#20702=CARTESIAN_POINT('Ctrl Pts',(-15.988528809768,13.6414881810142,7.19402416667735));
#20703=CARTESIAN_POINT('Ctrl Pts',(-16.4519492153176,13.8313119381252,7.21573220352747));
#20704=CARTESIAN_POINT('Ctrl Pts',(-16.6611974772414,13.9695253264105,7.22668237870974));
#20705=CARTESIAN_POINT('Ctrl Pts',(-17.0098172624393,14.3135223328633,7.2474134414162));
#20706=CARTESIAN_POINT('Ctrl Pts',(-17.1478236533182,14.5141271475301,7.25637345352264));
#20707=CARTESIAN_POINT('Ctrl Pts',(-17.3460828933711,14.9663857636705,7.2761572949986));
#20708=CARTESIAN_POINT('Ctrl Pts',(-17.4004688935963,15.2154557242057,7.28705274384091));
#20709=CARTESIAN_POINT('Ctrl Pts',(-17.4049096459225,15.4785717763734,7.29856263238718));
#20710=CARTESIAN_POINT('Ctrl Pts',(-17.405,15.4892878632759,7.29903140259292));
#20711=CARTESIAN_POINT('Ctrl Pts',(-17.405,15.5,7.29949999999993));
#20712=CARTESIAN_POINT('Ctrl Pts',(-17.405,15.5,7.36199999999997));
#20713=CARTESIAN_POINT('Ctrl Pts',(-17.405,15.2480559696299,7.35097882631798));
#20714=CARTESIAN_POINT('Ctrl Pts',(-17.3550184248228,14.9985489919044,7.34006426036327));
#20715=CARTESIAN_POINT('Ctrl Pts',(-17.1648009926083,14.5429999576051,7.32013648108508));
#20716=CARTESIAN_POINT('Ctrl Pts',(-17.0301331039721,14.3397800127035,7.31125739919347));
#20717=CARTESIAN_POINT('Ctrl Pts',(-16.6875547606706,13.9899554238771,7.29062774729064));
#20718=CARTESIAN_POINT('Ctrl Pts',(-16.481115413662,13.8483563120135,7.27970993124595));
#20719=CARTESIAN_POINT('Ctrl Pts',(-16.0216210024307,13.6505150043546,7.25797526427951));
#20720=CARTESIAN_POINT('Ctrl Pts',(-15.7723283761313,13.5977521369995,7.2473770498863));
#20721=CARTESIAN_POINT('Ctrl Pts',(-15.2784189513864,13.5925705913544,7.2285525143736));
#20722=CARTESIAN_POINT('Ctrl Pts',(-15.0385078305141,13.6360094360532,7.21861991861553));
#20723=CARTESIAN_POINT('Ctrl Pts',(-14.5790228459424,13.8136434960377,7.19732758706308));
#20724=CARTESIAN_POINT('Ctrl Pts',(-14.3651283543253,13.9494945162497,7.18625306503437));
#20725=CARTESIAN_POINT('Ctrl Pts',(-14.004140425649,14.2945374747623,7.16503057177324));
#20726=CARTESIAN_POINT('Ctrl Pts',(-13.8598809196958,14.4996329878048,7.15576058671019));
#20727=CARTESIAN_POINT('Ctrl Pts',(-13.6598155630892,14.9500111762076,7.13605900366546));
#20728=CARTESIAN_POINT('Ctrl Pts',(-13.6045079682599,15.190389739209,7.12554375594011));
#20729=CARTESIAN_POINT('Ctrl Pts',(-13.5874029842169,15.6885651694387,7.10375130492394));
#20730=CARTESIAN_POINT('Ctrl Pts',(-13.62957506411,15.9417120961294,7.09267751110545));
#20731=CARTESIAN_POINT('Ctrl Pts',(-13.8065794903464,16.4055974478555,7.07238506352337));
#20732=CARTESIAN_POINT('Ctrl Pts',(-13.9354099523288,16.6134811841275,7.06358504530741));
#20733=CARTESIAN_POINT('Ctrl Pts',(-14.2674053951108,16.9733859386865,7.04313583862896));
#20734=CARTESIAN_POINT('Ctrl Pts',(-14.4688273826557,17.1207496834881,7.03228201402286));
#20735=CARTESIAN_POINT('Ctrl Pts',(-14.9213369984178,17.332445292316,7.01050893322144));
#20736=CARTESIAN_POINT('Ctrl Pts',(-15.1689206323108,17.3929123707671,6.99980695353036));
#20737=CARTESIAN_POINT('Ctrl Pts',(-15.662041736227,17.4133525920293,6.98067854085473));
#20738=CARTESIAN_POINT('Ctrl Pts',(-15.9027237815361,17.3775040697993,6.97114186392743));
#20739=CARTESIAN_POINT('Ctrl Pts',(-16.3663937750528,17.2149213346843,6.95002019459603));
#20740=CARTESIAN_POINT('Ctrl Pts',(-16.5838442157415,17.0864664974281,6.93897273071463));
#20741=CARTESIAN_POINT('Ctrl Pts',(-16.9571170705607,16.7524798042926,6.91752666241261));
#20742=CARTESIAN_POINT('Ctrl Pts',(-17.1091169017913,16.5500566576449,6.90793423699233));
#20743=CARTESIAN_POINT('Ctrl Pts',(-17.3229804931394,16.1042880116648,6.8884342962233));
#20744=CARTESIAN_POINT('Ctrl Pts',(-17.3852518264387,15.8663707366947,6.87802671639084));
#20745=CARTESIAN_POINT('Ctrl Pts',(-17.4036733949879,15.5821367961441,6.86559303570184));
#20746=CARTESIAN_POINT('Ctrl Pts',(-17.405,15.5410465275867,6.86379556113674));
#20747=CARTESIAN_POINT('Ctrl Pts',(-17.405,15.5,6.86199999999996));
#20748=CARTESIAN_POINT('Origin',(-15.5,15.5,-1.713));
#20749=CARTESIAN_POINT('',(-17.405,15.5,6.29949999999991));
#20750=CARTESIAN_POINT('',(-17.405,15.5,6.36199999999995));
#20751=CARTESIAN_POINT('',(-17.405,15.5,-1.713));
#20752=CARTESIAN_POINT('Ctrl Pts',(-17.405,15.5,6.29949999999991));
#20753=CARTESIAN_POINT('Ctrl Pts',(-17.405,15.5669742781042,6.30242975844716));
#20754=CARTESIAN_POINT('Ctrl Pts',(-17.4014681653938,15.6340281976763,6.30536300077314));
#20755=CARTESIAN_POINT('Ctrl Pts',(-17.3687838133474,15.9422510559641,6.31884606544015));
#20756=CARTESIAN_POINT('Ctrl Pts',(-17.2972902898554,16.1765419380487,6.32909501041323));
#20757=CARTESIAN_POINT('Ctrl Pts',(-17.0647622138604,16.6158967725631,6.3483143820018));
#20758=CARTESIAN_POINT('Ctrl Pts',(-16.9019625998521,16.814627588759,6.35847544040902));
#20759=CARTESIAN_POINT('Ctrl Pts',(-16.5120200024818,17.1330523072791,6.3802126475219));
#20760=CARTESIAN_POINT('Ctrl Pts',(-16.2900949650584,17.2512273505908,6.39120478408358));
#20761=CARTESIAN_POINT('Ctrl Pts',(-15.8209460953331,17.3931862699167,6.4120829248973));
#20762=CARTESIAN_POINT('Ctrl Pts',(-15.5790321175968,17.4185669224691,6.42120921772569));
#20763=CARTESIAN_POINT('Ctrl Pts',(-15.0872730490648,17.3768088108984,6.44075230178849));
#20764=CARTESIAN_POINT('Ctrl Pts',(-14.8424897793338,17.3056617463602,6.45158178832733));
#20765=CARTESIAN_POINT('Ctrl Pts',(-14.4004491373596,17.0750001587067,6.47337309275785));
#20766=CARTESIAN_POINT('Ctrl Pts',(-14.2063049243362,16.9198602281328,6.48412128986035));
#20767=CARTESIAN_POINT('Ctrl Pts',(-13.8892586880858,16.5459772061103,6.504309899037));
#20768=CARTESIAN_POINT('Ctrl Pts',(-13.7686807192717,16.331318436343,6.51313436411438));
#20769=CARTESIAN_POINT('Ctrl Pts',(-13.6122230850309,15.8596154661282,6.53376878975806));
#20770=CARTESIAN_POINT('Ctrl Pts',(-13.5812057389649,15.6060313522453,6.54486170812565));
#20771=CARTESIAN_POINT('Ctrl Pts',(-13.6192942000783,15.1111421259293,6.56651040568978));
#20772=CARTESIAN_POINT('Ctrl Pts',(-13.6843089867792,14.8742591769762,6.57687273941476));
#20773=CARTESIAN_POINT('Ctrl Pts',(-13.9036751911704,14.4303598896421,6.59629090596482));
#20774=CARTESIAN_POINT('Ctrl Pts',(-14.0588191332799,14.2290142456763,6.6060351546427));
#20775=CARTESIAN_POINT('Ctrl Pts',(-14.4370019565762,13.8995415593533,6.62756850002376));
#20776=CARTESIAN_POINT('Ctrl Pts',(-14.6558129771089,13.7740855777316,6.63860191617512));
#20777=CARTESIAN_POINT('Ctrl Pts',(-15.1211196278604,13.6175516623919,6.65965328703122));
#20778=CARTESIAN_POINT('Ctrl Pts',(-15.362141385934,13.5847635605764,6.66905348724296));
#20779=CARTESIAN_POINT('Ctrl Pts',(-15.8548982851256,13.6114064367251,6.68830376854936));
#20780=CARTESIAN_POINT('Ctrl Pts',(-16.1017164620508,13.6749924589575,6.69904496813158));
#20781=CARTESIAN_POINT('Ctrl Pts',(-16.5512641515885,13.8922557714788,6.72082761798341));
#20782=CARTESIAN_POINT('Ctrl Pts',(-16.7505999094325,14.0419164102183,6.73165264639748));
#20783=CARTESIAN_POINT('Ctrl Pts',(-17.0782652109025,14.4059003364521,6.75202703126749));
#20784=CARTESIAN_POINT('Ctrl Pts',(-17.2047080459699,14.6157239430174,6.76081775778718));
#20785=CARTESIAN_POINT('Ctrl Pts',(-17.3655964399404,15.054098393127,6.77999424291883));
#20786=CARTESIAN_POINT('Ctrl Pts',(-17.405,15.2763071874294,6.78971466261713));
#20787=CARTESIAN_POINT('Ctrl Pts',(-17.405,15.5,6.79949999999992));
#20788=CARTESIAN_POINT('Ctrl Pts',(-17.405,15.5,6.86199999999996));
#20789=CARTESIAN_POINT('Ctrl Pts',(-17.405,15.2884438551032,6.85274557546379));
#20790=CARTESIAN_POINT('Ctrl Pts',(-17.3697559300109,15.0780496586515,6.84354197981851));
#20791=CARTESIAN_POINT('Ctrl Pts',(-17.2208852103652,14.6474394617906,6.82470513831103));
#20792=CARTESIAN_POINT('Ctrl Pts',(-17.0979639297337,14.4347222488425,6.81590369562122));
#20793=CARTESIAN_POINT('Ctrl Pts',(-16.776680761579,14.0647723813145,6.79564060204316));
#20794=CARTESIAN_POINT('Ctrl Pts',(-16.5804526031638,13.9117925937642,6.78486070423475));
#20795=CARTESIAN_POINT('Ctrl Pts',(-16.1353758746613,13.6864332346946,6.76307035283269));
#20796=CARTESIAN_POINT('Ctrl Pts',(-15.8897541185117,13.6182879012923,6.75227475584018));
#20797=CARTESIAN_POINT('Ctrl Pts',(-15.3975788836265,13.5825451244441,6.73284747478383));
#20798=CARTESIAN_POINT('Ctrl Pts',(-15.1560309139864,13.6108658278522,6.72362209621475));
#20799=CARTESIAN_POINT('Ctrl Pts',(-14.6883869547904,13.7585972478523,6.70267470957475));
#20800=CARTESIAN_POINT('Ctrl Pts',(-14.4676672708304,13.8796646900924,6.69166497315547));
#20801=CARTESIAN_POINT('Ctrl Pts',(-14.0823695986942,14.202494243938,6.67000739008409));
#20802=CARTESIAN_POINT('Ctrl Pts',(-13.92261554486,14.4022645182293,6.66001992483683));
#20803=CARTESIAN_POINT('Ctrl Pts',(-13.6952840840443,14.8434260196211,6.64072152145137));
#20804=CARTESIAN_POINT('Ctrl Pts',(-13.6263340880438,15.0787599025041,6.63042695089656));
#20805=CARTESIAN_POINT('Ctrl Pts',(-13.5796896196656,15.5720489222286,6.60884825362078));
#20806=CARTESIAN_POINT('Ctrl Pts',(-13.6061342350988,15.8256758352762,6.59775346302376));
#20807=CARTESIAN_POINT('Ctrl Pts',(-13.7540997980542,16.3004960162174,6.5769826764559));
#20808=CARTESIAN_POINT('Ctrl Pts',(-13.8712975287011,16.517981966357,6.56810265670043));
#20809=CARTESIAN_POINT('Ctrl Pts',(-14.1822445273313,16.8974862231662,6.54802216114273));
#20810=CARTESIAN_POINT('Ctrl Pts',(-14.3733621908496,17.0556737310417,6.5373219640449));
#20811=CARTESIAN_POINT('Ctrl Pts',(-14.8109417400543,17.2938623446181,6.51553502998647));
#20812=CARTESIAN_POINT('Ctrl Pts',(-15.0544577816917,17.3692926308519,6.5046598671954));
#20813=CARTESIAN_POINT('Ctrl Pts',(-15.5455752341148,17.4196719474759,6.4849525247478));
#20814=CARTESIAN_POINT('Ctrl Pts',(-15.7880388344627,17.3984894506981,6.47594557206593));
#20815=CARTESIAN_POINT('Ctrl Pts',(-16.2592911603662,17.2647405448217,6.45516731577707));
#20816=CARTESIAN_POINT('Ctrl Pts',(-16.4828667093827,17.1506970735552,6.44420301828159));
#20817=CARTESIAN_POINT('Ctrl Pts',(-16.8765598212287,16.8408277807641,6.42251085369063));
#20818=CARTESIAN_POINT('Ctrl Pts',(-17.0418698243712,16.6468750229317,6.41216951106434));
#20819=CARTESIAN_POINT('Ctrl Pts',(-17.2823828232524,16.2147224745612,6.393265200112));
#20820=CARTESIAN_POINT('Ctrl Pts',(-17.3587288208372,15.9825144586595,6.38310736914518));
#20821=CARTESIAN_POINT('Ctrl Pts',(-17.3998554219865,15.6617515569817,6.36907574614965));
#20822=CARTESIAN_POINT('Ctrl Pts',(-17.405,15.5808319110706,6.36553595411502));
#20823=CARTESIAN_POINT('Ctrl Pts',(-17.405,15.5,6.36199999999995));
#20824=CARTESIAN_POINT('Origin',(-15.5,15.5,-1.713));
#20825=CARTESIAN_POINT('',(-17.405,15.5,5.7994999999999));
#20826=CARTESIAN_POINT('',(-17.405,15.5,5.86199999999995));
#20827=CARTESIAN_POINT('',(-17.405,15.5,-1.713));
#20828=CARTESIAN_POINT('Ctrl Pts',(-17.405,15.5,5.7994999999999));
#20829=CARTESIAN_POINT('Ctrl Pts',(-17.405,15.607624307934,5.80420797497514));
#20830=CARTESIAN_POINT('Ctrl Pts',(-17.3958796715229,15.7153059195385,5.8089184566726));
#20831=CARTESIAN_POINT('Ctrl Pts',(-17.3347501370527,16.0718927659009,5.82451718136037));
#20832=CARTESIAN_POINT('Ctrl Pts',(-17.2423928614072,16.3108035450705,5.83455884913306));
#20833=CARTESIAN_POINT('Ctrl Pts',(-16.9753304835568,16.7294096435034,5.85383207104165));
#20834=CARTESIAN_POINT('Ctrl Pts',(-16.8066941725831,16.9073295516354,5.86411217967549));
#20835=CARTESIAN_POINT('Ctrl Pts',(-16.4040076320726,17.1957315044031,5.88567551083158));
#20836=CARTESIAN_POINT('Ctrl Pts',(-16.1716143212648,17.3004661290847,5.89677025375238));
#20837=CARTESIAN_POINT('Ctrl Pts',(-15.6867554165738,17.4115894323903,5.91756910678677));
#20838=CARTESIAN_POINT('Ctrl Pts',(-15.439647193832,17.419741280294,5.92646397301758));
#20839=CARTESIAN_POINT('Ctrl Pts',(-14.9551408247193,17.3418832337638,5.94652188409423));
#20840=CARTESIAN_POINT('Ctrl Pts',(-14.7223635928588,17.2563237175178,5.95721176836094));
#20841=CARTESIAN_POINT('Ctrl Pts',(-14.2964260852282,16.9980504147149,5.97899695442543));
#20842=CARTESIAN_POINT('Ctrl Pts',(-14.1087140860853,16.8255518986737,5.98988114593346));
#20843=CARTESIAN_POINT('Ctrl Pts',(-13.8180496036205,16.4264347437861,6.00962223968831));
#20844=CARTESIAN_POINT('Ctrl Pts',(-13.7143526760721,16.2061957186731,6.0186077988331));
#20845=CARTESIAN_POINT('Ctrl Pts',(-13.5928784167332,15.7316795459691,6.03936528670292));
#20846=CARTESIAN_POINT('Ctrl Pts',(-13.5789510576611,15.4811760614512,6.05032344433238));
#20847=CARTESIAN_POINT('Ctrl Pts',(-13.6471560950891,14.9954922943206,6.07156945339331));
#20848=CARTESIAN_POINT('Ctrl Pts',(-13.7261405569804,14.7644691566145,6.08167545246647));
#20849=CARTESIAN_POINT('Ctrl Pts',(-13.9714778376261,14.3354041651447,6.10044469968738));
#20850=CARTESIAN_POINT('Ctrl Pts',(-14.1389919316573,14.1433938326413,6.11094512343558));
#20851=CARTESIAN_POINT('Ctrl Pts',(-14.5359866799602,13.8382635693377,6.13265871349906));
#20852=CARTESIAN_POINT('Ctrl Pts',(-14.7605810771286,13.7268799501902,6.14360343191852));
#20853=CARTESIAN_POINT('Ctrl Pts',(-15.2331602037098,13.5983967279777,6.16431678012604));
#20854=CARTESIAN_POINT('Ctrl Pts',(-15.4759944676697,13.5799183708665,6.17326070798783));
#20855=CARTESIAN_POINT('Ctrl Pts',(-15.9666683923341,13.6358680227389,6.19307308373893));
#20856=CARTESIAN_POINT('Ctrl Pts',(-16.2093249528404,13.7140529016083,6.20397593523624));
#20857=CARTESIAN_POINT('Ctrl Pts',(-16.6439545254303,13.9570579311734,6.22575645867812));
#20858=CARTESIAN_POINT('Ctrl Pts',(-16.8330924862036,14.1171836157561,6.23642404927922));
#20859=CARTESIAN_POINT('Ctrl Pts',(-17.1400816581269,14.5003102399934,6.2564338364048));
#20860=CARTESIAN_POINT('Ctrl Pts',(-17.255080234941,14.7196511698602,6.26536400568057));
#20861=CARTESIAN_POINT('Ctrl Pts',(-17.3782592374228,15.1320480082316,6.28340411234599));
#20862=CARTESIAN_POINT('Ctrl Pts',(-17.405,15.3157225386145,6.29143886870571));
#20863=CARTESIAN_POINT('Ctrl Pts',(-17.405,15.5,6.29949999999991));
#20864=CARTESIAN_POINT('Ctrl Pts',(-17.405,15.5,6.36199999999995));
#20865=CARTESIAN_POINT('Ctrl Pts',(-17.405,15.3302508811004,6.35457440424756));
#20866=CARTESIAN_POINT('Ctrl Pts',(-17.3823098623818,15.1608886824466,6.34716573414024));
#20867=CARTESIAN_POINT('Ctrl Pts',(-17.2720539956363,14.7585888660469,6.3295673169749));
#20868=CARTESIAN_POINT('Ctrl Pts',(-17.1612889929575,14.5356460396956,6.32051012645561));
#20869=CARTESIAN_POINT('Ctrl Pts',(-16.8618897192935,14.1456273570438,6.30063712915929));
#20870=CARTESIAN_POINT('Ctrl Pts',(-16.6765800686231,13.9818721663105,6.29003518425932));
#20871=CARTESIAN_POINT('Ctrl Pts',(-16.2457052882105,13.7285967342994,6.26817226992455));
#20872=CARTESIAN_POINT('Ctrl Pts',(-16.0023445596127,13.6448414733778,6.25712090493287));
#20873=CARTESIAN_POINT('Ctrl Pts',(-15.510097417241,13.5797544998568,6.23704907566801));
#20874=CARTESIAN_POINT('Ctrl Pts',(-15.2666510046418,13.5939572944337,6.22818264194464));
#20875=CARTESIAN_POINT('Ctrl Pts',(-14.7920185730827,13.7141549326478,6.20757273108299));
#20876=CARTESIAN_POINT('Ctrl Pts',(-14.5658843790827,13.821339394038,6.19666152428667));
#20877=CARTESIAN_POINT('Ctrl Pts',(-14.1638391967449,14.1189278523225,6.17492156057207));
#20878=CARTESIAN_POINT('Ctrl Pts',(-13.9928464481022,14.3078589220662,6.16431134189055));
#20879=CARTESIAN_POINT('Ctrl Pts',(-13.7399799463516,14.7320915034382,6.14545285085959));
#20880=CARTESIAN_POINT('Ctrl Pts',(-13.656870508123,14.9612272192553,6.13556836311214));
#20881=CARTESIAN_POINT('Ctrl Pts',(-13.5792709743863,15.4475415209429,6.11429477161225));
#20882=CARTESIAN_POINT('Ctrl Pts',(-13.5890590453456,15.7006488462555,6.1032227101375));
#20883=CARTESIAN_POINT('Ctrl Pts',(-13.7056349573522,16.1863755603015,6.08197482238395));
#20884=CARTESIAN_POINT('Ctrl Pts',(-13.8104358762094,16.4144498835814,6.07267281343426));
#20885=CARTESIAN_POINT('Ctrl Pts',(-14.1039832532025,16.820568086407,6.05266937566003));
#20886=CARTESIAN_POINT('Ctrl Pts',(-14.2910746473196,16.9937345530823,6.04179408530873));
#20887=CARTESIAN_POINT('Ctrl Pts',(-14.716154040337,17.2535730471962,6.02000717367115));
#20888=CARTESIAN_POINT('Ctrl Pts',(-14.9487104303037,17.339980014467,6.00930712007716));
#20889=CARTESIAN_POINT('Ctrl Pts',(-15.4328494820932,17.4194924007523,5.98922694024529));
#20890=CARTESIAN_POINT('Ctrl Pts',(-15.6797989499746,17.4122329811197,5.98034672057336));
#20891=CARTESIAN_POINT('Ctrl Pts',(-16.1649834712463,17.3029388767399,5.95957554064623));
#20892=CARTESIAN_POINT('Ctrl Pts',(-16.3978464847786,17.1990156042947,5.94848074967756));
#20893=CARTESIAN_POINT('Ctrl Pts',(-16.8017084293941,16.9119567131846,5.92690226545998));
#20894=CARTESIAN_POINT('Ctrl Pts',(-16.9710288589272,16.7345697444875,5.91660789635657));
#20895=CARTESIAN_POINT('Ctrl Pts',(-17.2394016216833,16.3170980789924,5.89730984460776));
#20896=CARTESIAN_POINT('Ctrl Pts',(-17.3325199503514,16.0788524545823,5.88732162968424));
#20897=CARTESIAN_POINT('Ctrl Pts',(-17.3954472466174,15.72034309072,5.8716388053683));
#20898=CARTESIAN_POINT('Ctrl Pts',(-17.405,15.6101460660609,5.8668182881041));
#20899=CARTESIAN_POINT('Ctrl Pts',(-17.405,15.5,5.86199999999995));
#20900=CARTESIAN_POINT('Origin',(-15.5,15.5,-1.713));
#20901=CARTESIAN_POINT('',(-17.405,15.5,5.2994999999999));
#20902=CARTESIAN_POINT('',(-17.405,15.5,5.36199999999994));
#20903=CARTESIAN_POINT('',(-17.405,15.5,-1.713));
#20904=CARTESIAN_POINT('Ctrl Pts',(-17.405,15.5,5.2994999999999));
#20905=CARTESIAN_POINT('Ctrl Pts',(-17.405,15.6490875914274,5.30602176690398));
#20906=CARTESIAN_POINT('Ctrl Pts',(-17.3874977888974,15.7980127697812,5.31253642912411));
#20907=CARTESIAN_POINT('Ctrl Pts',(-17.2946926680793,16.1855303593754,5.32948820469691));
#20908=CARTESIAN_POINT('Ctrl Pts',(-17.189983289926,16.4136838746745,5.33879455276844));
#20909=CARTESIAN_POINT('Ctrl Pts',(-16.9013559622059,16.8133636006812,5.35847077591085));
#20910=CARTESIAN_POINT('Ctrl Pts',(-16.7215432471211,16.9820716592986,5.36897280602877));
#20911=CARTESIAN_POINT('Ctrl Pts',(-16.2998513511192,17.2475038146678,5.39075373219641));
#20912=CARTESIAN_POINT('Ctrl Pts',(-16.0599908077106,17.3384658143737,5.40183012431409));
#20913=CARTESIAN_POINT('Ctrl Pts',(-15.570056397893,17.4190962505169,5.42215430905432));
#20914=CARTESIAN_POINT('Ctrl Pts',(-15.325456662796,17.4124265145795,5.43094994342898));
#20915=CARTESIAN_POINT('Ctrl Pts',(-14.8473377086516,17.3066933148065,5.45137556723504));
#20916=CARTESIAN_POINT('Ctrl Pts',(-14.6187026292344,17.2068726812802,5.46222045366264));
#20917=CARTESIAN_POINT('Ctrl Pts',(-14.2080495792291,16.9225236407745,5.4839969407011));
#20918=CARTESIAN_POINT('Ctrl Pts',(-14.0311552063945,16.7390432767342,5.49471151649644));
#20919=CARTESIAN_POINT('Ctrl Pts',(-13.7652495010312,16.3232866491125,5.51387859478455));
#20920=CARTESIAN_POINT('Ctrl Pts',(-13.6750614412334,16.0973188620358,5.52337056596503));
#20921=CARTESIAN_POINT('Ctrl Pts',(-13.5821051334709,15.6149847480906,5.54447004601513));
#20922=CARTESIAN_POINT('Ctrl Pts',(-13.5835849443739,15.3625370642135,5.55551325178403));
#20923=CARTESIAN_POINT('Ctrl Pts',(-13.6841742256802,14.871643483799,5.57698716168843));
#20924=CARTESIAN_POINT('Ctrl Pts',(-13.7826847966996,14.6381052044559,5.58662636944033));
#20925=CARTESIAN_POINT('Ctrl Pts',(-14.0604137005514,14.2287920034237,5.60610042397301));
#20926=CARTESIAN_POINT('Ctrl Pts',(-14.2346020090227,14.0553110198802,5.61649377445202));
#20927=CARTESIAN_POINT('Ctrl Pts',(-14.6467831693807,13.7780403942228,5.63817333126129));
#20928=CARTESIAN_POINT('Ctrl Pts',(-14.8829419130355,13.6800069155095,5.649264154126));
#20929=CARTESIAN_POINT('Ctrl Pts',(-15.3703854233353,13.5838625400674,5.66983329894448));
#20930=CARTESIAN_POINT('Ctrl Pts',(-15.6162252426114,13.5830038782554,5.67864068030565));
#20931=CARTESIAN_POINT('Ctrl Pts',(-16.0976645942582,13.6744743713744,5.69888013592539));
#20932=CARTESIAN_POINT('Ctrl Pts',(-16.3285308321627,13.7670050027371,5.70965009841809));
#20933=CARTESIAN_POINT('Ctrl Pts',(-16.7472223115211,14.0380951674903,5.73144111065996));
#20934=CARTESIAN_POINT('Ctrl Pts',(-16.9297461722653,14.2160309225986,5.74224768011558));
#20935=CARTESIAN_POINT('Ctrl Pts',(-17.2083821419098,14.6233255343363,5.76171194669427));
#20936=CARTESIAN_POINT('Ctrl Pts',(-17.3054989818797,14.8463034602087,5.77090435084015));
#20937=CARTESIAN_POINT('Ctrl Pts',(-17.3894642425502,15.2191704996068,5.78721524495205));
#20938=CARTESIAN_POINT('Ctrl Pts',(-17.405,15.3595364453997,5.7933554875502));
#20939=CARTESIAN_POINT('Ctrl Pts',(-17.405,15.5,5.7994999999999));
#20940=CARTESIAN_POINT('Ctrl Pts',(-17.405,15.5,5.86199999999995));
#20941=CARTESIAN_POINT('Ctrl Pts',(-17.405,15.3619687117345,5.85596188590259));
#20942=CARTESIAN_POINT('Ctrl Pts',(-17.3899976664485,15.2240174501072,5.8499272725331));
#20943=CARTESIAN_POINT('Ctrl Pts',(-17.3079876536534,14.8532208083365,5.83370694699631));
#20944=CARTESIAN_POINT('Ctrl Pts',(-17.2117279799498,14.6298789440439,5.82448203792766));
#20945=CARTESIAN_POINT('Ctrl Pts',(-16.9346639441148,14.2215290025838,5.80505423984198));
#20946=CARTESIAN_POINT('Ctrl Pts',(-16.7528277205932,14.0428968294752,5.79425848850987));
#20947=CARTESIAN_POINT('Ctrl Pts',(-16.3351086117615,13.770152156226,5.77246812558253));
#20948=CARTESIAN_POINT('Ctrl Pts',(-16.1045063871937,13.6767162920844,5.76168836544625));
#20949=CARTESIAN_POINT('Ctrl Pts',(-15.6234730666851,13.5834768813911,5.74142560162412));
#20950=CARTESIAN_POINT('Ctrl Pts',(-15.3777916705263,13.5833958255771,5.73262408439776));
#20951=CARTESIAN_POINT('Ctrl Pts',(-14.8900277034025,13.6776059092146,5.71208510677751));
#20952=CARTESIAN_POINT('Ctrl Pts',(-14.6533962925942,13.7747647786244,5.70099550713628));
#20953=CARTESIAN_POINT('Ctrl Pts',(-14.2400110887766,14.0505762177703,5.67930225220943));
#20954=CARTESIAN_POINT('Ctrl Pts',(-14.0651143574527,14.2234717132942,5.66889486987666));
#20955=CARTESIAN_POINT('Ctrl Pts',(-13.7860184999547,14.6315843224716,5.64939528950602));
#20956=CARTESIAN_POINT('Ctrl Pts',(-13.6867258707621,14.8644412284995,5.63980222097551));
#20957=CARTESIAN_POINT('Ctrl Pts',(-13.5841493983871,15.3547072418563,5.61835576369831));
#20958=CARTESIAN_POINT('Ctrl Pts',(-13.5816439640591,15.6072509385608,5.60730835789322));
#20959=CARTESIAN_POINT('Ctrl Pts',(-13.6727049726614,16.0900852469167,5.58618699707275));
#20960=CARTESIAN_POINT('Ctrl Pts',(-13.7620126940766,16.316440786022,5.57665095211607));
#20961=CARTESIAN_POINT('Ctrl Pts',(-14.026297880845,16.7332610794051,5.55752200057289));
#20962=CARTESIAN_POINT('Ctrl Pts',(-14.2024659946565,16.9174315372379,5.5468198443693));
#20963=CARTESIAN_POINT('Ctrl Pts',(-14.6120694412223,17.2034450886869,5.52504671375127));
#20964=CARTESIAN_POINT('Ctrl Pts',(-14.8404054292413,17.3041867794144,5.51419301245704));
#20965=CARTESIAN_POINT('Ctrl Pts',(-15.3180958718409,17.4117254104433,5.49374413345657));
#20966=CARTESIAN_POINT('Ctrl Pts',(-15.5625458017275,17.4193406628748,5.48494418539988));
#20967=CARTESIAN_POINT('Ctrl Pts',(-16.0527803027092,17.3406608105051,5.46465129573029));
#20968=CARTESIAN_POINT('Ctrl Pts',(-16.2930916782223,17.2505967635547,5.45357746460658));
#20969=CARTESIAN_POINT('Ctrl Pts',(-16.7159552806254,16.9866743745706,5.43178517167092));
#20970=CARTESIAN_POINT('Ctrl Pts',(-16.8964656036269,16.8185786568013,5.42127010674313));
#20971=CARTESIAN_POINT('Ctrl Pts',(-17.1864527192459,16.4201107912361,5.40156887569857));
#20972=CARTESIAN_POINT('Ctrl Pts',(-17.2919300783062,16.1926212949345,5.3922983943541));
#20973=CARTESIAN_POINT('Ctrl Pts',(-17.3868794224892,15.803210383172,5.37526379628925));
#20974=CARTESIAN_POINT('Ctrl Pts',(-17.405,15.6516981483465,5.36863596449454));
#20975=CARTESIAN_POINT('Ctrl Pts',(-17.405,15.5,5.36199999999994));
#20976=CARTESIAN_POINT('Origin',(-15.5,15.5,-1.713));
#20977=CARTESIAN_POINT('',(-17.405,15.5,4.79949999999989));
#20978=CARTESIAN_POINT('',(-17.405,15.5,4.86199999999993));
#20979=CARTESIAN_POINT('',(-17.405,15.5,-1.713));
#20980=CARTESIAN_POINT('Ctrl Pts',(-17.405,15.5,4.79949999999989));
#20981=CARTESIAN_POINT('Ctrl Pts',(-17.405,15.6915631165309,4.80787983886826));
#20982=CARTESIAN_POINT('Ctrl Pts',(-17.3761027908371,15.8823946807576,4.81622767632339));
#20983=CARTESIAN_POINT('Ctrl Pts',(-17.2462428313094,16.2997547529611,4.83448489732968));
#20984=CARTESIAN_POINT('Ctrl Pts',(-17.1291261431025,16.5173088515136,4.84336657042241));
#20985=CARTESIAN_POINT('Ctrl Pts',(-16.8183251554813,16.8969470943868,4.86344446509599));
#20986=CARTESIAN_POINT('Ctrl Pts',(-16.6272803126036,17.0552066573078,4.87414347947283));
#20987=CARTESIAN_POINT('Ctrl Pts',(-16.1898088341769,17.2935739128674,4.89593022669629));
#20988=CARTESIAN_POINT('Ctrl Pts',(-15.9463239856834,17.3691061729049,4.90680643816831));
#20989=CARTESIAN_POINT('Ctrl Pts',(-15.4552225136842,17.4196913240906,4.9265176772838));
#20990=CARTESIAN_POINT('Ctrl Pts',(-15.2127454325004,17.398608859155,4.93552210512798));
#20991=CARTESIAN_POINT('Ctrl Pts',(-14.7414436346965,17.265055070943,4.95629796793872));
#20992=CARTESIAN_POINT('Ctrl Pts',(-14.5178297768122,17.1511100267658,4.96726156389913));
#20993=CARTESIAN_POINT('Ctrl Pts',(-14.124013342636,16.8414157801667,4.98895457176108));
#20994=CARTESIAN_POINT('Ctrl Pts',(-13.9586212615899,16.6475345981838,4.99930163612475));
#20995=CARTESIAN_POINT('Ctrl Pts',(-13.7179287628858,16.2154955524047,5.01820098195934));
#20996=CARTESIAN_POINT('Ctrl Pts',(-13.6414846626363,15.9833309251378,5.02835691491065));
#20997=CARTESIAN_POINT('Ctrl Pts',(-13.5784639975189,15.4935345675145,5.04978282731762));
#20998=CARTESIAN_POINT('Ctrl Pts',(-13.59611601601,15.2400493117157,5.06087142118459));
#20999=CARTESIAN_POINT('Ctrl Pts',(-13.7276102201286,14.7593829644292,5.08189794556283));
#21000=CARTESIAN_POINT('Ctrl Pts',(-13.8382890535805,14.5363664403885,5.090958131516));
#21001=CARTESIAN_POINT('Ctrl Pts',(-14.1375343006581,14.1462086260846,5.11082833681272));
#21002=CARTESIAN_POINT('Ctrl Pts',(-14.3227658536095,13.9823809721575,5.12142890800266));
#21003=CARTESIAN_POINT('Ctrl Pts',(-14.7535109844111,13.7289285569402,5.1432907817314));
#21004=CARTESIAN_POINT('Ctrl Pts',(-14.9968228405967,13.645068755593,5.15434258178268));
#21005=CARTESIAN_POINT('Ctrl Pts',(-15.4890379478735,13.5797580488182,5.1744180909872));
#21006=CARTESIAN_POINT('Ctrl Pts',(-15.7325002956529,13.5938523991739,5.18328291172378));
#21007=CARTESIAN_POINT('Ctrl Pts',(-16.2071841013761,13.7138405611191,5.20389018711722));
#21008=CARTESIAN_POINT('Ctrl Pts',(-16.4333562159829,13.8209186591222,5.2148005040848));
#21009=CARTESIAN_POINT('Ctrl Pts',(-16.8355292739374,14.1183170077084,5.23654115409353));
#21010=CARTESIAN_POINT('Ctrl Pts',(-17.0066088233403,14.3071704386349,5.24715296298741));
#21011=CARTESIAN_POINT('Ctrl Pts',(-17.2596650716638,14.7312810048394,5.2660159736058));
#21012=CARTESIAN_POINT('Ctrl Pts',(-17.3428774803348,14.9603698228013,5.27589413048106));
#21013=CARTESIAN_POINT('Ctrl Pts',(-17.397031820958,15.2987316456968,5.2906956100478));
#21014=CARTESIAN_POINT('Ctrl Pts',(-17.405,15.3994027954335,5.29509942237232));
#21015=CARTESIAN_POINT('Ctrl Pts',(-17.405,15.5,5.2994999999999));
#21016=CARTESIAN_POINT('Ctrl Pts',(-17.405,15.5,5.36199999999994));
#21017=CARTESIAN_POINT('Ctrl Pts',(-17.405,15.4019038262264,5.35770882879374));
#21018=CARTESIAN_POINT('Ctrl Pts',(-17.3974231139549,15.3037299106598,5.35341425680927));
#21019=CARTESIAN_POINT('Ctrl Pts',(-17.344979858954,14.9675672590125,5.33870897895943));
#21020=CARTESIAN_POINT('Ctrl Pts',(-17.262631280343,14.7380842724675,5.32877714796658));
#21021=CARTESIAN_POINT('Ctrl Pts',(-17.0111668090028,14.3129513102799,5.30995207791304));
#21022=CARTESIAN_POINT('Ctrl Pts',(-16.8408162368535,14.1234481187272,5.29935367376576));
#21023=CARTESIAN_POINT('Ctrl Pts',(-16.4397182602489,13.8244573193156,5.27761892149752));
#21024=CARTESIAN_POINT('Ctrl Pts',(-16.2138656386321,13.7164876949478,5.26670120846099));
#21025=CARTESIAN_POINT('Ctrl Pts',(-15.7396134010243,13.5947431526479,5.24607186652224));
#21026=CARTESIAN_POINT('Ctrl Pts',(-15.4962839632397,13.5797400887434,5.23719299096207));
#21027=CARTESIAN_POINT('Ctrl Pts',(-15.0038015418331,13.6431761226221,5.21714835820639));
#21028=CARTESIAN_POINT('Ctrl Pts',(-14.7600815571484,13.7261592765739,5.20610027093066));
#21029=CARTESIAN_POINT('Ctrl Pts',(-14.3282524044727,13.9781269882643,5.18422980408214));
#21030=CARTESIAN_POINT('Ctrl Pts',(-14.1423674143573,14.1413464337119,5.17361778105738));
#21031=CARTESIAN_POINT('Ctrl Pts',(-13.8418324877926,14.5303383904024,5.15372421765079));
#21032=CARTESIAN_POINT('Ctrl Pts',(-13.7304324860787,14.7527385717229,5.14468860141197));
#21033=CARTESIAN_POINT('Ctrl Pts',(-13.5971113315973,15.2327697208616,5.1236898634794));
#21034=CARTESIAN_POINT('Ctrl Pts',(-13.5784894764905,15.4862851087353,5.11259995149892));
#21035=CARTESIAN_POINT('Ctrl Pts',(-13.6397087259588,15.9764936508038,5.09115600827632));
#21036=CARTESIAN_POINT('Ctrl Pts',(-13.7153309275349,16.2090202047905,5.08098424301005));
#21037=CARTESIAN_POINT('Ctrl Pts',(-13.9545192833494,16.6420070811145,5.0620434347719));
#21038=CARTESIAN_POINT('Ctrl Pts',(-14.1192234089349,16.8364863803383,5.05174385015941));
#21039=CARTESIAN_POINT('Ctrl Pts',(-14.5120053035011,17.1476444104558,5.03005801840527));
#21040=CARTESIAN_POINT('Ctrl Pts',(-14.735297199777,17.2624129624023,5.01908860761755));
#21041=CARTESIAN_POINT('Ctrl Pts',(-15.2061841812833,17.3975998855666,4.99829273929394));
#21042=CARTESIAN_POINT('Ctrl Pts',(-15.448549029226,17.4195192309441,4.9892667306742));
#21043=CARTESIAN_POINT('Ctrl Pts',(-15.9397831942183,17.3706555599016,4.96958811730537));
#21044=CARTESIAN_POINT('Ctrl Pts',(-16.1835275815734,17.2959765775398,4.95872073661156));
#21045=CARTESIAN_POINT('Ctrl Pts',(-16.6219006739087,17.0591049338943,4.9369325451802));
#21046=CARTESIAN_POINT('Ctrl Pts',(-16.8135537499556,16.9014490198769,4.9262236917428));
#21047=CARTESIAN_POINT('Ctrl Pts',(-17.1255753275233,16.5229316751174,4.90612407297281));
#21048=CARTESIAN_POINT('Ctrl Pts',(-17.2433693043559,16.3059465957354,4.89725575659387));
#21049=CARTESIAN_POINT('Ctrl Pts',(-17.3753951061978,15.8870131088787,4.87892970730005));
#21050=CARTESIAN_POINT('Ctrl Pts',(-17.405,15.6938944322268,4.87048182118221));
#21051=CARTESIAN_POINT('Ctrl Pts',(-17.405,15.5,4.86199999999993));
#21052=CARTESIAN_POINT('Origin',(-15.5,15.5,-1.713));
#21053=CARTESIAN_POINT('',(-17.405,15.5,4.29949999999989));
#21054=CARTESIAN_POINT('',(-17.405,15.5,4.36199999999993));
#21055=CARTESIAN_POINT('',(-17.405,15.5,-1.713));
#21056=CARTESIAN_POINT('Ctrl Pts',(-17.405,15.5,4.29949999999989));
#21057=CARTESIAN_POINT('Ctrl Pts',(-17.405,15.7316143560873,4.30963186159601));
#21058=CARTESIAN_POINT('Ctrl Pts',(-17.3627567347742,15.961507388049,4.31968842467383));
#21059=CARTESIAN_POINT('Ctrl Pts',(-17.1938338138213,16.4048278056338,4.33908126883765));
#21060=CARTESIAN_POINT('Ctrl Pts',(-17.0650898508518,16.6127814998738,4.34788071653058));
#21061=CARTESIAN_POINT('Ctrl Pts',(-16.7332512944162,16.9728344984569,4.36832722217888));
#21062=CARTESIAN_POINT('Ctrl Pts',(-16.5319045679017,17.1202820929434,4.37918002958804));
#21063=CARTESIAN_POINT('Ctrl Pts',(-16.0795012341922,17.3321804659507,4.40095351892543));
#21064=CARTESIAN_POINT('Ctrl Pts',(-15.8319446713374,17.392760897025,4.41165695233938));
#21065=CARTESIAN_POINT('Ctrl Pts',(-15.3388363370757,17.4134262550738,4.43078980550267));
#21066=CARTESIAN_POINT('Ctrl Pts',(-15.0981422293757,17.3776890517327,4.44032128224835));
#21067=CARTESIAN_POINT('Ctrl Pts',(-14.6344121963986,17.2153265681764,4.46144040870655));
#21068=CARTESIAN_POINT('Ctrl Pts',(-14.4169115189193,17.086980672769,4.4724873929472));
#21069=CARTESIAN_POINT('Ctrl Pts',(-14.0434595959548,16.7531576246628,4.49393666575702));
#21070=CARTESIAN_POINT('Ctrl Pts',(-13.8913456195006,16.550773658121,4.50353439815721));
#21071=CARTESIAN_POINT('Ctrl Pts',(-13.6772812436004,16.1050729095015,4.52303136878798));
#21072=CARTESIAN_POINT('Ctrl Pts',(-13.6149094566655,15.8671928542976,4.53343732045919));
#21073=CARTESIAN_POINT('Ctrl Pts',(-13.5825512110825,15.3713167974186,4.5551291864644));
#21074=CARTESIAN_POINT('Ctrl Pts',(-13.6166230909332,15.1178055136802,4.5662189189114));
#21075=CARTESIAN_POINT('Ctrl Pts',(-13.7787288519487,14.6482137858557,4.58676098924494));
#21076=CARTESIAN_POINT('Ctrl Pts',(-13.901564546466,14.4354258053553,4.59556305285422));
#21077=CARTESIAN_POINT('Ctrl Pts',(-14.2226927406017,14.065331732804,4.6158234295064));
#21078=CARTESIAN_POINT('Ctrl Pts',(-14.4188449704033,13.9122723318701,4.62660219216974));
#21079=CARTESIAN_POINT('Ctrl Pts',(-14.8638116031428,13.6867180287382,4.64839263658595));
#21080=CARTESIAN_POINT('Ctrl Pts',(-15.1094033098687,13.618462555476,4.65918950419813));
#21081=CARTESIAN_POINT('Ctrl Pts',(-15.6015637489736,13.5824994210303,4.67862104445296));
#21082=CARTESIAN_POINT('Ctrl Pts',(-15.8431248716566,13.6107122496045,4.68784256256878));
#21083=CARTESIAN_POINT('Ctrl Pts',(-16.3108245138832,13.7582315620518,4.70878741942499));
#21084=CARTESIAN_POINT('Ctrl Pts',(-16.5315891397848,13.8791929198398,4.71979653811186));
#21085=CARTESIAN_POINT('Ctrl Pts',(-16.9170577878751,14.2018613025606,4.74145707323737));
#21086=CARTESIAN_POINT('Ctrl Pts',(-17.0769234362671,14.4015934816703,4.75145072098273));
#21087=CARTESIAN_POINT('Ctrl Pts',(-17.3044462179037,14.842688756663,4.77074622732537));
#21088=CARTESIAN_POINT('Ctrl Pts',(-17.3734901964393,15.0779846890365,4.78103913775291));
#21089=CARTESIAN_POINT('Ctrl Pts',(-17.4021618668534,15.3798527943734,4.79424421672653));
#21090=CARTESIAN_POINT('Ctrl Pts',(-17.405,15.439962325706,4.79687368003952));
#21091=CARTESIAN_POINT('Ctrl Pts',(-17.405,15.5,4.79949999999989));
#21092=CARTESIAN_POINT('Ctrl Pts',(-17.405,15.5,4.86199999999993));
#21093=CARTESIAN_POINT('Ctrl Pts',(-17.405,15.442180147366,4.85947069760999));
#21094=CARTESIAN_POINT('Ctrl Pts',(-17.4023676760667,15.384291310761,4.85693837754862));
#21095=CARTESIAN_POINT('Ctrl Pts',(-17.3749487573809,15.0844652353877,4.84382262621995));
#21096=CARTESIAN_POINT('Ctrl Pts',(-17.3066907671614,14.8488532982766,4.83351589231308));
#21097=CARTESIAN_POINT('Ctrl Pts',(-17.0807664256711,14.4072053923165,4.81419621138743));
#21098=CARTESIAN_POINT('Ctrl Pts',(-16.9218318768361,14.207155325346,4.80425372650585));
#21099=CARTESIAN_POINT('Ctrl Pts',(-16.5377915939255,13.8831427274651,4.7826179023581));
#21100=CARTESIAN_POINT('Ctrl Pts',(-16.3174037618294,13.7612960189594,4.77160369345465));
#21101=CARTESIAN_POINT('Ctrl Pts',(-15.8501699940223,13.6120055732969,4.75063774703041));
#21102=CARTESIAN_POINT('Ctrl Pts',(-15.608718013233,13.5828923181582,4.74138348216231));
#21103=CARTESIAN_POINT('Ctrl Pts',(-15.1164351703261,13.6170170003983,4.72198751589263));
#21104=CARTESIAN_POINT('Ctrl Pts',(-14.8705943170609,13.6843531721741,4.71120131685047));
#21105=CARTESIAN_POINT('Ctrl Pts',(-14.4247117857891,13.9082794227657,4.68941178384605));
#21106=CARTESIAN_POINT('Ctrl Pts',(-14.2279270505859,14.0606734938221,4.67862361169857));
#21107=CARTESIAN_POINT('Ctrl Pts',(-13.9055064884792,14.4295641212511,4.65834059721033));
#21108=CARTESIAN_POINT('Ctrl Pts',(-13.7819572656015,14.641762613156,4.64954319277536));
#21109=CARTESIAN_POINT('Ctrl Pts',(-13.6180694285514,15.1106825581303,4.62903050926817));
#21110=CARTESIAN_POINT('Ctrl Pts',(-13.5830318586544,15.3641634543827,4.61794210610752));
#21111=CARTESIAN_POINT('Ctrl Pts',(-13.6135760220822,15.8603378399028,4.59623718985554));
#21112=CARTESIAN_POINT('Ctrl Pts',(-13.6751098443104,16.0985268650805,4.58581772243744));
#21113=CARTESIAN_POINT('Ctrl Pts',(-13.8875008995235,16.5447927407348,4.56629603058904));
#21114=CARTESIAN_POINT('Ctrl Pts',(-14.0386649367322,16.7475029360245,4.55674198688621));
#21115=CARTESIAN_POINT('Ctrl Pts',(-14.4106247533747,17.0826873364552,4.53531946498705));
#21116=CARTESIAN_POINT('Ctrl Pts',(-14.6277054116799,17.2119400123398,4.52426855935693));
#21117=CARTESIAN_POINT('Ctrl Pts',(-15.0909343363085,17.3761369776451,4.50312829255253));
#21118=CARTESIAN_POINT('Ctrl Pts',(-15.3315286777462,17.4128011071027,4.49355297455963));
#21119=CARTESIAN_POINT('Ctrl Pts',(-15.8247422542316,17.3940092756639,4.4744571126853));
#21120=CARTESIAN_POINT('Ctrl Pts',(-16.0725224561213,17.3343724488225,4.46376584572063));
#21121=CARTESIAN_POINT('Ctrl Pts',(-16.5258074097486,17.1241629404857,4.44199589650089));
#21122=CARTESIAN_POINT('Ctrl Pts',(-16.7277793655432,16.9774142091866,4.43113468870475));
#21123=CARTESIAN_POINT('Ctrl Pts',(-17.0609228345532,16.6185952804082,4.41066573981338));
#21124=CARTESIAN_POINT('Ctrl Pts',(-17.1903862601901,16.4112227261169,4.40186101164118));
#21125=CARTESIAN_POINT('Ctrl Pts',(-17.3618494871938,15.9663776396961,4.38240147155279));
#21126=CARTESIAN_POINT('Ctrl Pts',(-17.405,15.7340888477603,4.37224010707606));
#21127=CARTESIAN_POINT('Ctrl Pts',(-17.405,15.5,4.36199999999993));
#21128=CARTESIAN_POINT('Origin',(-15.5,15.5,-1.713));
#21129=CARTESIAN_POINT('',(-17.405,15.5,3.79949999999988));
#21130=CARTESIAN_POINT('',(-17.405,15.5,3.86199999999992));
#21131=CARTESIAN_POINT('',(-17.405,15.5,-1.713));
#21132=CARTESIAN_POINT('Ctrl Pts',(-17.405,15.5,3.79949999999988));
#21133=CARTESIAN_POINT('Ctrl Pts',(-17.405,15.5176704969382,3.80027298761747));
#21134=CARTESIAN_POINT('Ctrl Pts',(-17.4047541376814,15.5353510584371,3.80104641550444));
#21135=CARTESIAN_POINT('Ctrl Pts',(-17.3972339401769,15.80536106744,3.81285787696563));
#21136=CARTESIAN_POINT('Ctrl Pts',(-17.3401239250485,16.0538100548939,3.82372616163116));
#21137=CARTESIAN_POINT('Ctrl Pts',(-17.1369822758118,16.5037390621237,3.84340809545575));
#21138=CARTESIAN_POINT('Ctrl Pts',(-16.9968851667794,16.7027258920315,3.85243186198737));
#21139=CARTESIAN_POINT('Ctrl Pts',(-16.6444891216015,17.0430522125178,3.87322569783866));
#21140=CARTESIAN_POINT('Ctrl Pts',(-16.4335067749666,17.1791147524432,3.88419452294358));
#21141=CARTESIAN_POINT('Ctrl Pts',(-15.9677211723474,17.3638605915779,3.90588109705348));
#21142=CARTESIAN_POINT('Ctrl Pts',(-15.7169626616863,17.4093499767944,3.91618546959334));
#21143=CARTESIAN_POINT('Ctrl Pts',(-15.2223975598373,17.4001805186165,3.93512206937967));
#21144=CARTESIAN_POINT('Ctrl Pts',(-14.9832024838002,17.349498823534,3.94529222947809));
#21145=CARTESIAN_POINT('Ctrl Pts',(-14.5280041766517,17.1575916214525,3.96673435103501));
#21146=CARTESIAN_POINT('Ctrl Pts',(-14.3177174993268,17.0147938586229,3.97782413607682));
#21147=CARTESIAN_POINT('Ctrl Pts',(-13.9685099193908,16.6594473181571,3.99882570675274));
#21148=CARTESIAN_POINT('Ctrl Pts',(-13.831514770583,16.4518042050906,4.00786377055572));
#21149=CARTESIAN_POINT('Ctrl Pts',(-13.6447368436005,15.9970916456269,4.02775495863375));
#21150=CARTESIAN_POINT('Ctrl Pts',(-13.5962401833917,15.7545273240917,4.03836582134307));
#21151=CARTESIAN_POINT('Ctrl Pts',(-13.593758117278,15.2545881601184,4.06023542606632));
#21152=CARTESIAN_POINT('Ctrl Pts',(-13.6436544882321,15.0020200803626,4.07128389849659));
#21153=CARTESIAN_POINT('Ctrl Pts',(-13.834779566897,14.5437277846285,4.09133168046222));
#21154=CARTESIAN_POINT('Ctrl Pts',(-13.969363896983,14.3404418930211,4.10020906843054));
#21155=CARTESIAN_POINT('Ctrl Pts',(-14.3117908874209,13.9904720051824,4.1208361645189));
#21156=CARTESIAN_POINT('Ctrl Pts',(-14.5181593317412,13.8487889523204,4.1317531304748));
#21157=CARTESIAN_POINT('Ctrl Pts',(-14.9775564642285,13.6507470886944,4.15348849875881));
#21158=CARTESIAN_POINT('Ctrl Pts',(-15.2268262960436,13.5978732610907,4.16408827656067));
#21159=CARTESIAN_POINT('Ctrl Pts',(-15.7207254532908,13.5924724783421,4.182917218313));
#21160=CARTESIAN_POINT('Ctrl Pts',(-15.960647006969,13.6358015845445,4.19284351716882));
#21161=CARTESIAN_POINT('Ctrl Pts',(-16.4201937842834,13.8132176501179,4.21413342163813));
#21162=CARTESIAN_POINT('Ctrl Pts',(-16.6341414924654,13.9489622633598,4.22520763235503));
#21163=CARTESIAN_POINT('Ctrl Pts',(-16.9953079945519,14.2938468480346,4.24643342667437));
#21164=CARTESIAN_POINT('Ctrl Pts',(-17.1396787721256,14.4989036810798,4.25570751010824));
#21165=CARTESIAN_POINT('Ctrl Pts',(-17.3399450798589,14.9492155337354,4.27540619132677));
#21166=CARTESIAN_POINT('Ctrl Pts',(-17.3953549173897,15.1895596350089,4.28591993153996));
#21167=CARTESIAN_POINT('Ctrl Pts',(-17.4046168492424,15.4558661493172,4.29756938535922));
#21168=CARTESIAN_POINT('Ctrl Pts',(-17.405,15.4779408815478,4.29853503418833));
#21169=CARTESIAN_POINT('Ctrl Pts',(-17.405,15.5,4.29949999999989));
#21170=CARTESIAN_POINT('Ctrl Pts',(-17.405,15.5,4.36199999999992));
#21171=CARTESIAN_POINT('Ctrl Pts',(-17.405,15.4802786628464,4.36113729933704));
#21172=CARTESIAN_POINT('Ctrl Pts',(-17.4046937566948,15.4605445496239,4.3602740397911));
#21173=CARTESIAN_POINT('Ctrl Pts',(-17.3964838036035,15.196462759103,4.34872190547259));
#21174=CARTESIAN_POINT('Ctrl Pts',(-17.3419245741628,14.9558334540293,4.33819568915266));
#21175=CARTESIAN_POINT('Ctrl Pts',(-17.1433286776143,14.5049708959333,4.31847291758239));
#21176=CARTESIAN_POINT('Ctrl Pts',(-16.9998815572957,14.2995927046866,4.30923236586305));
#21177=CARTESIAN_POINT('Ctrl Pts',(-16.6401991058068,13.9533939709778,4.28803404971522));
#21178=CARTESIAN_POINT('Ctrl Pts',(-16.4266950092731,13.8167660487444,4.2769573247578));
#21179=CARTESIAN_POINT('Ctrl Pts',(-15.9676626533492,13.6375389919569,4.25564729808314));
#21180=CARTESIAN_POINT('Ctrl Pts',(-15.7278271357321,13.5932983649885,4.24566819355739));
#21181=CARTESIAN_POINT('Ctrl Pts',(-15.2338436728025,13.5968793835659,4.22687586034501));
#21182=CARTESIAN_POINT('Ctrl Pts',(-14.9843861963398,13.6488319941837,4.2162891229395));
#21183=CARTESIAN_POINT('Ctrl Pts',(-14.5241843554176,13.8452078975466,4.19455970750693));
#21184=CARTESIAN_POINT('Ctrl Pts',(-14.3172284572202,13.9861932444804,4.18363574693085));
#21185=CARTESIAN_POINT('Ctrl Pts',(-13.9735457966652,14.3349566669919,4.16298746932207));
#21186=CARTESIAN_POINT('Ctrl Pts',(-13.8382681374568,14.5376960900176,4.15409553411999));
#21187=CARTESIAN_POINT('Ctrl Pts',(-13.6454549294062,14.9953080207069,4.1340775144048));
#21188=CARTESIAN_POINT('Ctrl Pts',(-13.594632734797,15.2477915561283,4.12303274032687));
#21189=CARTESIAN_POINT('Ctrl Pts',(-13.5953570499606,15.747914024217,4.10115511705089));
#21190=CARTESIAN_POINT('Ctrl Pts',(-13.6430324851627,15.9907274358747,4.09053335801075));
#21191=CARTESIAN_POINT('Ctrl Pts',(-13.8282206878626,16.4459517174347,4.07061978488913));
#21192=CARTESIAN_POINT('Ctrl Pts',(-13.9643588390081,16.6538987001136,4.06160432661678));
#21193=CARTESIAN_POINT('Ctrl Pts',(-14.3121609791575,17.0104560948599,4.04062951532048));
#21194=CARTESIAN_POINT('Ctrl Pts',(-14.5220046281817,17.1540729720191,4.02953859802139));
#21195=CARTESIAN_POINT('Ctrl Pts',(-14.9766756252456,17.3476734773997,4.00807941663418));
#21196=CARTESIAN_POINT('Ctrl Pts',(-15.2157743708606,17.3992116297402,3.99789417324461));
#21197=CARTESIAN_POINT('Ctrl Pts',(-15.710400153106,17.41008596889,3.97891798503961));
#21198=CARTESIAN_POINT('Ctrl Pts',(-15.9613230313347,17.3654556147342,3.96865837020476));
#21199=CARTESIAN_POINT('Ctrl Pts',(-16.4278239611227,17.1822738180355,3.94697890588126));
#21200=CARTESIAN_POINT('Ctrl Pts',(-16.6393341928236,17.0468755746498,3.93600461211458));
#21201=CARTESIAN_POINT('Ctrl Pts',(-16.9928872705094,16.7076783661737,3.91519163962551));
#21202=CARTESIAN_POINT('Ctrl Pts',(-17.1336257165707,16.5091847997703,3.90614631670038));
#21203=CARTESIAN_POINT('Ctrl Pts',(-17.3382578393871,16.0599716762618,3.88649569887411));
#21204=CARTESIAN_POINT('Ctrl Pts',(-17.3961992884504,15.8117186546584,3.87563598664299));
#21205=CARTESIAN_POINT('Ctrl Pts',(-17.404691385027,15.5396074743704,3.86373261042742));
#21206=CARTESIAN_POINT('Ctrl Pts',(-17.405,15.5197975511803,3.86286603460973));
#21207=CARTESIAN_POINT('Ctrl Pts',(-17.405,15.5,3.86199999999992));
#21208=CARTESIAN_POINT('Origin',(-15.5,15.5,-1.713));
#21209=CARTESIAN_POINT('',(-17.405,15.5,3.29949999999987));
#21210=CARTESIAN_POINT('',(-17.405,15.5,3.36199999999991));
#21211=CARTESIAN_POINT('',(-17.405,15.5,-1.713));
#21212=CARTESIAN_POINT('Ctrl Pts',(-17.405,15.5,3.29949999999987));
#21213=CARTESIAN_POINT('Ctrl Pts',(-17.405,15.5564229479164,3.30196819544678));
#21214=CARTESIAN_POINT('Ctrl Pts',(-17.4024933261743,15.61291045123,3.30443921483919));
#21215=CARTESIAN_POINT('Ctrl Pts',(-17.3750365175576,15.9206454284538,3.31790093737742));
#21216=CARTESIAN_POINT('Ctrl Pts',(-17.3028873277189,16.1650760840202,3.32859344199538));
#21217=CARTESIAN_POINT('Ctrl Pts',(-17.0727241164517,16.601693105207,3.34769304922141));
#21218=CARTESIAN_POINT('Ctrl Pts',(-16.920751105621,16.79177744042,3.35726387446552));
#21219=CARTESIAN_POINT('Ctrl Pts',(-16.547073310477,17.1109838535724,3.37840200526172));
#21220=CARTESIAN_POINT('Ctrl Pts',(-16.3266549814992,17.234437712566,3.38945252152817));
#21221=CARTESIAN_POINT('Ctrl Pts',(-15.8504405112782,17.3891718533417,3.41087775771578));
#21222=CARTESIAN_POINT('Ctrl Pts',(-15.5992868634806,17.4188283703308,3.42043617098827));
#21223=CARTESIAN_POINT('Ctrl Pts',(-15.1065785124235,17.3798068533132,3.43995536202857));
#21224=CARTESIAN_POINT('Ctrl Pts',(-14.8695183682189,17.3140913580522,3.45037346591032));
#21225=CARTESIAN_POINT('Ctrl Pts',(-14.4244806486061,17.0926303898112,3.47207707286342));
#21226=CARTESIAN_POINT('Ctrl Pts',(-14.2224268061852,16.9356296381043,3.4831656177594));
#21227=CARTESIAN_POINT('Ctrl Pts',(-13.8981248505675,16.5593608623171,3.50368128354923));
#21228=CARTESIAN_POINT('Ctrl Pts',(-13.7760423459017,16.3462976357972,3.51247910604536));
#21229=CARTESIAN_POINT('Ctrl Pts',(-13.6176127567415,15.8826803267161,3.53275982822738));
#21230=CARTESIAN_POINT('Ctrl Pts',(-13.583937438819,15.6360843793156,3.54354705252312));
#21231=CARTESIAN_POINT('Ctrl Pts',(-13.6127634592529,15.1379732216046,3.56533669196804));
#21232=CARTESIAN_POINT('Ctrl Pts',(-13.6772757298006,14.8913758199954,3.57612397987746));
#21233=CARTESIAN_POINT('Ctrl Pts',(-13.8936967036479,14.4479014725849,3.59552355762946));
#21234=CARTESIAN_POINT('Ctrl Pts',(-14.0395619017465,14.2532993430224,3.60477444596417));
#21235=CARTESIAN_POINT('Ctrl Pts',(-14.4023361163371,13.9231773424532,3.62573825549865));
#21236=CARTESIAN_POINT('Ctrl Pts',(-14.6179938004087,13.7931610755427,3.63675195481547));
#21237=CARTESIAN_POINT('Ctrl Pts',(-15.0905715941891,13.622384990327,3.65839029327942));
#21238=CARTESIAN_POINT('Ctrl Pts',(-15.3433065988528,13.5846707710406,3.66833792298843));
#21239=CARTESIAN_POINT('Ctrl Pts',(-15.8387796964528,13.609669902849,3.68765515200495));
#21240=CARTESIAN_POINT('Ctrl Pts',(-16.0769668684721,13.6682775324893,3.69796048694128));
#21241=CARTESIAN_POINT('Ctrl Pts',(-16.5270481052016,13.8758106202084,3.71955052756395));
#21242=CARTESIAN_POINT('Ctrl Pts',(-16.7331152783245,14.02614274918,3.73064525509223));
#21243=CARTESIAN_POINT('Ctrl Pts',(-17.0692569141695,14.3926031635416,3.75139492276905));
#21244=CARTESIAN_POINT('Ctrl Pts',(-17.1983589291318,14.6030775710289,3.76026454816374));
#21245=CARTESIAN_POINT('Ctrl Pts',(-17.3641119979468,15.0459327355284,3.77963704004911));
#21246=CARTESIAN_POINT('Ctrl Pts',(-17.405,15.272129525868,3.78953191276751));
#21247=CARTESIAN_POINT('Ctrl Pts',(-17.405,15.5,3.79949999999988));
#21248=CARTESIAN_POINT('Ctrl Pts',(-17.405,15.5,3.86199999999992));
#21249=CARTESIAN_POINT('Ctrl Pts',(-17.405,15.2742109308075,3.85212296285239));
#21250=CARTESIAN_POINT('Ctrl Pts',(-17.3648553701787,15.0500311101823,3.84231632153029));
#21251=CARTESIAN_POINT('Ctrl Pts',(-17.2013040268939,14.6087211876983,3.82301142553361));
#21252=CARTESIAN_POINT('Ctrl Pts',(-17.0729962895187,14.3979574338972,3.81415369482636));
#21253=CARTESIAN_POINT('Ctrl Pts',(-16.7381842898046,14.0303834987862,3.79343004369775));
#21254=CARTESIAN_POINT('Ctrl Pts',(-16.5325589824563,13.8792948756376,3.78233550951582));
#21255=CARTESIAN_POINT('Ctrl Pts',(-16.0830251392004,13.6701864876885,3.76073175089401));
#21256=CARTESIAN_POINT('Ctrl Pts',(-15.8449545163795,13.6107769922595,3.75041329267126));
#21257=CARTESIAN_POINT('Ctrl Pts',(-15.3497889743819,13.5841913498518,3.73107301447124));
#21258=CARTESIAN_POINT('Ctrl Pts',(-15.0972352470335,13.6209853811416,3.72117335090165));
#21259=CARTESIAN_POINT('Ctrl Pts',(-14.6242311443009,13.7899391912535,3.69955871948796));
#21260=CARTESIAN_POINT('Ctrl Pts',(-14.4080235381815,13.919219244812,3.68854028964674));
#21261=CARTESIAN_POINT('Ctrl Pts',(-14.0440081901868,14.2481090815363,3.6675564113837));
#21262=CARTESIAN_POINT('Ctrl Pts',(-13.8974505145118,14.4421925951016,3.65827328980309));
#21263=CARTESIAN_POINT('Ctrl Pts',(-13.6794547169359,14.8848901646036,3.63890769183713));
#21264=CARTESIAN_POINT('Ctrl Pts',(-13.6140657478863,15.1312521894653,3.62813070037336));
#21265=CARTESIAN_POINT('Ctrl Pts',(-13.5834593005368,15.6293376228352,3.6063421862277));
#21266=CARTESIAN_POINT('Ctrl Pts',(-13.6162831343669,15.8761359329288,3.59554610967067));
#21267=CARTESIAN_POINT('Ctrl Pts',(-13.7731034757767,16.3402450791531,3.57524387230302));
#21268=CARTESIAN_POINT('Ctrl Pts',(-13.8943614984445,16.5536165703811,3.56644949459541));
#21269=CARTESIAN_POINT('Ctrl Pts',(-14.2172608701428,16.9310322330413,3.54596187910604));
#21270=CARTESIAN_POINT('Ctrl Pts',(-14.4188276118528,17.088812946621,3.53487472793943));
#21271=CARTESIAN_POINT('Ctrl Pts',(-14.8632427821596,17.3119091088748,3.51315894016867));
#21272=CARTESIAN_POINT('Ctrl Pts',(-15.1001561943329,17.3784618194619,3.50272808326872));
#21273=CARTESIAN_POINT('Ctrl Pts',(-15.5925331225056,17.4191295483254,3.48318544142854));
#21274=CARTESIAN_POINT('Ctrl Pts',(-15.8435045405407,17.3904080860209,3.4736675583809));
#21275=CARTESIAN_POINT('Ctrl Pts',(-16.3201269499146,17.2375475037393,3.4522678468467));
#21276=CARTESIAN_POINT('Ctrl Pts',(-16.5410892612555,17.1148718894886,3.44121374439588));
#21277=CARTESIAN_POINT('Ctrl Pts',(-16.916037209688,16.7969507213421,3.42005560649069));
#21278=CARTESIAN_POINT('Ctrl Pts',(-17.0687256345697,16.6073873393512,3.41044214082902));
#21279=CARTESIAN_POINT('Ctrl Pts',(-17.3004763667435,16.1715738534205,3.39137768387667));
#21280=CARTESIAN_POINT('Ctrl Pts',(-17.3735054583902,15.9274098964587,3.38069684586435));
#21281=CARTESIAN_POINT('Ctrl Pts',(-17.4022858919956,15.617489805707,3.36713953655762));
#21282=CARTESIAN_POINT('Ctrl Pts',(-17.405,15.5587111509317,3.3645682918167));
#21283=CARTESIAN_POINT('Ctrl Pts',(-17.405,15.5,3.36199999999991));
#21284=CARTESIAN_POINT('Origin',(-15.5,15.5,-1.713));
#21285=CARTESIAN_POINT('',(-17.405,15.5,2.79949999999986));
#21286=CARTESIAN_POINT('',(-17.405,15.5,2.86199999999991));
#21287=CARTESIAN_POINT('',(-17.405,15.5,-1.713));
#21288=CARTESIAN_POINT('Ctrl Pts',(-17.405,15.5,2.79949999999986));
#21289=CARTESIAN_POINT('Ctrl Pts',(-17.405,15.5944999131661,2.80363385446907));
#21290=CARTESIAN_POINT('Ctrl Pts',(-17.3979684804714,15.6890787995141,2.80777116358316));
#21291=CARTESIAN_POINT('Ctrl Pts',(-17.3463774788093,16.0325724073037,2.82279713067807));
#21292=CARTESIAN_POINT('Ctrl Pts',(-17.2596502024004,16.2722222104947,2.83306121295661));
#21293=CARTESIAN_POINT('Ctrl Pts',(-17.0030714688162,16.6952243150178,2.8520334244009));
#21294=CARTESIAN_POINT('Ctrl Pts',(-16.8389585105207,16.8765724635878,2.86221715428976));
#21295=CARTESIAN_POINT('Ctrl Pts',(-16.4440809776058,17.1736602906283,2.88367462972319));
#21296=CARTESIAN_POINT('Ctrl Pts',(-16.2148322932427,17.2836617476485,2.89476543956363));
#21297=CARTESIAN_POINT('Ctrl Pts',(-15.7321781580959,17.4067720537753,2.91574295029601));
#21298=CARTESIAN_POINT('Ctrl Pts',(-15.4840051051965,17.4207876543533,2.92476063683499));
#21299=CARTESIAN_POINT('Ctrl Pts',(-14.9971397146739,17.3537176806962,2.9446719571869));
#21300=CARTESIAN_POINT('Ctrl Pts',(-14.7629996406341,17.2736833185551,2.95529262355756));
#21301=CARTESIAN_POINT('Ctrl Pts',(-14.3294458847818,17.0244119172388,2.97716945064122));
#21302=CARTESIAN_POINT('Ctrl Pts',(-14.1361456673276,16.8542333088828,2.98821460388052));
#21303=CARTESIAN_POINT('Ctrl Pts',(-13.8361042007355,16.4585591815783,3.00823562732364));
#21304=CARTESIAN_POINT('Ctrl Pts',(-13.7280829228089,16.2400686139527,3.01712604488369));
#21305=CARTESIAN_POINT('Ctrl Pts',(-13.5977175306194,15.7680977558765,3.03777218915649));
#21306=CARTESIAN_POINT('Ctrl Pts',(-13.5790079742218,15.5183920020373,3.0486954504793));
#21307=CARTESIAN_POINT('Ctrl Pts',(-13.6388562736904,15.0216435275147,3.07042547998597));
#21308=CARTESIAN_POINT('Ctrl Pts',(-13.7185028504376,14.779600489273,3.08101353940162));
#21309=CARTESIAN_POINT('Ctrl Pts',(-13.9622301456127,14.349923249031,3.0998095691585));
#21310=CARTESIAN_POINT('Ctrl Pts',(-14.1203860318548,14.1642864361832,3.10978329125428));
#21311=CARTESIAN_POINT('Ctrl Pts',(-14.5049850693437,13.8562297834734,3.13109129051462));
#21312=CARTESIAN_POINT('Ctrl Pts',(-14.7300056668644,13.739560292438,3.14216776905116));
#21313=CARTESIAN_POINT('Ctrl Pts',(-15.2096239685188,13.6009694456039,3.16336886514782));
#21314=CARTESIAN_POINT('Ctrl Pts',(-15.4592287489489,13.5793327691483,3.1726127491432));
#21315=CARTESIAN_POINT('Ctrl Pts',(-15.9490213858857,13.6326010275756,3.19233309014878));
#21316=CARTESIAN_POINT('Ctrl Pts',(-16.1847102553598,13.7055771748497,3.2028580517407));
#21317=CARTESIAN_POINT('Ctrl Pts',(-16.62414775939,13.9411815613598,3.22465884942753));
#21318=CARTESIAN_POINT('Ctrl Pts',(-16.8218756183518,14.1049075031833,3.23573060444978));
#21319=CARTESIAN_POINT('Ctrl Pts',(-17.1339506675152,14.4910683301043,3.25599942920582));
#21320=CARTESIAN_POINT('Ctrl Pts',(-17.2488960307138,14.7068395714669,3.26480356830537));
#21321=CARTESIAN_POINT('Ctrl Pts',(-17.3765543584212,15.1206105897759,3.28290378782895));
#21322=CARTESIAN_POINT('Ctrl Pts',(-17.405,15.3099390455677,3.29118587250939));
#21323=CARTESIAN_POINT('Ctrl Pts',(-17.405,15.5,3.29949999999987));
#21324=CARTESIAN_POINT('Ctrl Pts',(-17.405,15.5,3.36199999999991));
#21325=CARTESIAN_POINT('Ctrl Pts',(-17.405,15.3121642442446,3.35378321278402));
#21326=CARTESIAN_POINT('Ctrl Pts',(-17.3772165691224,15.1250194340757,3.34559665065949));
#21327=CARTESIAN_POINT('Ctrl Pts',(-17.251673036774,14.7130224484878,3.32757403536692));
#21328=CARTESIAN_POINT('Ctrl Pts',(-17.1375440348227,14.4969355114396,3.31876388843797));
#21329=CARTESIAN_POINT('Ctrl Pts',(-16.8268793902558,14.1096485908813,3.29852386505512));
#21330=CARTESIAN_POINT('Ctrl Pts',(-16.6296619290207,13.9451577431649,3.2874547156519));
#21331=CARTESIAN_POINT('Ctrl Pts',(-16.1908952481043,13.7079383025191,3.26564400645109));
#21332=CARTESIAN_POINT('Ctrl Pts',(-15.9553778095696,13.6341302556848,3.2551073437992));
#21333=CARTESIAN_POINT('Ctrl Pts',(-15.465925329409,13.5792333586909,3.23536426723483));
#21334=CARTESIAN_POINT('Ctrl Pts',(-15.2164932530801,13.5999633821052,3.22615110516058));
#21335=CARTESIAN_POINT('Ctrl Pts',(-14.7365036590348,13.7367192091974,3.20497607910888));
#21336=CARTESIAN_POINT('Ctrl Pts',(-14.5109722524345,13.8526064231924,3.19389735931602));
#21337=CARTESIAN_POINT('Ctrl Pts',(-14.1251351188222,14.1593845568473,3.17257042028456));
#21338=CARTESIAN_POINT('Ctrl Pts',(-13.9662734753601,14.3445213777374,3.16254587149006));
#21339=CARTESIAN_POINT('Ctrl Pts',(-13.7210204081244,14.7734075803916,3.14378444530221));
#21340=CARTESIAN_POINT('Ctrl Pts',(-13.6405337707849,15.0151666662594,3.13320880725025));
#21341=CARTESIAN_POINT('Ctrl Pts',(-13.5789452302557,15.5117811349214,3.11148463976722));
#21342=CARTESIAN_POINT('Ctrl Pts',(-13.5968070574536,15.7616351175305,3.10055489424626));
#21343=CARTESIAN_POINT('Ctrl Pts',(-13.7255942596754,16.2340614020054,3.07988882755881));
#21344=CARTESIAN_POINT('Ctrl Pts',(-13.8328436761047,16.4528611452913,3.07098377759962));
#21345=CARTESIAN_POINT('Ctrl Pts',(-14.129967623663,16.8475094767687,3.05109571756475));
#21346=CARTESIAN_POINT('Ctrl Pts',(-14.3204097543996,17.0170100655722,3.04017366955205));
#21347=CARTESIAN_POINT('Ctrl Pts',(-14.7500930156158,17.2682891865639,3.01839955842826));
#21348=CARTESIAN_POINT('Ctrl Pts',(-14.9838155763777,17.3500745688595,3.00775641030031));
#21349=CARTESIAN_POINT('Ctrl Pts',(-15.4699399590987,17.4205642683659,2.98779836504272));
#21350=CARTESIAN_POINT('Ctrl Pts',(-15.7177700447031,17.4084159155821,2.9788247404591));
#21351=CARTESIAN_POINT('Ctrl Pts',(-16.2011385886972,17.2891163202623,2.95790351403087));
#21352=CARTESIAN_POINT('Ctrl Pts',(-16.4313993908793,17.1807796518502,2.94681077394374));
#21353=CARTESIAN_POINT('Ctrl Pts',(-16.8287792218349,16.8864311625419,2.92531841728524));
#21354=CARTESIAN_POINT('Ctrl Pts',(-16.9943376052565,16.7061607028033,2.91510350058699));
#21355=CARTESIAN_POINT('Ctrl Pts',(-17.2540594787777,16.2848470967839,2.89604914610767));
#21356=CARTESIAN_POINT('Ctrl Pts',(-17.3425113232036,16.0458060378014,2.88587602965012));
#21357=CARTESIAN_POINT('Ctrl Pts',(-17.3972762380981,15.6981581272708,2.8706683345263));
#21358=CARTESIAN_POINT('Ctrl Pts',(-17.405,15.599042312654,2.86633255960857));
#21359=CARTESIAN_POINT('Ctrl Pts',(-17.405,15.5000000000001,2.86199999999991));
#21360=CARTESIAN_POINT('Origin',(-15.5,15.5,-1.713));
#21361=CARTESIAN_POINT('',(-17.405,15.5,2.29949999999986));
#21362=CARTESIAN_POINT('',(-17.405,15.5,2.3619999999999));
#21363=CARTESIAN_POINT('',(-17.405,15.5,-1.713));
#21364=CARTESIAN_POINT('Ctrl Pts',(-17.405,15.5,2.29949999999986));
#21365=CARTESIAN_POINT('Ctrl Pts',(-17.405,15.6349750892016,2.30540442209967));
#21366=CARTESIAN_POINT('Ctrl Pts',(-17.3906547175841,15.7698930104027,2.31130634341201));
#21367=CARTESIAN_POINT('Ctrl Pts',(-17.3091350371661,16.1470568170573,2.32780519759638));
#21368=CARTESIAN_POINT('Ctrl Pts',(-17.2085948138019,16.3788277748054,2.33732709422014));
#21369=CARTESIAN_POINT('Ctrl Pts',(-16.9273133283528,16.7850161734643,2.35686738780469));
#21370=CARTESIAN_POINT('Ctrl Pts',(-16.751285560269,16.9569676813291,2.3672969710446));
#21371=CARTESIAN_POINT('Ctrl Pts',(-16.3359816313264,17.2304306746696,2.38901154888475));
#21372=CARTESIAN_POINT('Ctrl Pts',(-16.0985993472981,17.326183728861,2.40009884614951));
#21373=CARTESIAN_POINT('Ctrl Pts',(-15.6103272733066,17.4172942791093,2.42058927900862));
#21374=CARTESIAN_POINT('Ctrl Pts',(-15.3648986121507,17.4157081120999,2.42938395353938));
#21375=CARTESIAN_POINT('Ctrl Pts',(-14.8845200628733,17.3196284646875,2.44968403450236));
#21376=CARTESIAN_POINT('Ctrl Pts',(-14.654349264037,17.2247397227717,2.46047922828888));
#21377=CARTESIAN_POINT('Ctrl Pts',(-14.2382060120843,16.9493443709446,2.48226786799658));
#21378=CARTESIAN_POINT('Ctrl Pts',(-14.0574801656378,16.7695991333544,2.49304589918372));
#21379=CARTESIAN_POINT('Ctrl Pts',(-13.7829441267767,16.3595582698038,2.51241491124335));
#21380=CARTESIAN_POINT('Ctrl Pts',(-13.6880618743612,16.1356280757084,2.52169474734417));
#21381=CARTESIAN_POINT('Ctrl Pts',(-13.585073025739,15.6559826280725,2.54267661294504));
#21382=CARTESIAN_POINT('Ctrl Pts',(-13.5811253210558,15.4041120390609,2.55369457396917));
#21383=CARTESIAN_POINT('Ctrl Pts',(-13.6711292410151,14.9099469975137,2.57531159240956));
#21384=CARTESIAN_POINT('Ctrl Pts',(-13.7654706440895,14.6727701017159,2.585216030766));
#21385=CARTESIAN_POINT('Ctrl Pts',(-14.0359546772966,14.2571304573011,2.60455399517033));
#21386=CARTESIAN_POINT('Ctrl Pts',(-14.206376233983,14.0806094442151,2.61487113882675));
#21387=CARTESIAN_POINT('Ctrl Pts',(-14.6121268718779,13.7957288906123,2.63647352888887));
#21388=CARTESIAN_POINT('Ctrl Pts',(-14.8457425680365,13.6931198901864,2.64756808828558));
#21389=CARTESIAN_POINT('Ctrl Pts',(-15.3314469326937,13.586779428234,2.66829435904228));
#21390=CARTESIAN_POINT('Ctrl Pts',(-15.5781422579797,13.5809598700289,2.6771532421492));
#21391=CARTESIAN_POINT('Ctrl Pts',(-16.0616840103632,13.6631481801623,2.69726932248259));
#21392=CARTESIAN_POINT('Ctrl Pts',(-16.293876506192,13.7509258641659,2.70798557103718));
#21393=CARTESIAN_POINT('Ctrl Pts',(-16.7175546481377,14.0132918520873,2.72977467986982));
#21394=CARTESIAN_POINT('Ctrl Pts',(-16.9036363424498,14.1875346364906,2.74063526021344));
#21395=CARTESIAN_POINT('Ctrl Pts',(-17.1904876517898,14.589264042189,2.76028903203523));
#21396=CARTESIAN_POINT('Ctrl Pts',(-17.2920941372137,14.8103627739561,2.76933214234265));
#21397=CARTESIAN_POINT('Ctrl Pts',(-17.3865337341854,15.1939311843254,2.78611116291874));
#21398=CARTESIAN_POINT('Ctrl Pts',(-17.405,15.3468618982312,2.7928010454168));
#21399=CARTESIAN_POINT('Ctrl Pts',(-17.405,15.5,2.79949999999986));
#21400=CARTESIAN_POINT('Ctrl Pts',(-17.405,15.5000000000001,2.86199999999991));
#21401=CARTESIAN_POINT('Ctrl Pts',(-17.405,15.3512516229631,2.85549307187056));
#21402=CARTESIAN_POINT('Ctrl Pts',(-17.3875773407963,15.2026690372746,2.84899339620625));
#21403=CARTESIAN_POINT('Ctrl Pts',(-17.2968195960562,14.8227897877569,2.83237575624485));
#21404=CARTESIAN_POINT('Ctrl Pts',(-17.1967725884005,14.6010434309328,2.8232847717177));
#21405=CARTESIAN_POINT('Ctrl Pts',(-16.9127711516358,14.197373883066,2.80369652880942));
#21406=CARTESIAN_POINT('Ctrl Pts',(-16.7279167244992,14.0218399237571,2.79285420118227));
#21407=CARTESIAN_POINT('Ctrl Pts',(-16.3059501787976,13.7564329807281,2.7710634216705));
#21408=CARTESIAN_POINT('Ctrl Pts',(-16.0742075216153,13.6670024169188,2.76032806252068));
#21409=CARTESIAN_POINT('Ctrl Pts',(-15.5913913266025,13.5815869421211,2.74016888370885));
#21410=CARTESIAN_POINT('Ctrl Pts',(-15.3449980770684,13.5856759097506,2.73133186536444));
#21411=CARTESIAN_POINT('Ctrl Pts',(-14.8586778930605,13.6884627347192,2.71065999107711));
#21412=CARTESIAN_POINT('Ctrl Pts',(-14.6241660972474,13.789483754856,2.69956621667948));
#21413=CARTESIAN_POINT('Ctrl Pts',(-14.2161583938901,14.0717277875137,2.67793598691674));
#21414=CARTESIAN_POINT('Ctrl Pts',(-14.0444178943956,14.2471981421006,2.66759185687674));
#21415=CARTESIAN_POINT('Ctrl Pts',(-13.7714012327442,14.6606332321423,2.64820616529025));
#21416=CARTESIAN_POINT('Ctrl Pts',(-13.6755976023477,14.8965330213078,2.63839838052026));
#21417=CARTESIAN_POINT('Ctrl Pts',(-13.5818831565501,15.3895650821121,2.61683092379216));
#21418=CARTESIAN_POINT('Ctrl Pts',(-13.5839352941782,15.641650445142,2.60580356757912));
#21419=CARTESIAN_POINT('Ctrl Pts',(-13.6834194236602,16.122242903278,2.58478027544718));
#21420=CARTESIAN_POINT('Ctrl Pts',(-13.776655110423,16.3468820683731,2.57543042080797));
#21421=CARTESIAN_POINT('Ctrl Pts',(-14.0481663058559,16.7589361605946,2.55613196766852));
#21422=CARTESIAN_POINT('Ctrl Pts',(-14.2275563446959,16.940001960658,2.54537565835736));
#21423=CARTESIAN_POINT('Ctrl Pts',(-14.6417946261065,17.218552411423,2.52359017715421));
#21424=CARTESIAN_POINT('Ctrl Pts',(-14.8714381905177,17.315174747068,2.51277703942813));
#21425=CARTESIAN_POINT('Ctrl Pts',(-15.3510290654114,17.4146453191073,2.49243263141847));
#21426=CARTESIAN_POINT('Ctrl Pts',(-15.5961612290483,17.4180226750135,2.48364187534089));
#21427=CARTESIAN_POINT('Ctrl Pts',(-16.0850284715075,17.3306030497403,2.4632096240861));
#21428=CARTESIAN_POINT('Ctrl Pts',(-16.3232942738259,17.2365307721866,2.45212561811769));
#21429=CARTESIAN_POINT('Ctrl Pts',(-16.7408656001719,16.9658803597754,2.43038665999374));
#21430=CARTESIAN_POINT('Ctrl Pts',(-16.9182333572259,16.7950621087425,2.41993109967277));
#21431=CARTESIAN_POINT('Ctrl Pts',(-17.2021096654342,16.3911655021351,2.40034263083006));
#21432=CARTESIAN_POINT('Ctrl Pts',(-17.3041266818208,16.1606781246921,2.39090105532342));
#21433=CARTESIAN_POINT('Ctrl Pts',(-17.3895750341878,15.7798334598907,2.3742411837223));
#21434=CARTESIAN_POINT('Ctrl Pts',(-17.405,15.6399618896503,2.36812256735118));
#21435=CARTESIAN_POINT('Ctrl Pts',(-17.405,15.5,2.3619999999999));
#21436=CARTESIAN_POINT('Origin',(-15.5,15.5,-1.713));
#21437=CARTESIAN_POINT('',(-17.405,15.5,1.79949999999985));
#21438=CARTESIAN_POINT('',(-17.405,15.5,1.86199999999989));
#21439=CARTESIAN_POINT('',(-17.405,15.5,-1.713));
#21440=CARTESIAN_POINT('Ctrl Pts',(-17.405,15.5,1.79949999999985));
#21441=CARTESIAN_POINT('Ctrl Pts',(-17.405,15.6758129035626,1.80719085317407));
#21442=CARTESIAN_POINT('Ctrl Pts',(-17.3806596497542,15.8511550139008,1.81486111171898));
#21443=CARTESIAN_POINT('Ctrl Pts',(-17.2650749842631,16.2577005203566,1.83264525460857));
#21444=CARTESIAN_POINT('Ctrl Pts',(-17.1525410716862,16.4791337298434,1.84164454575853));
#21445=CARTESIAN_POINT('Ctrl Pts',(-16.8499756822054,16.8662860371983,1.86157479367078));
#21446=CARTESIAN_POINT('Ctrl Pts',(-16.6630641861499,17.0285411759165,1.87220461314595));
#21447=CARTESIAN_POINT('Ctrl Pts',(-16.2295355547136,17.2781584906455,1.8940880543295));
#21448=CARTESIAN_POINT('Ctrl Pts',(-15.9851780470513,17.3597553999023,1.90512997313393));
#21449=CARTESIAN_POINT('Ctrl Pts',(-15.4922789879605,17.4202338148899,1.92512569991292));
#21450=CARTESIAN_POINT('Ctrl Pts',(-15.2491564026104,17.4037967993866,1.93402924444523));
#21451=CARTESIAN_POINT('Ctrl Pts',(-14.7755901589679,17.279275854445,1.95469332449074));
#21452=CARTESIAN_POINT('Ctrl Pts',(-14.5502497144695,17.1698983391235,1.96562242803827));
#21453=CARTESIAN_POINT('Ctrl Pts',(-14.1508645276189,16.8683975242138,1.98734719291853));
#21454=CARTESIAN_POINT('Ctrl Pts',(-13.981671743571,16.6778728715177,1.99792407723483));
#21455=CARTESIAN_POINT('Ctrl Pts',(-13.7327272831338,16.2511267747944,2.01668896241555));
#21456=CARTESIAN_POINT('Ctrl Pts',(-13.6517464023149,16.0210162929489,2.02670838613501));
#21457=CARTESIAN_POINT('Ctrl Pts',(-13.5788147179765,15.5335256561171,2.04803343586519));
#21458=CARTESIAN_POINT('Ctrl Pts',(-13.5911258922105,15.280271092335,2.05911193821786));
#21459=CARTESIAN_POINT('Ctrl Pts',(-13.7125093691987,14.7961503166125,2.08028957495113));
#21460=CARTESIAN_POINT('Ctrl Pts',(-13.819202861008,14.5697105895712,2.08950576046523));
#21461=CARTESIAN_POINT('Ctrl Pts',(-14.1113472156176,14.1731698218157,2.10924656608824));
#21462=CARTESIAN_POINT('Ctrl Pts',(-14.2929621670787,14.0060531995224,2.11978206358689));
#21463=CARTESIAN_POINT('Ctrl Pts',(-14.7176774141026,13.7445407599599,2.1415917929429));
#21464=CARTESIAN_POINT('Ctrl Pts',(-14.9586987854945,13.6559083064524,2.15266120926984));
#21465=CARTESIAN_POINT('Ctrl Pts',(-15.4494045149217,13.5803297812339,2.17290411784708));
#21466=CARTESIAN_POINT('Ctrl Pts',(-15.6936192208834,13.5894481237492,2.18171361442766));
#21467=CARTESIAN_POINT('Ctrl Pts',(-16.1706231028332,13.6998629991341,2.2021993938312));
#21468=CARTESIAN_POINT('Ctrl Pts',(-16.3984748931021,13.8020710132237,2.21306682365253));
#21469=CARTESIAN_POINT('Ctrl Pts',(-16.8063914917534,14.0907294601935,2.23483389979174));
#21470=CARTESIAN_POINT('Ctrl Pts',(-16.9813964057174,14.2759936634906,2.24551591216831));
#21471=CARTESIAN_POINT('Ctrl Pts',(-17.2430957761371,14.6945050877789,2.26458389183068));
#21472=CARTESIAN_POINT('Ctrl Pts',(-17.3309992678079,14.9214828069085,2.27419303617254));
#21473=CARTESIAN_POINT('Ctrl Pts',(-17.3947425846049,15.2716869136996,2.28951255090531));
#21474=CARTESIAN_POINT('Ctrl Pts',(-17.405,15.3858638959536,2.29450716955163));
#21475=CARTESIAN_POINT('Ctrl Pts',(-17.405,15.5,2.29949999999986));
#21476=CARTESIAN_POINT('Ctrl Pts',(-17.405,15.5,2.3619999999999));
#21477=CARTESIAN_POINT('Ctrl Pts',(-17.405,15.3906515670809,2.35721660398419));
#21478=CARTESIAN_POINT('Ctrl Pts',(-17.3955851122864,15.2812480043357,2.35243079634019));
#21479=CARTESIAN_POINT('Ctrl Pts',(-17.3352956387922,14.935218870948,2.33729391386478));
#21480=CARTESIAN_POINT('Ctrl Pts',(-17.2490540991717,14.707498955458,2.32759382153132));
#21481=CARTESIAN_POINT('Ctrl Pts',(-16.9904162426923,14.286994913319,2.3085982408156));
#21482=CARTESIAN_POINT('Ctrl Pts',(-16.8167952691443,14.100447590647,2.29794059273781));
#21483=CARTESIAN_POINT('Ctrl Pts',(-16.4108947458734,13.808675505369,2.27618179102299));
#21484=CARTESIAN_POINT('Ctrl Pts',(-16.1836271957613,13.7047368876666,2.26529864226079));
#21485=CARTESIAN_POINT('Ctrl Pts',(-15.7074406505977,13.5909239280283,2.24476950294009));
#21486=CARTESIAN_POINT('Ctrl Pts',(-15.4634983903644,13.5800347208373,2.23594450211546));
#21487=CARTESIAN_POINT('Ctrl Pts',(-14.9722466215299,13.6519590091507,2.21576083389054));
#21488=CARTESIAN_POINT('Ctrl Pts',(-14.7303994517394,13.7388986235731,2.2046971593462));
#21489=CARTESIAN_POINT('Ctrl Pts',(-14.3035204103725,13.9975567011301,2.1828678884387));
#21490=CARTESIAN_POINT('Ctrl Pts',(-14.1206111259464,14.163511083443,2.17230877741255));
#21491=CARTESIAN_POINT('Ctrl Pts',(-13.8259323840979,14.5577807002497,2.15252163459544));
#21492=CARTESIAN_POINT('Ctrl Pts',(-13.7178134794438,14.7829929281575,2.14336513875066));
#21493=CARTESIAN_POINT('Ctrl Pts',(-13.5928113341082,15.2658892729356,2.12224106417595));
#21494=CARTESIAN_POINT('Ctrl Pts',(-13.5785939146864,15.5192387751817,2.1111584087846));
#21495=CARTESIAN_POINT('Ctrl Pts',(-13.6479843183902,16.0075214670508,2.08979871097755));
#21496=CARTESIAN_POINT('Ctrl Pts',(-13.7273296613187,16.23837962393,2.07969992896183));
#21497=CARTESIAN_POINT('Ctrl Pts',(-13.973326260038,16.6670166536837,2.06094940272588));
#21498=CARTESIAN_POINT('Ctrl Pts',(-14.1411412929859,16.8587584931067,2.05042637418511));
#21499=CARTESIAN_POINT('Ctrl Pts',(-14.5385852068307,17.1632354950527,2.02871005629614));
#21500=CARTESIAN_POINT('Ctrl Pts',(-14.763317098085,17.274253239104,2.01776813158519));
#21501=CARTESIAN_POINT('Ctrl Pts',(-15.2360771136105,17.4020132521351,1.99706374882692));
#21502=CARTESIAN_POINT('Ctrl Pts',(-15.4789633995476,17.4201194492865,1.98812764457752));
#21503=CARTESIAN_POINT('Ctrl Pts',(-15.9695743949547,17.363402239757,1.96830086460536));
#21504=CARTESIAN_POINT('Ctrl Pts',(-16.2121100361483,17.2848386351519,1.95739431041028));
#21505=CARTESIAN_POINT('Ctrl Pts',(-16.6463290172403,17.0411728993748,1.93561489062376));
#21506=CARTESIAN_POINT('Ctrl Pts',(-16.8351927338306,16.8807820766524,1.92495189028335));
#21507=CARTESIAN_POINT('Ctrl Pts',(-17.1416354883154,16.4971568914956,1.90495189891119));
#21508=CARTESIAN_POINT('Ctrl Pts',(-17.2563300345455,16.2775586051926,1.89601393723492));
#21509=CARTESIAN_POINT('Ctrl Pts',(-17.3785616890088,15.8658792821985,1.87800521794384));
#21510=CARTESIAN_POINT('Ctrl Pts',(-17.405,15.683232457912,1.87001541810628));
#21511=CARTESIAN_POINT('Ctrl Pts',(-17.405,15.5,1.86199999999989));
#21512=CARTESIAN_POINT('Origin',(-15.5,15.5,11.20575));
#21513=CARTESIAN_POINT('',(-15.5,13.5679367061317,1.22137499999989));
#21514=CARTESIAN_POINT('',(-15.5,13.5679367061317,1.3858));
#21515=CARTESIAN_POINT('',(-15.5,13.5679367061317,11.20575));
#21516=CARTESIAN_POINT('',(-17.2021646372135,16.4140591443298,1.3857999999999));
#21517=CARTESIAN_POINT('Origin',(-15.5,15.5,1.3858));
#21518=CARTESIAN_POINT('Ctrl Pts',(-17.2021646372131,16.4140591443306,1.38579999999995));
#21519=CARTESIAN_POINT('Ctrl Pts',(-17.2835044921692,16.2625877372984,1.3792667682509));
#21520=CARTESIAN_POINT('Ctrl Pts',(-17.3442533198926,16.1009564770173,1.37229532392361));
#21521=CARTESIAN_POINT('Ctrl Pts',(-17.4225863575886,15.7606826337724,1.35761870660277));
#21522=CARTESIAN_POINT('Ctrl Pts',(-17.4383899414388,15.583279243606,1.3499669822032));
#21523=CARTESIAN_POINT('Ctrl Pts',(-17.4173618065871,15.150545952148,1.33130242409274));
#21524=CARTESIAN_POINT('Ctrl Pts',(-17.354246909013,14.8998465932948,1.32048931393011));
#21525=CARTESIAN_POINT('Ctrl Pts',(-17.1389102320616,14.4480453999454,1.30100232322681));
#21526=CARTESIAN_POINT('Ctrl Pts',(-16.9927945769671,14.2493134357546,1.29183017937045));
#21527=CARTESIAN_POINT('Ctrl Pts',(-16.6281426362718,13.9112799548102,1.27091926226126));
#21528=CARTESIAN_POINT('Ctrl Pts',(-16.410884372517,13.7774947329751,1.25991876919078));
#21529=CARTESIAN_POINT('Ctrl Pts',(-15.9581594815713,13.6089622530652,1.23937348400477));
#21530=CARTESIAN_POINT('Ctrl Pts',(-15.7298816359758,13.5679367061317,1.22996181912958));
#21531=CARTESIAN_POINT('Ctrl Pts',(-15.5,13.5679367061317,1.22137499999989));
#21532=CARTESIAN_POINT('Origin',(-15.5,15.5,11.20575));
#21533=CARTESIAN_POINT('',(-15.5,13.5679367061317,0.721374999999882));
#21534=CARTESIAN_POINT('',(-15.5,13.5679367061317,1.19012499999984));
#21535=CARTESIAN_POINT('',(-15.5,13.5679367061317,11.20575));
#21536=CARTESIAN_POINT('',(-16.7089831815964,17.0070594673503,1.3858));
#21537=CARTESIAN_POINT('Ctrl Pts',(-15.5,13.5679367061317,1.19012499999984));
#21538=CARTESIAN_POINT('Ctrl Pts',(-15.6209597157618,13.5679367061317,1.19464323477234));
#21539=CARTESIAN_POINT('Ctrl Pts',(-15.7419184750194,13.5792946957063,1.19940637898293));
#21540=CARTESIAN_POINT('Ctrl Pts',(-16.1137167329605,13.6500674067386,1.21482051737712));
#21541=CARTESIAN_POINT('Ctrl Pts',(-16.3540308512701,13.7479960405399,1.22590894156164));
#21542=CARTESIAN_POINT('Ctrl Pts',(-16.7741136008819,14.026702340501,1.24761093429799));
#21543=CARTESIAN_POINT('Ctrl Pts',(-16.9519823816307,14.2016401214962,1.258027594988));
#21544=CARTESIAN_POINT('Ctrl Pts',(-17.2359894885833,14.6147032779413,1.27754424976214));
#21545=CARTESIAN_POINT('Ctrl Pts',(-17.3372359040119,14.8503902891215,1.28710617538617));
#21546=CARTESIAN_POINT('Ctrl Pts',(-17.4426537117389,15.3471703745469,1.30853318586947));
#21547=CARTESIAN_POINT('Ctrl Pts',(-17.4459126157984,15.6033601229582,1.31958310631912));
#21548=CARTESIAN_POINT('Ctrl Pts',(-17.357744835181,16.0780177664297,1.34005593645267));
#21549=CARTESIAN_POINT('Ctrl Pts',(-17.2762233318702,16.2939199281608,1.34923226468177));
#21550=CARTESIAN_POINT('Ctrl Pts',(-17.0408566361002,16.6881134566224,1.36652510317405));
#21551=CARTESIAN_POINT('Ctrl Pts',(-16.8884973676933,16.8630507957942,1.37598889193056));
#21552=CARTESIAN_POINT('Ctrl Pts',(-16.7089831815964,17.0070594673503,1.38579999999999));
#21553=CARTESIAN_POINT('Origin',(-15.5,15.5,1.3858));
#21554=CARTESIAN_POINT('Ctrl Pts',(-15.5,13.5679367061317,1.22137499999989));
#21555=CARTESIAN_POINT('Ctrl Pts',(-15.4729341637143,13.5679367061317,1.22036400388534));
#21556=CARTESIAN_POINT('Ctrl Pts',(-15.4458469977579,13.5685054395913,1.2193399457951));
#21557=CARTESIAN_POINT('Ctrl Pts',(-15.1726369387374,13.5800041737923,1.20888669013352));
#21558=CARTESIAN_POINT('Ctrl Pts',(-14.9307787644431,13.6373364196089,1.19861608777127));
#21559=CARTESIAN_POINT('Ctrl Pts',(-14.4729009299767,13.8436681823131,1.17706314833877));
#21560=CARTESIAN_POINT('Ctrl Pts',(-14.2627623231917,13.9941383691091,1.16596877123743));
#21561=CARTESIAN_POINT('Ctrl Pts',(-13.9183617245921,14.3628583035511,1.14515252623231));
#21562=CARTESIAN_POINT('Ctrl Pts',(-13.7853340431921,14.5755603823523,1.13624772831502));
#21563=CARTESIAN_POINT('Ctrl Pts',(-13.6069662800139,15.0402511769473,1.11620478613719));
#21564=CARTESIAN_POINT('Ctrl Pts',(-13.563518985263,15.2879321565451,1.10552186405143));
#21565=CARTESIAN_POINT('Ctrl Pts',(-13.5731954041822,15.7929752639186,1.08373845470453));
#21566=CARTESIAN_POINT('Ctrl Pts',(-13.628926931347,16.0454493143052,1.07284879893307));
#21567=CARTESIAN_POINT('Ctrl Pts',(-13.8310245097158,16.5036338505738,1.05308648327279));
#21568=CARTESIAN_POINT('Ctrl Pts',(-13.9714260897244,16.7067442547807,1.0441143077112));
#21569=CARTESIAN_POINT('Ctrl Pts',(-14.3257784403693,17.0548537163586,1.02337081594498));
#21570=CARTESIAN_POINT('Ctrl Pts',(-14.5383567467269,17.1945806683055,1.01241699564406));
#21571=CARTESIAN_POINT('Ctrl Pts',(-15.0088443360005,17.3860429606324,0.990713714656131));
#21572=CARTESIAN_POINT('Ctrl Pts',(-15.2627143703035,17.4344332046964,0.980289491368659));
#21573=CARTESIAN_POINT('Ctrl Pts',(-15.764107690538,17.4296140644544,0.961456907738265));
#21574=CARTESIAN_POINT('Ctrl Pts',(-16.0069337839783,17.3804673298746,0.951326678324261));
#21575=CARTESIAN_POINT('Ctrl Pts',(-16.4699471299709,17.1903012304531,0.929930537938738));
#21576=CARTESIAN_POINT('Ctrl Pts',(-16.6843681043685,17.0476412723927,0.918844635164113));
#21577=CARTESIAN_POINT('Ctrl Pts',(-17.0422253707064,16.6904570711204,0.897774518665517));
#21578=CARTESIAN_POINT('Ctrl Pts',(-17.1834288053771,16.4806668481729,0.888672908979973));
#21579=CARTESIAN_POINT('Ctrl Pts',(-17.3770350149237,16.0208578484158,0.868840527314208));
#21580=CARTESIAN_POINT('Ctrl Pts',(-17.42837351161,15.7755220883528,0.858258758726811));
#21581=CARTESIAN_POINT('Ctrl Pts',(-17.4355092606312,15.2690019284845,0.836411641473291));
#21582=CARTESIAN_POINT('Ctrl Pts',(-17.3873412235869,15.0126438266187,0.825354459639089));
#21583=CARTESIAN_POINT('Ctrl Pts',(-17.1979533839632,14.5460700127244,0.805230299482811));
#21584=CARTESIAN_POINT('Ctrl Pts',(-17.063281790105,14.3384565933621,0.796385555323458));
#21585=CARTESIAN_POINT('Ctrl Pts',(-16.7193021674531,13.9803614873582,0.775814169018619));
#21586=CARTESIAN_POINT('Ctrl Pts',(-16.5115619839701,13.8348471766509,0.764916258632763));
#21587=CARTESIAN_POINT('Ctrl Pts',(-16.0477927715656,13.6296318245785,0.743167333659146));
#21588=CARTESIAN_POINT('Ctrl Pts',(-15.7954972631553,13.5735885359089,0.732534660777732));
#21589=CARTESIAN_POINT('Ctrl Pts',(-15.5263956112966,13.568071880497,0.722363876209219));
#21590=CARTESIAN_POINT('Ctrl Pts',(-15.5131950985184,13.5679367061317,0.721867879406689));
#21591=CARTESIAN_POINT('Ctrl Pts',(-15.5,13.5679367061317,0.721374999999882));
#21592=CARTESIAN_POINT('Origin',(-15.5,15.5,11.20575));
#21593=CARTESIAN_POINT('',(-15.5000000000001,13.5679367061317,0.22137499999988));
#21594=CARTESIAN_POINT('',(-15.5,13.5679367061317,0.69012499999983));
#21595=CARTESIAN_POINT('',(-15.5,13.5679367061317,11.20575));
#21596=CARTESIAN_POINT('Ctrl Pts',(-15.5,13.5679367061317,0.690124999999832));
#21597=CARTESIAN_POINT('Ctrl Pts',(-15.663197634803,13.5679367061317,0.696220957019179));
#21598=CARTESIAN_POINT('Ctrl Pts',(-15.8260698424807,13.5886111528802,0.702750621155672));
#21599=CARTESIAN_POINT('Ctrl Pts',(-16.2318407735952,13.6937750358444,0.720175424526367));
#21600=CARTESIAN_POINT('Ctrl Pts',(-16.4638288993578,13.8061679673983,0.731264781557265));
#21601=CARTESIAN_POINT('Ctrl Pts',(-16.8630470507188,14.108833797682,0.75270412300508));
#21602=CARTESIAN_POINT('Ctrl Pts',(-17.028761444196,14.2932884830899,0.762872018728106));
#21603=CARTESIAN_POINT('Ctrl Pts',(-17.2874053587738,14.7231251438683,0.781803012187292));
#21604=CARTESIAN_POINT('Ctrl Pts',(-17.3745003706305,14.9664736216104,0.79211305640892));
#21605=CARTESIAN_POINT('Ctrl Pts',(-17.4482099203794,15.4692792372004,0.813799958747375));
#21606=CARTESIAN_POINT('Ctrl Pts',(-17.4355847239787,15.723565875171,0.824767794651858));
#21607=CARTESIAN_POINT('Ctrl Pts',(-17.3151733744223,16.2055976541615,0.845558684393085));
#21608=CARTESIAN_POINT('Ctrl Pts',(-17.2113496874164,16.4295122772777,0.854579673980927));
#21609=CARTESIAN_POINT('Ctrl Pts',(-16.9190154733788,16.8359718966524,0.874264961849426));
#21610=CARTESIAN_POINT('Ctrl Pts',(-16.7296891979234,17.0120418978351,0.885134014187554));
#21611=CARTESIAN_POINT('Ctrl Pts',(-16.2991617620683,17.2766178136154,0.906921415251217));
#21612=CARTESIAN_POINT('Ctrl Pts',(-16.0634585876014,17.3648212635817,0.917627873583943));
#21613=CARTESIAN_POINT('Ctrl Pts',(-15.5727030691474,17.4465792698414,0.93772235628183));
#21614=CARTESIAN_POINT('Ctrl Pts',(-15.3223565583377,17.4398199793547,0.946593274573898));
#21615=CARTESIAN_POINT('Ctrl Pts',(-14.8300711076984,17.3302144103329,0.967345462670996));
#21616=CARTESIAN_POINT('Ctrl Pts',(-14.5935881752468,17.2253688342268,0.978439949755269));
#21617=CARTESIAN_POINT('Ctrl Pts',(-14.1832015334446,16.9351538432142,1.00002795682994));
#21618=CARTESIAN_POINT('Ctrl Pts',(-14.0110153602745,16.755615830377,1.01033156193278));
#21619=CARTESIAN_POINT('Ctrl Pts',(-13.7379425524706,16.3329965553295,1.02964587164791));
#21620=CARTESIAN_POINT('Ctrl Pts',(-13.6429845085471,16.0918227958046,1.03959862802551));
#21621=CARTESIAN_POINT('Ctrl Pts',(-13.5535333316269,15.5900949475556,1.06123904433767));
#21622=CARTESIAN_POINT('Ctrl Pts',(-13.5584675814187,15.3347633934782,1.07225194933617));
#21623=CARTESIAN_POINT('Ctrl Pts',(-13.6646353766633,14.8487842127048,1.09321309755165));
#21624=CARTESIAN_POINT('Ctrl Pts',(-13.761672278608,14.6220240391691,1.10246053097514));
#21625=CARTESIAN_POINT('Ctrl Pts',(-14.041585270235,14.2071591450873,1.12186311344001));
#21626=CARTESIAN_POINT('Ctrl Pts',(-14.2255255819044,14.0255156909769,1.13265117917155));
#21627=CARTESIAN_POINT('Ctrl Pts',(-14.648495420734,13.74776419308,1.1544404228268));
#21628=CARTESIAN_POINT('Ctrl Pts',(-14.8821830753995,13.6523788496886,1.16522647893842));
#21629=CARTESIAN_POINT('Ctrl Pts',(-15.2505243179915,13.5800170676889,1.18054575641211));
#21630=CARTESIAN_POINT('Ctrl Pts',(-15.3752528162562,13.5679367061317,1.18546529110574));
#21631=CARTESIAN_POINT('Ctrl Pts',(-15.5,13.5679367061317,1.19012499999984));
#21632=CARTESIAN_POINT('Ctrl Pts',(-15.5,13.5679367061317,0.721374999999882));
#21633=CARTESIAN_POINT('Ctrl Pts',(-15.2685828063486,13.5679367061317,0.712730822847808));
#21634=CARTESIAN_POINT('Ctrl Pts',(-15.0388969708039,13.6095133452991,0.703254680220421));
#21635=CARTESIAN_POINT('Ctrl Pts',(-14.5838672575743,13.7800568344395,0.682579933296358));
#21636=CARTESIAN_POINT('Ctrl Pts',(-14.3657373188852,13.9154007888411,0.67151326490416));
#21637=CARTESIAN_POINT('Ctrl Pts',(-13.9955563283149,14.2617096427834,0.650217354190035));
#21638=CARTESIAN_POINT('Ctrl Pts',(-13.8467023152938,14.4688321611842,0.640851106713065));
#21639=CARTESIAN_POINT('Ctrl Pts',(-13.6392165648734,14.9240794292194,0.621215480666726));
#21640=CARTESIAN_POINT('Ctrl Pts',(-13.5807974420006,15.1670698897687,0.610734869027327));
#21641=CARTESIAN_POINT('Ctrl Pts',(-13.5584324818228,15.6716078298641,0.588973248445474));
#21642=CARTESIAN_POINT('Ctrl Pts',(-13.598542278736,15.9284928588798,0.577893339304166));
#21643=CARTESIAN_POINT('Ctrl Pts',(-13.773173526214,16.4008511610958,0.557519683857022));
#21644=CARTESIAN_POINT('Ctrl Pts',(-13.9018579853462,16.6132862458172,0.54872840560789));
#21645=CARTESIAN_POINT('Ctrl Pts',(-14.2349802267053,16.9816699616753,0.528340694405922));
#21646=CARTESIAN_POINT('Ctrl Pts',(-14.4375333639109,17.1330265345501,0.517510543306561));
#21647=CARTESIAN_POINT('Ctrl Pts',(-14.8940137700958,17.3523384610088,0.495729873520459));
#21648=CARTESIAN_POINT('Ctrl Pts',(-15.1444779567369,17.4162475185621,0.484995974086985));
#21649=CARTESIAN_POINT('Ctrl Pts',(-15.644292945993,17.4421185607808,0.465768343173262));
#21650=CARTESIAN_POINT('Ctrl Pts',(-15.8886689106846,17.4083000037079,0.456344488469386));
#21651=CARTESIAN_POINT('Ctrl Pts',(-16.3602738338657,17.2484328206968,0.435280848151098));
#21652=CARTESIAN_POINT('Ctrl Pts',(-16.5819407282909,17.1206457359146,0.424245033703684));
#21653=CARTESIAN_POINT('Ctrl Pts',(-16.9645889726516,16.7856687238997,0.402727812195782));
#21654=CARTESIAN_POINT('Ctrl Pts',(-17.1213576046383,16.5812682862177,0.393012028302294));
#21655=CARTESIAN_POINT('Ctrl Pts',(-17.3428309783919,16.130730045467,0.373579510995516));
#21656=CARTESIAN_POINT('Ctrl Pts',(-17.4082697839647,15.8902976976571,0.363209235317829));
#21657=CARTESIAN_POINT('Ctrl Pts',(-17.4458200822696,15.3881980765453,0.341552783779496));
#21658=CARTESIAN_POINT('Ctrl Pts',(-17.4137884813012,15.1310281688062,0.330460587311118));
#21659=CARTESIAN_POINT('Ctrl Pts',(-17.2540504948445,14.6530287775216,0.309843621638471));
#21660=CARTESIAN_POINT('Ctrl Pts',(-17.1313390172738,14.4356759590614,0.301024334102504));
#21661=CARTESIAN_POINT('Ctrl Pts',(-16.8090342643691,14.0571971876884,0.280822982049281));
#21662=CARTESIAN_POINT('Ctrl Pts',(-16.6117620423532,13.9002426534532,0.27006936510708));
#21663=CARTESIAN_POINT('Ctrl Pts',(-16.1629040887197,13.6672548471105,0.248278485924882));
#21664=CARTESIAN_POINT('Ctrl Pts',(-15.9144966796287,13.5956339334636,0.237455100705018));
#21665=CARTESIAN_POINT('Ctrl Pts',(-15.6062624045507,13.5701259723312,0.225391456362187));
#21666=CARTESIAN_POINT('Ctrl Pts',(-15.5531033073173,13.5679367061317,0.223358579476269));
#21667=CARTESIAN_POINT('Ctrl Pts',(-15.5000000000001,13.5679367061317,0.221374999999879));
#21668=CARTESIAN_POINT('Origin',(-15.5,15.5,11.20575));
#21669=CARTESIAN_POINT('',(-15.5,13.5679367061317,-0.278625000000132));
#21670=CARTESIAN_POINT('',(-15.4999999999999,13.5679367061317,0.190124999999821));
#21671=CARTESIAN_POINT('',(-15.5,13.5679367061317,11.20575));
#21672=CARTESIAN_POINT('Ctrl Pts',(-15.4999999999999,13.5679367061317,0.190124999999821));
#21673=CARTESIAN_POINT('Ctrl Pts',(-15.7052232055908,13.5679367061317,0.197790747375166));
#21674=CARTESIAN_POINT('Ctrl Pts',(-15.9094431243975,13.6006312438211,0.206124105599975));
#21675=CARTESIAN_POINT('Ctrl Pts',(-16.3458500952319,13.7445092392223,0.225528168010864));
#21676=CARTESIAN_POINT('Ctrl Pts',(-16.5687690248994,13.8706006648951,0.236574181605322));
#21677=CARTESIAN_POINT('Ctrl Pts',(-16.9462938014503,14.1957983248931,0.257689124656267));
#21678=CARTESIAN_POINT('Ctrl Pts',(-17.0996068020759,14.3891741439698,0.267213101031684));
#21679=CARTESIAN_POINT('Ctrl Pts',(-17.3312210666002,14.8328987043052,0.286351732158294));
#21680=CARTESIAN_POINT('Ctrl Pts',(-17.403389189678,15.0810963874238,0.297056940587811));
#21681=CARTESIAN_POINT('Ctrl Pts',(-17.4463663432178,15.5859112111088,0.318830503652368));
#21682=CARTESIAN_POINT('Ctrl Pts',(-17.4188098289701,15.8374917549287,0.329681620893123));
#21683=CARTESIAN_POINT('Ctrl Pts',(-17.2705600347068,16.3114416099335,0.350123922848633));
#21684=CARTESIAN_POINT('Ctrl Pts',(-17.1530549287722,16.5299161239957,0.358922469304659));
#21685=CARTESIAN_POINT('Ctrl Pts',(-16.8349526369196,16.9202726297615,0.379222999836067));
#21686=CARTESIAN_POINT('Ctrl Pts',(-16.6338441663768,17.085451210082,0.390297271892839));
#21687=CARTESIAN_POINT('Ctrl Pts',(-16.1874197433205,17.3225641667436,0.412086213416755));
#21688=CARTESIAN_POINT('Ctrl Pts',(-15.9481982603318,17.3956324394973,0.422597688314654));
#21689=CARTESIAN_POINT('Ctrl Pts',(-15.4510757841914,17.4478128352924,0.442292129851002));
#21690=CARTESIAN_POINT('Ctrl Pts',(-15.1977325915627,17.4248413113895,0.451571409240313));
#21691=CARTESIAN_POINT('Ctrl Pts',(-14.7117348553567,17.2822086107985,0.472800990486173));
#21692=CARTESIAN_POINT('Ctrl Pts',(-14.4841033890512,17.1630032804563,0.483874527712213));
#21693=CARTESIAN_POINT('Ctrl Pts',(-14.0954494858794,16.8491384993429,0.505160775836598));
#21694=CARTESIAN_POINT('Ctrl Pts',(-13.935845283737,16.6603046231705,0.515078993620139));
#21695=CARTESIAN_POINT('Ctrl Pts',(-13.6903827463215,16.223642546113,0.533913007255683));
#21696=CARTESIAN_POINT('Ctrl Pts',(-13.6105539996563,15.9778499407052,0.544514480397023));
#21697=CARTESIAN_POINT('Ctrl Pts',(-13.5518158441316,15.4739117712167,0.566250231803642));
#21698=CARTESIAN_POINT('Ctrl Pts',(-13.571742794709,15.2208352901084,0.577165871485818));
#21699=CARTESIAN_POINT('Ctrl Pts',(-13.7057278794298,14.742684868917,0.597789351347523));
#21700=CARTESIAN_POINT('Ctrl Pts',(-13.8161488953126,14.5214408844327,0.606664573343451));
#21701=CARTESIAN_POINT('Ctrl Pts',(-14.1219606735895,14.1213400688706,0.626716158351945));
#21702=CARTESIAN_POINT('Ctrl Pts',(-14.318568611901,13.9495491173579,0.637764922719238));
#21703=CARTESIAN_POINT('Ctrl Pts',(-14.7590310485592,13.6984440207756,0.659632917824901));
#21704=CARTESIAN_POINT('Ctrl Pts',(-14.9966959458147,13.6181551918391,0.670241966963359));
#21705=CARTESIAN_POINT('Ctrl Pts',(-15.3284077888473,13.5736457522818,0.683592357862532));
#21706=CARTESIAN_POINT('Ctrl Pts',(-15.4142441778543,13.5679367061317,0.686921743980895));
#21707=CARTESIAN_POINT('Ctrl Pts',(-15.5,13.5679367061317,0.69012499999983));
#21708=CARTESIAN_POINT('Ctrl Pts',(-15.5000000000001,13.5679367061317,0.221374999999879));
#21709=CARTESIAN_POINT('Ctrl Pts',(-15.3093450221423,13.5679367061317,0.214253422827828));
#21710=CARTESIAN_POINT('Ctrl Pts',(-15.1194546083814,13.5961535790767,0.206551882575901));
#21711=CARTESIAN_POINT('Ctrl Pts',(-14.6948718232558,13.7256105046371,0.187900494787472));
#21712=CARTESIAN_POINT('Ctrl Pts',(-14.4700098904008,13.8459724738417,0.176905464603589));
#21713=CARTESIAN_POINT('Ctrl Pts',(-14.0753526090742,14.1696924217256,0.155182435525569));
#21714=CARTESIAN_POINT('Ctrl Pts',(-13.9107790537501,14.3714265999853,0.145052382171085));
#21715=CARTESIAN_POINT('Ctrl Pts',(-13.6758632413355,14.8173319838793,0.125819688237564));
#21716=CARTESIAN_POINT('Ctrl Pts',(-13.6037990124408,15.0551292052584,0.115563070259359));
#21717=CARTESIAN_POINT('Ctrl Pts',(-13.5518334963172,15.5544792850638,0.0940252113380078));
#21718=CARTESIAN_POINT('Ctrl Pts',(-13.5761558231528,15.8116932971635,0.0829311125699534));
#21719=CARTESIAN_POINT('Ctrl Pts',(-13.7215598037034,16.2949297857371,0.0620882615572829));
#21720=CARTESIAN_POINT('Ctrl Pts',(-13.8385708540846,16.5170608745389,0.0531675695736204));
#21721=CARTESIAN_POINT('Ctrl Pts',(-14.1505967901205,16.9049967004005,0.0331462146120232));
#21722=CARTESIAN_POINT('Ctrl Pts',(-14.3427581391604,17.0670614604204,0.0224732986552362));
#21723=CARTESIAN_POINT('Ctrl Pts',(-14.7840616507215,17.3126898337665,0.000691997111495622));
#21724=CARTESIAN_POINT('Ctrl Pts',(-15.0303088811274,17.3915129002971,-0.0102060193255635));
#21725=CARTESIAN_POINT('Ctrl Pts',(-15.5280187230135,17.4473055261743,-0.0300003018240521));
#21726=CARTESIAN_POINT('Ctrl Pts',(-15.7742335758728,17.4281050083783,-0.0389538708149526));
#21727=CARTESIAN_POINT('Ctrl Pts',(-16.2532901705975,17.296907710707,-0.0596775634273534));
#21728=CARTESIAN_POINT('Ctrl Pts',(-16.4808992967149,17.1834947938276,-0.0706253476172892));
#21729=CARTESIAN_POINT('Ctrl Pts',(-16.8829707781072,16.8732369847255,-0.0923349979158201));
#21730=CARTESIAN_POINT('Ctrl Pts',(-17.0524923783306,16.6781753243463,-0.102808198428218));
#21731=CARTESIAN_POINT('Ctrl Pts',(-17.3005030645304,16.2425026235966,-0.121599538500263));
#21732=CARTESIAN_POINT('Ctrl Pts',(-17.3801675176942,16.0080032121443,-0.131713916058721));
#21733=CARTESIAN_POINT('Ctrl Pts',(-17.4487724674381,15.5123656486931,-0.153091647532988));
#21734=CARTESIAN_POINT('Ctrl Pts',(-17.4333995515655,15.2553808907698,-0.164175858159823));
#21735=CARTESIAN_POINT('Ctrl Pts',(-17.3048200987405,14.7662503100071,-0.185272931873504));
#21736=CARTESIAN_POINT('Ctrl Pts',(-17.1944566843434,14.5384527982996,-0.194401543720054));
#21737=CARTESIAN_POINT('Ctrl Pts',(-16.894334784917,14.139727275418,-0.214210934024622));
#21738=CARTESIAN_POINT('Ctrl Pts',(-16.708188966555,13.9720032635188,-0.224781197355577));
#21739=CARTESIAN_POINT('Ctrl Pts',(-16.2741834170983,13.7111048249335,-0.246619209086019));
#21740=CARTESIAN_POINT('Ctrl Pts',(-16.0284985549801,13.6237773096857,-0.257679625272395));
#21741=CARTESIAN_POINT('Ctrl Pts',(-15.6823226738687,13.574383016875,-0.271675640769364));
#21742=CARTESIAN_POINT('Ctrl Pts',(-15.5911253193961,13.5679367061317,-0.275221175973618));
#21743=CARTESIAN_POINT('Ctrl Pts',(-15.5,13.5679367061317,-0.278625000000132));
#21744=CARTESIAN_POINT('Origin',(-15.5,15.5,11.20575));
#21745=CARTESIAN_POINT('',(-15.5,13.5679367061317,-0.778625000000138));
#21746=CARTESIAN_POINT('',(-15.5000000000213,13.5679367061317,-0.30987499999859));
#21747=CARTESIAN_POINT('',(-15.5,13.5679367061317,11.20575));
#21748=CARTESIAN_POINT('Ctrl Pts',(-15.5000000000426,13.5679367061317,-0.30987499999859));
#21749=CARTESIAN_POINT('Ctrl Pts',(-15.7451189900435,13.5679367061371,-0.300719016644455));
#21750=CARTESIAN_POINT('Ctrl Pts',(-15.9880788836297,13.6145849104549,-0.290637672395874));
#21751=CARTESIAN_POINT('Ctrl Pts',(-16.4525087353532,13.7998506160078,-0.269294302322051));
#21752=CARTESIAN_POINT('Ctrl Pts',(-16.6681650113368,13.9401358945745,-0.258213469136004));
#21753=CARTESIAN_POINT('Ctrl Pts',(-17.0300510391149,14.293798813587,-0.237068805018263));
#21754=CARTESIAN_POINT('Ctrl Pts',(-17.1737375672253,14.5027181075033,-0.227889545454448));
#21755=CARTESIAN_POINT('Ctrl Pts',(-17.3718881645073,14.9610456268797,-0.208121062677908));
#21756=CARTESIAN_POINT('Ctrl Pts',(-17.4255568606796,15.2056351161721,-0.197571482078929));
#21757=CARTESIAN_POINT('Ctrl Pts',(-17.437485526191,15.7028273877144,-0.176126693273793));
#21758=CARTESIAN_POINT('Ctrl Pts',(-17.3951930471992,15.9508283805331,-0.16542996844748));
#21759=CARTESIAN_POINT('Ctrl Pts',(-17.21903750586,16.416216845007,-0.145356934524323));
#21760=CARTESIAN_POINT('Ctrl Pts',(-17.087177913888,16.6293413959128,-0.136472617530199));
#21761=CARTESIAN_POINT('Ctrl Pts',(-16.7447233478944,16.9997020048593,-0.115693680499745));
#21762=CARTESIAN_POINT('Ctrl Pts',(-16.535223519972,17.1512859841674,-0.104599143917208));
#21763=CARTESIAN_POINT('Ctrl Pts',(-16.0781299074097,17.3599329092899,-0.0830255691567));
#21764=CARTESIAN_POINT('Ctrl Pts',(-15.8364334516315,17.4184418092008,-0.0727356319075368));
#21765=CARTESIAN_POINT('Ctrl Pts',(-15.3335771418074,17.4419572678446,-0.053445198139043));
#21766=CARTESIAN_POINT('Ctrl Pts',(-15.0770448720173,17.4026393126747,-0.0434417100341447));
#21767=CARTESIAN_POINT('Ctrl Pts',(-14.5982616364445,17.2273302215971,-0.0217769181315668));
#21768=CARTESIAN_POINT('Ctrl Pts',(-14.3801849192581,17.0946215718084,-0.010769070426221));
#21769=CARTESIAN_POINT('Ctrl Pts',(-14.0137016048736,16.7583973031524,0.0101712371105013));
#21770=CARTESIAN_POINT('Ctrl Pts',(-13.8665662971669,16.5604348396372,0.0193865553793818));
#21771=CARTESIAN_POINT('Ctrl Pts',(-13.648896034541,16.1097762694873,0.0388242627076077));
#21772=CARTESIAN_POINT('Ctrl Pts',(-13.5844810246986,15.8594139033154,0.0496228377752732));
#21773=CARTESIAN_POINT('Ctrl Pts',(-13.5572975229277,15.3542160204944,0.0714129228630835));
#21774=CARTESIAN_POINT('Ctrl Pts',(-13.5924291711366,15.1043600205154,0.0821896574543688));
#21775=CARTESIAN_POINT('Ctrl Pts',(-13.7549549306398,14.6347353821394,0.10244540510795));
#21776=CARTESIAN_POINT('Ctrl Pts',(-13.8797188217565,14.4190031858112,0.111248274994825));
#21777=CARTESIAN_POINT('Ctrl Pts',(-14.2102312356738,14.0387180251795,0.131795166002758));
#21778=CARTESIAN_POINT('Ctrl Pts',(-14.4157066951986,13.8803875205858,0.142884874300423));
#21779=CARTESIAN_POINT('Ctrl Pts',(-14.8677637645238,13.6576628179057,0.164573917775849));
#21780=CARTESIAN_POINT('Ctrl Pts',(-15.1083498919245,13.5919750720435,0.174977198896067));
#21781=CARTESIAN_POINT('Ctrl Pts',(-15.4031822744539,13.569754032749,0.186469354010824));
#21782=CARTESIAN_POINT('Ctrl Pts',(-15.4516175612204,13.5679367061317,0.188317760160552));
#21783=CARTESIAN_POINT('Ctrl Pts',(-15.4999999999999,13.5679367061317,0.190124999999822));
#21784=CARTESIAN_POINT('Ctrl Pts',(-15.5,13.5679367061317,-0.278625000000131));
#21785=CARTESIAN_POINT('Ctrl Pts',(-15.3467892597189,13.5679367061317,-0.284347914359666));
#21786=CARTESIAN_POINT('Ctrl Pts',(-15.1938118281016,13.5861582264254,-0.290455077212558));
#21787=CARTESIAN_POINT('Ctrl Pts',(-14.8002115590521,13.6816903721264,-0.30721755017852));
#21788=CARTESIAN_POINT('Ctrl Pts',(-14.5700164472504,13.7879612604545,-0.318107905048228));
#21789=CARTESIAN_POINT('Ctrl Pts',(-14.1593674324255,14.0854112710006,-0.339861742243558));
#21790=CARTESIAN_POINT('Ctrl Pts',(-13.9839732656644,14.2752366145712,-0.350507031688753));
#21791=CARTESIAN_POINT('Ctrl Pts',(-13.7231840673424,14.7026885542338,-0.369466729765817));
#21792=CARTESIAN_POINT('Ctrl Pts',(-13.6365422675758,14.9340075266013,-0.37921273586801));
#21793=CARTESIAN_POINT('Ctrl Pts',(-13.5527035685452,15.4259040924359,-0.400429111447581));
#21794=CARTESIAN_POINT('Ctrl Pts',(-13.5598498556332,15.6824101504194,-0.411492674857324));
#21795=CARTESIAN_POINT('Ctrl Pts',(-13.6708737217057,16.1685436044088,-0.432460477152238));
#21796=CARTESIAN_POINT('Ctrl Pts',(-13.7700581636469,16.3943923190575,-0.441627804171639));
#21797=CARTESIAN_POINT('Ctrl Pts',(-14.0539091255659,16.8066128735469,-0.46112045496409));
#21798=CARTESIAN_POINT('Ctrl Pts',(-14.2395717537967,16.9865111568954,-0.471935218600938));
#21799=CARTESIAN_POINT('Ctrl Pts',(-14.6649766982385,17.260117111467,-0.493726018953733));
#21800=CARTESIAN_POINT('Ctrl Pts',(-14.8993253045762,17.3532344934425,-0.50448785312903));
#21801=CARTESIAN_POINT('Ctrl Pts',(-15.3879151897707,17.4445879148856,-0.524708376132417));
#21802=CARTESIAN_POINT('Ctrl Pts',(-15.6373703514434,17.4429655287442,-0.533521108433316));
#21803=CARTESIAN_POINT('Ctrl Pts',(-16.1314699144086,17.3439130073667,-0.554113473589034));
#21804=CARTESIAN_POINT('Ctrl Pts',(-16.3705992585577,17.2437932713042,-0.565204895717519));
#21805=CARTESIAN_POINT('Ctrl Pts',(-16.7876645305446,16.9614315561499,-0.586873008236942));
#21806=CARTESIAN_POINT('Ctrl Pts',(-16.9637580966902,16.7850271274736,-0.597254988511056));
#21807=CARTESIAN_POINT('Ctrl Pts',(-17.2443400454302,16.3689556312255,-0.616708580128513));
#21808=CARTESIAN_POINT('Ctrl Pts',(-17.3436265737928,16.1315609718477,-0.626384649668764));
#21809=CARTESIAN_POINT('Ctrl Pts',(-17.4440644805083,15.6332086945697,-0.647879471588744));
#21810=CARTESIAN_POINT('Ctrl Pts',(-17.4447534368414,15.3772600500546,-0.658918992797644));
#21811=CARTESIAN_POINT('Ctrl Pts',(-17.3489811389163,14.8884838636653,-0.680000780850369));
#21812=CARTESIAN_POINT('Ctrl Pts',(-17.2568181639608,14.6596166093872,-0.689459136144938));
#21813=CARTESIAN_POINT('Ctrl Pts',(-16.9858620067821,14.238805099094,-0.708655396087524));
#21814=CARTESIAN_POINT('Ctrl Pts',(-16.8058878841893,14.0532686231487,-0.719379268374338));
#21815=CARTESIAN_POINT('Ctrl Pts',(-16.3885881553997,13.7662002686923,-0.741157641480895));
#21816=CARTESIAN_POINT('Ctrl Pts',(-16.1564785085564,13.665689225055,-0.751995294214013));
#21817=CARTESIAN_POINT('Ctrl Pts',(-15.7761115117429,13.5827427725166,-0.767992040173275));
#21818=CARTESIAN_POINT('Ctrl Pts',(-15.6381065100508,13.5679367061317,-0.773466277262654));
#21819=CARTESIAN_POINT('Ctrl Pts',(-15.5,13.5679367061317,-0.778625000000138));
#21820=CARTESIAN_POINT('Origin',(-15.5,15.5,11.20575));
#21821=CARTESIAN_POINT('',(-15.4999999999999,13.5679367061317,-1.27862500000015));
#21822=CARTESIAN_POINT('',(-15.5,13.5679367061317,-0.809875000000185));
#21823=CARTESIAN_POINT('',(-15.5,13.5679367061317,11.20575));
#21824=CARTESIAN_POINT('Ctrl Pts',(-15.5000000000001,13.5679367061317,-0.809875000000184));
#21825=CARTESIAN_POINT('Ctrl Pts',(-15.5387848588903,13.5679367061317,-0.808426260665929));
#21826=CARTESIAN_POINT('Ctrl Pts',(-15.5776081217821,13.569104553761,-0.806950901143725));
#21827=CARTESIAN_POINT('Ctrl Pts',(-15.8627498107999,13.5863172258654,-0.79592873452912));
#21828=CARTESIAN_POINT('Ctrl Pts',(-16.1039441624047,13.6482441649587,-0.785583839426258));
#21829=CARTESIAN_POINT('Ctrl Pts',(-16.5586938389718,13.8636040208236,-0.763953047887055));
#21830=CARTESIAN_POINT('Ctrl Pts',(-16.7663048606795,14.0184106751406,-0.752859564438582));
#21831=CARTESIAN_POINT('Ctrl Pts',(-17.1030886658293,14.3935142993235,-0.73219016123049));
#21832=CARTESIAN_POINT('Ctrl Pts',(-17.2315636886463,14.6078734364709,-0.723354008700342));
#21833=CARTESIAN_POINT('Ctrl Pts',(-17.4012591024431,15.0752831240919,-0.703193795820486));
#21834=CARTESIAN_POINT('Ctrl Pts',(-17.4401670421017,15.3241884796659,-0.692458064216697));
#21835=CARTESIAN_POINT('Ctrl Pts',(-17.4209116308134,15.8293918059367,-0.670667744343198));
#21836=CARTESIAN_POINT('Ctrl Pts',(-17.3604173282467,16.0807480284641,-0.659826302479591));
#21837=CARTESIAN_POINT('Ctrl Pts',(-17.1497816929781,16.5348352725858,-0.640240710332106));
#21838=CARTESIAN_POINT('Ctrl Pts',(-17.0057085011959,16.7351193667879,-0.631148276498292));
#21839=CARTESIAN_POINT('Ctrl Pts',(-16.6447314320371,17.0767669839641,-0.610296685602456));
#21840=CARTESIAN_POINT('Ctrl Pts',(-16.4291281586241,17.2126942752496,-0.599311816112351));
#21841=CARTESIAN_POINT('Ctrl Pts',(-15.9522914740593,17.396071415368,-0.577545739488896));
#21842=CARTESIAN_POINT('Ctrl Pts',(-15.6949512567242,17.4394863853226,-0.567317142600485));
#21843=CARTESIAN_POINT('Ctrl Pts',(-15.1907605692904,17.4229690903242,-0.548127787168027));
#21844=CARTESIAN_POINT('Ctrl Pts',(-14.9485965706545,17.3679857370151,-0.537896417242229));
#21845=CARTESIAN_POINT('Ctrl Pts',(-14.4891878782661,17.166282104194,-0.516386105083495));
#21846=CARTESIAN_POINT('Ctrl Pts',(-14.2777915836231,17.0180420352629,-0.505292843771063));
#21847=CARTESIAN_POINT('Ctrl Pts',(-13.9295152530061,16.6526099917286,-0.484402733995876));
#21848=CARTESIAN_POINT('Ctrl Pts',(-13.7941507738708,16.4407479085025,-0.475451133965662));
#21849=CARTESIAN_POINT('Ctrl Pts',(-13.611383887522,15.9774528011728,-0.455468390267086));
#21850=CARTESIAN_POINT('Ctrl Pts',(-13.5656468617909,15.7304237057034,-0.444813585105621));
#21851=CARTESIAN_POINT('Ctrl Pts',(-13.5704710073905,15.2255315160606,-0.423036685109424));
#21852=CARTESIAN_POINT('Ctrl Pts',(-13.623779229161,14.9725259783178,-0.412124105341039));
#21853=CARTESIAN_POINT('Ctrl Pts',(-13.8215336428728,14.5122846645607,-0.392273077201934));
#21854=CARTESIAN_POINT('Ctrl Pts',(-13.9600852553974,14.3077326406346,-0.383350131532038));
#21855=CARTESIAN_POINT('Ctrl Pts',(-14.311092329695,13.9563854884097,-0.362661772922335));
#21856=CARTESIAN_POINT('Ctrl Pts',(-14.5221235135244,13.814770334655,-0.351725021873647));
#21857=CARTESIAN_POINT('Ctrl Pts',(-14.9904064163151,13.6188695990394,-0.330008374038312));
#21858=CARTESIAN_POINT('Ctrl Pts',(-15.2437584839143,13.5679791180275,-0.319447360158956));
#21859=CARTESIAN_POINT('Ctrl Pts',(-15.4997866765027,13.5679367149642,-0.309882968509973));
#21860=CARTESIAN_POINT('Ctrl Pts',(-15.4998933384699,13.5679367061317,-0.309878984151688));
#21861=CARTESIAN_POINT('Ctrl Pts',(-15.5000000000426,13.5679367061317,-0.30987499999859));
#21862=CARTESIAN_POINT('Ctrl Pts',(-15.5,13.5679367061317,-0.778625000000138));
#21863=CARTESIAN_POINT('Ctrl Pts',(-15.3931460600035,13.5679367061317,-0.782616338639041));
#21864=CARTESIAN_POINT('Ctrl Pts',(-15.2862458066186,13.5768002208548,-0.786800556825666));
#21865=CARTESIAN_POINT('Ctrl Pts',(-14.9264097349309,13.6371564581267,-0.801543228515925));
#21866=CARTESIAN_POINT('Ctrl Pts',(-14.6835020776055,13.7301105172148,-0.812621248594988));
#21867=CARTESIAN_POINT('Ctrl Pts',(-14.2567488546817,14.0004851883713,-0.834392725983059));
#21868=CARTESIAN_POINT('Ctrl Pts',(-14.0749328111488,14.1720617647974,-0.844884342273106));
#21869=CARTESIAN_POINT('Ctrl Pts',(-13.7832732837112,14.5783544242248,-0.864540827785101));
#21870=CARTESIAN_POINT('Ctrl Pts',(-13.6776776440773,14.8102645186437,-0.873875479390643));
#21871=CARTESIAN_POINT('Ctrl Pts',(-13.5612057991943,15.3034623332341,-0.895147980148236));
#21872=CARTESIAN_POINT('Ctrl Pts',(-13.552197396611,15.5600993604861,-0.906217192531462));
#21873=CARTESIAN_POINT('Ctrl Pts',(-13.6325934592672,16.0528776431264,-0.927471598128334));
#21874=CARTESIAN_POINT('Ctrl Pts',(-13.7176559736562,16.2849105083636,-0.937309340873369));
#21875=CARTESIAN_POINT('Ctrl Pts',(-13.9755352339037,16.7142424065984,-0.956200886377741));
#21876=CARTESIAN_POINT('Ctrl Pts',(-14.1496041202698,16.9052695292978,-0.966822589771756));
#21877=CARTESIAN_POINT('Ctrl Pts',(-14.5583089435885,17.2056519897364,-0.988567046050803));
#21878=CARTESIAN_POINT('Ctrl Pts',(-14.7879324229243,17.3135593941174,-0.999471341534755));
#21879=CARTESIAN_POINT('Ctrl Pts',(-15.2696786466829,17.4338950578203,-1.02006125963416));
#21880=CARTESIAN_POINT('Ctrl Pts',(-15.5166980413127,17.4474891140478,-1.02891605403808));
#21881=CARTESIAN_POINT('Ctrl Pts',(-16.0156874195765,17.3798092848061,-1.04901448947301));
#21882=CARTESIAN_POINT('Ctrl Pts',(-16.2621352115938,17.2940873362134,-1.06006877807144));
#21883=CARTESIAN_POINT('Ctrl Pts',(-16.698154944133,17.0359029315518,-1.08192349546387));
#21884=CARTESIAN_POINT('Ctrl Pts',(-16.8855107789499,16.8692878721634,-1.09251504125555));
#21885=CARTESIAN_POINT('Ctrl Pts',(-17.1880123646469,16.472705598965,-1.11236709941354));
#21886=CARTESIAN_POINT('Ctrl Pts',(-17.2997096590055,16.2460520791468,-1.12144644415624));
#21887=CARTESIAN_POINT('Ctrl Pts',(-17.431671791372,15.7580841556283,-1.1424933703908));
#21888=CARTESIAN_POINT('Ctrl Pts',(-17.4488346169962,15.5010293356259,-1.15358060291997));
#21889=CARTESIAN_POINT('Ctrl Pts',(-17.383549418459,15.0046042925852,-1.17499229979244));
#21890=CARTESIAN_POINT('Ctrl Pts',(-17.3053971666591,14.7694246899964,-1.18513601520691));
#21891=CARTESIAN_POINT('Ctrl Pts',(-17.0601513563756,14.3319804120671,-1.20400376656016));
#21892=CARTESIAN_POINT('Ctrl Pts',(-16.8918928500653,14.1358043641068,-1.21438674923054));
#21893=CARTESIAN_POINT('Ctrl Pts',(-16.491712694381,13.8228284522729,-1.23608437073301));
#21894=CARTESIAN_POINT('Ctrl Pts',(-16.264686804895,13.7078902729296,-1.24704326280146));
#21895=CARTESIAN_POINT('Ctrl Pts',(-15.8517814524953,13.5920235017939,-1.26496537709516));
#21896=CARTESIAN_POINT('Ctrl Pts',(-15.676151507024,13.5679367061317,-1.27204517415274));
#21897=CARTESIAN_POINT('Ctrl Pts',(-15.4999999999999,13.5679367061317,-1.27862500000015));
#21898=CARTESIAN_POINT('Origin',(-15.5,15.5,11.20575));
#21899=CARTESIAN_POINT('',(-15.5,13.5679367061317,-1.77862500000015));
#21900=CARTESIAN_POINT('',(-15.5000000000001,13.5679367061317,-1.30987500000019));
#21901=CARTESIAN_POINT('',(-15.5,13.5679367061317,11.20575));
#21902=CARTESIAN_POINT('',(-16.6356236642092,13.9369173237082,-2.22824839960634));
#21903=CARTESIAN_POINT('Ctrl Pts',(-15.5,13.5679367061317,-1.77862500000015));
#21904=CARTESIAN_POINT('Ctrl Pts',(-15.4713110103049,13.5679367061317,-1.77969662611974));
#21905=CARTESIAN_POINT('Ctrl Pts',(-15.4425999921594,13.5685756992767,-1.78078285552937));
#21906=CARTESIAN_POINT('Ctrl Pts',(-15.1581590399474,13.5812658327421,-1.79168131479254));
#21907=CARTESIAN_POINT('Ctrl Pts',(-14.9072543398391,13.6433835357265,-1.80239303666449));
#21908=CARTESIAN_POINT('Ctrl Pts',(-14.4490712181685,13.8594981524984,-1.82416835552268));
#21909=CARTESIAN_POINT('Ctrl Pts',(-14.2453192502126,14.0095359244182,-1.83501484569199));
#21910=CARTESIAN_POINT('Ctrl Pts',(-13.9097095424868,14.3755767710421,-1.85544494570745));
#21911=CARTESIAN_POINT('Ctrl Pts',(-13.779653496445,14.5868970845778,-1.86424124385709));
#21912=CARTESIAN_POINT('Ctrl Pts',(-13.601624809573,15.0579406863098,-1.88455819392919));
#21913=CARTESIAN_POINT('Ctrl Pts',(-13.5596639923122,15.314726118177,-1.89563380726797));
#21914=CARTESIAN_POINT('Ctrl Pts',(-13.5785378997819,15.8197591251871,-1.9174167809682));
#21915=CARTESIAN_POINT('Ctrl Pts',(-13.635337470358,16.063306547793,-1.92792141537377));
#21916=CARTESIAN_POINT('Ctrl Pts',(-13.8396294894159,16.5196132324098,-1.94760273594545));
#21917=CARTESIAN_POINT('Ctrl Pts',(-13.98670541897,16.7273518608751,-1.95690084581238));
#21918=CARTESIAN_POINT('Ctrl Pts',(-14.3540458828622,17.0761951408069,-1.97814531086595));
#21919=CARTESIAN_POINT('Ctrl Pts',(-14.5713394118551,17.213239044857,-1.9892173975925));
#21920=CARTESIAN_POINT('Ctrl Pts',(-15.0377637904636,17.3918917772351,-2.01049265500658));
#21921=CARTESIAN_POINT('Ctrl Pts',(-15.2811490461273,17.4351931175239,-2.02038271492023));
#21922=CARTESIAN_POINT('Ctrl Pts',(-15.7819930616688,17.4284331863443,-2.03923663513813));
#21923=CARTESIAN_POINT('Ctrl Pts',(-16.0346645547899,17.3741617366328,-2.04984514097278));
#21924=CARTESIAN_POINT('Ctrl Pts',(-16.500008982865,17.1721421784805,-2.0715839851788));
#21925=CARTESIAN_POINT('Ctrl Pts',(-16.7088902825659,17.0279622254971,-2.08249574331544));
#21926=CARTESIAN_POINT('Ctrl Pts',(-17.055293507135,16.6721862680338,-2.10310764444889));
#21927=CARTESIAN_POINT('Ctrl Pts',(-17.191302469575,16.4656337932766,-2.11197549347074));
#21928=CARTESIAN_POINT('Ctrl Pts',(-17.383958897045,16.0003669873985,-2.13204328004182));
#21929=CARTESIAN_POINT('Ctrl Pts',(-17.4339176130592,15.7441588929761,-2.14309399178763));
#21930=CARTESIAN_POINT('Ctrl Pts',(-17.4301770605656,15.2372592429962,-2.16495747712602));
#21931=CARTESIAN_POINT('Ctrl Pts',(-17.3804225882662,14.9914303047801,-2.17556051736614));
#21932=CARTESIAN_POINT('Ctrl Pts',(-17.2188593063871,14.6006806202927,-2.19241424768163));
#21933=CARTESIAN_POINT('Ctrl Pts',(-17.1307744677382,14.4493679380718,-2.19870147391129));
#21934=CARTESIAN_POINT('Ctrl Pts',(-16.9124347549226,14.1693732822038,-2.21289549932321));
#21935=CARTESIAN_POINT('Ctrl Pts',(-16.78183780444,14.0431460180095,-2.22049591927456));
#21936=CARTESIAN_POINT('Ctrl Pts',(-16.6356236661869,13.9369173213456,-2.22824840453312));
#21937=CARTESIAN_POINT('',(-16.6356257705294,13.936918850212,-1.75949829183042));
#21938=CARTESIAN_POINT('',(-16.6356252385745,13.9369184637308,-1.75949832116282));
#21939=CARTESIAN_POINT('Ctrl Pts',(-16.6356257705685,13.9369188502404,-1.75949829295571));
#21940=CARTESIAN_POINT('Ctrl Pts',(-16.8232265616208,14.073216503712,-1.74955141913567));
#21941=CARTESIAN_POINT('Ctrl Pts',(-16.9847823163708,14.2421926306507,-1.73987267086338));
#21942=CARTESIAN_POINT('Ctrl Pts',(-17.2378815903649,14.625688547538,-1.72214816701709));
#21943=CARTESIAN_POINT('Ctrl Pts',(-17.3287014043758,14.8362794639401,-1.71350244965325));
#21944=CARTESIAN_POINT('Ctrl Pts',(-17.4385845729922,15.3036899854237,-1.69334220080741));
#21945=CARTESIAN_POINT('Ctrl Pts',(-17.447619886958,15.5584934383095,-1.68235207375453));
#21946=CARTESIAN_POINT('Ctrl Pts',(-17.366264820819,16.0626255591014,-1.66060795688251));
#21947=CARTESIAN_POINT('Ctrl Pts',(-17.2745029457006,16.306592918934,-1.65043016901723));
#21948=CARTESIAN_POINT('Ctrl Pts',(-17.0069230177962,16.7339605492266,-1.63121863353647));
#21949=CARTESIAN_POINT('Ctrl Pts',(-16.8376064327547,16.9157196559878,-1.62097431691814));
#21950=CARTESIAN_POINT('Ctrl Pts',(-16.4321558772125,17.2115388605548,-1.59944982869592));
#21951=CARTESIAN_POINT('Ctrl Pts',(-16.1976492003962,17.3197729456469,-1.58835608490562));
#21952=CARTESIAN_POINT('Ctrl Pts',(-15.7067373188973,17.4370349875308,-1.56749008537743));
#21953=CARTESIAN_POINT('Ctrl Pts',(-15.4557223788825,17.44753196976,-1.558554684095));
#21954=CARTESIAN_POINT('Ctrl Pts',(-14.9634366275307,17.3726902789252,-1.53855219877784));
#21955=CARTESIAN_POINT('Ctrl Pts',(-14.726821985697,17.2880297167385,-1.52788809973695));
#21956=CARTESIAN_POINT('Ctrl Pts',(-14.2927306055592,17.0300046441306,-1.50610884865212));
#21957=CARTESIAN_POINT('Ctrl Pts',(-14.1008202908091,16.8567343671546,-1.49520365267535));
#21958=CARTESIAN_POINT('Ctrl Pts',(-13.8024087055843,16.4544579219329,-1.47538156930738));
#21959=CARTESIAN_POINT('Ctrl Pts',(-13.6952482164322,16.2319055093249,-1.46644338907453));
#21960=CARTESIAN_POINT('Ctrl Pts',(-13.5679372308721,15.7518323297933,-1.44573697721874));
#21961=CARTESIAN_POINT('Ctrl Pts',(-13.5515962723608,15.4981347275301,-1.43479454747414));
#21962=CARTESIAN_POINT('Ctrl Pts',(-13.6177050294595,14.9946779887315,-1.41307956103121));
#21963=CARTESIAN_POINT('Ctrl Pts',(-13.7011232772003,14.7500889892398,-1.4025630039161));
#21964=CARTESIAN_POINT('Ctrl Pts',(-13.9530518157522,14.3167686917902,-1.38380772364012));
#21965=CARTESIAN_POINT('Ctrl Pts',(-14.1156697545305,14.1300765218333,-1.37370723711988));
#21966=CARTESIAN_POINT('Ctrl Pts',(-14.5094994028657,13.8216873535972,-1.35234574472332));
#21967=CARTESIAN_POINT('Ctrl Pts',(-14.7392900935943,13.7058009544622,-1.34126312922332));
#21968=CARTESIAN_POINT('Ctrl Pts',(-15.1530393767014,13.5913602763721,-1.32334024636833));
#21969=CARTESIAN_POINT('Ctrl Pts',(-15.3262907155805,13.5679367061317,-1.31636360097141));
#21970=CARTESIAN_POINT('Ctrl Pts',(-15.5000000000001,13.5679367061317,-1.30987500000019));
#21971=CARTESIAN_POINT('Origin',(15.4999999999998,15.5000000000002,11.20575));
#21972=CARTESIAN_POINT('',(13.5679367061315,15.5000000000002,1.22137499999984));
#21973=CARTESIAN_POINT('',(13.5679367061315,15.5000000000002,1.38580000000003));
#21974=CARTESIAN_POINT('',(13.5679367061315,15.5000000000002,11.20575));
#21975=CARTESIAN_POINT('',(16.4140591443296,17.2021646372137,1.3857999999999));
#21976=CARTESIAN_POINT('Origin',(15.4999999999998,15.5000000000002,1.3858));
#21977=CARTESIAN_POINT('Ctrl Pts',(16.4140591443296,17.2021646372137,1.38579999999989));
#21978=CARTESIAN_POINT('Ctrl Pts',(16.2625891375117,17.2835037402574,1.37926682864456));
#21979=CARTESIAN_POINT('Ctrl Pts',(16.1009499217413,17.3442553078036,1.37229504118279));
#21980=CARTESIAN_POINT('Ctrl Pts',(15.7606791264406,17.422586671179,1.35761855532521));
#21981=CARTESIAN_POINT('Ctrl Pts',(15.5832774891468,17.4383898562024,1.34996690653027));
#21982=CARTESIAN_POINT('Ctrl Pts',(15.1505459519398,17.4173618065492,1.33130242408378));
#21983=CARTESIAN_POINT('Ctrl Pts',(14.8998465930936,17.354246908948,1.32048931392145));
#21984=CARTESIAN_POINT('Ctrl Pts',(14.4480453997679,17.1389102319479,1.30100232321918));
#21985=CARTESIAN_POINT('Ctrl Pts',(14.2493134355933,16.9927945768321,1.29183017936196));
#21986=CARTESIAN_POINT('Ctrl Pts',(13.9112799546867,16.6281426360987,1.27091926225214));
#21987=CARTESIAN_POINT('Ctrl Pts',(13.7774947328739,16.4108843723267,1.25991876918149));
#21988=CARTESIAN_POINT('Ctrl Pts',(13.608962253039,15.9581594814273,1.23937348399882));
#21989=CARTESIAN_POINT('Ctrl Pts',(13.5679367061315,15.7298816359029,1.22996181912679));
#21990=CARTESIAN_POINT('Ctrl Pts',(13.5679367061316,15.5000000000002,1.22137499999984));
#21991=CARTESIAN_POINT('Origin',(15.4999999999998,15.5000000000002,11.20575));
#21992=CARTESIAN_POINT('',(13.5679367061316,15.5000000000002,0.721374999999831));
#21993=CARTESIAN_POINT('',(13.5679367061315,15.5000000000002,1.19012499999989));
#21994=CARTESIAN_POINT('',(13.5679367061315,15.5000000000002,11.20575));
#21995=CARTESIAN_POINT('',(17.0070594673501,16.7089831815966,1.3858));
#21996=CARTESIAN_POINT('Ctrl Pts',(13.5679367061316,15.5000000000002,1.19012499999989));
#21997=CARTESIAN_POINT('Ctrl Pts',(13.5679367061316,15.6209597157626,1.19464323477242));
#21998=CARTESIAN_POINT('Ctrl Pts',(13.5792946957062,15.7419184750208,1.19940637898304));
#21999=CARTESIAN_POINT('Ctrl Pts',(13.650067406739,16.1137167329625,1.21482051737726));
#22000=CARTESIAN_POINT('Ctrl Pts',(13.7479960405405,16.354030851272,1.22590894156177));
#22001=CARTESIAN_POINT('Ctrl Pts',(14.026702340502,16.7741136008835,1.2476109342981));
#22002=CARTESIAN_POINT('Ctrl Pts',(14.2016401214973,16.951982381632,1.2580275949881));
#22003=CARTESIAN_POINT('Ctrl Pts',(14.6147032779426,17.2359894885843,1.27754424976224));
#22004=CARTESIAN_POINT('Ctrl Pts',(14.8503902891229,17.3372359040127,1.2871061753863));
#22005=CARTESIAN_POINT('Ctrl Pts',(15.3471703745486,17.4426537117393,1.30853318586962));
#22006=CARTESIAN_POINT('Ctrl Pts',(15.6033601229598,17.4459126157985,1.31958310631927));
#22007=CARTESIAN_POINT('Ctrl Pts',(16.0780177664312,17.3577448351807,1.3400559364528));
#22008=CARTESIAN_POINT('Ctrl Pts',(16.2939199281618,17.2762233318698,1.34923226468184));
#22009=CARTESIAN_POINT('Ctrl Pts',(16.6881134566226,17.0408566361,1.36652510317408));
#22010=CARTESIAN_POINT('Ctrl Pts',(16.863050795795,16.8884973676924,1.37598889193061));
#22011=CARTESIAN_POINT('Ctrl Pts',(17.0070594673508,16.7089831815957,1.38580000000003));
#22012=CARTESIAN_POINT('Origin',(15.4999999999998,15.5000000000002,1.3858));
#22013=CARTESIAN_POINT('Ctrl Pts',(13.5679367061315,15.5000000000002,1.22137499999984));
#22014=CARTESIAN_POINT('Ctrl Pts',(13.5679367061315,15.472934163652,1.22036400388295));
#22015=CARTESIAN_POINT('Ctrl Pts',(13.5685054395939,15.445846997633,1.21933994579038));
#22016=CARTESIAN_POINT('Ctrl Pts',(13.5800041738241,15.1726369385485,1.2088866901258));
#22017=CARTESIAN_POINT('Ctrl Pts',(13.6373364196653,14.9307787642574,1.19861608776315));
#22018=CARTESIAN_POINT('Ctrl Pts',(13.8436681824179,14.4729009298073,1.17706314833023));
#22019=CARTESIAN_POINT('Ctrl Pts',(13.9941383692371,14.2627623230356,1.16596877122891));
#22020=CARTESIAN_POINT('Ctrl Pts',(14.3628583037133,13.9183617244766,1.14515252622457));
#22021=CARTESIAN_POINT('Ctrl Pts',(14.5755603825233,13.785334043101,1.1362477283077));
#22022=CARTESIAN_POINT('Ctrl Pts',(15.0402511771328,13.6069662799688,1.11620478612924));
#22023=CARTESIAN_POINT('Ctrl Pts',(15.2879321567374,13.5635189852419,1.10552186404319));
#22024=CARTESIAN_POINT('Ctrl Pts',(15.7929752641122,13.573195404212,1.08373845469624));
#22025=CARTESIAN_POINT('Ctrl Pts',(16.0454493144931,13.6289269314022,1.07284879892505));
#22026=CARTESIAN_POINT('Ctrl Pts',(16.5036338507401,13.8310245098165,1.05308648326572));
#22027=CARTESIAN_POINT('Ctrl Pts',(16.7067442549318,13.9714260898445,1.04411430770358));
#22028=CARTESIAN_POINT('Ctrl Pts',(17.0548537164756,14.3257784405245,1.02337081593677));
#22029=CARTESIAN_POINT('Ctrl Pts',(17.1945806684026,14.5383567468982,1.01241699563566));
#22030=CARTESIAN_POINT('Ctrl Pts',(17.3860429606825,15.008844336194,0.990713714647896));
#22031=CARTESIAN_POINT('Ctrl Pts',(17.4344332047204,15.2627143705022,0.980289491361847));
#22032=CARTESIAN_POINT('Ctrl Pts',(17.4296140644269,15.764107690739,0.961456907730253));
#22033=CARTESIAN_POINT('Ctrl Pts',(17.3804673298212,16.0069337841767,0.951326678315792));
#22034=CARTESIAN_POINT('Ctrl Pts',(17.1903012303483,16.4699471301539,0.929930537929737));
#22035=CARTESIAN_POINT('Ctrl Pts',(17.0476412722629,16.6843681045384,0.918844635155068));
#22036=CARTESIAN_POINT('Ctrl Pts',(16.6904570709538,17.0422253708337,0.897774518657255));
#22037=CARTESIAN_POINT('Ctrl Pts',(16.4806668479972,17.1834288054785,0.888672908972444));
#22038=CARTESIAN_POINT('Ctrl Pts',(16.0208578482245,17.3770350149772,0.868840527305979));
#22039=CARTESIAN_POINT('Ctrl Pts',(15.7755220881537,17.4283735116388,0.858258758718241));
#22040=CARTESIAN_POINT('Ctrl Pts',(15.2690019282793,17.4355092606072,0.836411641464455));
#22041=CARTESIAN_POINT('Ctrl Pts',(15.0126438264158,17.387341223535,0.825354459630359));
#22042=CARTESIAN_POINT('Ctrl Pts',(14.5460700125418,17.1979533838604,0.805230299474962));
#22043=CARTESIAN_POINT('Ctrl Pts',(14.3384565931961,17.0632817899814,0.796385555315291));
#22044=CARTESIAN_POINT('Ctrl Pts',(13.9803614872282,16.7193021672918,0.775814169009818));
#22045=CARTESIAN_POINT('Ctrl Pts',(13.8348471765416,16.5115619837911,0.764916258623728));
#22046=CARTESIAN_POINT('Ctrl Pts',(13.6296318245187,16.047792771362,0.743167333650249));
#22047=CARTESIAN_POINT('Ctrl Pts',(13.5735885358767,15.7954972629457,0.732534660769201));
#22048=CARTESIAN_POINT('Ctrl Pts',(13.5680718804954,15.5263956111567,0.722363876203961));
#22049=CARTESIAN_POINT('Ctrl Pts',(13.5679367061315,15.5131950984485,0.721867879404021));
#22050=CARTESIAN_POINT('Ctrl Pts',(13.5679367061315,15.5000000000002,0.72137499999983));
#22051=CARTESIAN_POINT('Origin',(15.4999999999998,15.5000000000002,11.20575));
#22052=CARTESIAN_POINT('',(13.5679367061315,15.5000000000002,0.221374999999826));
#22053=CARTESIAN_POINT('',(13.5679367061316,15.5000000000002,0.690124999999888));
#22054=CARTESIAN_POINT('',(13.5679367061315,15.5000000000002,11.20575));
#22055=CARTESIAN_POINT('Ctrl Pts',(13.5679367061316,15.5000000000001,0.690124999999887));
#22056=CARTESIAN_POINT('Ctrl Pts',(13.5679367061315,15.6631976348036,0.696220957019254));
#22057=CARTESIAN_POINT('Ctrl Pts',(13.5886111528802,15.8260698424817,0.702750621155699));
#22058=CARTESIAN_POINT('Ctrl Pts',(13.6937750358448,16.2318407735967,0.720175424526415));
#22059=CARTESIAN_POINT('Ctrl Pts',(13.8061679673989,16.4638288993592,0.731264781557297));
#22060=CARTESIAN_POINT('Ctrl Pts',(14.1088337976828,16.8630470507198,0.752704123005099));
#22061=CARTESIAN_POINT('Ctrl Pts',(14.2932884830908,17.028761444197,0.762872018728113));
#22062=CARTESIAN_POINT('Ctrl Pts',(14.7231251438693,17.2874053587743,0.781803012187303));
#22063=CARTESIAN_POINT('Ctrl Pts',(14.9664736216112,17.374500370631,0.79211305640897));
#22064=CARTESIAN_POINT('Ctrl Pts',(15.4692792372015,17.4482099203795,0.81379995874744));
#22065=CARTESIAN_POINT('Ctrl Pts',(15.7235658751721,17.4355847239787,0.824767794651923));
#22066=CARTESIAN_POINT('Ctrl Pts',(16.2055976541626,17.3151733744219,0.845558684393129));
#22067=CARTESIAN_POINT('Ctrl Pts',(16.4295122772787,17.2113496874159,0.854579673980942));
#22068=CARTESIAN_POINT('Ctrl Pts',(16.8359718966532,16.919015473378,0.874264961849427));
#22069=CARTESIAN_POINT('Ctrl Pts',(17.0120418978357,16.7296891979224,0.885134014187555));
#22070=CARTESIAN_POINT('Ctrl Pts',(17.2766178136157,16.2991617620672,0.906921415251218));
#22071=CARTESIAN_POINT('Ctrl Pts',(17.3648212635818,16.0634585876003,0.917627873583951));
#22072=CARTESIAN_POINT('Ctrl Pts',(17.4465792698412,15.5727030691462,0.937722356281839));
#22073=CARTESIAN_POINT('Ctrl Pts',(17.4398199793544,15.3223565583365,0.946593274573915));
#22074=CARTESIAN_POINT('Ctrl Pts',(17.3302144103321,14.8300711076972,0.967345462671009));
#22075=CARTESIAN_POINT('Ctrl Pts',(17.2253688342258,14.5935881752457,0.978439949755262));
#22076=CARTESIAN_POINT('Ctrl Pts',(16.9351538432129,14.1832015334437,1.00002795682992));
#22077=CARTESIAN_POINT('Ctrl Pts',(16.7556158303756,14.0110153602739,1.01033156193274));
#22078=CARTESIAN_POINT('Ctrl Pts',(16.332996555328,13.7379425524703,1.02964587164789));
#22079=CARTESIAN_POINT('Ctrl Pts',(16.0918227958031,13.6429845085469,1.03959862802553));
#22080=CARTESIAN_POINT('Ctrl Pts',(15.5900949475536,13.5535333316271,1.06123904433773));
#22081=CARTESIAN_POINT('Ctrl Pts',(15.3347633934763,13.5584675814191,1.07225194933623));
#22082=CARTESIAN_POINT('Ctrl Pts',(14.8487842127029,13.6646353766641,1.09321309755172));
#22083=CARTESIAN_POINT('Ctrl Pts',(14.6220240391674,13.761672278609,1.10246053097519));
#22084=CARTESIAN_POINT('Ctrl Pts',(14.2071591450859,14.0415852702364,1.12186311344006));
#22085=CARTESIAN_POINT('Ctrl Pts',(14.0255156909756,14.2255255819059,1.13265117917161));
#22086=CARTESIAN_POINT('Ctrl Pts',(13.7477641930791,14.6484954207358,1.15444042282688));
#22087=CARTESIAN_POINT('Ctrl Pts',(13.6523788496879,14.8821830754014,1.16522647893853));
#22088=CARTESIAN_POINT('Ctrl Pts',(13.5800170676886,15.2505243179928,1.1805457564122));
#22089=CARTESIAN_POINT('Ctrl Pts',(13.5679367061316,15.375252816257,1.18546529110582));
#22090=CARTESIAN_POINT('Ctrl Pts',(13.5679367061316,15.5000000000002,1.19012499999989));
#22091=CARTESIAN_POINT('Ctrl Pts',(13.5679367061316,15.5000000000002,0.721374999999831));
#22092=CARTESIAN_POINT('Ctrl Pts',(13.5679367061316,15.2685828062759,0.71273082284504));
#22093=CARTESIAN_POINT('Ctrl Pts',(13.6095133453252,15.0388969706604,0.703254680214518));
#22094=CARTESIAN_POINT('Ctrl Pts',(13.7800568345428,14.5838672573797,0.682579933286903));
#22095=CARTESIAN_POINT('Ctrl Pts',(13.9154007889708,14.3657373187035,0.671513264894632));
#22096=CARTESIAN_POINT('Ctrl Pts',(14.2617096429524,13.9955563281774,0.650217354181319));
#22097=CARTESIAN_POINT('Ctrl Pts',(14.4688321613627,13.8467023151839,0.640851106705407));
#22098=CARTESIAN_POINT('Ctrl Pts',(14.9240794294144,13.6392165648129,0.62121548065835));
#22099=CARTESIAN_POINT('Ctrl Pts',(15.1670698899724,13.5807974419652,0.610734869018579));
#22100=CARTESIAN_POINT('Ctrl Pts',(15.6716078300757,13.5584324818414,0.588973248436394));
#22101=CARTESIAN_POINT('Ctrl Pts',(15.92849285909,13.5985422787833,0.577893339295162));
#22102=CARTESIAN_POINT('Ctrl Pts',(16.4008511612857,13.773173526314,0.557519683848905));
#22103=CARTESIAN_POINT('Ctrl Pts',(16.6132862459897,13.9018579854675,0.548728405599746));
#22104=CARTESIAN_POINT('Ctrl Pts',(16.9816699618116,14.2349802268651,0.52834069439712));
#22105=CARTESIAN_POINT('Ctrl Pts',(17.1330265346661,14.4375333640891,0.517510543297487));
#22106=CARTESIAN_POINT('Ctrl Pts',(17.3523384610754,14.8940137703006,0.495729873511439));
#22107=CARTESIAN_POINT('Ctrl Pts',(17.4162475186011,15.1444779569485,0.484995974078288));
#22108=CARTESIAN_POINT('Ctrl Pts',(17.4421185607647,15.6442929462081,0.465768343165624));
#22109=CARTESIAN_POINT('Ctrl Pts',(17.4083000036646,15.8886689108966,0.456344488460597));
#22110=CARTESIAN_POINT('Ctrl Pts',(17.2484328205998,16.3602738340633,0.435280848141696));
#22111=CARTESIAN_POINT('Ctrl Pts',(17.120645735791,16.5819407284765,0.424245033694158));
#22112=CARTESIAN_POINT('Ctrl Pts',(16.7856687237361,16.9645889727935,0.402727812187014));
#22113=CARTESIAN_POINT('Ctrl Pts',(16.5812682860446,17.1213576047524,0.393012028294842));
#22114=CARTESIAN_POINT('Ctrl Pts',(16.1307300452772,17.3428309784573,0.373579510987316));
#22115=CARTESIAN_POINT('Ctrl Pts',(15.8902976974581,17.4082697840059,0.363209235309224));
#22116=CARTESIAN_POINT('Ctrl Pts',(15.388198076337,17.4458200822582,0.341552783770483));
#22117=CARTESIAN_POINT('Ctrl Pts',(15.1310281685985,17.4137884812617,0.330460587302136));
#22118=CARTESIAN_POINT('Ctrl Pts',(14.6530287773331,17.254050494753,0.309843621630324));
#22119=CARTESIAN_POINT('Ctrl Pts',(14.4356759588901,17.1313390171616,0.301024334094614));
#22120=CARTESIAN_POINT('Ctrl Pts',(14.0571971875519,16.8090342642195,0.280822982040742));
#22121=CARTESIAN_POINT('Ctrl Pts',(13.9002426533357,16.6117620421852,0.270069365098247));
#22122=CARTESIAN_POINT('Ctrl Pts',(13.6672548470398,16.1629040885246,0.248278485916038));
#22123=CARTESIAN_POINT('Ctrl Pts',(13.5956339334193,15.9144966794261,0.237455100696454));
#22124=CARTESIAN_POINT('Ctrl Pts',(13.5701259723254,15.606262404414,0.22539145635692));
#22125=CARTESIAN_POINT('Ctrl Pts',(13.5679367061316,15.5531033072491,0.22335857947366));
#22126=CARTESIAN_POINT('Ctrl Pts',(13.5679367061315,15.5000000000003,0.221374999999826));
#22127=CARTESIAN_POINT('Origin',(15.4999999999998,15.5000000000002,11.20575));
#22128=CARTESIAN_POINT('',(13.5679367061315,15.5000000000002,-0.278625000000181));
#22129=CARTESIAN_POINT('',(13.5679367061316,15.5000000000001,0.190124999999878));
#22130=CARTESIAN_POINT('',(13.5679367061315,15.5000000000002,11.20575));
#22131=CARTESIAN_POINT('Ctrl Pts',(13.5679367061316,15.5000000000001,0.190124999999878));
#22132=CARTESIAN_POINT('Ctrl Pts',(13.5679367061315,15.7052232055912,0.197790747375235));
#22133=CARTESIAN_POINT('Ctrl Pts',(13.6006312438211,15.909443124398,0.206124105599977));
#22134=CARTESIAN_POINT('Ctrl Pts',(13.7445092392225,16.3458500952327,0.225528168010872));
#22135=CARTESIAN_POINT('Ctrl Pts',(13.8706006648954,16.5687690249,0.236574181605313));
#22136=CARTESIAN_POINT('Ctrl Pts',(14.1957983248935,16.9462938014509,0.25768912465625));
#22137=CARTESIAN_POINT('Ctrl Pts',(14.3891741439702,17.0996068020763,0.267213101031667));
#22138=CARTESIAN_POINT('Ctrl Pts',(14.8328987043057,17.3312210666005,0.286351732158286));
#22139=CARTESIAN_POINT('Ctrl Pts',(15.0810963874242,17.4033891896782,0.29705694058781));
#22140=CARTESIAN_POINT('Ctrl Pts',(15.5859112111093,17.4463663432178,0.318830503652366));
#22141=CARTESIAN_POINT('Ctrl Pts',(15.8374917549291,17.41880982897,0.32968162089312));
#22142=CARTESIAN_POINT('Ctrl Pts',(16.311441609934,17.2705600347065,0.35012392284861));
#22143=CARTESIAN_POINT('Ctrl Pts',(16.5299161239961,17.1530549287718,0.358922469304605));
#22144=CARTESIAN_POINT('Ctrl Pts',(16.9202726297617,16.8349526369191,0.379222999835996));
#22145=CARTESIAN_POINT('Ctrl Pts',(17.0854512100821,16.6338441663763,0.39029727189277));
#22146=CARTESIAN_POINT('Ctrl Pts',(17.3225641667435,16.1874197433199,0.412086213416689));
#22147=CARTESIAN_POINT('Ctrl Pts',(17.3956324394972,15.9481982603312,0.422597688314598));
#22148=CARTESIAN_POINT('Ctrl Pts',(17.4478128352921,15.4510757841907,0.442292129850948));
#22149=CARTESIAN_POINT('Ctrl Pts',(17.4248413113891,15.197732591562,0.451571409240266));
#22150=CARTESIAN_POINT('Ctrl Pts',(17.2822086107977,14.711734855356,0.472800990486119));
#22151=CARTESIAN_POINT('Ctrl Pts',(17.1630032804554,14.4841033890506,0.48387452771214));
#22152=CARTESIAN_POINT('Ctrl Pts',(16.8491384993419,14.0954494858789,0.505160775836514));
#22153=CARTESIAN_POINT('Ctrl Pts',(16.6603046231694,13.9358452837368,0.51507899362005));
#22154=CARTESIAN_POINT('Ctrl Pts',(16.2236425461118,13.6903827463215,0.533913007255612));
#22155=CARTESIAN_POINT('Ctrl Pts',(15.977849940704,13.6105539996564,0.544514480396965));
#22156=CARTESIAN_POINT('Ctrl Pts',(15.4739117712155,13.551815844132,0.5662502318036));
#22157=CARTESIAN_POINT('Ctrl Pts',(15.2208352901073,13.5717427947095,0.577165871485784));
#22158=CARTESIAN_POINT('Ctrl Pts',(14.7426848689158,13.7057278794306,0.597789351347489));
#22159=CARTESIAN_POINT('Ctrl Pts',(14.5214408844316,13.8161488953135,0.606664573343399));
#22160=CARTESIAN_POINT('Ctrl Pts',(14.1213400688697,14.1219606735906,0.626716158351901));
#22161=CARTESIAN_POINT('Ctrl Pts',(13.9495491173572,14.3185686119022,0.637764922719205));
#22162=CARTESIAN_POINT('Ctrl Pts',(13.6984440207751,14.7590310485604,0.659632917824892));
#22163=CARTESIAN_POINT('Ctrl Pts',(13.6181551918388,14.996695945816,0.670241966963368));
#22164=CARTESIAN_POINT('Ctrl Pts',(13.5736457522817,15.3284077888483,0.683592357862537));
#22165=CARTESIAN_POINT('Ctrl Pts',(13.5679367061315,15.4142441778549,0.686921743980967));
#22166=CARTESIAN_POINT('Ctrl Pts',(13.5679367061315,15.5000000000001,0.690124999999889));
#22167=CARTESIAN_POINT('Ctrl Pts',(13.5679367061315,15.5000000000003,0.221374999999828));
#22168=CARTESIAN_POINT('Ctrl Pts',(13.5679367061315,15.3093450220739,0.214253422825221));
#22169=CARTESIAN_POINT('Ctrl Pts',(13.5961535790968,15.1194546082456,0.206551882570376));
#22170=CARTESIAN_POINT('Ctrl Pts',(13.7256105047228,14.6948718230659,0.187900494778529));
#22171=CARTESIAN_POINT('Ctrl Pts',(13.845972473953,14.4700098902214,0.176905464594504));
#22172=CARTESIAN_POINT('Ctrl Pts',(14.1696924218756,14.075352608936,0.155182435517201));
#22173=CARTESIAN_POINT('Ctrl Pts',(14.3714266001445,13.9107790536386,0.145052382164217));
#22174=CARTESIAN_POINT('Ctrl Pts',(14.8173319840546,13.6758632412697,0.125819688229996));
#22175=CARTESIAN_POINT('Ctrl Pts',(15.0551292054429,13.6037990123974,0.115563070251393));
#22176=CARTESIAN_POINT('Ctrl Pts',(15.5544792852584,13.5518334963225,0.0940252113296194));
#22177=CARTESIAN_POINT('Ctrl Pts',(15.8116932973583,13.5761558231843,0.082931112561566));
#22178=CARTESIAN_POINT('Ctrl Pts',(16.2949297859146,13.7215598037838,0.0620882615496575));
#22179=CARTESIAN_POINT('Ctrl Pts',(16.5170608746999,13.8385708541843,0.0531675695664913));
#22180=CARTESIAN_POINT('Ctrl Pts',(16.9049967005296,14.150596790255,0.0331462146042882));
#22181=CARTESIAN_POINT('Ctrl Pts',(17.0670614605326,14.3427581393122,0.0224732986472017));
#22182=CARTESIAN_POINT('Ctrl Pts',(17.3126898338364,14.7840616508994,0.000691997103376874));
#22183=CARTESIAN_POINT('Ctrl Pts',(17.3915129003429,15.030308881313,-0.0102060193334657));
#22184=CARTESIAN_POINT('Ctrl Pts',(17.4473055261712,15.5280187232032,-0.0300003018310558));
#22185=CARTESIAN_POINT('Ctrl Pts',(17.4281050083514,15.7742335760592,-0.0389538708224634));
#22186=CARTESIAN_POINT('Ctrl Pts',(17.2969077106339,16.2532901707722,-0.0596775634354227));
#22187=CARTESIAN_POINT('Ctrl Pts',(17.1834947937312,16.4808992968809,-0.0706253476255288));
#22188=CARTESIAN_POINT('Ctrl Pts',(16.8732369845877,16.882970778244,-0.0923349979238737));
#22189=CARTESIAN_POINT('Ctrl Pts',(16.6781753241914,17.0524923784484,-0.102808198434923));
#22190=CARTESIAN_POINT('Ctrl Pts',(16.2425026234143,17.3005030646061,-0.121599538508183));
#22191=CARTESIAN_POINT('Ctrl Pts',(16.0080032119515,17.3801675177468,-0.131713916067101));
#22192=CARTESIAN_POINT('Ctrl Pts',(15.512365648488,17.44877246744,-0.153091647541905));
#22193=CARTESIAN_POINT('Ctrl Pts',(15.2553808905635,17.43339955154,-0.164175858168785));
#22194=CARTESIAN_POINT('Ctrl Pts',(14.7662503098183,17.3048200986632,-0.185272931881702));
#22195=CARTESIAN_POINT('Ctrl Pts',(14.5384527981285,17.1944566842457,-0.194401543727441));
#22196=CARTESIAN_POINT('Ctrl Pts',(14.1397272752797,16.8943347847829,-0.214210934032653));
#22197=CARTESIAN_POINT('Ctrl Pts',(13.9720032633974,16.7081889664025,-0.224781197363946));
#22198=CARTESIAN_POINT('Ctrl Pts',(13.7111048248534,16.2741834169149,-0.246619209094661));
#22199=CARTESIAN_POINT('Ctrl Pts',(13.6237773096301,16.028498554785,-0.257679625280961));
#22200=CARTESIAN_POINT('Ctrl Pts',(13.5743830168652,15.6823226737332,-0.271675640774711));
#22201=CARTESIAN_POINT('Ctrl Pts',(13.5679367061315,15.5911253193284,-0.275221175976205));
#22202=CARTESIAN_POINT('Ctrl Pts',(13.5679367061315,15.5000000000002,-0.278625000000181));
#22203=CARTESIAN_POINT('Origin',(15.4999999999998,15.5000000000002,11.20575));
#22204=CARTESIAN_POINT('',(13.5679367061315,15.5000000000002,-0.778625000000188));
#22205=CARTESIAN_POINT('',(13.5679367061315,15.5000000000215,-0.309874999998533));
#22206=CARTESIAN_POINT('',(13.5679367061315,15.5000000000002,11.20575));
#22207=CARTESIAN_POINT('Ctrl Pts',(13.5679367061315,15.5000000000427,-0.309874999998534));
#22208=CARTESIAN_POINT('Ctrl Pts',(13.5679367061369,15.7451189900437,-0.300719016644392));
#22209=CARTESIAN_POINT('Ctrl Pts',(13.6145849104547,15.9880788836299,-0.290637672395828));
#22210=CARTESIAN_POINT('Ctrl Pts',(13.7998506160076,16.4525087353534,-0.269294302322016));
#22211=CARTESIAN_POINT('Ctrl Pts',(13.9401358945743,16.6681650113369,-0.258213469135985));
#22212=CARTESIAN_POINT('Ctrl Pts',(14.2937988135868,17.030051039115,-0.23706880501825));
#22213=CARTESIAN_POINT('Ctrl Pts',(14.5027181075031,17.1737375672255,-0.227889545454423));
#22214=CARTESIAN_POINT('Ctrl Pts',(14.9610456268795,17.3718881645075,-0.208121062677875));
#22215=CARTESIAN_POINT('Ctrl Pts',(15.2056351161719,17.4255568606797,-0.197571482078912));
#22216=CARTESIAN_POINT('Ctrl Pts',(15.7028273877143,17.4374855261911,-0.1761266932738));
#22217=CARTESIAN_POINT('Ctrl Pts',(15.9508283805329,17.3951930471992,-0.165429968447515));
#22218=CARTESIAN_POINT('Ctrl Pts',(16.4162168450068,17.2190375058601,-0.145356934524384));
#22219=CARTESIAN_POINT('Ctrl Pts',(16.6293413959125,17.087177913888,-0.136472617530292));
#22220=CARTESIAN_POINT('Ctrl Pts',(16.9997020048589,16.7447233478946,-0.115693680499858));
#22221=CARTESIAN_POINT('Ctrl Pts',(17.151285984167,16.5352235199722,-0.104599143917318));
#22222=CARTESIAN_POINT('Ctrl Pts',(17.3599329092895,16.0781299074099,-0.0830255691568057));
#22223=CARTESIAN_POINT('Ctrl Pts',(17.4184418092005,15.8364334516317,-0.0727356319076326));
#22224=CARTESIAN_POINT('Ctrl Pts',(17.4419572678442,15.3335771418076,-0.0534451981391343));
#22225=CARTESIAN_POINT('Ctrl Pts',(17.4026393126743,15.0770448720175,-0.0434417100342342));
#22226=CARTESIAN_POINT('Ctrl Pts',(17.2273302215967,14.5982616364446,-0.0217769181316676));
#22227=CARTESIAN_POINT('Ctrl Pts',(17.094621571808,14.3801849192583,-0.0107690704263424));
#22228=CARTESIAN_POINT('Ctrl Pts',(16.7583973031519,14.0137016048738,0.0101712371103755));
#22229=CARTESIAN_POINT('Ctrl Pts',(16.5604348396368,13.8665662971672,0.019386555379266));
#22230=CARTESIAN_POINT('Ctrl Pts',(16.1097762694868,13.6488960345413,0.0388242627075083));
#22231=CARTESIAN_POINT('Ctrl Pts',(15.859413903315,13.584481024699,0.0496228377751859));
#22232=CARTESIAN_POINT('Ctrl Pts',(15.354216020494,13.5572975229281,0.0714129228630083));
#22233=CARTESIAN_POINT('Ctrl Pts',(15.104360020515,13.592429171137,0.0821896574543013));
#22234=CARTESIAN_POINT('Ctrl Pts',(14.634735382139,13.7549549306403,0.102445405107882));
#22235=CARTESIAN_POINT('Ctrl Pts',(14.4190031858108,13.8797188217571,0.11124827499474));
#22236=CARTESIAN_POINT('Ctrl Pts',(14.0387180251792,14.2102312356744,0.131795166002679));
#22237=CARTESIAN_POINT('Ctrl Pts',(13.8803875205855,14.4157066951992,0.142884874300359));
#22238=CARTESIAN_POINT('Ctrl Pts',(13.6576628179055,14.8677637645245,0.164573917775808));
#22239=CARTESIAN_POINT('Ctrl Pts',(13.5919750720433,15.1083498919251,0.174977198896046));
#22240=CARTESIAN_POINT('Ctrl Pts',(13.5697540327489,15.4031822744544,0.186469354010808));
#22241=CARTESIAN_POINT('Ctrl Pts',(13.5679367061315,15.4516175612208,0.188317760160613));
#22242=CARTESIAN_POINT('Ctrl Pts',(13.5679367061315,15.5000000000001,0.190124999999879));
#22243=CARTESIAN_POINT('Ctrl Pts',(13.5679367061315,15.5000000000002,-0.278625000000181));
#22244=CARTESIAN_POINT('Ctrl Pts',(13.5679367061315,15.3467892596533,-0.284347914362165));
#22245=CARTESIAN_POINT('Ctrl Pts',(13.5861582264408,15.193811827971,-0.290455077217825));
#22246=CARTESIAN_POINT('Ctrl Pts',(13.681690372198,14.8002115588649,-0.307217550187096));
#22247=CARTESIAN_POINT('Ctrl Pts',(13.7879612605511,14.5700164470718,-0.318107905057002));
#22248=CARTESIAN_POINT('Ctrl Pts',(14.085411271142,14.1593674322763,-0.339861742252181));
#22249=CARTESIAN_POINT('Ctrl Pts',(14.2752366147309,13.9839732655354,-0.350507031697016));
#22250=CARTESIAN_POINT('Ctrl Pts',(14.7026885544222,13.7231840672578,-0.369466729773054));
#22251=CARTESIAN_POINT('Ctrl Pts',(14.9340075268005,13.6365422675152,-0.379212735876613));
#22252=CARTESIAN_POINT('Ctrl Pts',(15.4259040926485,13.552703568537,-0.400429111456754));
#22253=CARTESIAN_POINT('Ctrl Pts',(15.6824101506341,13.5598498556532,-0.411492674866595));
#22254=CARTESIAN_POINT('Ctrl Pts',(16.1685436046143,13.670873721781,-0.432460477161097));
#22255=CARTESIAN_POINT('Ctrl Pts',(16.3943923192522,13.7700581637479,-0.441627804179568));
#22256=CARTESIAN_POINT('Ctrl Pts',(16.80661287371,14.0539091257136,-0.461120454973073));
#22257=CARTESIAN_POINT('Ctrl Pts',(16.9865111570376,14.2395717539648,-0.471935218610241));
#22258=CARTESIAN_POINT('Ctrl Pts',(17.2601171115597,14.6649766984353,-0.493726018963056));
#22259=CARTESIAN_POINT('Ctrl Pts',(17.3532344935082,14.8993253047808,-0.504487853138082));
#22260=CARTESIAN_POINT('Ctrl Pts',(17.4445879148985,15.3879151899874,-0.524708376140794));
#22261=CARTESIAN_POINT('Ctrl Pts',(17.442965528729,15.6373703516649,-0.533521108441911));
#22262=CARTESIAN_POINT('Ctrl Pts',(17.3439130072936,16.1314699146203,-0.55411347359851));
#22263=CARTESIAN_POINT('Ctrl Pts',(17.2437932712051,16.3705992587551,-0.565204895727018));
#22264=CARTESIAN_POINT('Ctrl Pts',(16.9614315560074,16.7876645307058,-0.586873008246029));
#22265=CARTESIAN_POINT('Ctrl Pts',(16.7850271273137,16.9637580968302,-0.597254988519727));
#22266=CARTESIAN_POINT('Ctrl Pts',(16.3689556310297,17.2443400455292,-0.616708580136453));
#22267=CARTESIAN_POINT('Ctrl Pts',(16.1315609716315,17.3436265738683,-0.626384649678148));
#22268=CARTESIAN_POINT('Ctrl Pts',(15.6332086943346,17.4440644805243,-0.647879471598956));
#22269=CARTESIAN_POINT('Ctrl Pts',(15.3772600498225,17.4447534368266,-0.658918992807723));
#22270=CARTESIAN_POINT('Ctrl Pts',(14.8884838634483,17.3489811388447,-0.680000780859792));
#22271=CARTESIAN_POINT('Ctrl Pts',(14.6596166091818,17.2568181638627,-0.6894591361531));
#22272=CARTESIAN_POINT('Ctrl Pts',(14.2388050989207,16.9858620066354,-0.7086553960968));
#22273=CARTESIAN_POINT('Ctrl Pts',(14.0532686229962,16.8058878840209,-0.719379268383982));
#22274=CARTESIAN_POINT('Ctrl Pts',(13.7662002685901,16.3885881552,-0.741157641490634));
#22275=CARTESIAN_POINT('Ctrl Pts',(13.6656892249804,16.1564785083478,-0.751995294223503));
#22276=CARTESIAN_POINT('Ctrl Pts',(13.5827427725009,15.7761115115987,-0.767992040179092));
#22277=CARTESIAN_POINT('Ctrl Pts',(13.5679367061315,15.6381065099785,-0.773466277265415));
#22278=CARTESIAN_POINT('Ctrl Pts',(13.5679367061315,15.5000000000002,-0.778625000000189));
#22279=CARTESIAN_POINT('Origin',(15.4999999999998,15.5000000000002,11.20575));
#22280=CARTESIAN_POINT('',(13.5679367061315,15.5000000000001,-1.2786250000002));
#22281=CARTESIAN_POINT('',(13.5679367061315,15.5000000000002,-0.809875000000126));
#22282=CARTESIAN_POINT('',(13.5679367061315,15.5000000000002,11.20575));
#22283=CARTESIAN_POINT('Ctrl Pts',(13.5679367061315,15.5000000000003,-0.809875000000126));
#22284=CARTESIAN_POINT('Ctrl Pts',(13.5679367061316,15.5387848588904,-0.808426260665874));
#22285=CARTESIAN_POINT('Ctrl Pts',(13.5691045537608,15.5776081217821,-0.806950901143693));
#22286=CARTESIAN_POINT('Ctrl Pts',(13.5863172258652,15.8627498107998,-0.795928734529088));
#22287=CARTESIAN_POINT('Ctrl Pts',(13.6482441649584,16.1039441624046,-0.785583839426238));
#22288=CARTESIAN_POINT('Ctrl Pts',(13.8636040208233,16.5586938389718,-0.763953047887043));
#22289=CARTESIAN_POINT('Ctrl Pts',(14.0184106751403,16.7663048606795,-0.752859564438586));
#22290=CARTESIAN_POINT('Ctrl Pts',(14.3935142993231,17.1030886658294,-0.732190161230492));
#22291=CARTESIAN_POINT('Ctrl Pts',(14.6078734364705,17.2315636886463,-0.723354008700334));
#22292=CARTESIAN_POINT('Ctrl Pts',(15.0752831240914,17.4012591024431,-0.703193795820476));
#22293=CARTESIAN_POINT('Ctrl Pts',(15.3241884796655,17.4401670421019,-0.692458064216684));
#22294=CARTESIAN_POINT('Ctrl Pts',(15.8293918059363,17.4209116308136,-0.67066774434319));
#22295=CARTESIAN_POINT('Ctrl Pts',(16.0807480284636,17.3604173282469,-0.659826302479593));
#22296=CARTESIAN_POINT('Ctrl Pts',(16.5348352725854,17.1497816929783,-0.640240710332137));
#22297=CARTESIAN_POINT('Ctrl Pts',(16.7351193667875,17.0057085011961,-0.631148276498336));
#22298=CARTESIAN_POINT('Ctrl Pts',(17.0767669839638,16.6447314320374,-0.61029668560251));
#22299=CARTESIAN_POINT('Ctrl Pts',(17.2126942752492,16.4291281586245,-0.599311816112398));
#22300=CARTESIAN_POINT('Ctrl Pts',(17.3960714153677,15.9522914740598,-0.577545739488941));
#22301=CARTESIAN_POINT('Ctrl Pts',(17.4394863853224,15.6949512567246,-0.567317142600507));
#22302=CARTESIAN_POINT('Ctrl Pts',(17.422969090324,15.1907605692907,-0.548127787168051));
#22303=CARTESIAN_POINT('Ctrl Pts',(17.3679857370148,14.9485965706548,-0.537896417242269));
#22304=CARTESIAN_POINT('Ctrl Pts',(17.1662821041939,14.4891878782663,-0.516386105083552));
#22305=CARTESIAN_POINT('Ctrl Pts',(17.0180420352627,14.2777915836234,-0.505292843771136));
#22306=CARTESIAN_POINT('Ctrl Pts',(16.6526099917284,13.9295152530064,-0.484402733995948));
#22307=CARTESIAN_POINT('Ctrl Pts',(16.4407479085024,13.7941507738711,-0.47545113396572));
#22308=CARTESIAN_POINT('Ctrl Pts',(15.9774528011727,13.6113838875223,-0.45546839026713));
#22309=CARTESIAN_POINT('Ctrl Pts',(15.7304237057033,13.5656468617912,-0.444813585105653));
#22310=CARTESIAN_POINT('Ctrl Pts',(15.2255315160606,13.5704710073907,-0.423036685109443));
#22311=CARTESIAN_POINT('Ctrl Pts',(14.9725259783177,13.6237792291612,-0.412124105341057));
#22312=CARTESIAN_POINT('Ctrl Pts',(14.5122846645605,13.821533642873,-0.392273077201959));
#22313=CARTESIAN_POINT('Ctrl Pts',(14.3077326406345,13.9600852553975,-0.383350131532067));
#22314=CARTESIAN_POINT('Ctrl Pts',(13.9563854884096,14.3110923296951,-0.362661772922356));
#22315=CARTESIAN_POINT('Ctrl Pts',(13.8147703346549,14.5221235135245,-0.351725021873652));
#22316=CARTESIAN_POINT('Ctrl Pts',(13.6188695990393,14.9904064163151,-0.330008374038293));
#22317=CARTESIAN_POINT('Ctrl Pts',(13.5679791180273,15.2437584839144,-0.31944736015892));
#22318=CARTESIAN_POINT('Ctrl Pts',(13.567936714964,15.4997866765028,-0.309882968509927));
#22319=CARTESIAN_POINT('Ctrl Pts',(13.5679367061315,15.4998933384701,-0.309878984151632));
#22320=CARTESIAN_POINT('Ctrl Pts',(13.5679367061315,15.5000000000427,-0.309874999998532));
#22321=CARTESIAN_POINT('Ctrl Pts',(13.5679367061316,15.5000000000002,-0.778625000000188));
#22322=CARTESIAN_POINT('Ctrl Pts',(13.5679367061316,15.3931460599276,-0.782616338641927));
#22323=CARTESIAN_POINT('Ctrl Pts',(13.5768002208671,15.2862458064669,-0.786800556831684));
#22324=CARTESIAN_POINT('Ctrl Pts',(13.6371564581937,14.9264097347141,-0.801543228525542));
#22325=CARTESIAN_POINT('Ctrl Pts',(13.7301105173089,14.6835020774024,-0.812621248604655));
#22326=CARTESIAN_POINT('Ctrl Pts',(14.0004851885106,14.2567488545141,-0.834392725992354));
#22327=CARTESIAN_POINT('Ctrl Pts',(14.172061764955,14.0749328110024,-0.844884342281997));
#22328=CARTESIAN_POINT('Ctrl Pts',(14.5783544244189,13.7832732836059,-0.864540827793249));
#22329=CARTESIAN_POINT('Ctrl Pts',(14.8102645188579,13.6776776439952,-0.873875479399929));
#22330=CARTESIAN_POINT('Ctrl Pts',(15.3034623334679,13.5612057991712,-0.895147980158364));
#22331=CARTESIAN_POINT('Ctrl Pts',(15.5600993607178,13.5521973966187,-0.906217192541493));
#22332=CARTESIAN_POINT('Ctrl Pts',(16.0528776433435,13.632593459332,-0.92747159813772));
#22333=CARTESIAN_POINT('Ctrl Pts',(16.2849105085688,13.7176559737471,-0.937309340881192));
#22334=CARTESIAN_POINT('Ctrl Pts',(16.7142424067725,13.9755352340427,-0.956200886386672));
#22335=CARTESIAN_POINT('Ctrl Pts',(16.9052695294522,14.1496041204308,-0.966822589781085));
#22336=CARTESIAN_POINT('Ctrl Pts',(17.2056519898425,14.5583089437818,-0.98856704606031));
#22337=CARTESIAN_POINT('Ctrl Pts',(17.3135593941965,14.7879324231272,-0.999471341544057));
#22338=CARTESIAN_POINT('Ctrl Pts',(17.4338950578462,15.2696786468988,-1.02006125964282));
#22339=CARTESIAN_POINT('Ctrl Pts',(17.4474891140461,15.5166980415326,-1.02891605404637));
#22340=CARTESIAN_POINT('Ctrl Pts',(17.3798092847476,16.0156874197882,-1.04901448948222));
#22341=CARTESIAN_POINT('Ctrl Pts',(17.2940873361283,16.262135211793,-1.06006877808074));
#22342=CARTESIAN_POINT('Ctrl Pts',(17.0359029314218,16.6981549442992,-1.0819234954729));
#22343=CARTESIAN_POINT('Ctrl Pts',(16.869287872015,16.8855107790962,-1.09251504126423));
#22344=CARTESIAN_POINT('Ctrl Pts',(16.4727055987813,17.1880123647539,-1.11236709942155));
#22345=CARTESIAN_POINT('Ctrl Pts',(16.2460520789443,17.2997096590906,-1.12144644416506));
#22346=CARTESIAN_POINT('Ctrl Pts',(15.7580841554065,17.4316717914015,-1.14249337040046));
#22347=CARTESIAN_POINT('Ctrl Pts',(15.5010293354052,17.4488346169962,-1.15358060292959));
#22348=CARTESIAN_POINT('Ctrl Pts',(15.0046042923773,17.3835494184043,-1.1749922998015));
#22349=CARTESIAN_POINT('Ctrl Pts',(14.7694246897996,17.3053971665795,-1.18513601521548));
#22350=CARTESIAN_POINT('Ctrl Pts',(14.3319804118993,17.0601513562503,-1.20400376656747));
#22351=CARTESIAN_POINT('Ctrl Pts',(14.1358043639573,16.8918928499191,-1.21438674923931));
#22352=CARTESIAN_POINT('Ctrl Pts',(13.822828452168,16.4917126942036,-1.23608437074198));
#22353=CARTESIAN_POINT('Ctrl Pts',(13.7078902728498,16.2646868047079,-1.24704326281027));
#22354=CARTESIAN_POINT('Ctrl Pts',(13.5920235017753,15.8517814523629,-1.26496537710061));
#22355=CARTESIAN_POINT('Ctrl Pts',(13.5679367061315,15.6761515069574,-1.27204517415529));
#22356=CARTESIAN_POINT('Ctrl Pts',(13.5679367061315,15.5000000000001,-1.2786250000002));
#22357=CARTESIAN_POINT('Origin',(15.4999999999998,15.5000000000002,11.20575));
#22358=CARTESIAN_POINT('',(13.5679367061315,15.5000000000002,-1.7786250000002));
#22359=CARTESIAN_POINT('',(13.5679367061315,15.5000000000002,-1.30987500000013));
#22360=CARTESIAN_POINT('',(13.5679367061315,15.5000000000002,11.20575));
#22361=CARTESIAN_POINT('',(13.936917323708,16.6356236642094,-2.22824839960636));
#22362=CARTESIAN_POINT('Ctrl Pts',(13.5679367061315,15.5000000000002,-1.7786250000002));
#22363=CARTESIAN_POINT('Ctrl Pts',(13.5679367061315,15.4713110102307,-1.77969662612257));
#22364=CARTESIAN_POINT('Ctrl Pts',(13.5685756992797,15.4425999920107,-1.78078285553511));
#22365=CARTESIAN_POINT('Ctrl Pts',(13.5812658327813,15.1581590397254,-1.79168131480178));
#22366=CARTESIAN_POINT('Ctrl Pts',(13.6433835357949,14.9072543396241,-1.80239303667409));
#22367=CARTESIAN_POINT('Ctrl Pts',(13.8594981526188,14.449071217981,-1.82416835553235));
#22368=CARTESIAN_POINT('Ctrl Pts',(14.0095359245601,14.2453192500445,-1.83501484570138));
#22369=CARTESIAN_POINT('Ctrl Pts',(14.375576771222,13.9097095423591,-1.85544494571614));
#22370=CARTESIAN_POINT('Ctrl Pts',(14.5868970847757,13.7796534963394,-1.86424124386568));
#22371=CARTESIAN_POINT('Ctrl Pts',(15.057940686529,13.6016248095225,-1.8845581939387));
#22372=CARTESIAN_POINT('Ctrl Pts',(15.3147261183979,13.5596639922916,-1.89563380727755));
#22373=CARTESIAN_POINT('Ctrl Pts',(15.8197591254003,13.5785378998179,-1.91741678097743));
#22374=CARTESIAN_POINT('Ctrl Pts',(16.0633065479973,13.6353374704203,-1.9279214153826));
#22375=CARTESIAN_POINT('Ctrl Pts',(16.519613232597,13.8396294895299,-1.94760273595353));
#22376=CARTESIAN_POINT('Ctrl Pts',(16.7273518610523,13.9867054191127,-1.95690084582151));
#22377=CARTESIAN_POINT('Ctrl Pts',(17.0761951409432,14.3540458830506,-1.97814531087592));
#22378=CARTESIAN_POINT('Ctrl Pts',(17.2132390449659,14.5713394120571,-1.98921739760241));
#22379=CARTESIAN_POINT('Ctrl Pts',(17.3918917772879,15.0377637906816,-2.0104926550159));
#22380=CARTESIAN_POINT('Ctrl Pts',(17.4351931175485,15.281149046348,-2.02038271492798));
#22381=CARTESIAN_POINT('Ctrl Pts',(17.4284331863123,15.7819930618869,-2.039236635147));
#22382=CARTESIAN_POINT('Ctrl Pts',(17.3741617365723,16.034664555002,-2.04984514098204));
#22383=CARTESIAN_POINT('Ctrl Pts',(17.1721421783683,16.500008983052,-2.07158398518824));
#22384=CARTESIAN_POINT('Ctrl Pts',(17.0279622253633,16.7088902827345,-2.08249574332465));
#22385=CARTESIAN_POINT('Ctrl Pts',(16.6721862678626,17.0552935072645,-2.10310764445746));
#22386=CARTESIAN_POINT('Ctrl Pts',(16.4656337930884,17.191302469683,-2.11197549347892));
#22387=CARTESIAN_POINT('Ctrl Pts',(16.0003669871892,17.3839588971004,-2.13204328005094));
#22388=CARTESIAN_POINT('Ctrl Pts',(15.7441588927643,17.4339176130858,-2.14309399179686));
#22389=CARTESIAN_POINT('Ctrl Pts',(15.2372592427903,17.4301770605375,-2.164957477135));
#22390=CARTESIAN_POINT('Ctrl Pts',(14.9914303045821,17.3804225882126,-2.17556051737478));
#22391=CARTESIAN_POINT('Ctrl Pts',(14.6006806201442,17.2188593063065,-2.19241424768811));
#22392=CARTESIAN_POINT('Ctrl Pts',(14.4493679379594,17.1307744676622,-2.19870147391655));
#22393=CARTESIAN_POINT('Ctrl Pts',(14.1693732821569,16.9124347548744,-2.21289549932602));
#22394=CARTESIAN_POINT('Ctrl Pts',(14.0431460179899,16.7818378044134,-2.22049591927601));
#22395=CARTESIAN_POINT('Ctrl Pts',(13.9369173213454,16.6356236661871,-2.22824840453314));
#22396=CARTESIAN_POINT('',(13.9369188502118,16.6356257705296,-1.75949829183043));
#22397=CARTESIAN_POINT('',(13.9369184637306,16.6356252385746,-1.75949832116282));
#22398=CARTESIAN_POINT('Ctrl Pts',(13.9369188502402,16.6356257705687,-1.75949829295567));
#22399=CARTESIAN_POINT('Ctrl Pts',(14.0732165037117,16.8232265616208,-1.74955141913567));
#22400=CARTESIAN_POINT('Ctrl Pts',(14.2421926306503,16.9847823163708,-1.73987267086338));
#22401=CARTESIAN_POINT('Ctrl Pts',(14.6256885475373,17.2378815903649,-1.72214816701704));
#22402=CARTESIAN_POINT('Ctrl Pts',(14.8362794639394,17.3287014043758,-1.71350244965322));
#22403=CARTESIAN_POINT('Ctrl Pts',(15.3036899854226,17.4385845729923,-1.69334220080739));
#22404=CARTESIAN_POINT('Ctrl Pts',(15.5584934383084,17.4476198869582,-1.68235207375451));
#22405=CARTESIAN_POINT('Ctrl Pts',(16.0626255591007,17.3662648208194,-1.6606079568825));
#22406=CARTESIAN_POINT('Ctrl Pts',(16.3065929189333,17.274502945701,-1.65043016901725));
#22407=CARTESIAN_POINT('Ctrl Pts',(16.733960549226,17.0069230177967,-1.63121863353652));
#22408=CARTESIAN_POINT('Ctrl Pts',(16.9157196559872,16.8376064327553,-1.6209743169182));
#22409=CARTESIAN_POINT('Ctrl Pts',(17.2115388605543,16.4321558772132,-1.59944982869598));
#22410=CARTESIAN_POINT('Ctrl Pts',(17.3197729456465,16.197649200397,-1.58835608490567));
#22411=CARTESIAN_POINT('Ctrl Pts',(17.4370349875305,15.7067373188981,-1.56749008537747));
#22412=CARTESIAN_POINT('Ctrl Pts',(17.4475319697598,15.4557223788833,-1.55855468409504));
#22413=CARTESIAN_POINT('Ctrl Pts',(17.3726902789251,14.9634366275315,-1.53855219877789));
#22414=CARTESIAN_POINT('Ctrl Pts',(17.2880297167384,14.7268219856976,-1.52788809973701));
#22415=CARTESIAN_POINT('Ctrl Pts',(17.0300046441306,14.2927306055598,-1.5061088486522));
#22416=CARTESIAN_POINT('Ctrl Pts',(16.8567343671547,14.1008202908097,-1.49520365267544));
#22417=CARTESIAN_POINT('Ctrl Pts',(16.4544579219332,13.8024087055848,-1.47538156930746));
#22418=CARTESIAN_POINT('Ctrl Pts',(16.2319055093252,13.6952482164326,-1.4664433890746));
#22419=CARTESIAN_POINT('Ctrl Pts',(15.7518323297936,13.5679372308724,-1.44573697721879));
#22420=CARTESIAN_POINT('Ctrl Pts',(15.4981347275305,13.551596272361,-1.43479454747419));
#22421=CARTESIAN_POINT('Ctrl Pts',(14.9946779887316,13.6177050294597,-1.41307956103124));
#22422=CARTESIAN_POINT('Ctrl Pts',(14.7500889892401,13.7011232772005,-1.40256300391617));
#22423=CARTESIAN_POINT('Ctrl Pts',(14.3167686917906,13.9530518157521,-1.3838077236402));
#22424=CARTESIAN_POINT('Ctrl Pts',(14.1300765218336,14.1156697545303,-1.37370723711996));
#22425=CARTESIAN_POINT('Ctrl Pts',(13.8216873535974,14.5094994028654,-1.35234574472338));
#22426=CARTESIAN_POINT('Ctrl Pts',(13.7058009544624,14.7392900935939,-1.34126312922336));
#22427=CARTESIAN_POINT('Ctrl Pts',(13.591360276372,15.1530393767012,-1.32334024636834));
#22428=CARTESIAN_POINT('Ctrl Pts',(13.5679367061315,15.3262907155804,-1.31636360097137));
#22429=CARTESIAN_POINT('Ctrl Pts',(13.5679367061315,15.5000000000003,-1.30987500000013));
#22430=CARTESIAN_POINT('Origin',(15.5,-15.5,11.20575));
#22431=CARTESIAN_POINT('',(15.5,-13.5679367061317,1.22137499999989));
#22432=CARTESIAN_POINT('',(15.5,-13.5679367061317,1.3858));
#22433=CARTESIAN_POINT('',(15.5,-13.5679367061317,11.20575));
#22434=CARTESIAN_POINT('',(17.2021646372135,-16.4140591443298,1.3857999999999));
#22435=CARTESIAN_POINT('Origin',(15.5,-15.5,1.3858));
#22436=CARTESIAN_POINT('Ctrl Pts',(17.2021646372131,-16.4140591443306,1.38579999999995));
#22437=CARTESIAN_POINT('Ctrl Pts',(17.2835044921692,-16.2625877372984,1.3792667682509));
#22438=CARTESIAN_POINT('Ctrl Pts',(17.3442533198926,-16.1009564770173,1.37229532392361));
#22439=CARTESIAN_POINT('Ctrl Pts',(17.4225863575886,-15.7606826337724,1.35761870660277));
#22440=CARTESIAN_POINT('Ctrl Pts',(17.4383899414388,-15.583279243606,1.3499669822032));
#22441=CARTESIAN_POINT('Ctrl Pts',(17.4173618065871,-15.150545952148,1.33130242409274));
#22442=CARTESIAN_POINT('Ctrl Pts',(17.354246909013,-14.8998465932948,1.32048931393011));
#22443=CARTESIAN_POINT('Ctrl Pts',(17.1389102320616,-14.4480453999454,1.30100232322681));
#22444=CARTESIAN_POINT('Ctrl Pts',(16.9927945769671,-14.2493134357546,1.29183017937045));
#22445=CARTESIAN_POINT('Ctrl Pts',(16.6281426362718,-13.9112799548102,1.27091926226126));
#22446=CARTESIAN_POINT('Ctrl Pts',(16.410884372517,-13.7774947329751,1.25991876919078));
#22447=CARTESIAN_POINT('Ctrl Pts',(15.9581594815713,-13.6089622530652,1.23937348400477));
#22448=CARTESIAN_POINT('Ctrl Pts',(15.7298816359758,-13.5679367061317,1.22996181912958));
#22449=CARTESIAN_POINT('Ctrl Pts',(15.5,-13.5679367061317,1.22137499999989));
#22450=CARTESIAN_POINT('Origin',(15.5,-15.5,11.20575));
#22451=CARTESIAN_POINT('',(15.5,-13.5679367061317,0.721374999999882));
#22452=CARTESIAN_POINT('',(15.5,-13.5679367061317,1.19012499999984));
#22453=CARTESIAN_POINT('',(15.5,-13.5679367061317,11.20575));
#22454=CARTESIAN_POINT('',(16.7089831815964,-17.0070594673503,1.3858));
#22455=CARTESIAN_POINT('Ctrl Pts',(15.5,-13.5679367061317,1.19012499999984));
#22456=CARTESIAN_POINT('Ctrl Pts',(15.6209597157618,-13.5679367061317,1.19464323477234));
#22457=CARTESIAN_POINT('Ctrl Pts',(15.7419184750194,-13.5792946957063,1.19940637898293));
#22458=CARTESIAN_POINT('Ctrl Pts',(16.1137167329605,-13.6500674067386,1.21482051737712));
#22459=CARTESIAN_POINT('Ctrl Pts',(16.3540308512701,-13.7479960405399,1.22590894156164));
#22460=CARTESIAN_POINT('Ctrl Pts',(16.7741136008819,-14.026702340501,1.24761093429799));
#22461=CARTESIAN_POINT('Ctrl Pts',(16.9519823816307,-14.2016401214962,1.258027594988));
#22462=CARTESIAN_POINT('Ctrl Pts',(17.2359894885833,-14.6147032779413,1.27754424976214));
#22463=CARTESIAN_POINT('Ctrl Pts',(17.3372359040119,-14.8503902891215,1.28710617538617));
#22464=CARTESIAN_POINT('Ctrl Pts',(17.4426537117389,-15.3471703745469,1.30853318586947));
#22465=CARTESIAN_POINT('Ctrl Pts',(17.4459126157984,-15.6033601229582,1.31958310631912));
#22466=CARTESIAN_POINT('Ctrl Pts',(17.357744835181,-16.0780177664297,1.34005593645267));
#22467=CARTESIAN_POINT('Ctrl Pts',(17.2762233318702,-16.2939199281608,1.34923226468177));
#22468=CARTESIAN_POINT('Ctrl Pts',(17.0408566361002,-16.6881134566224,1.36652510317405));
#22469=CARTESIAN_POINT('Ctrl Pts',(16.8884973676933,-16.8630507957942,1.37598889193056));
#22470=CARTESIAN_POINT('Ctrl Pts',(16.7089831815964,-17.0070594673503,1.38579999999999));
#22471=CARTESIAN_POINT('Origin',(15.5,-15.5,1.3858));
#22472=CARTESIAN_POINT('Ctrl Pts',(15.5,-13.5679367061317,1.22137499999989));
#22473=CARTESIAN_POINT('Ctrl Pts',(15.4729341637143,-13.5679367061317,1.22036400388534));
#22474=CARTESIAN_POINT('Ctrl Pts',(15.4458469977579,-13.5685054395913,1.2193399457951));
#22475=CARTESIAN_POINT('Ctrl Pts',(15.1726369387374,-13.5800041737923,1.20888669013352));
#22476=CARTESIAN_POINT('Ctrl Pts',(14.9307787644431,-13.6373364196089,1.19861608777127));
#22477=CARTESIAN_POINT('Ctrl Pts',(14.4729009299767,-13.8436681823131,1.17706314833877));
#22478=CARTESIAN_POINT('Ctrl Pts',(14.2627623231917,-13.9941383691091,1.16596877123743));
#22479=CARTESIAN_POINT('Ctrl Pts',(13.9183617245921,-14.3628583035511,1.14515252623231));
#22480=CARTESIAN_POINT('Ctrl Pts',(13.7853340431921,-14.5755603823523,1.13624772831502));
#22481=CARTESIAN_POINT('Ctrl Pts',(13.6069662800139,-15.0402511769473,1.11620478613719));
#22482=CARTESIAN_POINT('Ctrl Pts',(13.563518985263,-15.2879321565451,1.10552186405143));
#22483=CARTESIAN_POINT('Ctrl Pts',(13.5731954041822,-15.7929752639186,1.08373845470453));
#22484=CARTESIAN_POINT('Ctrl Pts',(13.628926931347,-16.0454493143052,1.07284879893307));
#22485=CARTESIAN_POINT('Ctrl Pts',(13.8310245097158,-16.5036338505738,1.05308648327279));
#22486=CARTESIAN_POINT('Ctrl Pts',(13.9714260897244,-16.7067442547807,1.0441143077112));
#22487=CARTESIAN_POINT('Ctrl Pts',(14.3257784403693,-17.0548537163586,1.02337081594498));
#22488=CARTESIAN_POINT('Ctrl Pts',(14.5383567467269,-17.1945806683055,1.01241699564406));
#22489=CARTESIAN_POINT('Ctrl Pts',(15.0088443360005,-17.3860429606324,0.990713714656131));
#22490=CARTESIAN_POINT('Ctrl Pts',(15.2627143703035,-17.4344332046964,0.980289491368659));
#22491=CARTESIAN_POINT('Ctrl Pts',(15.764107690538,-17.4296140644544,0.961456907738265));
#22492=CARTESIAN_POINT('Ctrl Pts',(16.0069337839783,-17.3804673298746,0.951326678324261));
#22493=CARTESIAN_POINT('Ctrl Pts',(16.4699471299709,-17.1903012304531,0.929930537938738));
#22494=CARTESIAN_POINT('Ctrl Pts',(16.6843681043685,-17.0476412723927,0.918844635164113));
#22495=CARTESIAN_POINT('Ctrl Pts',(17.0422253707064,-16.6904570711204,0.897774518665517));
#22496=CARTESIAN_POINT('Ctrl Pts',(17.1834288053771,-16.4806668481729,0.888672908979973));
#22497=CARTESIAN_POINT('Ctrl Pts',(17.3770350149237,-16.0208578484158,0.868840527314208));
#22498=CARTESIAN_POINT('Ctrl Pts',(17.42837351161,-15.7755220883528,0.858258758726811));
#22499=CARTESIAN_POINT('Ctrl Pts',(17.4355092606312,-15.2690019284845,0.836411641473291));
#22500=CARTESIAN_POINT('Ctrl Pts',(17.3873412235869,-15.0126438266187,0.825354459639089));
#22501=CARTESIAN_POINT('Ctrl Pts',(17.1979533839632,-14.5460700127244,0.805230299482811));
#22502=CARTESIAN_POINT('Ctrl Pts',(17.063281790105,-14.3384565933621,0.796385555323458));
#22503=CARTESIAN_POINT('Ctrl Pts',(16.7193021674531,-13.9803614873582,0.775814169018619));
#22504=CARTESIAN_POINT('Ctrl Pts',(16.5115619839701,-13.8348471766509,0.764916258632763));
#22505=CARTESIAN_POINT('Ctrl Pts',(16.0477927715656,-13.6296318245785,0.743167333659146));
#22506=CARTESIAN_POINT('Ctrl Pts',(15.7954972631553,-13.5735885359089,0.732534660777732));
#22507=CARTESIAN_POINT('Ctrl Pts',(15.5263956112966,-13.568071880497,0.722363876209219));
#22508=CARTESIAN_POINT('Ctrl Pts',(15.5131950985184,-13.5679367061317,0.721867879406689));
#22509=CARTESIAN_POINT('Ctrl Pts',(15.5,-13.5679367061317,0.721374999999882));
#22510=CARTESIAN_POINT('Origin',(15.5,-15.5,11.20575));
#22511=CARTESIAN_POINT('',(15.5000000000001,-13.5679367061317,0.22137499999988));
#22512=CARTESIAN_POINT('',(15.5,-13.5679367061317,0.690124999999829));
#22513=CARTESIAN_POINT('',(15.5,-13.5679367061317,11.20575));
#22514=CARTESIAN_POINT('Ctrl Pts',(15.4999999999999,-13.5679367061317,0.69012499999983));
#22515=CARTESIAN_POINT('Ctrl Pts',(15.663197634803,-13.5679367061317,0.696220957019176));
#22516=CARTESIAN_POINT('Ctrl Pts',(15.8260698424807,-13.5886111528802,0.702750621155672));
#22517=CARTESIAN_POINT('Ctrl Pts',(16.2318407735952,-13.6937750358444,0.720175424526367));
#22518=CARTESIAN_POINT('Ctrl Pts',(16.4638288993578,-13.8061679673983,0.731264781557265));
#22519=CARTESIAN_POINT('Ctrl Pts',(16.8630470507188,-14.108833797682,0.75270412300508));
#22520=CARTESIAN_POINT('Ctrl Pts',(17.028761444196,-14.2932884830899,0.762872018728106));
#22521=CARTESIAN_POINT('Ctrl Pts',(17.2874053587738,-14.7231251438683,0.781803012187292));
#22522=CARTESIAN_POINT('Ctrl Pts',(17.3745003706305,-14.9664736216104,0.79211305640892));
#22523=CARTESIAN_POINT('Ctrl Pts',(17.4482099203794,-15.4692792372004,0.813799958747375));
#22524=CARTESIAN_POINT('Ctrl Pts',(17.4355847239787,-15.723565875171,0.824767794651858));
#22525=CARTESIAN_POINT('Ctrl Pts',(17.3151733744223,-16.2055976541615,0.845558684393085));
#22526=CARTESIAN_POINT('Ctrl Pts',(17.2113496874164,-16.4295122772777,0.854579673980927));
#22527=CARTESIAN_POINT('Ctrl Pts',(16.9190154733788,-16.8359718966524,0.874264961849426));
#22528=CARTESIAN_POINT('Ctrl Pts',(16.7296891979234,-17.0120418978351,0.885134014187554));
#22529=CARTESIAN_POINT('Ctrl Pts',(16.2991617620683,-17.2766178136154,0.906921415251217));
#22530=CARTESIAN_POINT('Ctrl Pts',(16.0634585876014,-17.3648212635817,0.917627873583943));
#22531=CARTESIAN_POINT('Ctrl Pts',(15.5727030691474,-17.4465792698414,0.93772235628183));
#22532=CARTESIAN_POINT('Ctrl Pts',(15.3223565583377,-17.4398199793547,0.946593274573899));
#22533=CARTESIAN_POINT('Ctrl Pts',(14.8300711076984,-17.3302144103329,0.967345462670997));
#22534=CARTESIAN_POINT('Ctrl Pts',(14.5935881752468,-17.2253688342268,0.978439949755269));
#22535=CARTESIAN_POINT('Ctrl Pts',(14.1832015334446,-16.9351538432142,1.00002795682994));
#22536=CARTESIAN_POINT('Ctrl Pts',(14.0110153602745,-16.755615830377,1.01033156193278));
#22537=CARTESIAN_POINT('Ctrl Pts',(13.7379425524706,-16.3329965553295,1.02964587164791));
#22538=CARTESIAN_POINT('Ctrl Pts',(13.6429845085471,-16.0918227958046,1.03959862802551));
#22539=CARTESIAN_POINT('Ctrl Pts',(13.5535333316269,-15.5900949475556,1.06123904433767));
#22540=CARTESIAN_POINT('Ctrl Pts',(13.5584675814187,-15.3347633934782,1.07225194933617));
#22541=CARTESIAN_POINT('Ctrl Pts',(13.6646353766633,-14.8487842127048,1.09321309755165));
#22542=CARTESIAN_POINT('Ctrl Pts',(13.761672278608,-14.6220240391691,1.10246053097514));
#22543=CARTESIAN_POINT('Ctrl Pts',(14.041585270235,-14.2071591450873,1.12186311344001));
#22544=CARTESIAN_POINT('Ctrl Pts',(14.2255255819044,-14.0255156909769,1.13265117917155));
#22545=CARTESIAN_POINT('Ctrl Pts',(14.648495420734,-13.74776419308,1.1544404228268));
#22546=CARTESIAN_POINT('Ctrl Pts',(14.8821830753995,-13.6523788496886,1.16522647893842));
#22547=CARTESIAN_POINT('Ctrl Pts',(15.2505243179915,-13.5800170676889,1.18054575641211));
#22548=CARTESIAN_POINT('Ctrl Pts',(15.3752528162562,-13.5679367061317,1.18546529110574));
#22549=CARTESIAN_POINT('Ctrl Pts',(15.5,-13.5679367061317,1.19012499999984));
#22550=CARTESIAN_POINT('Ctrl Pts',(15.5,-13.5679367061317,0.721374999999882));
#22551=CARTESIAN_POINT('Ctrl Pts',(15.2685828063486,-13.5679367061317,0.712730822847808));
#22552=CARTESIAN_POINT('Ctrl Pts',(15.0388969708039,-13.6095133452991,0.703254680220421));
#22553=CARTESIAN_POINT('Ctrl Pts',(14.5838672575743,-13.7800568344395,0.682579933296358));
#22554=CARTESIAN_POINT('Ctrl Pts',(14.3657373188852,-13.9154007888411,0.67151326490416));
#22555=CARTESIAN_POINT('Ctrl Pts',(13.9955563283149,-14.2617096427834,0.650217354190035));
#22556=CARTESIAN_POINT('Ctrl Pts',(13.8467023152938,-14.4688321611842,0.640851106713065));
#22557=CARTESIAN_POINT('Ctrl Pts',(13.6392165648734,-14.9240794292194,0.621215480666726));
#22558=CARTESIAN_POINT('Ctrl Pts',(13.5807974420006,-15.1670698897687,0.610734869027327));
#22559=CARTESIAN_POINT('Ctrl Pts',(13.5584324818228,-15.6716078298641,0.588973248445474));
#22560=CARTESIAN_POINT('Ctrl Pts',(13.598542278736,-15.9284928588798,0.577893339304166));
#22561=CARTESIAN_POINT('Ctrl Pts',(13.773173526214,-16.4008511610958,0.557519683857022));
#22562=CARTESIAN_POINT('Ctrl Pts',(13.9018579853462,-16.6132862458172,0.54872840560789));
#22563=CARTESIAN_POINT('Ctrl Pts',(14.2349802267053,-16.9816699616753,0.528340694405922));
#22564=CARTESIAN_POINT('Ctrl Pts',(14.4375333639109,-17.1330265345501,0.517510543306561));
#22565=CARTESIAN_POINT('Ctrl Pts',(14.8940137700958,-17.3523384610088,0.495729873520459));
#22566=CARTESIAN_POINT('Ctrl Pts',(15.1444779567369,-17.4162475185621,0.484995974086985));
#22567=CARTESIAN_POINT('Ctrl Pts',(15.644292945993,-17.4421185607808,0.465768343173262));
#22568=CARTESIAN_POINT('Ctrl Pts',(15.8886689106846,-17.4083000037079,0.456344488469386));
#22569=CARTESIAN_POINT('Ctrl Pts',(16.3602738338657,-17.2484328206968,0.435280848151098));
#22570=CARTESIAN_POINT('Ctrl Pts',(16.5819407282909,-17.1206457359146,0.424245033703684));
#22571=CARTESIAN_POINT('Ctrl Pts',(16.9645889726516,-16.7856687238997,0.402727812195782));
#22572=CARTESIAN_POINT('Ctrl Pts',(17.1213576046383,-16.5812682862177,0.393012028302294));
#22573=CARTESIAN_POINT('Ctrl Pts',(17.3428309783919,-16.130730045467,0.373579510995516));
#22574=CARTESIAN_POINT('Ctrl Pts',(17.4082697839647,-15.8902976976571,0.363209235317829));
#22575=CARTESIAN_POINT('Ctrl Pts',(17.4458200822696,-15.3881980765453,0.341552783779496));
#22576=CARTESIAN_POINT('Ctrl Pts',(17.4137884813012,-15.1310281688062,0.330460587311118));
#22577=CARTESIAN_POINT('Ctrl Pts',(17.2540504948445,-14.6530287775216,0.309843621638471));
#22578=CARTESIAN_POINT('Ctrl Pts',(17.1313390172738,-14.4356759590614,0.301024334102504));
#22579=CARTESIAN_POINT('Ctrl Pts',(16.8090342643691,-14.0571971876884,0.280822982049281));
#22580=CARTESIAN_POINT('Ctrl Pts',(16.6117620423532,-13.9002426534532,0.27006936510708));
#22581=CARTESIAN_POINT('Ctrl Pts',(16.1629040887197,-13.6672548471105,0.248278485924882));
#22582=CARTESIAN_POINT('Ctrl Pts',(15.9144966796287,-13.5956339334636,0.237455100705018));
#22583=CARTESIAN_POINT('Ctrl Pts',(15.6062624045507,-13.5701259723312,0.225391456362187));
#22584=CARTESIAN_POINT('Ctrl Pts',(15.5531033073173,-13.5679367061317,0.223358579476269));
#22585=CARTESIAN_POINT('Ctrl Pts',(15.5000000000001,-13.5679367061317,0.221374999999879));
#22586=CARTESIAN_POINT('Origin',(15.5,-15.5,11.20575));
#22587=CARTESIAN_POINT('',(15.5,-13.5679367061317,-0.278625000000132));
#22588=CARTESIAN_POINT('',(15.4999999999999,-13.5679367061317,0.190124999999821));
#22589=CARTESIAN_POINT('',(15.5,-13.5679367061317,11.20575));
#22590=CARTESIAN_POINT('Ctrl Pts',(15.4999999999999,-13.5679367061317,0.190124999999821));
#22591=CARTESIAN_POINT('Ctrl Pts',(15.7052232055908,-13.5679367061317,0.197790747375166));
#22592=CARTESIAN_POINT('Ctrl Pts',(15.9094431243975,-13.6006312438211,0.206124105599974));
#22593=CARTESIAN_POINT('Ctrl Pts',(16.3458500952319,-13.7445092392223,0.225528168010863));
#22594=CARTESIAN_POINT('Ctrl Pts',(16.5687690248994,-13.8706006648951,0.236574181605321));
#22595=CARTESIAN_POINT('Ctrl Pts',(16.9462938014503,-14.1957983248931,0.257689124656267));
#22596=CARTESIAN_POINT('Ctrl Pts',(17.0996068020759,-14.3891741439698,0.267213101031684));
#22597=CARTESIAN_POINT('Ctrl Pts',(17.3312210666002,-14.8328987043052,0.286351732158293));
#22598=CARTESIAN_POINT('Ctrl Pts',(17.403389189678,-15.0810963874238,0.297056940587811));
#22599=CARTESIAN_POINT('Ctrl Pts',(17.4463663432178,-15.5859112111088,0.318830503652366));
#22600=CARTESIAN_POINT('Ctrl Pts',(17.4188098289701,-15.8374917549286,0.329681620893121));
#22601=CARTESIAN_POINT('Ctrl Pts',(17.2705600347068,-16.3114416099335,0.350123922848632));
#22602=CARTESIAN_POINT('Ctrl Pts',(17.1530549287722,-16.5299161239957,0.358922469304659));
#22603=CARTESIAN_POINT('Ctrl Pts',(16.8349526369196,-16.9202726297615,0.379222999836066));
#22604=CARTESIAN_POINT('Ctrl Pts',(16.6338441663768,-17.085451210082,0.390297271892839));
#22605=CARTESIAN_POINT('Ctrl Pts',(16.1874197433205,-17.3225641667436,0.412086213416755));
#22606=CARTESIAN_POINT('Ctrl Pts',(15.9481982603318,-17.3956324394973,0.422597688314654));
#22607=CARTESIAN_POINT('Ctrl Pts',(15.4510757841914,-17.4478128352924,0.442292129851002));
#22608=CARTESIAN_POINT('Ctrl Pts',(15.1977325915627,-17.4248413113895,0.451571409240313));
#22609=CARTESIAN_POINT('Ctrl Pts',(14.7117348553567,-17.2822086107985,0.472800990486173));
#22610=CARTESIAN_POINT('Ctrl Pts',(14.4841033890512,-17.1630032804563,0.483874527712213));
#22611=CARTESIAN_POINT('Ctrl Pts',(14.0954494858794,-16.8491384993429,0.505160775836598));
#22612=CARTESIAN_POINT('Ctrl Pts',(13.935845283737,-16.6603046231705,0.515078993620139));
#22613=CARTESIAN_POINT('Ctrl Pts',(13.6903827463215,-16.223642546113,0.533913007255683));
#22614=CARTESIAN_POINT('Ctrl Pts',(13.6105539996563,-15.9778499407052,0.544514480397023));
#22615=CARTESIAN_POINT('Ctrl Pts',(13.5518158441316,-15.4739117712167,0.566250231803642));
#22616=CARTESIAN_POINT('Ctrl Pts',(13.571742794709,-15.2208352901084,0.577165871485818));
#22617=CARTESIAN_POINT('Ctrl Pts',(13.7057278794298,-14.742684868917,0.597789351347523));
#22618=CARTESIAN_POINT('Ctrl Pts',(13.8161488953126,-14.5214408844327,0.606664573343451));
#22619=CARTESIAN_POINT('Ctrl Pts',(14.1219606735895,-14.1213400688706,0.626716158351945));
#22620=CARTESIAN_POINT('Ctrl Pts',(14.318568611901,-13.9495491173579,0.637764922719238));
#22621=CARTESIAN_POINT('Ctrl Pts',(14.7590310485592,-13.6984440207756,0.659632917824901));
#22622=CARTESIAN_POINT('Ctrl Pts',(14.9966959458147,-13.6181551918391,0.670241966963359));
#22623=CARTESIAN_POINT('Ctrl Pts',(15.3284077888473,-13.5736457522818,0.683592357862532));
#22624=CARTESIAN_POINT('Ctrl Pts',(15.4142441778543,-13.5679367061317,0.686921743980895));
#22625=CARTESIAN_POINT('Ctrl Pts',(15.4999999999999,-13.5679367061317,0.690124999999829));
#22626=CARTESIAN_POINT('Ctrl Pts',(15.5000000000001,-13.5679367061317,0.221374999999879));
#22627=CARTESIAN_POINT('Ctrl Pts',(15.3093450221423,-13.5679367061317,0.214253422827828));
#22628=CARTESIAN_POINT('Ctrl Pts',(15.1194546083814,-13.5961535790767,0.206551882575901));
#22629=CARTESIAN_POINT('Ctrl Pts',(14.6948718232558,-13.7256105046371,0.187900494787472));
#22630=CARTESIAN_POINT('Ctrl Pts',(14.4700098904008,-13.8459724738417,0.176905464603589));
#22631=CARTESIAN_POINT('Ctrl Pts',(14.0753526090742,-14.1696924217256,0.155182435525569));
#22632=CARTESIAN_POINT('Ctrl Pts',(13.9107790537501,-14.3714265999853,0.145052382171085));
#22633=CARTESIAN_POINT('Ctrl Pts',(13.6758632413355,-14.8173319838793,0.125819688237564));
#22634=CARTESIAN_POINT('Ctrl Pts',(13.6037990124408,-15.0551292052584,0.115563070259359));
#22635=CARTESIAN_POINT('Ctrl Pts',(13.5518334963172,-15.5544792850638,0.0940252113380078));
#22636=CARTESIAN_POINT('Ctrl Pts',(13.5761558231528,-15.8116932971635,0.0829311125699534));
#22637=CARTESIAN_POINT('Ctrl Pts',(13.7215598037034,-16.2949297857371,0.0620882615572829));
#22638=CARTESIAN_POINT('Ctrl Pts',(13.8385708540846,-16.5170608745389,0.0531675695736204));
#22639=CARTESIAN_POINT('Ctrl Pts',(14.1505967901205,-16.9049967004005,0.0331462146120232));
#22640=CARTESIAN_POINT('Ctrl Pts',(14.3427581391604,-17.0670614604204,0.0224732986552362));
#22641=CARTESIAN_POINT('Ctrl Pts',(14.7840616507215,-17.3126898337665,0.000691997111495622));
#22642=CARTESIAN_POINT('Ctrl Pts',(15.0303088811274,-17.3915129002971,-0.0102060193255635));
#22643=CARTESIAN_POINT('Ctrl Pts',(15.5280187230135,-17.4473055261743,-0.0300003018240521));
#22644=CARTESIAN_POINT('Ctrl Pts',(15.7742335758728,-17.4281050083783,-0.0389538708149526));
#22645=CARTESIAN_POINT('Ctrl Pts',(16.2532901705975,-17.296907710707,-0.0596775634273534));
#22646=CARTESIAN_POINT('Ctrl Pts',(16.4808992967149,-17.1834947938276,-0.0706253476172892));
#22647=CARTESIAN_POINT('Ctrl Pts',(16.8829707781072,-16.8732369847255,-0.0923349979158201));
#22648=CARTESIAN_POINT('Ctrl Pts',(17.0524923783306,-16.6781753243463,-0.102808198428218));
#22649=CARTESIAN_POINT('Ctrl Pts',(17.3005030645304,-16.2425026235966,-0.121599538500263));
#22650=CARTESIAN_POINT('Ctrl Pts',(17.3801675176942,-16.0080032121443,-0.131713916058721));
#22651=CARTESIAN_POINT('Ctrl Pts',(17.4487724674381,-15.5123656486931,-0.153091647532988));
#22652=CARTESIAN_POINT('Ctrl Pts',(17.4333995515655,-15.2553808907698,-0.164175858159823));
#22653=CARTESIAN_POINT('Ctrl Pts',(17.3048200987405,-14.7662503100071,-0.185272931873504));
#22654=CARTESIAN_POINT('Ctrl Pts',(17.1944566843434,-14.5384527982996,-0.194401543720054));
#22655=CARTESIAN_POINT('Ctrl Pts',(16.894334784917,-14.139727275418,-0.214210934024622));
#22656=CARTESIAN_POINT('Ctrl Pts',(16.708188966555,-13.9720032635188,-0.224781197355577));
#22657=CARTESIAN_POINT('Ctrl Pts',(16.2741834170983,-13.7111048249335,-0.246619209086019));
#22658=CARTESIAN_POINT('Ctrl Pts',(16.0284985549801,-13.6237773096857,-0.257679625272395));
#22659=CARTESIAN_POINT('Ctrl Pts',(15.6823226738687,-13.574383016875,-0.271675640769364));
#22660=CARTESIAN_POINT('Ctrl Pts',(15.5911253193961,-13.5679367061317,-0.275221175973618));
#22661=CARTESIAN_POINT('Ctrl Pts',(15.5,-13.5679367061317,-0.278625000000132));
#22662=CARTESIAN_POINT('Origin',(15.5,-15.5,11.20575));
#22663=CARTESIAN_POINT('',(15.5,-13.5679367061317,-0.778625000000138));
#22664=CARTESIAN_POINT('',(15.5000000000213,-13.5679367061317,-0.30987499999859));
#22665=CARTESIAN_POINT('',(15.5,-13.5679367061317,11.20575));
#22666=CARTESIAN_POINT('Ctrl Pts',(15.5000000000426,-13.5679367061317,-0.30987499999859));
#22667=CARTESIAN_POINT('Ctrl Pts',(15.7451189900435,-13.5679367061371,-0.300719016644455));
#22668=CARTESIAN_POINT('Ctrl Pts',(15.9880788836297,-13.6145849104549,-0.290637672395874));
#22669=CARTESIAN_POINT('Ctrl Pts',(16.4525087353532,-13.7998506160078,-0.269294302322051));
#22670=CARTESIAN_POINT('Ctrl Pts',(16.6681650113368,-13.9401358945745,-0.258213469136004));
#22671=CARTESIAN_POINT('Ctrl Pts',(17.0300510391149,-14.293798813587,-0.237068805018263));
#22672=CARTESIAN_POINT('Ctrl Pts',(17.1737375672253,-14.5027181075033,-0.227889545454448));
#22673=CARTESIAN_POINT('Ctrl Pts',(17.3718881645073,-14.9610456268797,-0.208121062677908));
#22674=CARTESIAN_POINT('Ctrl Pts',(17.4255568606796,-15.2056351161721,-0.19757148207893));
#22675=CARTESIAN_POINT('Ctrl Pts',(17.437485526191,-15.7028273877144,-0.176126693273793));
#22676=CARTESIAN_POINT('Ctrl Pts',(17.3951930471992,-15.9508283805331,-0.16542996844748));
#22677=CARTESIAN_POINT('Ctrl Pts',(17.21903750586,-16.416216845007,-0.145356934524323));
#22678=CARTESIAN_POINT('Ctrl Pts',(17.087177913888,-16.6293413959128,-0.1364726175302));
#22679=CARTESIAN_POINT('Ctrl Pts',(16.7447233478944,-16.9997020048593,-0.115693680499745));
#22680=CARTESIAN_POINT('Ctrl Pts',(16.535223519972,-17.1512859841674,-0.104599143917209));
#22681=CARTESIAN_POINT('Ctrl Pts',(16.0781299074097,-17.3599329092899,-0.0830255691567002));
#22682=CARTESIAN_POINT('Ctrl Pts',(15.8364334516315,-17.4184418092008,-0.072735631907537));
#22683=CARTESIAN_POINT('Ctrl Pts',(15.3335771418074,-17.4419572678446,-0.0534451981390429));
#22684=CARTESIAN_POINT('Ctrl Pts',(15.0770448720173,-17.4026393126747,-0.0434417100341444));
#22685=CARTESIAN_POINT('Ctrl Pts',(14.5982616364445,-17.2273302215971,-0.0217769181315674));
#22686=CARTESIAN_POINT('Ctrl Pts',(14.3801849192581,-17.0946215718084,-0.0107690704262214));
#22687=CARTESIAN_POINT('Ctrl Pts',(14.0137016048736,-16.7583973031524,0.010171237110501));
#22688=CARTESIAN_POINT('Ctrl Pts',(13.8665662971669,-16.5604348396372,0.0193865553793814));
#22689=CARTESIAN_POINT('Ctrl Pts',(13.648896034541,-16.1097762694873,0.0388242627076073));
#22690=CARTESIAN_POINT('Ctrl Pts',(13.5844810246986,-15.8594139033154,0.0496228377752729));
#22691=CARTESIAN_POINT('Ctrl Pts',(13.5572975229277,-15.3542160204943,0.0714129228630833));
#22692=CARTESIAN_POINT('Ctrl Pts',(13.5924291711366,-15.1043600205154,0.0821896574543681));
#22693=CARTESIAN_POINT('Ctrl Pts',(13.7549549306398,-14.6347353821395,0.102445405107949));
#22694=CARTESIAN_POINT('Ctrl Pts',(13.8797188217565,-14.4190031858112,0.111248274994824));
#22695=CARTESIAN_POINT('Ctrl Pts',(14.2102312356738,-14.0387180251795,0.131795166002757));
#22696=CARTESIAN_POINT('Ctrl Pts',(14.4157066951986,-13.8803875205858,0.142884874300422));
#22697=CARTESIAN_POINT('Ctrl Pts',(14.8677637645239,-13.6576628179057,0.164573917775848));
#22698=CARTESIAN_POINT('Ctrl Pts',(15.1083498919245,-13.5919750720435,0.174977198896065));
#22699=CARTESIAN_POINT('Ctrl Pts',(15.4031822744539,-13.569754032749,0.186469354010822));
#22700=CARTESIAN_POINT('Ctrl Pts',(15.4516175612204,-13.5679367061317,0.188317760160551));
#22701=CARTESIAN_POINT('Ctrl Pts',(15.4999999999999,-13.5679367061317,0.190124999999821));
#22702=CARTESIAN_POINT('Ctrl Pts',(15.5,-13.5679367061317,-0.278625000000131));
#22703=CARTESIAN_POINT('Ctrl Pts',(15.3467892597189,-13.5679367061317,-0.284347914359666));
#22704=CARTESIAN_POINT('Ctrl Pts',(15.1938118281016,-13.5861582264254,-0.290455077212558));
#22705=CARTESIAN_POINT('Ctrl Pts',(14.8002115590521,-13.6816903721264,-0.30721755017852));
#22706=CARTESIAN_POINT('Ctrl Pts',(14.5700164472504,-13.7879612604545,-0.318107905048228));
#22707=CARTESIAN_POINT('Ctrl Pts',(14.1593674324255,-14.0854112710006,-0.339861742243558));
#22708=CARTESIAN_POINT('Ctrl Pts',(13.9839732656644,-14.2752366145712,-0.350507031688753));
#22709=CARTESIAN_POINT('Ctrl Pts',(13.7231840673424,-14.7026885542338,-0.369466729765817));
#22710=CARTESIAN_POINT('Ctrl Pts',(13.6365422675758,-14.9340075266013,-0.37921273586801));
#22711=CARTESIAN_POINT('Ctrl Pts',(13.5527035685452,-15.4259040924359,-0.400429111447581));
#22712=CARTESIAN_POINT('Ctrl Pts',(13.5598498556332,-15.6824101504194,-0.411492674857324));
#22713=CARTESIAN_POINT('Ctrl Pts',(13.6708737217057,-16.1685436044088,-0.432460477152238));
#22714=CARTESIAN_POINT('Ctrl Pts',(13.7700581636469,-16.3943923190575,-0.441627804171639));
#22715=CARTESIAN_POINT('Ctrl Pts',(14.0539091255659,-16.8066128735469,-0.46112045496409));
#22716=CARTESIAN_POINT('Ctrl Pts',(14.2395717537967,-16.9865111568954,-0.471935218600938));
#22717=CARTESIAN_POINT('Ctrl Pts',(14.6649766982385,-17.260117111467,-0.493726018953733));
#22718=CARTESIAN_POINT('Ctrl Pts',(14.8993253045762,-17.3532344934425,-0.50448785312903));
#22719=CARTESIAN_POINT('Ctrl Pts',(15.3879151897707,-17.4445879148856,-0.524708376132417));
#22720=CARTESIAN_POINT('Ctrl Pts',(15.6373703514434,-17.4429655287442,-0.533521108433316));
#22721=CARTESIAN_POINT('Ctrl Pts',(16.1314699144086,-17.3439130073667,-0.554113473589034));
#22722=CARTESIAN_POINT('Ctrl Pts',(16.3705992585577,-17.2437932713042,-0.565204895717519));
#22723=CARTESIAN_POINT('Ctrl Pts',(16.7876645305446,-16.9614315561499,-0.586873008236942));
#22724=CARTESIAN_POINT('Ctrl Pts',(16.9637580966902,-16.7850271274736,-0.597254988511056));
#22725=CARTESIAN_POINT('Ctrl Pts',(17.2443400454302,-16.3689556312255,-0.616708580128513));
#22726=CARTESIAN_POINT('Ctrl Pts',(17.3436265737928,-16.1315609718477,-0.626384649668764));
#22727=CARTESIAN_POINT('Ctrl Pts',(17.4440644805083,-15.6332086945697,-0.647879471588744));
#22728=CARTESIAN_POINT('Ctrl Pts',(17.4447534368414,-15.3772600500546,-0.658918992797644));
#22729=CARTESIAN_POINT('Ctrl Pts',(17.3489811389163,-14.8884838636653,-0.680000780850369));
#22730=CARTESIAN_POINT('Ctrl Pts',(17.2568181639608,-14.6596166093872,-0.689459136144938));
#22731=CARTESIAN_POINT('Ctrl Pts',(16.9858620067821,-14.238805099094,-0.708655396087524));
#22732=CARTESIAN_POINT('Ctrl Pts',(16.8058878841893,-14.0532686231487,-0.719379268374338));
#22733=CARTESIAN_POINT('Ctrl Pts',(16.3885881553997,-13.7662002686923,-0.741157641480895));
#22734=CARTESIAN_POINT('Ctrl Pts',(16.1564785085564,-13.665689225055,-0.751995294214013));
#22735=CARTESIAN_POINT('Ctrl Pts',(15.7761115117429,-13.5827427725166,-0.767992040173275));
#22736=CARTESIAN_POINT('Ctrl Pts',(15.6381065100508,-13.5679367061317,-0.773466277262654));
#22737=CARTESIAN_POINT('Ctrl Pts',(15.5,-13.5679367061317,-0.778625000000138));
#22738=CARTESIAN_POINT('Origin',(15.5,-15.5,11.20575));
#22739=CARTESIAN_POINT('',(15.4999999999999,-13.5679367061317,-1.27862500000015));
#22740=CARTESIAN_POINT('',(15.5,-13.5679367061317,-0.809875000000185));
#22741=CARTESIAN_POINT('',(15.5,-13.5679367061317,11.20575));
#22742=CARTESIAN_POINT('Ctrl Pts',(15.5000000000001,-13.5679367061317,-0.809875000000184));
#22743=CARTESIAN_POINT('Ctrl Pts',(15.5387848588903,-13.5679367061317,-0.808426260665929));
#22744=CARTESIAN_POINT('Ctrl Pts',(15.5776081217821,-13.569104553761,-0.806950901143725));
#22745=CARTESIAN_POINT('Ctrl Pts',(15.8627498107999,-13.5863172258654,-0.79592873452912));
#22746=CARTESIAN_POINT('Ctrl Pts',(16.1039441624047,-13.6482441649587,-0.785583839426259));
#22747=CARTESIAN_POINT('Ctrl Pts',(16.5586938389718,-13.8636040208236,-0.763953047887055));
#22748=CARTESIAN_POINT('Ctrl Pts',(16.7663048606795,-14.0184106751406,-0.752859564438582));
#22749=CARTESIAN_POINT('Ctrl Pts',(17.1030886658293,-14.3935142993235,-0.73219016123049));
#22750=CARTESIAN_POINT('Ctrl Pts',(17.2315636886463,-14.6078734364709,-0.723354008700342));
#22751=CARTESIAN_POINT('Ctrl Pts',(17.4012591024431,-15.0752831240919,-0.703193795820486));
#22752=CARTESIAN_POINT('Ctrl Pts',(17.4401670421017,-15.3241884796659,-0.692458064216697));
#22753=CARTESIAN_POINT('Ctrl Pts',(17.4209116308134,-15.8293918059367,-0.670667744343198));
#22754=CARTESIAN_POINT('Ctrl Pts',(17.3604173282467,-16.0807480284641,-0.659826302479591));
#22755=CARTESIAN_POINT('Ctrl Pts',(17.1497816929781,-16.5348352725858,-0.640240710332106));
#22756=CARTESIAN_POINT('Ctrl Pts',(17.0057085011959,-16.7351193667879,-0.631148276498292));
#22757=CARTESIAN_POINT('Ctrl Pts',(16.6447314320371,-17.0767669839641,-0.610296685602457));
#22758=CARTESIAN_POINT('Ctrl Pts',(16.4291281586241,-17.2126942752496,-0.599311816112351));
#22759=CARTESIAN_POINT('Ctrl Pts',(15.9522914740593,-17.396071415368,-0.577545739488896));
#22760=CARTESIAN_POINT('Ctrl Pts',(15.6949512567242,-17.4394863853226,-0.567317142600485));
#22761=CARTESIAN_POINT('Ctrl Pts',(15.1907605692904,-17.4229690903241,-0.548127787168027));
#22762=CARTESIAN_POINT('Ctrl Pts',(14.9485965706545,-17.3679857370151,-0.53789641724223));
#22763=CARTESIAN_POINT('Ctrl Pts',(14.4891878782661,-17.166282104194,-0.516386105083495));
#22764=CARTESIAN_POINT('Ctrl Pts',(14.2777915836231,-17.0180420352629,-0.505292843771063));
#22765=CARTESIAN_POINT('Ctrl Pts',(13.9295152530061,-16.6526099917286,-0.484402733995875));
#22766=CARTESIAN_POINT('Ctrl Pts',(13.7941507738708,-16.4407479085025,-0.475451133965662));
#22767=CARTESIAN_POINT('Ctrl Pts',(13.611383887522,-15.9774528011728,-0.455468390267086));
#22768=CARTESIAN_POINT('Ctrl Pts',(13.5656468617909,-15.7304237057034,-0.444813585105621));
#22769=CARTESIAN_POINT('Ctrl Pts',(13.5704710073905,-15.2255315160606,-0.423036685109424));
#22770=CARTESIAN_POINT('Ctrl Pts',(13.623779229161,-14.9725259783178,-0.412124105341039));
#22771=CARTESIAN_POINT('Ctrl Pts',(13.8215336428728,-14.5122846645607,-0.392273077201934));
#22772=CARTESIAN_POINT('Ctrl Pts',(13.9600852553974,-14.3077326406346,-0.383350131532038));
#22773=CARTESIAN_POINT('Ctrl Pts',(14.311092329695,-13.9563854884097,-0.362661772922335));
#22774=CARTESIAN_POINT('Ctrl Pts',(14.5221235135244,-13.814770334655,-0.351725021873647));
#22775=CARTESIAN_POINT('Ctrl Pts',(14.9904064163151,-13.6188695990394,-0.330008374038312));
#22776=CARTESIAN_POINT('Ctrl Pts',(15.2437584839143,-13.5679791180275,-0.319447360158956));
#22777=CARTESIAN_POINT('Ctrl Pts',(15.4997866765027,-13.5679367149642,-0.309882968509973));
#22778=CARTESIAN_POINT('Ctrl Pts',(15.4998933384699,-13.5679367061317,-0.309878984151688));
#22779=CARTESIAN_POINT('Ctrl Pts',(15.5000000000426,-13.5679367061317,-0.30987499999859));
#22780=CARTESIAN_POINT('Ctrl Pts',(15.5,-13.5679367061317,-0.778625000000138));
#22781=CARTESIAN_POINT('Ctrl Pts',(15.3931460600035,-13.5679367061317,-0.782616338639041));
#22782=CARTESIAN_POINT('Ctrl Pts',(15.2862458066186,-13.5768002208548,-0.786800556825666));
#22783=CARTESIAN_POINT('Ctrl Pts',(14.9264097349309,-13.6371564581267,-0.801543228515925));
#22784=CARTESIAN_POINT('Ctrl Pts',(14.6835020776055,-13.7301105172148,-0.812621248594988));
#22785=CARTESIAN_POINT('Ctrl Pts',(14.2567488546817,-14.0004851883713,-0.834392725983059));
#22786=CARTESIAN_POINT('Ctrl Pts',(14.0749328111488,-14.1720617647974,-0.844884342273106));
#22787=CARTESIAN_POINT('Ctrl Pts',(13.7832732837112,-14.5783544242248,-0.864540827785101));
#22788=CARTESIAN_POINT('Ctrl Pts',(13.6776776440773,-14.8102645186437,-0.873875479390643));
#22789=CARTESIAN_POINT('Ctrl Pts',(13.5612057991943,-15.3034623332341,-0.895147980148236));
#22790=CARTESIAN_POINT('Ctrl Pts',(13.552197396611,-15.5600993604861,-0.906217192531462));
#22791=CARTESIAN_POINT('Ctrl Pts',(13.6325934592672,-16.0528776431264,-0.927471598128334));
#22792=CARTESIAN_POINT('Ctrl Pts',(13.7176559736562,-16.2849105083636,-0.937309340873369));
#22793=CARTESIAN_POINT('Ctrl Pts',(13.9755352339037,-16.7142424065984,-0.956200886377741));
#22794=CARTESIAN_POINT('Ctrl Pts',(14.1496041202698,-16.9052695292978,-0.966822589771756));
#22795=CARTESIAN_POINT('Ctrl Pts',(14.5583089435885,-17.2056519897364,-0.988567046050803));
#22796=CARTESIAN_POINT('Ctrl Pts',(14.7879324229243,-17.3135593941174,-0.999471341534755));
#22797=CARTESIAN_POINT('Ctrl Pts',(15.2696786466829,-17.4338950578203,-1.02006125963416));
#22798=CARTESIAN_POINT('Ctrl Pts',(15.5166980413127,-17.4474891140478,-1.02891605403808));
#22799=CARTESIAN_POINT('Ctrl Pts',(16.0156874195765,-17.3798092848061,-1.04901448947301));
#22800=CARTESIAN_POINT('Ctrl Pts',(16.2621352115938,-17.2940873362134,-1.06006877807144));
#22801=CARTESIAN_POINT('Ctrl Pts',(16.698154944133,-17.0359029315518,-1.08192349546387));
#22802=CARTESIAN_POINT('Ctrl Pts',(16.8855107789499,-16.8692878721634,-1.09251504125555));
#22803=CARTESIAN_POINT('Ctrl Pts',(17.1880123646469,-16.472705598965,-1.11236709941354));
#22804=CARTESIAN_POINT('Ctrl Pts',(17.2997096590055,-16.2460520791468,-1.12144644415624));
#22805=CARTESIAN_POINT('Ctrl Pts',(17.431671791372,-15.7580841556283,-1.1424933703908));
#22806=CARTESIAN_POINT('Ctrl Pts',(17.4488346169962,-15.5010293356259,-1.15358060291997));
#22807=CARTESIAN_POINT('Ctrl Pts',(17.383549418459,-15.0046042925852,-1.17499229979244));
#22808=CARTESIAN_POINT('Ctrl Pts',(17.3053971666591,-14.7694246899964,-1.18513601520691));
#22809=CARTESIAN_POINT('Ctrl Pts',(17.0601513563756,-14.3319804120671,-1.20400376656016));
#22810=CARTESIAN_POINT('Ctrl Pts',(16.8918928500653,-14.1358043641068,-1.21438674923054));
#22811=CARTESIAN_POINT('Ctrl Pts',(16.491712694381,-13.8228284522729,-1.23608437073301));
#22812=CARTESIAN_POINT('Ctrl Pts',(16.264686804895,-13.7078902729296,-1.24704326280146));
#22813=CARTESIAN_POINT('Ctrl Pts',(15.8517814524953,-13.5920235017939,-1.26496537709516));
#22814=CARTESIAN_POINT('Ctrl Pts',(15.676151507024,-13.5679367061317,-1.27204517415274));
#22815=CARTESIAN_POINT('Ctrl Pts',(15.4999999999999,-13.5679367061317,-1.27862500000015));
#22816=CARTESIAN_POINT('Origin',(15.5,-15.5,11.20575));
#22817=CARTESIAN_POINT('',(15.5,-13.5679367061317,-1.77862500000015));
#22818=CARTESIAN_POINT('',(15.5,-13.5679367061317,-1.30987500000019));
#22819=CARTESIAN_POINT('',(15.5,-13.5679367061317,11.20575));
#22820=CARTESIAN_POINT('',(16.6356236642092,-13.9369173237082,-2.22824839960634));
#22821=CARTESIAN_POINT('Ctrl Pts',(15.5,-13.5679367061317,-1.77862500000015));
#22822=CARTESIAN_POINT('Ctrl Pts',(15.4713110103049,-13.5679367061317,-1.77969662611974));
#22823=CARTESIAN_POINT('Ctrl Pts',(15.4425999921594,-13.5685756992767,-1.78078285552937));
#22824=CARTESIAN_POINT('Ctrl Pts',(15.1581590399474,-13.5812658327421,-1.79168131479254));
#22825=CARTESIAN_POINT('Ctrl Pts',(14.9072543398391,-13.6433835357265,-1.80239303666449));
#22826=CARTESIAN_POINT('Ctrl Pts',(14.4490712181685,-13.8594981524984,-1.82416835552268));
#22827=CARTESIAN_POINT('Ctrl Pts',(14.2453192502126,-14.0095359244182,-1.83501484569199));
#22828=CARTESIAN_POINT('Ctrl Pts',(13.9097095424868,-14.3755767710421,-1.85544494570745));
#22829=CARTESIAN_POINT('Ctrl Pts',(13.779653496445,-14.5868970845778,-1.86424124385709));
#22830=CARTESIAN_POINT('Ctrl Pts',(13.601624809573,-15.0579406863098,-1.88455819392919));
#22831=CARTESIAN_POINT('Ctrl Pts',(13.5596639923122,-15.314726118177,-1.89563380726797));
#22832=CARTESIAN_POINT('Ctrl Pts',(13.5785378997819,-15.8197591251871,-1.9174167809682));
#22833=CARTESIAN_POINT('Ctrl Pts',(13.635337470358,-16.063306547793,-1.92792141537377));
#22834=CARTESIAN_POINT('Ctrl Pts',(13.8396294894159,-16.5196132324098,-1.94760273594545));
#22835=CARTESIAN_POINT('Ctrl Pts',(13.98670541897,-16.7273518608751,-1.95690084581238));
#22836=CARTESIAN_POINT('Ctrl Pts',(14.3540458828622,-17.0761951408069,-1.97814531086595));
#22837=CARTESIAN_POINT('Ctrl Pts',(14.5713394118551,-17.213239044857,-1.9892173975925));
#22838=CARTESIAN_POINT('Ctrl Pts',(15.0377637904636,-17.3918917772351,-2.01049265500658));
#22839=CARTESIAN_POINT('Ctrl Pts',(15.2811490461273,-17.4351931175239,-2.02038271492023));
#22840=CARTESIAN_POINT('Ctrl Pts',(15.7819930616688,-17.4284331863443,-2.03923663513813));
#22841=CARTESIAN_POINT('Ctrl Pts',(16.0346645547899,-17.3741617366328,-2.04984514097278));
#22842=CARTESIAN_POINT('Ctrl Pts',(16.500008982865,-17.1721421784805,-2.0715839851788));
#22843=CARTESIAN_POINT('Ctrl Pts',(16.7088902825659,-17.0279622254971,-2.08249574331544));
#22844=CARTESIAN_POINT('Ctrl Pts',(17.055293507135,-16.6721862680338,-2.10310764444889));
#22845=CARTESIAN_POINT('Ctrl Pts',(17.191302469575,-16.4656337932766,-2.11197549347074));
#22846=CARTESIAN_POINT('Ctrl Pts',(17.383958897045,-16.0003669873985,-2.13204328004182));
#22847=CARTESIAN_POINT('Ctrl Pts',(17.4339176130592,-15.7441588929761,-2.14309399178763));
#22848=CARTESIAN_POINT('Ctrl Pts',(17.4301770605656,-15.2372592429962,-2.16495747712602));
#22849=CARTESIAN_POINT('Ctrl Pts',(17.3804225882662,-14.9914303047801,-2.17556051736614));
#22850=CARTESIAN_POINT('Ctrl Pts',(17.2188593063871,-14.6006806202927,-2.19241424768163));
#22851=CARTESIAN_POINT('Ctrl Pts',(17.1307744677382,-14.4493679380718,-2.19870147391129));
#22852=CARTESIAN_POINT('Ctrl Pts',(16.9124347549226,-14.1693732822038,-2.21289549932321));
#22853=CARTESIAN_POINT('Ctrl Pts',(16.78183780444,-14.0431460180095,-2.22049591927456));
#22854=CARTESIAN_POINT('Ctrl Pts',(16.6356236661869,-13.9369173213456,-2.22824840453312));
#22855=CARTESIAN_POINT('',(16.6356257705294,-13.936918850212,-1.75949829183042));
#22856=CARTESIAN_POINT('',(16.6356252385745,-13.9369184637308,-1.75949832116282));
#22857=CARTESIAN_POINT('Ctrl Pts',(16.6356257705685,-13.9369188502404,-1.75949829295571));
#22858=CARTESIAN_POINT('Ctrl Pts',(16.8232265616208,-14.0732165037121,-1.74955141913566));
#22859=CARTESIAN_POINT('Ctrl Pts',(16.9847823163708,-14.2421926306508,-1.73987267086339));
#22860=CARTESIAN_POINT('Ctrl Pts',(17.2378815903649,-14.625688547538,-1.72214816701709));
#22861=CARTESIAN_POINT('Ctrl Pts',(17.3287014043758,-14.8362794639401,-1.71350244965325));
#22862=CARTESIAN_POINT('Ctrl Pts',(17.4385845729922,-15.3036899854237,-1.69334220080742));
#22863=CARTESIAN_POINT('Ctrl Pts',(17.447619886958,-15.5584934383095,-1.68235207375453));
#22864=CARTESIAN_POINT('Ctrl Pts',(17.366264820819,-16.0626255591014,-1.66060795688252));
#22865=CARTESIAN_POINT('Ctrl Pts',(17.2745029457006,-16.306592918934,-1.65043016901723));
#22866=CARTESIAN_POINT('Ctrl Pts',(17.0069230177962,-16.7339605492266,-1.63121863353648));
#22867=CARTESIAN_POINT('Ctrl Pts',(16.8376064327547,-16.9157196559878,-1.62097431691815));
#22868=CARTESIAN_POINT('Ctrl Pts',(16.4321558772125,-17.2115388605548,-1.59944982869592));
#22869=CARTESIAN_POINT('Ctrl Pts',(16.1976492003963,-17.3197729456469,-1.58835608490563));
#22870=CARTESIAN_POINT('Ctrl Pts',(15.7067373188974,-17.4370349875308,-1.56749008537744));
#22871=CARTESIAN_POINT('Ctrl Pts',(15.4557223788825,-17.44753196976,-1.55855468409501));
#22872=CARTESIAN_POINT('Ctrl Pts',(14.9634366275308,-17.3726902789252,-1.53855219877784));
#22873=CARTESIAN_POINT('Ctrl Pts',(14.726821985697,-17.2880297167385,-1.52788809973695));
#22874=CARTESIAN_POINT('Ctrl Pts',(14.2927306055592,-17.0300046441306,-1.50610884865212));
#22875=CARTESIAN_POINT('Ctrl Pts',(14.1008202908092,-16.8567343671546,-1.49520365267535));
#22876=CARTESIAN_POINT('Ctrl Pts',(13.8024087055843,-16.454457921933,-1.47538156930739));
#22877=CARTESIAN_POINT('Ctrl Pts',(13.6952482164322,-16.2319055093249,-1.46644338907454));
#22878=CARTESIAN_POINT('Ctrl Pts',(13.5679372308721,-15.7518323297933,-1.44573697721874));
#22879=CARTESIAN_POINT('Ctrl Pts',(13.5515962723608,-15.4981347275301,-1.43479454747415));
#22880=CARTESIAN_POINT('Ctrl Pts',(13.6177050294595,-14.9946779887315,-1.41307956103122));
#22881=CARTESIAN_POINT('Ctrl Pts',(13.7011232772003,-14.7500889892398,-1.4025630039161));
#22882=CARTESIAN_POINT('Ctrl Pts',(13.9530518157521,-14.3167686917903,-1.38380772364012));
#22883=CARTESIAN_POINT('Ctrl Pts',(14.1156697545305,-14.1300765218334,-1.37370723711989));
#22884=CARTESIAN_POINT('Ctrl Pts',(14.5094994028657,-13.8216873535972,-1.35234574472332));
#22885=CARTESIAN_POINT('Ctrl Pts',(14.7392900935943,-13.7058009544623,-1.34126312922332));
#22886=CARTESIAN_POINT('Ctrl Pts',(15.1530393767014,-13.5913602763721,-1.32334024636833));
#22887=CARTESIAN_POINT('Ctrl Pts',(15.3262907155804,-13.5679367061317,-1.31636360097141));
#22888=CARTESIAN_POINT('Ctrl Pts',(15.5000000000001,-13.5679367061317,-1.30987500000019));
#22889=CARTESIAN_POINT('Origin',(-15.5,-15.5000000000001,11.20575));
#22890=CARTESIAN_POINT('',(-13.5679367061318,-15.5000000000001,1.22137499999992));
#22891=CARTESIAN_POINT('',(-13.5679367061318,-15.5000000000001,1.38580000000001));
#22892=CARTESIAN_POINT('',(-13.5679367061318,-15.5000000000001,11.20575));
#22893=CARTESIAN_POINT('',(-16.4140591443297,-17.2021646372136,1.3857999999999));
#22894=CARTESIAN_POINT('Origin',(-15.5,-15.5000000000001,1.3858));
#22895=CARTESIAN_POINT('Ctrl Pts',(-16.4140591443298,-17.2021646372136,
1.38579999999988));
#22896=CARTESIAN_POINT('Ctrl Pts',(-16.2625891374719,-17.2835037402787,
1.37926682864284));
#22897=CARTESIAN_POINT('Ctrl Pts',(-16.1009499216563,-17.3442553078355,
1.37229504117912));
#22898=CARTESIAN_POINT('Ctrl Pts',(-15.7606791262596,-17.4225866712077,
1.35761855531741));
#22899=CARTESIAN_POINT('Ctrl Pts',(-15.5832774889169,-17.4383898562165,
1.34996690652036));
#22900=CARTESIAN_POINT('Ctrl Pts',(-15.1505459516663,-17.4173618064992,
1.33130242407199));
#22901=CARTESIAN_POINT('Ctrl Pts',(-14.8998465928292,-17.3542469088622,
1.32048931391007));
#22902=CARTESIAN_POINT('Ctrl Pts',(-14.4480453995349,-17.138910231798,1.30100232320917));
#22903=CARTESIAN_POINT('Ctrl Pts',(-14.2493134353814,-16.9927945766542,
1.29183017935079));
#22904=CARTESIAN_POINT('Ctrl Pts',(-13.9112799545244,-16.6281426358706,
1.27091926224018));
#22905=CARTESIAN_POINT('Ctrl Pts',(-13.7774947327411,-16.4108843720761,
1.25991876916933));
#22906=CARTESIAN_POINT('Ctrl Pts',(-13.608962253005,-15.9581594812378,1.23937348399107));
#22907=CARTESIAN_POINT('Ctrl Pts',(-13.5679367061318,-15.7298816358067,
1.22996181912328));
#22908=CARTESIAN_POINT('Ctrl Pts',(-13.5679367061318,-15.5000000000001,
1.22137499999992));
#22909=CARTESIAN_POINT('Origin',(-15.5,-15.5000000000001,11.20575));
#22910=CARTESIAN_POINT('',(-13.5679367061318,-15.5000000000001,0.721374999999908));
#22911=CARTESIAN_POINT('',(-13.5679367061318,-15.5000000000001,1.19012499999982));
#22912=CARTESIAN_POINT('',(-13.5679367061318,-15.5000000000001,11.20575));
#22913=CARTESIAN_POINT('',(-17.0070594673502,-16.7089831815964,1.3858));
#22914=CARTESIAN_POINT('Ctrl Pts',(-13.5679367061318,-15.5000000000001,
1.19012499999982));
#22915=CARTESIAN_POINT('Ctrl Pts',(-13.5679367061318,-15.6209597157623,
1.19464323477233));
#22916=CARTESIAN_POINT('Ctrl Pts',(-13.5792946957064,-15.7419184750203,
1.19940637898297));
#22917=CARTESIAN_POINT('Ctrl Pts',(-13.650067406739,-16.1137167329617,1.21482051737718));
#22918=CARTESIAN_POINT('Ctrl Pts',(-13.7479960405404,-16.3540308512713,
1.22590894156169));
#22919=CARTESIAN_POINT('Ctrl Pts',(-14.0267023405018,-16.7741136008829,
1.24761093429803));
#22920=CARTESIAN_POINT('Ctrl Pts',(-14.201640121497,-16.9519823816315,1.25802759498804));
#22921=CARTESIAN_POINT('Ctrl Pts',(-14.6147032779422,-17.2359894885839,
1.2775442497622));
#22922=CARTESIAN_POINT('Ctrl Pts',(-14.8503902891224,-17.3372359040124,
1.28710617538626));
#22923=CARTESIAN_POINT('Ctrl Pts',(-15.3471703745481,-17.4426537117391,
1.30853318586959));
#22924=CARTESIAN_POINT('Ctrl Pts',(-15.6033601229594,-17.4459126157984,
1.31958310631925));
#22925=CARTESIAN_POINT('Ctrl Pts',(-16.0780162130539,-17.3577451237209,
1.34005586945288));
#22926=CARTESIAN_POINT('Ctrl Pts',(-16.2939169603254,-17.2762244544319,
1.3492321587465));
#22927=CARTESIAN_POINT('Ctrl Pts',(-16.6881081787936,-17.0408604404304,
1.36652484724902));
#22928=CARTESIAN_POINT('Ctrl Pts',(-16.8630519069466,-16.8884959825849,
1.37598896763183));
#22929=CARTESIAN_POINT('Ctrl Pts',(-17.0070594673503,-16.7089831815965,
1.38580000000001));
#22930=CARTESIAN_POINT('Origin',(-15.5,-15.5000000000001,1.3858));
#22931=CARTESIAN_POINT('Ctrl Pts',(-13.5679367061318,-15.5000000000001,
1.22137499999992));
#22932=CARTESIAN_POINT('Ctrl Pts',(-13.5679367061318,-15.4729341635697,
1.22036400387996));
#22933=CARTESIAN_POINT('Ctrl Pts',(-13.5685054395976,-15.4458469974684,
1.21933994578423));
#22934=CARTESIAN_POINT('Ctrl Pts',(-13.5800041738663,-15.1726369382998,
1.20888669011567));
#22935=CARTESIAN_POINT('Ctrl Pts',(-13.6373364197397,-14.9307787640132,
1.1986160877525));
#22936=CARTESIAN_POINT('Ctrl Pts',(-13.8436681825557,-14.4729009295844,
1.177063148319));
#22937=CARTESIAN_POINT('Ctrl Pts',(-13.9941383694055,-14.2627623228301,
1.16596877121766));
#22938=CARTESIAN_POINT('Ctrl Pts',(-14.3628583039267,-13.9183617243244,
1.14515252621433));
#22939=CARTESIAN_POINT('Ctrl Pts',(-14.5755603827482,-13.7853340429807,
1.13624772829804));
#22940=CARTESIAN_POINT('Ctrl Pts',(-15.0402511773768,-13.6069662799091,
1.11620478611874));
#22941=CARTESIAN_POINT('Ctrl Pts',(-15.2879321569902,-13.5635189852138,
1.10552186403231));
#22942=CARTESIAN_POINT('Ctrl Pts',(-15.7929752643667,-13.5731954042506,
1.08373845468527));
#22943=CARTESIAN_POINT('Ctrl Pts',(-16.0454493147401,-13.6289269314741,
1.07284879891439));
#22944=CARTESIAN_POINT('Ctrl Pts',(-16.5036338509587,-13.831024509948,1.05308648325627));
#22945=CARTESIAN_POINT('Ctrl Pts',(-16.7067442551307,-13.9714260900016,
1.0441143076934));
#22946=CARTESIAN_POINT('Ctrl Pts',(-17.0548537166298,-14.3257784407275,
1.02337081592583));
#22947=CARTESIAN_POINT('Ctrl Pts',(-17.1945806685306,-14.5383567471224,
1.01241699562448));
#22948=CARTESIAN_POINT('Ctrl Pts',(-17.3860429607487,-15.0088443364473,
0.99071371463696));
#22949=CARTESIAN_POINT('Ctrl Pts',(-17.4344332047526,-15.2627143707624,
0.980289491352765));
#22950=CARTESIAN_POINT('Ctrl Pts',(-17.4296140643915,-15.7641076910023,
0.961456907719596));
#22951=CARTESIAN_POINT('Ctrl Pts',(-17.3804673297517,-16.0069337844365,
0.951326678304535));
#22952=CARTESIAN_POINT('Ctrl Pts',(-17.1903012302114,-16.4699471303935,
0.929930537917788));
#22953=CARTESIAN_POINT('Ctrl Pts',(-17.0476412720934,-16.6843681047608,
0.918844635143063));
#22954=CARTESIAN_POINT('Ctrl Pts',(-16.6904570707359,-17.0422253710005,
0.897774518646293));
#22955=CARTESIAN_POINT('Ctrl Pts',(-16.4806668477673,-17.1834288056111,
0.888672908962502));
#22956=CARTESIAN_POINT('Ctrl Pts',(-16.0208578479742,-17.377035015047,0.868840527295173));
#22957=CARTESIAN_POINT('Ctrl Pts',(-15.7755220878932,-17.4283735116763,
0.858258758707007));
#22958=CARTESIAN_POINT('Ctrl Pts',(-15.2690019280109,-17.4355092605755,
0.836411641452892));
#22959=CARTESIAN_POINT('Ctrl Pts',(-15.0126438261503,-17.3873412234668,
0.82535445961893));
#22960=CARTESIAN_POINT('Ctrl Pts',(-14.5460700123029,-17.1979533837254,
0.805230299464693));
#22961=CARTESIAN_POINT('Ctrl Pts',(-14.3384565929788,-17.0632817898192,
0.796385555304599));
#22962=CARTESIAN_POINT('Ctrl Pts',(-13.9803614870582,-16.7193021670802,
0.775814168998308));
#22963=CARTESIAN_POINT('Ctrl Pts',(-13.8348471763986,-16.5115619835562,
0.764916258611936));
#22964=CARTESIAN_POINT('Ctrl Pts',(-13.6296318244408,-16.0477927710948,
0.743167333638657));
#22965=CARTESIAN_POINT('Ctrl Pts',(-13.5735885358348,-15.7954972626707,
0.732534660758096));
#22966=CARTESIAN_POINT('Ctrl Pts',(-13.5680718804938,-15.526395610973,0.722363876197133));
#22967=CARTESIAN_POINT('Ctrl Pts',(-13.5679367061318,-15.5131950983567,
0.721867879400674));
#22968=CARTESIAN_POINT('Ctrl Pts',(-13.5679367061318,-15.5000000000001,
0.72137499999991));
#22969=CARTESIAN_POINT('Origin',(-15.5,-15.5000000000001,11.20575));
#22970=CARTESIAN_POINT('',(-13.5679367061318,-15.5000000000002,0.221374999999906));
#22971=CARTESIAN_POINT('',(-13.5679367061318,-15.5000000000001,0.690124999999812));
#22972=CARTESIAN_POINT('',(-13.5679367061318,-15.5000000000001,11.20575));
#22973=CARTESIAN_POINT('Ctrl Pts',(-13.5679367061318,-15.5,0.690124999999811));
#22974=CARTESIAN_POINT('Ctrl Pts',(-13.5679367061318,-15.6631976348033,
0.696220957019171));
#22975=CARTESIAN_POINT('Ctrl Pts',(-13.5886111528804,-15.8260698424813,
0.702750621155628));
#22976=CARTESIAN_POINT('Ctrl Pts',(-13.6937750358448,-16.231840773596,0.720175424526339));
#22977=CARTESIAN_POINT('Ctrl Pts',(-13.8061679673988,-16.4638288993586,
0.731264781557226));
#22978=CARTESIAN_POINT('Ctrl Pts',(-14.1088337976827,-16.8630470507194,
0.75270412300504));
#22979=CARTESIAN_POINT('Ctrl Pts',(-14.2932884830906,-17.0287614441965,
0.762872018728063));
#22980=CARTESIAN_POINT('Ctrl Pts',(-14.723125143869,-17.287405358774,0.781803012187269));
#22981=CARTESIAN_POINT('Ctrl Pts',(-14.9664736216109,-17.3745003706307,
0.79211305640894));
#22982=CARTESIAN_POINT('Ctrl Pts',(-15.4692792372012,-17.4482099203794,
0.813799958747424));
#22983=CARTESIAN_POINT('Ctrl Pts',(-15.7235658751718,-17.4355847239786,
0.824767794651914));
#22984=CARTESIAN_POINT('Ctrl Pts',(-16.2055976541623,-17.315173374422,0.845558684393136));
#22985=CARTESIAN_POINT('Ctrl Pts',(-16.4295122772784,-17.211349687416,0.854579673980957));
#22986=CARTESIAN_POINT('Ctrl Pts',(-16.835971896653,-16.9190154733783,0.874264961849451));
#22987=CARTESIAN_POINT('Ctrl Pts',(-17.0120418978356,-16.7296891979227,
0.885134014187586));
#22988=CARTESIAN_POINT('Ctrl Pts',(-17.2766178136157,-16.2991617620676,
0.906921415251255));
#22989=CARTESIAN_POINT('Ctrl Pts',(-17.3648212635819,-16.0634585876007,
0.917627873583991));
#22990=CARTESIAN_POINT('Ctrl Pts',(-17.4465792698413,-15.5727030691466,
0.937722356281882));
#22991=CARTESIAN_POINT('Ctrl Pts',(-17.4398199793546,-15.3223565583369,
0.946593274573956));
#22992=CARTESIAN_POINT('Ctrl Pts',(-17.3302144103325,-14.8300711076976,
0.96734546267104));
#22993=CARTESIAN_POINT('Ctrl Pts',(-17.2253688342262,-14.5935881752461,
0.978439949755289));
#22994=CARTESIAN_POINT('Ctrl Pts',(-16.9351538432135,-14.183201533444,1.00002795682994));
#22995=CARTESIAN_POINT('Ctrl Pts',(-16.7556158303762,-14.0110153602741,
1.01033156193276));
#22996=CARTESIAN_POINT('Ctrl Pts',(-16.3329965553288,-13.7379425524705,
1.02964587164789));
#22997=CARTESIAN_POINT('Ctrl Pts',(-16.0918227958039,-13.6429845085469,
1.03959862802553));
#22998=CARTESIAN_POINT('Ctrl Pts',(-15.5900949475545,-13.553533331627,1.06123904433771));
#22999=CARTESIAN_POINT('Ctrl Pts',(-15.3347633934771,-13.5584675814189,
1.0722519493362));
#23000=CARTESIAN_POINT('Ctrl Pts',(-14.8487842127037,-13.6646353766638,
1.09321309755167));
#23001=CARTESIAN_POINT('Ctrl Pts',(-14.6220240391682,-13.7616722786086,
1.10246053097514));
#23002=CARTESIAN_POINT('Ctrl Pts',(-14.2071591450865,-14.0415852702359,
1.12186311344));
#23003=CARTESIAN_POINT('Ctrl Pts',(-14.0255156909762,-14.2255255819053,
1.13265117917154));
#23004=CARTESIAN_POINT('Ctrl Pts',(-13.7477641930796,-14.6484954207351,
1.1544404228268));
#23005=CARTESIAN_POINT('Ctrl Pts',(-13.6523788496883,-14.8821830754006,
1.16522647893844));
#23006=CARTESIAN_POINT('Ctrl Pts',(-13.5800170676888,-15.2505243179923,
1.18054575641213));
#23007=CARTESIAN_POINT('Ctrl Pts',(-13.5679367061318,-15.3752528162567,
1.18546529110573));
#23008=CARTESIAN_POINT('Ctrl Pts',(-13.5679367061318,-15.5000000000001,
1.19012499999982));
#23009=CARTESIAN_POINT('Ctrl Pts',(-13.5679367061318,-15.5000000000001,
0.721374999999909));
#23010=CARTESIAN_POINT('Ctrl Pts',(-13.5679367061318,-15.2685828061803,
0.712730822841552));
#23011=CARTESIAN_POINT('Ctrl Pts',(-13.6095133453597,-15.0388969704722,
0.703254680206819));
#23012=CARTESIAN_POINT('Ctrl Pts',(-13.7800568346783,-14.5838672571245,
0.682579933274515));
#23013=CARTESIAN_POINT('Ctrl Pts',(-13.9154007891409,-14.3657373184651,
0.671513264882122));
#23014=CARTESIAN_POINT('Ctrl Pts',(-14.2617096431742,-13.9955563279968,
0.65021735416984));
#23015=CARTESIAN_POINT('Ctrl Pts',(-14.468832161597,-13.8467023150394,0.64085110669535));
#23016=CARTESIAN_POINT('Ctrl Pts',(-14.9240794296703,-13.6392165647333,
0.621215480647348));
#23017=CARTESIAN_POINT('Ctrl Pts',(-15.1670698902397,-13.5807974419184,
0.610734869007077));
#23018=CARTESIAN_POINT('Ctrl Pts',(-15.6716078303532,-13.5584324818654,
0.588973248424435));
#23019=CARTESIAN_POINT('Ctrl Pts',(-15.9284928593656,-13.5985422788448,
0.577893339283274));
#23020=CARTESIAN_POINT('Ctrl Pts',(-16.4008511615348,-13.7731735264444,
0.55751968383815));
#23021=CARTESIAN_POINT('Ctrl Pts',(-16.6132862462162,-13.9018579856258,
0.548728405588926));
#23022=CARTESIAN_POINT('Ctrl Pts',(-16.9816699619906,-14.2349802270737,
0.52834069438543));
#23023=CARTESIAN_POINT('Ctrl Pts',(-17.1330265348185,-14.4375333643221,
0.517510543285457));
#23024=CARTESIAN_POINT('Ctrl Pts',(-17.3523384611631,-14.8940137705683,
0.495729873499502));
#23025=CARTESIAN_POINT('Ctrl Pts',(-17.4162475186526,-15.1444779572253,
0.484995974066794));
#23026=CARTESIAN_POINT('Ctrl Pts',(-17.4421185607441,-15.6442929464891,
0.465768343155524));
#23027=CARTESIAN_POINT('Ctrl Pts',(-17.4083000036084,-15.8886689111737,
0.456344488448985));
#23028=CARTESIAN_POINT('Ctrl Pts',(-17.2484328204734,-16.3602738343215,
0.43528084812928));
#23029=CARTESIAN_POINT('Ctrl Pts',(-17.1206457356298,-16.581940728719,0.42424503368158));
#23030=CARTESIAN_POINT('Ctrl Pts',(-16.7856687235223,-16.9645889729791,
0.40272781217544));
#23031=CARTESIAN_POINT('Ctrl Pts',(-16.5812682858183,-17.1213576049014,
0.393012028285058));
#23032=CARTESIAN_POINT('Ctrl Pts',(-16.1307300450291,-17.3428309785426,
0.373579510976611));
#23033=CARTESIAN_POINT('Ctrl Pts',(-15.8902976971979,-17.4082697840594,
0.363209235298005));
#23034=CARTESIAN_POINT('Ctrl Pts',(-15.3881980760648,-17.4458200822429,
0.341552783758757));
#23035=CARTESIAN_POINT('Ctrl Pts',(-15.131028168327,-17.4137884812097,0.33046058729045));
#23036=CARTESIAN_POINT('Ctrl Pts',(-14.6530287770869,-17.2540504946331,
0.309843621619741));
#23037=CARTESIAN_POINT('Ctrl Pts',(-14.4356759586665,-17.1313390170145,
0.301024334084349));
#23038=CARTESIAN_POINT('Ctrl Pts',(-14.0571971873737,-16.8090342640234,
0.280822982029637));
#23039=CARTESIAN_POINT('Ctrl Pts',(-13.9002426531824,-16.6117620419649,
0.270069365086781));
#23040=CARTESIAN_POINT('Ctrl Pts',(-13.6672548469476,-16.162904088269,0.248278485904575));
#23041=CARTESIAN_POINT('Ctrl Pts',(-13.5956339333618,-15.9144966791606,
0.237455100685372));
#23042=CARTESIAN_POINT('Ctrl Pts',(-13.5701259723183,-15.6062624042348,
0.225391456350146));
#23043=CARTESIAN_POINT('Ctrl Pts',(-13.5679367061318,-15.5531033071595,
0.223358579470397));
#23044=CARTESIAN_POINT('Ctrl Pts',(-13.5679367061318,-15.5000000000002,
0.221374999999906));
#23045=CARTESIAN_POINT('Origin',(-15.5,-15.5000000000001,11.20575));
#23046=CARTESIAN_POINT('',(-13.5679367061318,-15.5000000000001,-0.278625000000104));
#23047=CARTESIAN_POINT('',(-13.5679367061318,-15.5000000000001,0.190124999999801));
#23048=CARTESIAN_POINT('',(-13.5679367061318,-15.5000000000001,11.20575));
#23049=CARTESIAN_POINT('Ctrl Pts',(-13.5679367061318,-15.5,0.190124999999802));
#23050=CARTESIAN_POINT('Ctrl Pts',(-13.5679367061318,-15.7052232055909,
0.197790747375155));
#23051=CARTESIAN_POINT('Ctrl Pts',(-13.6006312438213,-15.9094431243977,
0.206124105599912));
#23052=CARTESIAN_POINT('Ctrl Pts',(-13.7445092392226,-16.3458500952323,
0.225528168010807));
#23053=CARTESIAN_POINT('Ctrl Pts',(-13.8706006648954,-16.5687690248997,
0.236574181605254));
#23054=CARTESIAN_POINT('Ctrl Pts',(-14.1957983248934,-16.9462938014505,
0.257689124656201));
#23055=CARTESIAN_POINT('Ctrl Pts',(-14.3891741439701,-17.099606802076,0.267213101031626));
#23056=CARTESIAN_POINT('Ctrl Pts',(-14.8328987043056,-17.3312210666003,
0.286351732158258));
#23057=CARTESIAN_POINT('Ctrl Pts',(-15.0810963874241,-17.4033891896781,
0.297056940587791));
#23058=CARTESIAN_POINT('Ctrl Pts',(-15.5859112111092,-17.4463663432178,
0.318830503652362));
#23059=CARTESIAN_POINT('Ctrl Pts',(-15.837491754929,-17.4188098289699,0.329681620893124));
#23060=CARTESIAN_POINT('Ctrl Pts',(-16.3114416099339,-17.2705600347065,
0.350123922848628));
#23061=CARTESIAN_POINT('Ctrl Pts',(-16.529916123996,-17.1530549287719,0.35892246930463));
#23062=CARTESIAN_POINT('Ctrl Pts',(-16.9202726297616,-16.8349526369193,
0.379222999836032));
#23063=CARTESIAN_POINT('Ctrl Pts',(-17.0854512100821,-16.6338441663765,
0.39029727189281));
#23064=CARTESIAN_POINT('Ctrl Pts',(-17.3225641667436,-16.1874197433201,
0.412086213416735));
#23065=CARTESIAN_POINT('Ctrl Pts',(-17.3956324394973,-15.9481982603314,
0.422597688314646));
#23066=CARTESIAN_POINT('Ctrl Pts',(-17.4478128352923,-15.451075784191,0.442292129850996));
#23067=CARTESIAN_POINT('Ctrl Pts',(-17.4248413113893,-15.1977325915623,
0.451571409240311));
#23068=CARTESIAN_POINT('Ctrl Pts',(-17.2822086107981,-14.7117348553562,
0.472800990486158));
#23069=CARTESIAN_POINT('Ctrl Pts',(-17.1630032804558,-14.4841033890508,
0.483874527712175));
#23070=CARTESIAN_POINT('Ctrl Pts',(-16.8491384993424,-14.0954494858791,
0.505160775836539));
#23071=CARTESIAN_POINT('Ctrl Pts',(-16.66030462317,-13.9358452837369,0.515078993620071));
#23072=CARTESIAN_POINT('Ctrl Pts',(-16.2236425461124,-13.6903827463216,
0.533913007255616));
#23073=CARTESIAN_POINT('Ctrl Pts',(-15.9778499407047,-13.6105539996565,
0.54451448039696));
#23074=CARTESIAN_POINT('Ctrl Pts',(-15.4739117712162,-13.5518158441319,
0.566250231803577));
#23075=CARTESIAN_POINT('Ctrl Pts',(-15.2208352901079,-13.5717427947093,
0.577165871485754));
#23076=CARTESIAN_POINT('Ctrl Pts',(-14.7426848689165,-13.7057278794303,
0.597789351347446));
#23077=CARTESIAN_POINT('Ctrl Pts',(-14.5214408844322,-13.8161488953131,
0.60666457334335));
#23078=CARTESIAN_POINT('Ctrl Pts',(-14.1213400688703,-14.1219606735901,
0.626716158351838));
#23079=CARTESIAN_POINT('Ctrl Pts',(-13.9495491173577,-14.3185686119017,
0.637764922719137));
#23080=CARTESIAN_POINT('Ctrl Pts',(-13.6984440207755,-14.7590310485599,
0.659632917824817));
#23081=CARTESIAN_POINT('Ctrl Pts',(-13.6181551918391,-14.9966959458154,
0.670241966963291));
#23082=CARTESIAN_POINT('Ctrl Pts',(-13.5736457522819,-15.3284077888479,
0.683592357862467));
#23083=CARTESIAN_POINT('Ctrl Pts',(-13.5679367061318,-15.4142441778546,
0.686921743980885));
#23084=CARTESIAN_POINT('Ctrl Pts',(-13.5679367061318,-15.5,0.690124999999813));
#23085=CARTESIAN_POINT('Ctrl Pts',(-13.5679367061318,-15.5000000000002,
0.221374999999905));
#23086=CARTESIAN_POINT('Ctrl Pts',(-13.5679367061318,-15.3093450219841,
0.214253422821946));
#23087=CARTESIAN_POINT('Ctrl Pts',(-13.5961535791236,-15.1194546080678,
0.206551882563236));
#23088=CARTESIAN_POINT('Ctrl Pts',(-13.7256105048354,-14.6948718228171,
0.187900494766885));
#23089=CARTESIAN_POINT('Ctrl Pts',(-13.845972474099,-14.4700098899864,0.176905464582649));
#23090=CARTESIAN_POINT('Ctrl Pts',(-14.1696924220725,-14.0753526087545,
0.155182435506234));
#23091=CARTESIAN_POINT('Ctrl Pts',(-14.3714266003534,-13.9107790534924,
0.145052382155262));
#23092=CARTESIAN_POINT('Ctrl Pts',(-14.8173319842844,-13.6758632411833,
0.125819688220126));
#23093=CARTESIAN_POINT('Ctrl Pts',(-15.0551292056848,-13.6037990123402,
0.115563070240994));
#23094=CARTESIAN_POINT('Ctrl Pts',(-15.5544792855134,-13.5518334963291,
0.0940252113186381));
#23095=CARTESIAN_POINT('Ctrl Pts',(-15.8116932976136,-13.5761558232251,
0.0829311125505648));
#23096=CARTESIAN_POINT('Ctrl Pts',(-16.2949297861469,-13.7215598038885,
0.0620882615396313));
#23097=CARTESIAN_POINT('Ctrl Pts',(-16.5170608749109,-13.8385708543143,
0.0531675695570689));
#23098=CARTESIAN_POINT('Ctrl Pts',(-16.904996700699,-14.1505967904306,0.0331462145940504));
#23099=CARTESIAN_POINT('Ctrl Pts',(-17.0670614606798,-14.3427581395106,
0.0224732986365848));
#23100=CARTESIAN_POINT('Ctrl Pts',(-17.3126898339284,-14.7840616511319,
0.000691997092672782));
#23101=CARTESIAN_POINT('Ctrl Pts',(-17.3915129004033,-15.0303088815555,
-0.0102060193438629));
#23102=CARTESIAN_POINT('Ctrl Pts',(-17.4473055261676,-15.5280187234508,
-0.030000301840267));
#23103=CARTESIAN_POINT('Ctrl Pts',(-17.4281050083167,-15.7742335763025,
-0.0389538708323471));
#23104=CARTESIAN_POINT('Ctrl Pts',(-17.2969077105388,-16.2532901710004,
-0.0596775634460382));
#23105=CARTESIAN_POINT('Ctrl Pts',(-17.1834947936056,-16.4808992970974,
-0.0706253476363654));
#23106=CARTESIAN_POINT('Ctrl Pts',(-16.8732369844076,-16.882970778423,-0.092334997934469));
#23107=CARTESIAN_POINT('Ctrl Pts',(-16.6781753239889,-17.0524923786021,
-0.102808198443676));
#23108=CARTESIAN_POINT('Ctrl Pts',(-16.2425026231762,-17.3005030647046,
-0.121599538518457));
#23109=CARTESIAN_POINT('Ctrl Pts',(-16.0080032116997,-17.3801675178151,
-0.131713916077958));
#23110=CARTESIAN_POINT('Ctrl Pts',(-15.5123656482203,-17.448772467442,-0.153091647553434));
#23111=CARTESIAN_POINT('Ctrl Pts',(-15.2553808902943,-17.4333995515062,
-0.164175858180371));
#23112=CARTESIAN_POINT('Ctrl Pts',(-14.7662503095724,-17.3048200985618,
-0.185272931892274));
#23113=CARTESIAN_POINT('Ctrl Pts',(-14.5384527979055,-17.1944566841175,
-0.194401543736984));
#23114=CARTESIAN_POINT('Ctrl Pts',(-14.1397272750994,-16.8943347846072,
-0.214210934043039));
#23115=CARTESIAN_POINT('Ctrl Pts',(-13.9720032632392,-16.7081889662025,
-0.224781197374756));
#23116=CARTESIAN_POINT('Ctrl Pts',(-13.7111048247492,-16.2741834166746,
-0.246619209105808));
#23117=CARTESIAN_POINT('Ctrl Pts',(-13.6237773095579,-16.0284985545294,
-0.257679625291989));
#23118=CARTESIAN_POINT('Ctrl Pts',(-13.5743830168529,-15.6823226735556,
-0.271675640781532));
#23119=CARTESIAN_POINT('Ctrl Pts',(-13.5679367061318,-15.5911253192395,
-0.275221175979445));
#23120=CARTESIAN_POINT('Ctrl Pts',(-13.5679367061318,-15.5000000000001,
-0.278625000000103));
#23121=CARTESIAN_POINT('Origin',(-15.5,-15.5000000000001,11.20575));
#23122=CARTESIAN_POINT('',(-13.5679367061318,-15.5000000000001,-0.778625000000111));
#23123=CARTESIAN_POINT('',(-13.5679367061318,-15.5000000000214,-0.30987499999861));
#23124=CARTESIAN_POINT('',(-13.5679367061318,-15.5000000000001,11.20575));
#23125=CARTESIAN_POINT('Ctrl Pts',(-13.5679367061318,-15.5000000000426,
-0.309874999998611));
#23126=CARTESIAN_POINT('Ctrl Pts',(-13.5679367061372,-15.7451189900435,
-0.30071901664447));
#23127=CARTESIAN_POINT('Ctrl Pts',(-13.614584910455,-15.9880788836298,-0.290637672395915));
#23128=CARTESIAN_POINT('Ctrl Pts',(-13.7998506160078,-16.4525087353532,
-0.269294302322098));
#23129=CARTESIAN_POINT('Ctrl Pts',(-13.9401358945745,-16.6681650113367,
-0.25821346913606));
#23130=CARTESIAN_POINT('Ctrl Pts',(-14.2937988135869,-17.0300510391149,
-0.237068805018314));
#23131=CARTESIAN_POINT('Ctrl Pts',(-14.5027181075032,-17.1737375672253,
-0.227889545454481));
#23132=CARTESIAN_POINT('Ctrl Pts',(-14.9610456268796,-17.3718881645073,
-0.20812106267792));
#23133=CARTESIAN_POINT('Ctrl Pts',(-15.205635116172,-17.4255568606796,-0.19757148207894));
#23134=CARTESIAN_POINT('Ctrl Pts',(-15.7028273877143,-17.437485526191,-0.176126693273804));
#23135=CARTESIAN_POINT('Ctrl Pts',(-15.950828380533,-17.3951930471992,-0.165429968447499));
#23136=CARTESIAN_POINT('Ctrl Pts',(-16.4162168450069,-17.21903750586,-0.145356934524352));
#23137=CARTESIAN_POINT('Ctrl Pts',(-16.6293413959127,-17.0871779138879,
-0.136472617530252));
#23138=CARTESIAN_POINT('Ctrl Pts',(-16.9997020048591,-16.7447233478946,
-0.115693680499808));
#23139=CARTESIAN_POINT('Ctrl Pts',(-17.1512859841672,-16.5352235199722,
-0.104599143917264));
#23140=CARTESIAN_POINT('Ctrl Pts',(-17.3599329092897,-16.0781299074099,
-0.083025569156745));
#23141=CARTESIAN_POINT('Ctrl Pts',(-17.4184418092007,-15.8364334516317,
-0.07273563190757));
#23142=CARTESIAN_POINT('Ctrl Pts',(-17.4419572678445,-15.3335771418076,
-0.0534451981390733));
#23143=CARTESIAN_POINT('Ctrl Pts',(-17.4026393126746,-15.0770448720175,
-0.0434417100341766));
#23144=CARTESIAN_POINT('Ctrl Pts',(-17.2273302215969,-14.5982616364446,
-0.0217769181316164));
#23145=CARTESIAN_POINT('Ctrl Pts',(-17.0946215718083,-14.3801849192583,
-0.0107690704262966));
#23146=CARTESIAN_POINT('Ctrl Pts',(-16.7583973031523,-14.0137016048738,
0.0101712371104099));
#23147=CARTESIAN_POINT('Ctrl Pts',(-16.5604348396371,-13.8665662971671,
0.0193865553792948));
#23148=CARTESIAN_POINT('Ctrl Pts',(-16.1097762694872,-13.6488960345413,
0.0388242627075219));
#23149=CARTESIAN_POINT('Ctrl Pts',(-15.8594139033153,-13.5844810246989,
0.0496228377751917));
#23150=CARTESIAN_POINT('Ctrl Pts',(-15.3542160204943,-13.557297522928,0.0714129228629977));
#23151=CARTESIAN_POINT('Ctrl Pts',(-15.1043600205154,-13.5924291711368,
0.0821896574542814));
#23152=CARTESIAN_POINT('Ctrl Pts',(-14.6347353821394,-13.7549549306401,
0.102445405107847));
#23153=CARTESIAN_POINT('Ctrl Pts',(-14.4190031858112,-13.8797188217568,
0.111248274994699));
#23154=CARTESIAN_POINT('Ctrl Pts',(-14.0387180251795,-14.2102312356741,
0.131795166002626));
#23155=CARTESIAN_POINT('Ctrl Pts',(-13.8803875205859,-14.4157066951989,
0.1428848743003));
#23156=CARTESIAN_POINT('Ctrl Pts',(-13.6576628179058,-14.8677637645241,
0.164573917775743));
#23157=CARTESIAN_POINT('Ctrl Pts',(-13.5919750720436,-15.1083498919248,
0.174977198895978));
#23158=CARTESIAN_POINT('Ctrl Pts',(-13.5697540327492,-15.4031822744542,
0.186469354010744));
#23159=CARTESIAN_POINT('Ctrl Pts',(-13.5679367061318,-15.4516175612206,
0.188317760160533));
#23160=CARTESIAN_POINT('Ctrl Pts',(-13.5679367061318,-15.5,0.190124999999802));
#23161=CARTESIAN_POINT('Ctrl Pts',(-13.5679367061318,-15.5000000000001,
-0.278625000000104));
#23162=CARTESIAN_POINT('Ctrl Pts',(-13.5679367061318,-15.3467892595674,
-0.284347914365298));
#23163=CARTESIAN_POINT('Ctrl Pts',(-13.5861582264615,-15.1938118278,-0.290455077224571));
#23164=CARTESIAN_POINT('Ctrl Pts',(-13.6816903722921,-14.8002115586198,
-0.307217550198197));
#23165=CARTESIAN_POINT('Ctrl Pts',(-13.7879612606778,-14.570016446838,-0.31810790506839));
#23166=CARTESIAN_POINT('Ctrl Pts',(-14.0854112713272,-14.1593674320811,
-0.339861742263403));
#23167=CARTESIAN_POINT('Ctrl Pts',(-14.2752366149402,-13.9839732653664,
-0.350507031707781));
#23168=CARTESIAN_POINT('Ctrl Pts',(-14.702688554669,-13.7231840671468,-0.369466729782478));
#23169=CARTESIAN_POINT('Ctrl Pts',(-14.9340075270615,-13.6365422674356,
-0.379212735887829));
#23170=CARTESIAN_POINT('Ctrl Pts',(-15.4259040929271,-13.5527035685258,
-0.400429111468748));
#23171=CARTESIAN_POINT('Ctrl Pts',(-15.6824101509155,-13.5598498556791,
-0.4114926748787));
#23172=CARTESIAN_POINT('Ctrl Pts',(-16.1685436048833,-13.6708737218792,
-0.432460477172683));
#23173=CARTESIAN_POINT('Ctrl Pts',(-16.3943923195072,-13.7700581638794,
-0.441627804189991));
#23174=CARTESIAN_POINT('Ctrl Pts',(-16.8066128739237,-14.0539091259065,
-0.461120454984909));
#23175=CARTESIAN_POINT('Ctrl Pts',(-16.986511157224,-14.2395717541843,-0.471935218622489));
#23176=CARTESIAN_POINT('Ctrl Pts',(-17.2601171116814,-14.6649766986924,
-0.493726018975322));
#23177=CARTESIAN_POINT('Ctrl Pts',(-17.3532344935945,-14.899325305048,-0.504487853149966));
#23178=CARTESIAN_POINT('Ctrl Pts',(-17.4445879149158,-15.3879151902704,
-0.524708376151779));
#23179=CARTESIAN_POINT('Ctrl Pts',(-17.4429655287095,-15.6373703519541,
-0.533521108453184));
#23180=CARTESIAN_POINT('Ctrl Pts',(-17.3439130071985,-16.1314699148968,
-0.554113473610937));
#23181=CARTESIAN_POINT('Ctrl Pts',(-17.2437932710759,-16.370599259013,-0.56520489573948));
#23182=CARTESIAN_POINT('Ctrl Pts',(-16.9614315558214,-16.7876645309164,
-0.586873008257939));
#23183=CARTESIAN_POINT('Ctrl Pts',(-16.7850271271049,-16.9637580970129,
-0.597254988531082));
#23184=CARTESIAN_POINT('Ctrl Pts',(-16.368955630774,-17.2443400456584,-0.616708580146808));
#23185=CARTESIAN_POINT('Ctrl Pts',(-16.131560971349,-17.3436265739668,-0.62638464969034));
#23186=CARTESIAN_POINT('Ctrl Pts',(-15.6332086940277,-17.4440644805447,
-0.647879471612186));
#23187=CARTESIAN_POINT('Ctrl Pts',(-15.3772600495196,-17.4447534368068,
-0.658918992820774));
#23188=CARTESIAN_POINT('Ctrl Pts',(-14.8884838631652,-17.3489811387507,
-0.680000780871976));
#23189=CARTESIAN_POINT('Ctrl Pts',(-14.6596166089138,-17.2568181637342,
-0.689459136163638));
#23190=CARTESIAN_POINT('Ctrl Pts',(-14.2388050986946,-16.9858620064432,
-0.708655396108797));
#23191=CARTESIAN_POINT('Ctrl Pts',(-14.0532686227974,-16.8058878838003,
-0.719379268396446));
#23192=CARTESIAN_POINT('Ctrl Pts',(-13.7662002684568,-16.3885881549385,
-0.741157641503204));
#23193=CARTESIAN_POINT('Ctrl Pts',(-13.6656892248834,-16.1564785080748,
-0.75199529423572));
#23194=CARTESIAN_POINT('Ctrl Pts',(-13.5827427724808,-15.7761115114099,
-0.767992040186503));
#23195=CARTESIAN_POINT('Ctrl Pts',(-13.5679367061318,-15.6381065098838,
-0.773466277268877));
#23196=CARTESIAN_POINT('Ctrl Pts',(-13.5679367061318,-15.5000000000001,
-0.778625000000112));
#23197=CARTESIAN_POINT('Origin',(-15.5,-15.5000000000001,11.20575));
#23198=CARTESIAN_POINT('',(-13.5679367061318,-15.5000000000001,-1.27862500000012));
#23199=CARTESIAN_POINT('',(-13.5679367061318,-15.5000000000001,-0.809875000000204));
#23200=CARTESIAN_POINT('',(-13.5679367061318,-15.5000000000001,11.20575));
#23201=CARTESIAN_POINT('Ctrl Pts',(-13.5679367061318,-15.5000000000002,
-0.809875000000203));
#23202=CARTESIAN_POINT('Ctrl Pts',(-13.5679367061318,-15.5387848588903,
-0.808426260665952));
#23203=CARTESIAN_POINT('Ctrl Pts',(-13.5691045537611,-15.5776081217819,
-0.806950901143784));
#23204=CARTESIAN_POINT('Ctrl Pts',(-13.5863172258655,-15.8627498107997,
-0.795928734529179));
#23205=CARTESIAN_POINT('Ctrl Pts',(-13.6482441649587,-16.1039441624044,
-0.785583839426325));
#23206=CARTESIAN_POINT('Ctrl Pts',(-13.8636040208235,-16.5586938389716,
-0.763953047887124));
#23207=CARTESIAN_POINT('Ctrl Pts',(-14.0184106751405,-16.7663048606793,
-0.752859564438659));
#23208=CARTESIAN_POINT('Ctrl Pts',(-14.3935142993233,-17.1030886658291,
-0.732190161230552));
#23209=CARTESIAN_POINT('Ctrl Pts',(-14.6078734364707,-17.2315636886461,
-0.723354008700389));
#23210=CARTESIAN_POINT('Ctrl Pts',(-15.0752831240916,-17.401259102443,-0.703193795820516));
#23211=CARTESIAN_POINT('Ctrl Pts',(-15.3241884796656,-17.4401670421017,
-0.692458064216716));
#23212=CARTESIAN_POINT('Ctrl Pts',(-15.8293918059364,-17.4209116308134,
-0.670667744343207));
#23213=CARTESIAN_POINT('Ctrl Pts',(-16.0807480284637,-17.3604173282468,
-0.659826302479602));
#23214=CARTESIAN_POINT('Ctrl Pts',(-16.5348352725855,-17.1497816929782,
-0.640240710332132));
#23215=CARTESIAN_POINT('Ctrl Pts',(-16.7351193667876,-17.0057085011961,
-0.631148276498325));
#23216=CARTESIAN_POINT('Ctrl Pts',(-17.0767669839639,-16.6447314320374,
-0.610296685602489));
#23217=CARTESIAN_POINT('Ctrl Pts',(-17.2126942752493,-16.4291281586244,
-0.599311816112374));
#23218=CARTESIAN_POINT('Ctrl Pts',(-17.3960714153678,-15.9522914740598,
-0.577545739488913));
#23219=CARTESIAN_POINT('Ctrl Pts',(-17.4394863853225,-15.6949512567246,
-0.567317142600478));
#23220=CARTESIAN_POINT('Ctrl Pts',(-17.4229690903241,-15.1907605692907,
-0.548127787168025));
#23221=CARTESIAN_POINT('Ctrl Pts',(-17.367985737015,-14.9485965706548,-0.537896417242245));
#23222=CARTESIAN_POINT('Ctrl Pts',(-17.1662821041941,-14.4891878782664,
-0.516386105083534));
#23223=CARTESIAN_POINT('Ctrl Pts',(-17.0180420352629,-14.2777915836234,
-0.505292843771123));
#23224=CARTESIAN_POINT('Ctrl Pts',(-16.6526099917287,-13.9295152530064,
-0.484402733995946));
#23225=CARTESIAN_POINT('Ctrl Pts',(-16.4407479085027,-13.7941507738711,
-0.475451133965726));
#23226=CARTESIAN_POINT('Ctrl Pts',(-15.977452801173,-13.6113838875222,-0.45546839026715));
#23227=CARTESIAN_POINT('Ctrl Pts',(-15.7304237057036,-13.5656468617911,
-0.444813585105682));
#23228=CARTESIAN_POINT('Ctrl Pts',(-15.2255315160609,-13.5704710073907,
-0.423036685109488));
#23229=CARTESIAN_POINT('Ctrl Pts',(-14.9725259783181,-13.6237792291611,
-0.412124105341109));
#23230=CARTESIAN_POINT('Ctrl Pts',(-14.5122846645609,-13.8215336428728,
-0.392273077202022));
#23231=CARTESIAN_POINT('Ctrl Pts',(-14.3077326406348,-13.9600852553974,
-0.383350131532138));
#23232=CARTESIAN_POINT('Ctrl Pts',(-13.9563854884099,-14.311092329695,-0.362661772922435));
#23233=CARTESIAN_POINT('Ctrl Pts',(-13.8147703346551,-14.5221235135244,
-0.351725021873736));
#23234=CARTESIAN_POINT('Ctrl Pts',(-13.6188695990396,-14.9904064163149,
-0.330008374038385));
#23235=CARTESIAN_POINT('Ctrl Pts',(-13.5679791180276,-15.2437584839142,
-0.319447360159011));
#23236=CARTESIAN_POINT('Ctrl Pts',(-13.5679367149643,-15.4997866765026,
-0.309882968510016));
#23237=CARTESIAN_POINT('Ctrl Pts',(-13.5679367061318,-15.4998933384699,
-0.30987898415171));
#23238=CARTESIAN_POINT('Ctrl Pts',(-13.5679367061318,-15.5000000000426,
-0.309874999998609));
#23239=CARTESIAN_POINT('Ctrl Pts',(-13.5679367061318,-15.5000000000001,
-0.778625000000111));
#23240=CARTESIAN_POINT('Ctrl Pts',(-13.5679367061318,-15.3931460598282,
-0.78261633864556));
#23241=CARTESIAN_POINT('Ctrl Pts',(-13.5768002208838,-15.2862458062684,
-0.786800556839377));
#23242=CARTESIAN_POINT('Ctrl Pts',(-13.6371564582819,-14.9264097344303,
-0.801543228537963));
#23243=CARTESIAN_POINT('Ctrl Pts',(-13.7301105174323,-14.6835020771365,
-0.812621248617171));
#23244=CARTESIAN_POINT('Ctrl Pts',(-14.0004851886932,-14.2567488542947,
-0.834392726004424));
#23245=CARTESIAN_POINT('Ctrl Pts',(-14.1720617651617,-14.0749328108105,
-0.844884342293561));
#23246=CARTESIAN_POINT('Ctrl Pts',(-14.5783544246733,-13.7832732834677,
-0.864540827803848));
#23247=CARTESIAN_POINT('Ctrl Pts',(-14.8102645191385,-13.6776776438874,
-0.873875479411993));
#23248=CARTESIAN_POINT('Ctrl Pts',(-15.303462333774,-13.5612057991406,-0.895147980171542));
#23249=CARTESIAN_POINT('Ctrl Pts',(-15.5600993610212,-13.5521973966285,
-0.906217192554563));
#23250=CARTESIAN_POINT('Ctrl Pts',(-16.0528776436279,-13.6325934594164,
-0.927471598149985));
#23251=CARTESIAN_POINT('Ctrl Pts',(-16.2849105088377,-13.7176559738657,
-0.937309340891435));
#23252=CARTESIAN_POINT('Ctrl Pts',(-16.7142424070008,-13.9755352342243,
-0.956200886398405));
#23253=CARTESIAN_POINT('Ctrl Pts',(-16.9052695296546,-14.1496041206411,
-0.96682258979334));
#23254=CARTESIAN_POINT('Ctrl Pts',(-17.2056519899816,-14.5583089440343,
-0.988567046072784));
#23255=CARTESIAN_POINT('Ctrl Pts',(-17.3135593943002,-14.7879324233922,
-0.99947134155624));
#23256=CARTESIAN_POINT('Ctrl Pts',(-17.4338950578804,-15.2696786471809,
-1.02006125965414));
#23257=CARTESIAN_POINT('Ctrl Pts',(-17.4474891140443,-15.51669804182,-1.0289160540572));
#23258=CARTESIAN_POINT('Ctrl Pts',(-17.3798092846713,-16.0156874200649,
-1.04901448949424));
#23259=CARTESIAN_POINT('Ctrl Pts',(-17.2940873360173,-16.2621352120533,
-1.0600687780929));
#23260=CARTESIAN_POINT('Ctrl Pts',(-17.0359029312521,-16.6981549445161,
-1.08192349548471));
#23261=CARTESIAN_POINT('Ctrl Pts',(-16.8692878718213,-16.8855107792871,
-1.09251504127557));
#23262=CARTESIAN_POINT('Ctrl Pts',(-16.4727055985413,-17.1880123648935,
-1.11236709943196));
#23263=CARTESIAN_POINT('Ctrl Pts',(-16.2460520786798,-17.2997096592015,
-1.12144644417648));
#23264=CARTESIAN_POINT('Ctrl Pts',(-15.7580841551168,-17.4316717914396,
-1.14249337041296));
#23265=CARTESIAN_POINT('Ctrl Pts',(-15.5010293351169,-17.4488346169957,
-1.15358060294202));
#23266=CARTESIAN_POINT('Ctrl Pts',(-15.0046042921056,-17.3835494183322,
-1.1749922998132));
#23267=CARTESIAN_POINT('Ctrl Pts',(-14.7694246895426,-17.3053971664748,
-1.18513601522654));
#23268=CARTESIAN_POINT('Ctrl Pts',(-14.3319804116802,-17.0601513560859,
-1.20400376657688));
#23269=CARTESIAN_POINT('Ctrl Pts',(-14.1358043637621,-16.8918928497275,
-1.21438674925062));
#23270=CARTESIAN_POINT('Ctrl Pts',(-13.8228284520313,-16.491712693971,-1.23608437075356));
#23271=CARTESIAN_POINT('Ctrl Pts',(-13.7078902727458,-16.2646868044627,
-1.24704326282161));
#23272=CARTESIAN_POINT('Ctrl Pts',(-13.5920235017517,-15.8517814521893,
-1.26496537710754));
#23273=CARTESIAN_POINT('Ctrl Pts',(-13.5679367061318,-15.6761515068699,
-1.27204517415848));
#23274=CARTESIAN_POINT('Ctrl Pts',(-13.5679367061318,-15.5,-1.27862500000012));
#23275=CARTESIAN_POINT('Origin',(-15.5,-15.5000000000001,11.20575));
#23276=CARTESIAN_POINT('',(-13.5679367061318,-15.5000000000001,-1.77862500000012));
#23277=CARTESIAN_POINT('',(-13.5679367061318,-15.5000000000001,-1.30987500000021));
#23278=CARTESIAN_POINT('',(-13.5679367061318,-15.5000000000001,11.20575));
#23279=CARTESIAN_POINT('',(-13.9369173237898,-16.6356236641577,-2.22824839946604));
#23280=CARTESIAN_POINT('Ctrl Pts',(-13.5679367061318,-15.5000000000001,
-1.77862500000012));
#23281=CARTESIAN_POINT('Ctrl Pts',(-13.5679367061318,-15.471311010133,-1.77969662612613));
#23282=CARTESIAN_POINT('Ctrl Pts',(-13.5685756992843,-15.4425999918154,
-1.78078285554243));
#23283=CARTESIAN_POINT('Ctrl Pts',(-13.5812658328334,-15.1581590394341,
-1.79168131481371));
#23284=CARTESIAN_POINT('Ctrl Pts',(-13.6433835358851,-14.907254339342,-1.8023930366865));
#23285=CARTESIAN_POINT('Ctrl Pts',(-13.8594981527771,-14.4490712177349,
-1.82416835554489));
#23286=CARTESIAN_POINT('Ctrl Pts',(-14.0095359247466,-14.2453192498238,
-1.83501484571359));
#23287=CARTESIAN_POINT('Ctrl Pts',(-14.3755767714584,-13.9097095421912,
-1.85544494572747));
#23288=CARTESIAN_POINT('Ctrl Pts',(-14.5868970850357,-13.7796534962008,
-1.86424124387686));
#23289=CARTESIAN_POINT('Ctrl Pts',(-15.0579406868171,-13.6016248094559,
-1.88455819395111));
#23290=CARTESIAN_POINT('Ctrl Pts',(-15.3147261186882,-13.5596639922644,
-1.89563380729006));
#23291=CARTESIAN_POINT('Ctrl Pts',(-15.8197591256804,-13.5785378998648,
-1.91741678098951));
#23292=CARTESIAN_POINT('Ctrl Pts',(-16.0633065482656,-13.6353374705016,
-1.92792141539418));
#23293=CARTESIAN_POINT('Ctrl Pts',(-16.5196132328428,-13.839629489679,-1.94760273596416));
#23294=CARTESIAN_POINT('Ctrl Pts',(-16.7273518612851,-13.9867054192994,
-1.95690084583355));
#23295=CARTESIAN_POINT('Ctrl Pts',(-17.0761951411224,-14.3540458832977,
-1.97814531088906));
#23296=CARTESIAN_POINT('Ctrl Pts',(-17.2132390451091,-14.571339412322,-1.98921739761544));
#23297=CARTESIAN_POINT('Ctrl Pts',(-17.3918917773575,-15.0377637909672,
-2.01049265502812));
#23298=CARTESIAN_POINT('Ctrl Pts',(-17.435193117581,-15.2811490466372,-2.02038271493815));
#23299=CARTESIAN_POINT('Ctrl Pts',(-17.4284331862708,-15.7819930621726,
-2.03923663515864));
#23300=CARTESIAN_POINT('Ctrl Pts',(-17.3741617364932,-16.0346645552799,
-2.04984514099419));
#23301=CARTESIAN_POINT('Ctrl Pts',(-17.1721421782215,-16.5000089832968,
-2.0715839852006));
#23302=CARTESIAN_POINT('Ctrl Pts',(-17.0279622251882,-16.7088902829552,
-2.08249574333672));
#23303=CARTESIAN_POINT('Ctrl Pts',(-16.6721862676384,-17.055293507434,-2.10310764446866));
#23304=CARTESIAN_POINT('Ctrl Pts',(-16.4656337928419,-17.1913024698242,
-2.11197549348959));
#23305=CARTESIAN_POINT('Ctrl Pts',(-16.0003669869149,-17.3839588971727,
-2.13204328006278));
#23306=CARTESIAN_POINT('Ctrl Pts',(-15.7441588924868,-17.4339176131202,
-2.14309399180884));
#23307=CARTESIAN_POINT('Ctrl Pts',(-15.2372592425206,-17.4301770605002,
-2.16495747714662));
#23308=CARTESIAN_POINT('Ctrl Pts',(-14.9914303043227,-17.3804225881419,
-2.17556051738595));
#23309=CARTESIAN_POINT('Ctrl Pts',(-14.6006806199507,-17.2188593062006,
-2.19241424769643));
#23310=CARTESIAN_POINT('Ctrl Pts',(-14.4493679378134,-17.1307744675633,
-2.19870147392335));
#23311=CARTESIAN_POINT('Ctrl Pts',(-14.1693732820954,-16.9124347548105,
-2.21289549932969));
#23312=CARTESIAN_POINT('Ctrl Pts',(-14.0431460179722,-16.7818378043867,
-2.22049591927733));
#23313=CARTESIAN_POINT('Ctrl Pts',(-13.9369173213529,-16.6356236661969,
-2.22824840453255));
#23314=CARTESIAN_POINT('',(-13.936918850212,-16.6356257705295,-1.75949829183043));
#23315=CARTESIAN_POINT('',(-13.9369184637307,-16.6356252385745,-1.75949832116282));
#23316=CARTESIAN_POINT('Ctrl Pts',(-13.9369188502404,-16.6356257705685,
-1.75949829295574));
#23317=CARTESIAN_POINT('Ctrl Pts',(-14.0732165037119,-16.8232265616206,
-1.74955141913573));
#23318=CARTESIAN_POINT('Ctrl Pts',(-14.2421926306504,-16.9847823163706,
-1.73987267086344));
#23319=CARTESIAN_POINT('Ctrl Pts',(-14.6256885475374,-17.2378815903647,
-1.72214816701709));
#23320=CARTESIAN_POINT('Ctrl Pts',(-14.8362794639394,-17.3287014043756,
-1.71350244965326));
#23321=CARTESIAN_POINT('Ctrl Pts',(-15.3036899854226,-17.4385845729922,
-1.69334220080743));
#23322=CARTESIAN_POINT('Ctrl Pts',(-15.5584934383084,-17.4476198869581,
-1.68235207375454));
#23323=CARTESIAN_POINT('Ctrl Pts',(-16.0626255591007,-17.3662648208193,
-1.66060795688251));
#23324=CARTESIAN_POINT('Ctrl Pts',(-16.3065929189332,-17.2745029457009,
-1.65043016901726));
#23325=CARTESIAN_POINT('Ctrl Pts',(-16.733960549226,-17.0069230177967,-1.63121863353652));
#23326=CARTESIAN_POINT('Ctrl Pts',(-16.9157196559872,-16.8376064327553,
-1.62097431691818));
#23327=CARTESIAN_POINT('Ctrl Pts',(-17.2115388605544,-16.4321558772132,
-1.59944982869596));
#23328=CARTESIAN_POINT('Ctrl Pts',(-17.3197729456466,-16.1976492003971,
-1.58835608490565));
#23329=CARTESIAN_POINT('Ctrl Pts',(-17.4370349875307,-15.7067373188983,
-1.56749008537745));
#23330=CARTESIAN_POINT('Ctrl Pts',(-17.44753196976,-15.4557223788834,-1.55855468409502));
#23331=CARTESIAN_POINT('Ctrl Pts',(-17.3726902789254,-14.9634366275316,
-1.53855219877786));
#23332=CARTESIAN_POINT('Ctrl Pts',(-17.2880297167387,-14.7268219856977,
-1.52788809973699));
#23333=CARTESIAN_POINT('Ctrl Pts',(-17.0300046441309,-14.2927306055599,
-1.50610884865219));
#23334=CARTESIAN_POINT('Ctrl Pts',(-16.856734367155,-14.1008202908098,-1.49520365267543));
#23335=CARTESIAN_POINT('Ctrl Pts',(-16.4544579219336,-13.8024087055848,
-1.47538156930747));
#23336=CARTESIAN_POINT('Ctrl Pts',(-16.2319055093256,-13.6952482164327,
-1.46644338907461));
#23337=CARTESIAN_POINT('Ctrl Pts',(-15.751832329794,-13.5679372308724,-1.44573697721882));
#23338=CARTESIAN_POINT('Ctrl Pts',(-15.4981347275309,-13.5515962723609,
-1.43479454747422));
#23339=CARTESIAN_POINT('Ctrl Pts',(-14.994677988732,-13.6177050294596,-1.41307956103129));
#23340=CARTESIAN_POINT('Ctrl Pts',(-14.7500889892405,-13.7011232772003,
-1.40256300391622));
#23341=CARTESIAN_POINT('Ctrl Pts',(-14.316768691791,-13.9530518157519,-1.38380772364027));
#23342=CARTESIAN_POINT('Ctrl Pts',(-14.130076521834,-14.1156697545301,-1.37370723712004));
#23343=CARTESIAN_POINT('Ctrl Pts',(-13.8216873535977,-14.5094994028651,
-1.35234574472347));
#23344=CARTESIAN_POINT('Ctrl Pts',(-13.7058009544627,-14.7392900935936,
-1.34126312922345));
#23345=CARTESIAN_POINT('Ctrl Pts',(-13.5913602763723,-15.1530393767009,
-1.32334024636843));
#23346=CARTESIAN_POINT('Ctrl Pts',(-13.5679367061318,-15.3262907155802,
-1.31636360097145));
#23347=CARTESIAN_POINT('Ctrl Pts',(-13.5679367061318,-15.5000000000002,
-1.30987500000021));
#23348=CARTESIAN_POINT('Origin',(-15.5,-15.5000000000001,11.20575));
#23349=CARTESIAN_POINT('Ctrl Pts',(-13.5679367061318,-15.5000000000002,
-1.30987500000021));
#23350=CARTESIAN_POINT('Ctrl Pts',(-13.5679367061318,-15.5762794463022,
-1.30702571712501));
#23351=CARTESIAN_POINT('Ctrl Pts',(-13.572453778509,-15.6526398620169,-1.30407599509047));
#23352=CARTESIAN_POINT('Ctrl Pts',(-13.6108964642078,-15.9751450143037,
-1.29120033868173));
#23353=CARTESIAN_POINT('Ctrl Pts',(-13.6874920713322,-16.2136336424646,
-1.28064016816177));
#23354=CARTESIAN_POINT('Ctrl Pts',(-13.9314508386655,-16.6572017226074,
-1.258810284233));
#23355=CARTESIAN_POINT('Ctrl Pts',(-14.099870499122,-16.8561400321267,-1.24774717789517));
#23356=CARTESIAN_POINT('Ctrl Pts',(-14.494999203763,-17.1682578349238,-1.22756727057358));
#23357=CARTESIAN_POINT('Ctrl Pts',(-14.7148147242685,-17.2823015923697,
-1.21874144035887));
#23358=CARTESIAN_POINT('Ctrl Pts',(-15.1908203591575,-17.4236222475759,
-1.19821046895298));
#23359=CARTESIAN_POINT('Ctrl Pts',(-15.4431561242079,-17.4474792441872,
-1.18732677767453));
#23360=CARTESIAN_POINT('Ctrl Pts',(-15.9476066067072,-17.3968415255677,
-1.16556892929466));
#23361=CARTESIAN_POINT('Ctrl Pts',(-16.1946658536917,-17.3209404210907,
-1.15491282364461));
#23362=CARTESIAN_POINT('Ctrl Pts',(-16.634975992356,-17.0825888205037,-1.13592146261012));
#23363=CARTESIAN_POINT('Ctrl Pts',(-16.8261410473283,-16.9262354938107,
-1.12621674018239));
#23364=CARTESIAN_POINT('Ctrl Pts',(-17.1458740756934,-16.5433162646628,
-1.10501814661225));
#23365=CARTESIAN_POINT('Ctrl Pts',(-17.2686545572972,-16.3180913830561,
-1.09395740174899));
#23366=CARTESIAN_POINT('Ctrl Pts',(-17.4197688669729,-15.8338668009503,
-1.07261114005866));
#23367=CARTESIAN_POINT('Ctrl Pts',(-17.4469489334785,-15.5797125649259,
-1.06317354299107));
#23368=CARTESIAN_POINT('Ctrl Pts',(-17.4022619456061,-15.0810498002785,
-1.04358316874007));
#23369=CARTESIAN_POINT('Ctrl Pts',(-17.3330146958169,-14.8410934256471,
-1.03312664703887));
#23370=CARTESIAN_POINT('Ctrl Pts',(-17.103339970937,-14.3916950333676,-1.01138703028765));
#23371=CARTESIAN_POINT('Ctrl Pts',(-16.9416955633754,-14.1882964703834,
-1.000303433491));
#23372=CARTESIAN_POINT('Ctrl Pts',(-16.5565376106631,-13.8637511465985,
-0.979874346405003));
#23373=CARTESIAN_POINT('Ctrl Pts',(-16.3394926778595,-13.742491770238,-0.97108381540342));
#23374=CARTESIAN_POINT('Ctrl Pts',(-15.8677779963459,-13.586815206346,-0.950737920464291));
#23375=CARTESIAN_POINT('Ctrl Pts',(-15.617066435513,-13.5553093488706,-0.939924284008528));
#23376=CARTESIAN_POINT('Ctrl Pts',(-15.1119904982334,-13.5900705720839,
-0.918139458649265));
#23377=CARTESIAN_POINT('Ctrl Pts',(-14.8626360597541,-13.6582150358001,
-0.907384357299389));
#23378=CARTESIAN_POINT('Ctrl Pts',(-14.415286943223,-13.8825858943853,-0.888089392604112));
#23379=CARTESIAN_POINT('Ctrl Pts',(-14.2195307589344,-14.0326711922678,
-0.878736660945362));
#23380=CARTESIAN_POINT('Ctrl Pts',(-13.888558418963,-14.404439389832,-0.857712208531265));
#23381=CARTESIAN_POINT('Ctrl Pts',(-13.7589900789029,-14.624853845409,-0.846684762349222));
#23382=CARTESIAN_POINT('Ctrl Pts',(-13.6042442375735,-15.0687257239406,
-0.826767486822917));
#23383=CARTESIAN_POINT('Ctrl Pts',(-13.5679367061318,-15.2837368797497,
-0.817953123727358));
#23384=CARTESIAN_POINT('Ctrl Pts',(-13.5679367061318,-15.5000000000002,
-0.809875000000204));
#23385=CARTESIAN_POINT('Ctrl Pts',(-13.5679367061318,-15.5,-1.27862500000012));
#23386=CARTESIAN_POINT('Ctrl Pts',(-13.5679367061318,-15.4323298280073,
-1.28115269876523));
#23387=CARTESIAN_POINT('Ctrl Pts',(-13.5714917240295,-15.3645884444351,
-1.28375972464103));
#23388=CARTESIAN_POINT('Ctrl Pts',(-13.6055206308558,-15.0424237115268,
-1.29652747821543));
#23389=CARTESIAN_POINT('Ctrl Pts',(-13.682764182422,-14.7956826309076,-1.30740987789996));
#23390=CARTESIAN_POINT('Ctrl Pts',(-13.9256313093853,-14.3526857719949,
-1.32919488267955));
#23391=CARTESIAN_POINT('Ctrl Pts',(-14.0865851623327,-14.1593885173579,
-1.33988627066607));
#23392=CARTESIAN_POINT('Ctrl Pts',(-14.4724436684446,-13.8450923874922,
-1.35994762542375));
#23393=CARTESIAN_POINT('Ctrl Pts',(-14.6935102311441,-13.7268197743643,
-1.36883965888249));
#23394=CARTESIAN_POINT('Ctrl Pts',(-15.1756013089239,-13.5782346236499,
-1.3896331062862));
#23395=CARTESIAN_POINT('Ctrl Pts',(-15.4328247709742,-13.552207619699,-1.40072761264747));
#23396=CARTESIAN_POINT('Ctrl Pts',(-15.9328184705041,-13.6009921106949,
-1.42229323203465));
#23397=CARTESIAN_POINT('Ctrl Pts',(-16.1712147184524,-13.671597546139,-1.43257568709642));
#23398=CARTESIAN_POINT('Ctrl Pts',(-16.618156863512,-13.9035318490541,-1.45185309838682));
#23399=CARTESIAN_POINT('Ctrl Pts',(-16.8204876400156,-14.0663572621764,
-1.46188465464224));
#23400=CARTESIAN_POINT('Ctrl Pts',(-17.1467361911896,-14.4583495489556,
-1.48356266917816));
#23401=CARTESIAN_POINT('Ctrl Pts',(-17.2687582051385,-14.6825207434489,
-1.49456769840488));
#23402=CARTESIAN_POINT('Ctrl Pts',(-17.4170635504822,-15.1571942806963,
-1.51549662000442));
#23403=CARTESIAN_POINT('Ctrl Pts',(-17.4450135091226,-15.4022628476122,
-1.52469491979447));
#23404=CARTESIAN_POINT('Ctrl Pts',(-17.4071872139687,-15.9013115829333,
-1.54415175434035));
#23405=CARTESIAN_POINT('Ctrl Pts',(-17.3372890130251,-16.1502012038136,
-1.55495599988825));
#23406=CARTESIAN_POINT('Ctrl Pts',(-17.1073436483912,-16.6008033545264,
-1.57674641747953));
#23407=CARTESIAN_POINT('Ctrl Pts',(-16.9516283692376,-16.7992722722736,
-1.58751800921948));
#23408=CARTESIAN_POINT('Ctrl Pts',(-16.5754069871356,-17.1240092467816,
-1.60776152996803));
#23409=CARTESIAN_POINT('Ctrl Pts',(-16.3591691893559,-17.2480659982536,
-1.61656750158718));
#23410=CARTESIAN_POINT('Ctrl Pts',(-15.8824275687686,-17.4111698385855,
-1.63713021736795));
#23411=CARTESIAN_POINT('Ctrl Pts',(-15.6253005633504,-17.4450216013441,
-1.64822056338276));
#23412=CARTESIAN_POINT('Ctrl Pts',(-15.1226120634958,-17.4108856794204,
-1.6699024143108));
#23413=CARTESIAN_POINT('Ctrl Pts',(-14.8815852150972,-17.3470216561184,
-1.68029833185843));
#23414=CARTESIAN_POINT('Ctrl Pts',(-14.4299734275499,-17.1287077735559,
-1.69977715315189));
#23415=CARTESIAN_POINT('Ctrl Pts',(-14.2249541814665,-16.9737451489754,
-1.70940670711442));
#23416=CARTESIAN_POINT('Ctrl Pts',(-13.8873840854283,-16.5939162203865,
-1.73087454027017));
#23417=CARTESIAN_POINT('Ctrl Pts',(-13.7578745391481,-16.3730298263104,
-1.74191834693414));
#23418=CARTESIAN_POINT('Ctrl Pts',(-13.6039590632987,-15.9295232152934,
-1.76180407097136));
#23419=CARTESIAN_POINT('Ctrl Pts',(-13.5679367061318,-15.7154111956131,
-1.77057869840067));
#23420=CARTESIAN_POINT('Ctrl Pts',(-13.5679367061318,-15.5000000000001,
-1.77862500000012));
#23421=CARTESIAN_POINT('Origin',(15.5,-15.5,11.20575));
#23422=CARTESIAN_POINT('Ctrl Pts',(15.5000000000001,-13.5679367061317,-1.30987500000019));
#23423=CARTESIAN_POINT('Ctrl Pts',(15.5762794463024,-13.5679367061317,-1.30702571712498));
#23424=CARTESIAN_POINT('Ctrl Pts',(15.6526398620174,-13.5724537785089,-1.30407599509039));
#23425=CARTESIAN_POINT('Ctrl Pts',(15.9751450143044,-13.6108964642079,-1.29120033868165));
#23426=CARTESIAN_POINT('Ctrl Pts',(16.2136336424653,-13.6874920713324,-1.28064016816167));
#23427=CARTESIAN_POINT('Ctrl Pts',(16.657201722608,-13.9314508386658,-1.2588102842329));
#23428=CARTESIAN_POINT('Ctrl Pts',(16.8561400321273,-14.0998704991224,-1.24774717789506));
#23429=CARTESIAN_POINT('Ctrl Pts',(17.1682578349242,-14.4949992037636,-1.2275672705735));
#23430=CARTESIAN_POINT('Ctrl Pts',(17.28230159237,-14.7148147242691,-1.2187414403588));
#23431=CARTESIAN_POINT('Ctrl Pts',(17.423622247576,-15.1908203591582,-1.19821046895292));
#23432=CARTESIAN_POINT('Ctrl Pts',(17.4474792441873,-15.4431561242087,-1.18732677767448));
#23433=CARTESIAN_POINT('Ctrl Pts',(17.3968415255676,-15.9476066067079,-1.16556892929462));
#23434=CARTESIAN_POINT('Ctrl Pts',(17.3209404210904,-16.1946658536924,-1.15491282364457));
#23435=CARTESIAN_POINT('Ctrl Pts',(17.0825888205032,-16.6349759923567,-1.13592146261006));
#23436=CARTESIAN_POINT('Ctrl Pts',(16.9262354938101,-16.826141047329,-1.12621674018233));
#23437=CARTESIAN_POINT('Ctrl Pts',(16.5433162646621,-17.145874075694,-1.10501814661218));
#23438=CARTESIAN_POINT('Ctrl Pts',(16.3180913830553,-17.2686545572977,-1.09395740174894));
#23439=CARTESIAN_POINT('Ctrl Pts',(15.8338668009495,-17.4197688669732,-1.07261114005862));
#23440=CARTESIAN_POINT('Ctrl Pts',(15.579712564925,-17.4469489334786,-1.06317354299105));
#23441=CARTESIAN_POINT('Ctrl Pts',(15.0810498002778,-17.402261945606,-1.04358316874003));
#23442=CARTESIAN_POINT('Ctrl Pts',(14.8410934256464,-17.3330146958168,-1.03312664703881));
#23443=CARTESIAN_POINT('Ctrl Pts',(14.391695033367,-17.1033399709368,-1.01138703028757));
#23444=CARTESIAN_POINT('Ctrl Pts',(14.1882964703829,-16.9416955633752,-1.0003034334909));
#23445=CARTESIAN_POINT('Ctrl Pts',(13.863751146598,-16.5565376106627,-0.979874346404903));
#23446=CARTESIAN_POINT('Ctrl Pts',(13.7424917702376,-16.3394926778591,-0.971083815403324));
#23447=CARTESIAN_POINT('Ctrl Pts',(13.5868152063457,-15.8677779963454,-0.950737920464194));
#23448=CARTESIAN_POINT('Ctrl Pts',(13.5553093488703,-15.6170664355125,-0.939924284008434));
#23449=CARTESIAN_POINT('Ctrl Pts',(13.5900705720838,-15.1119904982328,-0.918139458649165));
#23450=CARTESIAN_POINT('Ctrl Pts',(13.6582150358001,-14.8626360597536,-0.907384357299283));
#23451=CARTESIAN_POINT('Ctrl Pts',(13.8825858943854,-14.4152869432226,-0.888089392603988));
#23452=CARTESIAN_POINT('Ctrl Pts',(14.0326711922679,-14.219530758934,-0.878736660945231));
#23453=CARTESIAN_POINT('Ctrl Pts',(14.4044393898322,-13.8885584189627,-0.857712208531138));
#23454=CARTESIAN_POINT('Ctrl Pts',(14.6248538454093,-13.7589900789026,-0.846684762349108));
#23455=CARTESIAN_POINT('Ctrl Pts',(15.0687257239408,-13.6042442375733,-0.826767486822827));
#23456=CARTESIAN_POINT('Ctrl Pts',(15.2837368797498,-13.5679367061317,-0.817953123727326));
#23457=CARTESIAN_POINT('Ctrl Pts',(15.5000000000001,-13.5679367061317,-0.809875000000185));
#23458=CARTESIAN_POINT('Ctrl Pts',(15.4999999999999,-13.5679367061317,-1.27862500000015));
#23459=CARTESIAN_POINT('Ctrl Pts',(15.4323298281631,-13.5679367061317,-1.28115269875943));
#23460=CARTESIAN_POINT('Ctrl Pts',(15.364588444747,-13.5714917240132,-1.28375972462899));
#23461=CARTESIAN_POINT('Ctrl Pts',(15.0424237119866,-13.6055206307448,-1.29652747819584));
#23462=CARTESIAN_POINT('Ctrl Pts',(14.795682631349,-13.6827641822509,-1.30740987787979));
#23463=CARTESIAN_POINT('Ctrl Pts',(14.3526857723723,-13.9256313091094,-1.32919488265952));
#23464=CARTESIAN_POINT('Ctrl Pts',(14.1593885176923,-14.0865851620145,-1.33988627064674));
#23465=CARTESIAN_POINT('Ctrl Pts',(13.8450923877406,-14.4724436680476,-1.35994762540591));
#23466=CARTESIAN_POINT('Ctrl Pts',(13.7268197745649,-14.6935102307068,-1.36883965886362));
#23467=CARTESIAN_POINT('Ctrl Pts',(13.5782346237301,-15.175601308443,-1.38963310626542));
#23468=CARTESIAN_POINT('Ctrl Pts',(13.5522076197147,-15.4328247704935,-1.4007276126267));
#23469=CARTESIAN_POINT('Ctrl Pts',(13.6009921105901,-15.9328184700475,-1.42229323201492));
#23470=CARTESIAN_POINT('Ctrl Pts',(13.6715975459788,-16.1712147180183,-1.43257568707766));
#23471=CARTESIAN_POINT('Ctrl Pts',(13.9035318487812,-16.618156863117,-1.45185309836975));
#23472=CARTESIAN_POINT('Ctrl Pts',(14.0663572618374,-16.8204876396432,-1.46188465462152));
#23473=CARTESIAN_POINT('Ctrl Pts',(14.4583495485159,-17.1467361909125,-1.48356266915572));
#23474=CARTESIAN_POINT('Ctrl Pts',(14.6825207429828,-17.268758204924,-1.49456769838278));
#23475=CARTESIAN_POINT('Ctrl Pts',(15.1571942801975,-17.4170635503929,-1.51549661998378));
#23476=CARTESIAN_POINT('Ctrl Pts',(15.4022628471055,-17.445013509097,-1.524694919776));
#23477=CARTESIAN_POINT('Ctrl Pts',(15.9013115824355,-17.4071872140733,-1.5441517543194));
#23478=CARTESIAN_POINT('Ctrl Pts',(16.1502012033337,-17.3372890131948,-1.55495599986658));
#23479=CARTESIAN_POINT('Ctrl Pts',(16.6008033541118,-17.1073436486759,-1.57674641745783));
#23480=CARTESIAN_POINT('Ctrl Pts',(16.7992722719041,-16.9516283695692,-1.58751800919846));
#23481=CARTESIAN_POINT('Ctrl Pts',(17.1240092465038,-16.5754069875524,-1.60776152994859));
#23482=CARTESIAN_POINT('Ctrl Pts',(17.2480659980264,-16.3591691898146,-1.6165675015673));
#23483=CARTESIAN_POINT('Ctrl Pts',(17.411169838485,-15.8824275692749,-1.63713021734601));
#23484=CARTESIAN_POINT('Ctrl Pts',(17.4450216013122,-15.6253005638585,-1.64822056336075));
#23485=CARTESIAN_POINT('Ctrl Pts',(17.4108856795171,-15.1226120639822,-1.66990241428974));
#23486=CARTESIAN_POINT('Ctrl Pts',(17.3470216562745,-14.8815852155614,-1.68029833183834));
#23487=CARTESIAN_POINT('Ctrl Pts',(17.1287077738309,-14.4299734279737,-1.69977715313357));
#23488=CARTESIAN_POINT('Ctrl Pts',(16.9737451493181,-14.2249541818671,-1.70940670709295));
#23489=CARTESIAN_POINT('Ctrl Pts',(16.5939162208352,-13.8873840857317,-1.73087454024684));
#23490=CARTESIAN_POINT('Ctrl Pts',(16.3730298267886,-13.7578745393868,-1.74191834691109));
#23491=CARTESIAN_POINT('Ctrl Pts',(15.9295232156415,-13.6039590633578,-1.76180407095704));
#23492=CARTESIAN_POINT('Ctrl Pts',(15.7154111957893,-13.5679367061317,-1.77057869839411));
#23493=CARTESIAN_POINT('Ctrl Pts',(15.5,-13.5679367061317,-1.77862500000015));
#23494=CARTESIAN_POINT('Origin',(15.4999999999998,15.5000000000002,11.20575));
#23495=CARTESIAN_POINT('Ctrl Pts',(13.5679367061316,15.5000000000003,-1.30987500000013));
#23496=CARTESIAN_POINT('Ctrl Pts',(13.5679367061316,15.5762794463024,-1.30702571712493));
#23497=CARTESIAN_POINT('Ctrl Pts',(13.5724537785087,15.6526398620172,-1.30407599509038));
#23498=CARTESIAN_POINT('Ctrl Pts',(13.6108964642076,15.975145014304,-1.29120033868164));
#23499=CARTESIAN_POINT('Ctrl Pts',(13.6874920713321,16.213633642465,-1.28064016816168));
#23500=CARTESIAN_POINT('Ctrl Pts',(13.9314508386654,16.6572017226077,-1.25881028423292));
#23501=CARTESIAN_POINT('Ctrl Pts',(14.0998704991219,16.856140032127,-1.24774717789509));
#23502=CARTESIAN_POINT('Ctrl Pts',(14.494999203763,17.168257834924,-1.22756727057352));
#23503=CARTESIAN_POINT('Ctrl Pts',(14.7148147242685,17.2823015923699,-1.21874144035882));
#23504=CARTESIAN_POINT('Ctrl Pts',(15.1908203591575,17.4236222475761,-1.19821046895294));
#23505=CARTESIAN_POINT('Ctrl Pts',(15.4431561242079,17.4474792441874,-1.18732677767449));
#23506=CARTESIAN_POINT('Ctrl Pts',(15.9476066067072,17.3968415255678,-1.16556892929464));
#23507=CARTESIAN_POINT('Ctrl Pts',(16.1946658536917,17.3209404210907,-1.1549128236446));
#23508=CARTESIAN_POINT('Ctrl Pts',(16.634975992356,17.0825888205037,-1.13592146261013));
#23509=CARTESIAN_POINT('Ctrl Pts',(16.8261410473284,16.9262354938106,-1.1262167401824));
#23510=CARTESIAN_POINT('Ctrl Pts',(17.1458740756934,16.5433162646627,-1.10501814661226));
#23511=CARTESIAN_POINT('Ctrl Pts',(17.2686545572972,16.318091383056,-1.09395740174901));
#23512=CARTESIAN_POINT('Ctrl Pts',(17.4197688669728,15.8338668009502,-1.07261114005869));
#23513=CARTESIAN_POINT('Ctrl Pts',(17.4469489334783,15.5797125649257,-1.0631735429911));
#23514=CARTESIAN_POINT('Ctrl Pts',(17.4022619456059,15.0810498002784,-1.04358316874009));
#23515=CARTESIAN_POINT('Ctrl Pts',(17.3330146958167,14.8410934256471,-1.03312664703889));
#23516=CARTESIAN_POINT('Ctrl Pts',(17.1033399709367,14.3916950333675,-1.01138703028766));
#23517=CARTESIAN_POINT('Ctrl Pts',(16.9416955633752,14.1882964703834,-1.00030343349101));
#23518=CARTESIAN_POINT('Ctrl Pts',(16.5565376106628,13.8637511465985,-0.979874346405002));
#23519=CARTESIAN_POINT('Ctrl Pts',(16.3394926778592,13.742491770238,-0.971083815403412));
#23520=CARTESIAN_POINT('Ctrl Pts',(15.8677779963456,13.5868152063461,-0.950737920464266));
#23521=CARTESIAN_POINT('Ctrl Pts',(15.6170664355127,13.5553093488706,-0.939924284008494));
#23522=CARTESIAN_POINT('Ctrl Pts',(15.111990498233,13.590070572084,-0.918139458649215));
#23523=CARTESIAN_POINT('Ctrl Pts',(14.8626360597538,13.6582150358002,-0.907384357299333));
#23524=CARTESIAN_POINT('Ctrl Pts',(14.4152869432227,13.8825858943855,-0.888089392604046));
#23525=CARTESIAN_POINT('Ctrl Pts',(14.2195307589341,14.0326711922679,-0.878736660945288));
#23526=CARTESIAN_POINT('Ctrl Pts',(13.8885584189627,14.4044393898322,-0.857712208531179));
#23527=CARTESIAN_POINT('Ctrl Pts',(13.7589900789026,14.6248538454092,-0.846684762349132));
#23528=CARTESIAN_POINT('Ctrl Pts',(13.6042442375732,15.0687257239408,-0.826767486822827));
#23529=CARTESIAN_POINT('Ctrl Pts',(13.5679367061315,15.2837368797499,-0.817953123727281));
#23530=CARTESIAN_POINT('Ctrl Pts',(13.5679367061315,15.5000000000003,-0.809875000000128));
#23531=CARTESIAN_POINT('Ctrl Pts',(13.5679367061315,15.5000000000001,-1.2786250000002));
#23532=CARTESIAN_POINT('Ctrl Pts',(13.5679367061315,15.4323298280958,-1.281152698762));
#23533=CARTESIAN_POINT('Ctrl Pts',(13.57149172402,15.364588444612,-1.28375972463429));
#23534=CARTESIAN_POINT('Ctrl Pts',(13.6055206307927,15.0424237117876,-1.2965274782044));
#23535=CARTESIAN_POINT('Ctrl Pts',(13.6827641823248,14.7956826311579,-1.30740987788859));
#23536=CARTESIAN_POINT('Ctrl Pts',(13.9256313092287,14.3526857722089,-1.32919488266825));
#23537=CARTESIAN_POINT('Ctrl Pts',(14.0865851621521,14.1593885175476,-1.33988627065515));
#23538=CARTESIAN_POINT('Ctrl Pts',(14.4724436682193,13.8450923876331,-1.35994762541367));
#23539=CARTESIAN_POINT('Ctrl Pts',(14.6935102308959,13.7268197744781,-1.36883965887183));
#23540=CARTESIAN_POINT('Ctrl Pts',(15.1756013086511,13.5782346236955,-1.38963310627446));
#23541=CARTESIAN_POINT('Ctrl Pts',(15.4328247707015,13.552207619708,-1.40072761263572));
#23542=CARTESIAN_POINT('Ctrl Pts',(15.932818470245,13.6009921106356,-1.42229323202347));
#23543=CARTESIAN_POINT('Ctrl Pts',(16.1712147182061,13.6715975460483,-1.43257568708578));
#23544=CARTESIAN_POINT('Ctrl Pts',(16.6181568632879,13.9035318488995,-1.45185309837713));
#23545=CARTESIAN_POINT('Ctrl Pts',(16.8204876398043,14.0663572619843,-1.46188465463047));
#23546=CARTESIAN_POINT('Ctrl Pts',(17.1467361910322,14.4583495487063,-1.48356266916542));
#23547=CARTESIAN_POINT('Ctrl Pts',(17.2687582050167,14.6825207431847,-1.49456769839234));
#23548=CARTESIAN_POINT('Ctrl Pts',(17.4170635504314,15.1571942804135,-1.51549661999271));
#23549=CARTESIAN_POINT('Ctrl Pts',(17.4450135091079,15.402262847325,-1.524694919784));
#23550=CARTESIAN_POINT('Ctrl Pts',(17.4071872140279,15.9013115826512,-1.54415175432848));
#23551=CARTESIAN_POINT('Ctrl Pts',(17.3372890131212,16.1502012035416,-1.55495599987596));
#23552=CARTESIAN_POINT('Ctrl Pts',(17.1073436485524,16.6008033542915,-1.57674641746723));
#23553=CARTESIAN_POINT('Ctrl Pts',(16.9516283694255,16.7992722720642,-1.58751800920757));
#23554=CARTESIAN_POINT('Ctrl Pts',(16.5754069873718,17.1240092466243,-1.60776152995703));
#23555=CARTESIAN_POINT('Ctrl Pts',(16.3591691896159,17.248065998125,-1.61656750157594));
#23556=CARTESIAN_POINT('Ctrl Pts',(15.8824275690554,17.4111698385287,-1.63713021735557));
#23557=CARTESIAN_POINT('Ctrl Pts',(15.6253005636383,17.4450216013262,-1.64822056337034));
#23558=CARTESIAN_POINT('Ctrl Pts',(15.1226120637714,17.4108856794754,-1.66990241429892));
#23559=CARTESIAN_POINT('Ctrl Pts',(14.8815852153602,17.3470216562071,-1.68029833184711));
#23560=CARTESIAN_POINT('Ctrl Pts',(14.42997342779,17.1287077737121,-1.69977715314157));
#23561=CARTESIAN_POINT('Ctrl Pts',(14.2249541816935,16.97374514917,-1.70940670710231));
#23562=CARTESIAN_POINT('Ctrl Pts',(13.8873840856002,16.5939162206412,-1.73087454025701));
#23563=CARTESIAN_POINT('Ctrl Pts',(13.7578745392833,16.3730298265818,-1.74191834692115));
#23564=CARTESIAN_POINT('Ctrl Pts',(13.603959063332,15.9295232154911,-1.76180407096332));
#23565=CARTESIAN_POINT('Ctrl Pts',(13.5679367061315,15.7154111957132,-1.77057869839701));
#23566=CARTESIAN_POINT('Ctrl Pts',(13.5679367061315,15.5000000000002,-1.7786250000002));
#23567=CARTESIAN_POINT('Origin',(-15.5,15.5,11.20575));
#23568=CARTESIAN_POINT('Ctrl Pts',(-15.5000000000001,13.5679367061317,-1.30987500000019));
#23569=CARTESIAN_POINT('Ctrl Pts',(-15.5762794463024,13.5679367061317,-1.30702571712498));
#23570=CARTESIAN_POINT('Ctrl Pts',(-15.6526398620174,13.5724537785089,-1.30407599509039));
#23571=CARTESIAN_POINT('Ctrl Pts',(-15.9751450143044,13.6108964642079,-1.29120033868165));
#23572=CARTESIAN_POINT('Ctrl Pts',(-16.2136336424653,13.6874920713324,-1.28064016816167));
#23573=CARTESIAN_POINT('Ctrl Pts',(-16.657201722608,13.9314508386658,-1.2588102842329));
#23574=CARTESIAN_POINT('Ctrl Pts',(-16.8561400321273,14.0998704991224,-1.24774717789506));
#23575=CARTESIAN_POINT('Ctrl Pts',(-17.1682578349242,14.4949992037636,-1.2275672705735));
#23576=CARTESIAN_POINT('Ctrl Pts',(-17.28230159237,14.7148147242692,-1.2187414403588));
#23577=CARTESIAN_POINT('Ctrl Pts',(-17.423622247576,15.1908203591582,-1.19821046895292));
#23578=CARTESIAN_POINT('Ctrl Pts',(-17.4474792441873,15.4431561242087,-1.18732677767448));
#23579=CARTESIAN_POINT('Ctrl Pts',(-17.3968415255676,15.9476066067079,-1.16556892929462));
#23580=CARTESIAN_POINT('Ctrl Pts',(-17.3209404210904,16.1946658536924,-1.15491282364457));
#23581=CARTESIAN_POINT('Ctrl Pts',(-17.0825888205032,16.6349759923567,-1.13592146261006));
#23582=CARTESIAN_POINT('Ctrl Pts',(-16.9262354938101,16.826141047329,-1.12621674018233));
#23583=CARTESIAN_POINT('Ctrl Pts',(-16.5433162646621,17.145874075694,-1.10501814661218));
#23584=CARTESIAN_POINT('Ctrl Pts',(-16.3180913830553,17.2686545572977,-1.09395740174894));
#23585=CARTESIAN_POINT('Ctrl Pts',(-15.8338668009495,17.4197688669732,-1.07261114005862));
#23586=CARTESIAN_POINT('Ctrl Pts',(-15.579712564925,17.4469489334786,-1.06317354299105));
#23587=CARTESIAN_POINT('Ctrl Pts',(-15.0810498002778,17.402261945606,-1.04358316874003));
#23588=CARTESIAN_POINT('Ctrl Pts',(-14.8410934256464,17.3330146958168,-1.03312664703881));
#23589=CARTESIAN_POINT('Ctrl Pts',(-14.391695033367,17.1033399709368,-1.01138703028757));
#23590=CARTESIAN_POINT('Ctrl Pts',(-14.1882964703828,16.9416955633752,-1.0003034334909));
#23591=CARTESIAN_POINT('Ctrl Pts',(-13.863751146598,16.5565376106627,-0.979874346404903));
#23592=CARTESIAN_POINT('Ctrl Pts',(-13.7424917702376,16.3394926778591,-0.971083815403324));
#23593=CARTESIAN_POINT('Ctrl Pts',(-13.5868152063457,15.8677779963454,-0.950737920464194));
#23594=CARTESIAN_POINT('Ctrl Pts',(-13.5553093488703,15.6170664355125,-0.939924284008433));
#23595=CARTESIAN_POINT('Ctrl Pts',(-13.5900705720838,15.1119904982328,-0.918139458649165));
#23596=CARTESIAN_POINT('Ctrl Pts',(-13.6582150358001,14.8626360597536,-0.907384357299283));
#23597=CARTESIAN_POINT('Ctrl Pts',(-13.8825858943854,14.4152869432226,-0.888089392603988));
#23598=CARTESIAN_POINT('Ctrl Pts',(-14.0326711922679,14.219530758934,-0.878736660945231));
#23599=CARTESIAN_POINT('Ctrl Pts',(-14.4044393898322,13.8885584189627,-0.857712208531138));
#23600=CARTESIAN_POINT('Ctrl Pts',(-14.6248538454093,13.7589900789026,-0.846684762349108));
#23601=CARTESIAN_POINT('Ctrl Pts',(-15.0687257239408,13.6042442375733,-0.826767486822827));
#23602=CARTESIAN_POINT('Ctrl Pts',(-15.2837368797498,13.5679367061317,-0.817953123727327));
#23603=CARTESIAN_POINT('Ctrl Pts',(-15.5000000000001,13.5679367061317,-0.809875000000185));
#23604=CARTESIAN_POINT('Ctrl Pts',(-15.4999999999999,13.5679367061317,-1.27862500000015));
#23605=CARTESIAN_POINT('Ctrl Pts',(-15.4323298281631,13.5679367061317,-1.28115269875943));
#23606=CARTESIAN_POINT('Ctrl Pts',(-15.364588444747,13.5714917240132,-1.28375972462899));
#23607=CARTESIAN_POINT('Ctrl Pts',(-15.0424237119866,13.6055206307448,-1.29652747819584));
#23608=CARTESIAN_POINT('Ctrl Pts',(-14.795682631349,13.6827641822509,-1.30740987787979));
#23609=CARTESIAN_POINT('Ctrl Pts',(-14.3526857723723,13.9256313091094,-1.32919488265952));
#23610=CARTESIAN_POINT('Ctrl Pts',(-14.1593885176923,14.0865851620145,-1.33988627064674));
#23611=CARTESIAN_POINT('Ctrl Pts',(-13.8450923877406,14.4724436680476,-1.35994762540591));
#23612=CARTESIAN_POINT('Ctrl Pts',(-13.7268197745649,14.6935102307068,-1.36883965886362));
#23613=CARTESIAN_POINT('Ctrl Pts',(-13.5782346237301,15.175601308443,-1.38963310626542));
#23614=CARTESIAN_POINT('Ctrl Pts',(-13.5522076197147,15.4328247704935,-1.4007276126267));
#23615=CARTESIAN_POINT('Ctrl Pts',(-13.6009921105901,15.9328184700475,-1.42229323201492));
#23616=CARTESIAN_POINT('Ctrl Pts',(-13.6715975459788,16.1712147180183,-1.43257568707766));
#23617=CARTESIAN_POINT('Ctrl Pts',(-13.9035318487812,16.618156863117,-1.45185309836975));
#23618=CARTESIAN_POINT('Ctrl Pts',(-14.0663572618374,16.8204876396432,-1.46188465462152));
#23619=CARTESIAN_POINT('Ctrl Pts',(-14.4583495485159,17.1467361909125,-1.48356266915572));
#23620=CARTESIAN_POINT('Ctrl Pts',(-14.6825207429828,17.268758204924,-1.49456769838278));
#23621=CARTESIAN_POINT('Ctrl Pts',(-15.1571942801975,17.4170635503929,-1.51549661998378));
#23622=CARTESIAN_POINT('Ctrl Pts',(-15.4022628471055,17.445013509097,-1.524694919776));
#23623=CARTESIAN_POINT('Ctrl Pts',(-15.9013115824355,17.4071872140733,-1.5441517543194));
#23624=CARTESIAN_POINT('Ctrl Pts',(-16.1502012033337,17.3372890131948,-1.55495599986658));
#23625=CARTESIAN_POINT('Ctrl Pts',(-16.6008033541118,17.1073436486759,-1.57674641745783));
#23626=CARTESIAN_POINT('Ctrl Pts',(-16.7992722719041,16.9516283695692,-1.58751800919846));
#23627=CARTESIAN_POINT('Ctrl Pts',(-17.1240092465038,16.5754069875524,-1.60776152994859));
#23628=CARTESIAN_POINT('Ctrl Pts',(-17.2480659980264,16.3591691898146,-1.6165675015673));
#23629=CARTESIAN_POINT('Ctrl Pts',(-17.411169838485,15.8824275692749,-1.63713021734601));
#23630=CARTESIAN_POINT('Ctrl Pts',(-17.4450216013122,15.6253005638585,-1.64822056336075));
#23631=CARTESIAN_POINT('Ctrl Pts',(-17.4108856795171,15.1226120639822,-1.66990241428974));
#23632=CARTESIAN_POINT('Ctrl Pts',(-17.3470216562745,14.8815852155614,-1.68029833183834));
#23633=CARTESIAN_POINT('Ctrl Pts',(-17.1287077738309,14.4299734279737,-1.69977715313357));
#23634=CARTESIAN_POINT('Ctrl Pts',(-16.9737451493181,14.2249541818671,-1.70940670709295));
#23635=CARTESIAN_POINT('Ctrl Pts',(-16.5939162208352,13.8873840857317,-1.73087454024684));
#23636=CARTESIAN_POINT('Ctrl Pts',(-16.3730298267886,13.7578745393868,-1.74191834691109));
#23637=CARTESIAN_POINT('Ctrl Pts',(-15.9295232156415,13.6039590633578,-1.76180407095704));
#23638=CARTESIAN_POINT('Ctrl Pts',(-15.7154111957893,13.5679367061317,-1.77057869839411));
#23639=CARTESIAN_POINT('Ctrl Pts',(-15.5,13.5679367061317,-1.77862500000015));
#23640=CARTESIAN_POINT('Origin',(-15.5,15.5,-1.713));
#23641=CARTESIAN_POINT('',(-17.32565468021,16.0440680000031,1.3858));
#23642=CARTESIAN_POINT('Ctrl Pts',(-17.405,15.5,1.86199999999989));
#23643=CARTESIAN_POINT('Ctrl Pts',(-17.405,15.4320300859014,1.85902668792209));
#23644=CARTESIAN_POINT('Ctrl Pts',(-17.4013623773891,15.3639795867244,1.85604985068775));
#23645=CARTESIAN_POINT('Ctrl Pts',(-17.3680903519982,15.0548487108932,1.84252706521832));
#23646=CARTESIAN_POINT('Ctrl Pts',(-17.2962463427199,14.8207041548242,1.8322845212083));
#23647=CARTESIAN_POINT('Ctrl Pts',(-17.0629990902563,14.3816006382695,1.81307614340625));
#23648=CARTESIAN_POINT('Ctrl Pts',(-16.8997756224006,14.1830144823051,1.80289013515953));
#23649=CARTESIAN_POINT('Ctrl Pts',(-16.5091900816921,13.8652038277476,1.7811420018313));
#23650=CARTESIAN_POINT('Ctrl Pts',(-16.2871007630363,13.7474308444605,1.77015243562359));
#23651=CARTESIAN_POINT('Ctrl Pts',(-15.8177448508294,13.6062726464789,1.74928396482839));
#23652=CARTESIAN_POINT('Ctrl Pts',(-15.5757787768183,13.5813005437059,1.74017043193075));
#23653=CARTESIAN_POINT('Ctrl Pts',(-15.0840796797206,13.6238960707691,1.72061130364396));
#23654=CARTESIAN_POINT('Ctrl Pts',(-14.8394161266748,13.6954601884097,1.70977723054079));
#23655=CARTESIAN_POINT('Ctrl Pts',(-14.3978031730946,13.9268566861076,1.68798605445638));
#23656=CARTESIAN_POINT('Ctrl Pts',(-14.2039509059274,14.082295157107,1.67724238763888));
#23657=CARTESIAN_POINT('Ctrl Pts',(-13.8874957229304,14.4567250042913,1.65706420954498));
#23658=CARTESIAN_POINT('Ctrl Pts',(-13.7672449283597,14.67165607392,1.64823551732623));
#23659=CARTESIAN_POINT('Ctrl Pts',(-13.6116074571869,15.1436631098165,1.62758779047162));
#23660=CARTESIAN_POINT('Ctrl Pts',(-13.5810328132329,15.3972548412816,1.61649453887646));
#23661=CARTESIAN_POINT('Ctrl Pts',(-13.6199507818047,15.8919955927732,1.59485233627403));
#23662=CARTESIAN_POINT('Ctrl Pts',(-13.6853476751625,16.1287315281175,1.58449643359055));
#23663=CARTESIAN_POINT('Ctrl Pts',(-13.9054834861942,16.572367937139,1.56508976652923));
#23664=CARTESIAN_POINT('Ctrl Pts',(-14.0610698096642,16.7735622211342,1.55532322784484));
#23665=CARTESIAN_POINT('Ctrl Pts',(-14.4399397318407,17.1023987051858,1.53377776768035));
#23666=CARTESIAN_POINT('Ctrl Pts',(-14.6589383366756,17.2274330903607,1.52274646637818));
#23667=CARTESIAN_POINT('Ctrl Pts',(-15.124472454443,17.3831189075426,1.50170502801835));
#23668=CARTESIAN_POINT('Ctrl Pts',(-15.3655432554421,17.4154773378446,1.49232290574879));
#23669=CARTESIAN_POINT('Ctrl Pts',(-15.8582468171056,17.3879615174967,1.47305555180698));
#23670=CARTESIAN_POINT('Ctrl Pts',(-16.1049540011558,17.3239372389492,1.46230897140638));
#23671=CARTESIAN_POINT('Ctrl Pts',(-16.5540792357571,17.10589348966,1.44052525586438));
#23672=CARTESIAN_POINT('Ctrl Pts',(-16.7531192799618,16.9559118142615,1.42970440842995));
#23673=CARTESIAN_POINT('Ctrl Pts',(-17.0114997971817,16.6679033966798,1.41361655626258));
#23674=CARTESIAN_POINT('Ctrl Pts',(-17.0932012813456,16.5537180410099,1.40809440249374));
#23675=CARTESIAN_POINT('Ctrl Pts',(-17.2304684005269,16.3088931485296,1.39738465216653));
#23676=CARTESIAN_POINT('Ctrl Pts',(-17.2854690953382,16.1789132787142,1.39169874360068));
#23677=CARTESIAN_POINT('Ctrl Pts',(-17.32565468021,16.0440680000031,1.38580000000002));
#23678=CARTESIAN_POINT('',(-16.3931641176038,17.1826416311934,1.3858));
#23679=CARTESIAN_POINT('Origin',(-15.5,15.5,1.3858));
#23680=CARTESIAN_POINT('Ctrl Pts',(-16.3931641176044,17.182641631193,1.38579999999996));
#23681=CARTESIAN_POINT('Ctrl Pts',(-16.2723883324171,17.2467507056418,1.3917776655887));
#23682=CARTESIAN_POINT('Ctrl Pts',(-16.1450664179259,17.2976688253463,1.3977148078573));
#23683=CARTESIAN_POINT('Ctrl Pts',(-15.8851785600351,17.3703971986234,1.40915110154527));
#23684=CARTESIAN_POINT('Ctrl Pts',(-15.7535588097723,17.3927389340048,1.41462603221265));
#23685=CARTESIAN_POINT('Ctrl Pts',(-15.3801305916486,17.4164430131056,1.4292914024198));
#23686=CARTESIAN_POINT('Ctrl Pts',(-15.1388459584443,17.3859249483997,1.43859912950402));
#23687=CARTESIAN_POINT('Ctrl Pts',(-14.6723439861098,17.23386825394,1.45959785680879));
#23688=CARTESIAN_POINT('Ctrl Pts',(-14.4525515511058,17.110640943444,1.47061970665662));
#23689=CARTESIAN_POINT('Ctrl Pts',(-14.0707452475483,16.7845360897548,1.49221666138324));
#23690=CARTESIAN_POINT('Ctrl Pts',(-13.9132616040367,16.5839904470103,1.50208134527492));
#23691=CARTESIAN_POINT('Ctrl Pts',(-13.6898378009267,16.1414810943751,1.52143870978214));
#23692=CARTESIAN_POINT('Ctrl Pts',(-13.6228129384099,15.9053796762351,1.53176685580751));
#23693=CARTESIAN_POINT('Ctrl Pts',(-13.580357781213,15.4112880829908,1.55338066128627));
#23694=CARTESIAN_POINT('Ctrl Pts',(-13.6090431492827,15.1576722103972,1.56447496892379));
#23695=CARTESIAN_POINT('Ctrl Pts',(-13.7611758077611,14.6843730255031,1.58517922023149));
#23696=CARTESIAN_POINT('Ctrl Pts',(-13.8800302566413,14.4682765188114,1.59402873094833));
#23697=CARTESIAN_POINT('Ctrl Pts',(-14.1939644866156,14.0915194243571,1.61416230774197));
#23698=CARTESIAN_POINT('Ctrl Pts',(-14.3865682657467,13.9348153522307,1.62488635855805));
#23699=CARTESIAN_POINT('Ctrl Pts',(-14.8263458369783,13.7002975223377,1.64667627385321));
#23700=CARTESIAN_POINT('Ctrl Pts',(-15.0704913068452,13.6269593374867,1.65752952282736));
#23701=CARTESIAN_POINT('Ctrl Pts',(-15.5619293145468,13.5807968238314,1.67715677811531));
#23702=CARTESIAN_POINT('Ctrl Pts',(-15.804120411355,13.6040306004054,1.68621877962558));
#23703=CARTESIAN_POINT('Ctrl Pts',(-16.2743516095945,13.7417859609585,1.70704598188298));
#23704=CARTESIAN_POINT('Ctrl Pts',(-16.4971311158611,13.8578481105359,1.7180242752626));
#23705=CARTESIAN_POINT('Ctrl Pts',(-16.8882752695545,14.1713019326203,1.73969827721722));
#23706=CARTESIAN_POINT('Ctrl Pts',(-17.0518930224525,14.3667173602226,1.74992508137436));
#23707=CARTESIAN_POINT('Ctrl Pts',(-17.288707924895,14.8011847488145,1.76893065392868));
#23708=CARTESIAN_POINT('Ctrl Pts',(-17.3630339890476,15.0342747992455,1.77912706908314));
#23709=CARTESIAN_POINT('Ctrl Pts',(-17.4005657968241,15.3498262737769,1.79293072063744));
#23710=CARTESIAN_POINT('Ctrl Pts',(-17.405,15.4249560243541,1.79621723641079));
#23711=CARTESIAN_POINT('Ctrl Pts',(-17.405,15.5,1.79949999999985));
#23712=CARTESIAN_POINT('Origin',(15.5,15.5,-1.713));
#23713=CARTESIAN_POINT('',(16.0440680000052,17.3256546802097,1.3858));
#23714=CARTESIAN_POINT('Ctrl Pts',(13.595,15.5,1.73699999999994));
#23715=CARTESIAN_POINT('Ctrl Pts',(13.595,15.4699273628645,1.73586073194578));
#23716=CARTESIAN_POINT('Ctrl Pts',(13.5957120893792,15.4398306754848,1.73470497776689));
#23717=CARTESIAN_POINT('Ctrl Pts',(13.6090996130625,15.1576110183613,1.72372058781246));
#23718=CARTESIAN_POINT('Ctrl Pts',(13.6710479482893,14.9103855829078,1.71299977962444));
#23719=CARTESIAN_POINT('Ctrl Pts',(13.8853907466994,14.4592729280394,1.69122172108156));
#23720=CARTESIAN_POINT('Ctrl Pts',(14.0338479961768,14.258837749694,1.68038136320761));
#23721=CARTESIAN_POINT('Ctrl Pts',(14.3956899669362,13.9288953046006,1.65996756073088));
#23722=CARTESIAN_POINT('Ctrl Pts',(14.6044910974772,13.8011967843423,1.651173617783));
#23723=CARTESIAN_POINT('Ctrl Pts',(15.0694642475063,13.6269920348691,1.63083358497329));
#23724=CARTESIAN_POINT('Ctrl Pts',(15.3226988387298,13.5863464627192,1.61975595631083));
#23725=CARTESIAN_POINT('Ctrl Pts',(15.8204761748578,13.6063323454247,1.59798091973478));
#23726=CARTESIAN_POINT('Ctrl Pts',(16.0604000490661,13.6629773403858,1.58748556215787));
#23727=CARTESIAN_POINT('Ctrl Pts',(16.5099074456352,13.8656749614721,1.56782207149429));
#23728=CARTESIAN_POINT('Ctrl Pts',(16.7144958138179,14.0113953950104,1.55849700337696));
#23729=CARTESIAN_POINT('Ctrl Pts',(17.0574581079868,14.3747233338918,1.53723137030345));
#23730=CARTESIAN_POINT('Ctrl Pts',(17.1919121858965,14.589311632061,1.52616111848699));
#23731=CARTESIAN_POINT('Ctrl Pts',(17.3666878890906,15.049604046309,1.50490071710883));
#23732=CARTESIAN_POINT('Ctrl Pts',(17.4086874588649,15.2896536370031,1.49504938859915));
#23733=CARTESIAN_POINT('Ctrl Pts',(17.4006271908752,15.7834258159291,1.4761670883093));
#23734=CARTESIAN_POINT('Ctrl Pts',(17.3464078918416,16.0324150395295,1.46554851252527));
#23735=CARTESIAN_POINT('Ctrl Pts',(17.1459365086778,16.4906249151765,1.44380498303461));
#23736=CARTESIAN_POINT('Ctrl Pts',(17.0032377368195,16.6961304680377,1.43289849067567));
#23737=CARTESIAN_POINT('Ctrl Pts',(16.7155289154758,16.9747253572526,1.41605139259624));
#23738=CARTESIAN_POINT('Ctrl Pts',(16.5934948001371,17.0673550935378,1.40987305653158));
#23739=CARTESIAN_POINT('Ctrl Pts',(16.3302699480926,17.2212965079858,1.39828383511302));
#23740=CARTESIAN_POINT('Ctrl Pts',(16.1900656890046,17.2821455371494,1.3921866005688));
#23741=CARTESIAN_POINT('Ctrl Pts',(16.0440680000051,17.3256546802094,1.38580000000015));
#23742=CARTESIAN_POINT('',(17.1826416311923,16.393164117606,1.3858));
#23743=CARTESIAN_POINT('Origin',(15.5,15.5,1.3858));
#23744=CARTESIAN_POINT('Ctrl Pts',(17.1826416311919,16.3931641176066,1.38579999999991));
#23745=CARTESIAN_POINT('Ctrl Pts',(17.24665362517,16.2725712233782,1.39176861360038));
#23746=CARTESIAN_POINT('Ctrl Pts',(17.2975148512645,16.1454515121981,1.39769685123167));
#23747=CARTESIAN_POINT('Ctrl Pts',(17.3702201242742,15.8859713444243,1.40911719478266));
#23748=CARTESIAN_POINT('Ctrl Pts',(17.3925920222397,15.7545528306264,1.41458516155685));
#23749=CARTESIAN_POINT('Ctrl Pts',(17.4165176652001,15.3813317017817,1.42924753252314));
#23750=CARTESIAN_POINT('Ctrl Pts',(17.3861509933302,15.1400292056562,1.43854935939874));
#23751=CARTESIAN_POINT('Ctrl Pts',(17.234392581011,14.6734480786425,1.45954456128325));
#23752=CARTESIAN_POINT('Ctrl Pts',(17.1113140091714,14.4535910385712,1.47056560536997));
#23753=CARTESIAN_POINT('Ctrl Pts',(16.7854343398408,14.0715436685454,1.49216676733657));
#23754=CARTESIAN_POINT('Ctrl Pts',(16.5849420836776,13.9139037708014,1.50203971637447));
#23755=CARTESIAN_POINT('Ctrl Pts',(16.1425255215973,13.6902101009022,1.52139302180229));
#23756=CARTESIAN_POINT('Ctrl Pts',(15.906476643006,13.6230519475303,1.5317188695097));
#23757=CARTESIAN_POINT('Ctrl Pts',(15.4124393942654,13.5803069603505,1.55333029771356));
#23758=CARTESIAN_POINT('Ctrl Pts',(15.1588221439251,13.6088374167553,1.56442466561995));
#23759=CARTESIAN_POINT('Ctrl Pts',(14.6854174034196,13.7606823527963,1.58513353440842));
#23760=CARTESIAN_POINT('Ctrl Pts',(14.4692250920796,13.8794222936253,1.59398495150606));
#23761=CARTESIAN_POINT('Ctrl Pts',(14.0922776263441,14.1931499146905,1.61411486500468));
#23762=CARTESIAN_POINT('Ctrl Pts',(13.935470385775,14.3856511393828,1.62483728718873));
#23763=CARTESIAN_POINT('Ctrl Pts',(13.7006976935149,14.8252774899478,1.64662704807638));
#23764=CARTESIAN_POINT('Ctrl Pts',(13.6272144555416,15.0693799656232,1.65748184090438));
#23765=CARTESIAN_POINT('Ctrl Pts',(13.5978121805544,15.3804101463148,1.66990796405906));
#23766=CARTESIAN_POINT('Ctrl Pts',(13.595,15.440236933533,1.67223594340449));
#23767=CARTESIAN_POINT('Ctrl Pts',(13.595,15.4999999999999,1.67449999999978));
#23768=CARTESIAN_POINT('Origin',(15.5,-15.5,-1.713));
#23769=CARTESIAN_POINT('',(17.32565468021,-16.0440680000029,1.3858));
#23770=CARTESIAN_POINT('Ctrl Pts',(13.595,-15.5,1.61199999999989));
#23771=CARTESIAN_POINT('Ctrl Pts',(13.595,-15.536390811308,1.61040810099254));
#23772=CARTESIAN_POINT('Ctrl Pts',(13.5960427336748,-15.5728179794516,1.60881461157244));
#23773=CARTESIAN_POINT('Ctrl Pts',(13.6121171890736,-15.8526811699943,1.59657212729673));
#23774=CARTESIAN_POINT('Ctrl Pts',(13.6727140897741,-16.091211600863,1.58613772524647));
#23775=CARTESIAN_POINT('Ctrl Pts',(13.8832384335276,-16.538105979127,1.56658853984559));
#23776=CARTESIAN_POINT('Ctrl Pts',(14.033346321881,-16.7411793436505,1.55708178792549));
#23777=CARTESIAN_POINT('Ctrl Pts',(14.4036422324888,-17.0778758818557,1.53568922735653));
#23778=CARTESIAN_POINT('Ctrl Pts',(14.6202507282492,-17.208137086823,1.52463415025734));
#23779=CARTESIAN_POINT('Ctrl Pts',(15.0829186266929,-17.3743776635122,1.50347043888761));
#23780=CARTESIAN_POINT('Ctrl Pts',(15.3234036970219,-17.412073738625,1.49384487112439));
#23781=CARTESIAN_POINT('Ctrl Pts',(15.8167315474728,-17.3953646239746,1.47479023384486));
#23782=CARTESIAN_POINT('Ctrl Pts',(16.0647559828302,-17.3367775777424,1.46411267545049));
#23783=CARTESIAN_POINT('Ctrl Pts',(16.5190134240267,-17.1284495137126,1.44234703608263));
#23784=CARTESIAN_POINT('Ctrl Pts',(16.721677544645,-16.9824805684246,1.43147666208721));
#23785=CARTESIAN_POINT('Ctrl Pts',(16.9912576203034,-16.6944874199144,1.41496486120666));
#23786=CARTESIAN_POINT('Ctrl Pts',(17.0789552713108,-16.575884089482,1.40906404590897));
#23787=CARTESIAN_POINT('Ctrl Pts',(17.2254012201848,-16.3207782997712,1.39790456254455));
#23788=CARTESIAN_POINT('Ctrl Pts',(17.28362719674,-16.1850938862784,1.39196911138564));
#23789=CARTESIAN_POINT('Ctrl Pts',(17.3256546802103,-16.0440680000022,1.38579999999998));
#23790=CARTESIAN_POINT('',(16.3931641176036,-17.1826416311934,1.3858));
#23791=CARTESIAN_POINT('Origin',(15.5,-15.5,1.3858));
#23792=CARTESIAN_POINT('Ctrl Pts',(16.3931641176036,-17.1826416311935,1.3858));
#23793=CARTESIAN_POINT('Ctrl Pts',(16.2759070945517,-17.2448829091848,1.39160350829969));
#23794=CARTESIAN_POINT('Ctrl Pts',(16.1524707830423,-17.2946955088363,1.39736926863837));
#23795=CARTESIAN_POINT('Ctrl Pts',(15.9004262675809,-17.3669323901444,1.40849767607179));
#23796=CARTESIAN_POINT('Ctrl Pts',(15.7726845826618,-17.3898214067908,1.41383766087422));
#23797=CARTESIAN_POINT('Ctrl Pts',(15.4032482695823,-17.4177501133806,1.428444204422));
#23798=CARTESIAN_POINT('Ctrl Pts',(15.1616129530288,-17.3901425823975,1.43764437829329));
#23799=CARTESIAN_POINT('Ctrl Pts',(14.6936015261495,-17.2438130087807,1.45857502447647));
#23800=CARTESIAN_POINT('Ctrl Pts',(14.4725857350829,-17.1234469739703,1.46958063721079));
#23801=CARTESIAN_POINT('Ctrl Pts',(14.0861584798649,-16.8016835834113,1.49125769386053));
#23802=CARTESIAN_POINT('Ctrl Pts',(13.9256664401826,-16.6021652185474,1.50128629840102));
#23803=CARTESIAN_POINT('Ctrl Pts',(13.6970710454032,-16.1614416400184,1.52056554505583));
#23804=CARTESIAN_POINT('Ctrl Pts',(13.6275006434827,-15.9263591104517,1.53084912027747));
#23805=CARTESIAN_POINT('Ctrl Pts',(13.5979805133499,-15.6231241110188,1.54411399339352));
#23806=CARTESIAN_POINT('Ctrl Pts',(13.595,-15.561525211074,1.5468086084393));
#23807=CARTESIAN_POINT('Ctrl Pts',(13.595,-15.5,1.54949999999984));
#23808=CARTESIAN_POINT('Origin',(-15.5,-15.5,-1.713));
#23809=CARTESIAN_POINT('',(-16.0440680000367,-17.3256546802026,1.3858));
#23810=CARTESIAN_POINT('Ctrl Pts',(-17.405,-15.5,1.48699999999984));
#23811=CARTESIAN_POINT('Ctrl Pts',(-17.405,-15.5186265321859,1.48629435476548));
#23812=CARTESIAN_POINT('Ctrl Pts',(-17.4047268139491,-15.5372634348496,
1.48558234145932));
#23813=CARTESIAN_POINT('Ctrl Pts',(-17.3967729604905,-15.8081805965321,
1.47514498052024));
#23814=CARTESIAN_POINT('Ctrl Pts',(-17.3393068162074,-16.0564605136505,
1.46448226015211));
#23815=CARTESIAN_POINT('Ctrl Pts',(-17.1329906165269,-16.5117466633973,
1.44272165334931));
#23816=CARTESIAN_POINT('Ctrl Pts',(-16.9878569403636,-16.7151458811511,
1.43184170025367));
#23817=CARTESIAN_POINT('Ctrl Pts',(-16.699905912139,-16.9870454132385,1.41524295063963));
#23818=CARTESIAN_POINT('Ctrl Pts',(-16.5804094676046,-17.0759978712803,
1.40926200645678));
#23819=CARTESIAN_POINT('Ctrl Pts',(-16.3232094764869,-17.2243558857854,
1.39801091323203));
#23820=CARTESIAN_POINT('Ctrl Pts',(-16.1863597090227,-17.2832499656779,
1.3920244842091));
#23821=CARTESIAN_POINT('Ctrl Pts',(-16.0440680000359,-17.3256546802002,
1.38580000000145));
#23822=CARTESIAN_POINT('',(-17.1826416312037,-16.3931641175801,1.3858));
#23823=CARTESIAN_POINT('Origin',(-15.5,-15.5,1.3858));
#23824=CARTESIAN_POINT('Ctrl Pts',(-17.1826416312051,-16.3931641175817,
1.38580000000111));
#23825=CARTESIAN_POINT('Ctrl Pts',(-17.243819155217,-16.2779111122602,1.39150432163177));
#23826=CARTESIAN_POINT('Ctrl Pts',(-17.2929918586721,-16.1566832784271,
1.39717242029638));
#23827=CARTESIAN_POINT('Ctrl Pts',(-17.3649044547202,-15.9091049784493,
1.40812453732309));
#23828=CARTESIAN_POINT('Ctrl Pts',(-17.3880739083904,-15.783577621763,1.41338676858269));
#23829=CARTESIAN_POINT('Ctrl Pts',(-17.4028534332033,-15.6044814179587,
1.42049488864491));
#23830=CARTESIAN_POINT('Ctrl Pts',(-17.405,-15.5522133244187,1.42252195689568));
#23831=CARTESIAN_POINT('Ctrl Pts',(-17.405,-15.5000000000001,1.42449999999991));
#23832=CARTESIAN_POINT('Origin',(0.,0.,-37.019));
#23833=CARTESIAN_POINT('',(-2.62699999999999,-3.21714714136009E-16,1.3858));
#23834=CARTESIAN_POINT('Origin',(0.,0.,1.3858));
#23835=CARTESIAN_POINT('',(-2.62699999999999,-3.21714714136009E-16,6.669));
#23836=CARTESIAN_POINT('',(-2.62699999999999,-3.21714714136008E-16,-37.019));
#23837=CARTESIAN_POINT('Origin',(0.,0.,6.669));
#23838=CARTESIAN_POINT('Origin',(0.,0.,6.669));
#23839=CARTESIAN_POINT('',(-3.76999999999999,-4.61691843278552E-16,6.669));
#23840=CARTESIAN_POINT('Origin',(0.,0.,6.669));
#23841=CARTESIAN_POINT('',(-3.76999999999999,-4.61691843278552E-16,13.019));
#23842=CARTESIAN_POINT('',(-3.76999999999999,-4.61691843278551E-16,6.669));
#23843=CARTESIAN_POINT('Origin',(0.,0.,13.019));
#23844=CARTESIAN_POINT('Origin',(0.,0.,11.495));
#23845=CARTESIAN_POINT('',(11.493,-1.40748656626005E-15,10.987));
#23846=CARTESIAN_POINT('Origin',(0.,0.,10.987));
#23847=CARTESIAN_POINT('',(10.985,-1.34527450886337E-15,11.495));
#23848=CARTESIAN_POINT('',(10.985,-1.34527450886337E-15,11.495));
#23849=CARTESIAN_POINT('Origin',(0.,0.,11.495));
#23850=CARTESIAN_POINT('Origin',(0.,0.,13.019));
#23851=CARTESIAN_POINT('',(10.985,-1.34527450886337E-15,13.019));
#23852=CARTESIAN_POINT('',(10.985,-1.34527450886337E-15,13.019));
#23853=CARTESIAN_POINT('Origin',(0.,0.,13.019));
#23854=CARTESIAN_POINT('Origin',(-15.4999999999999,-15.5000000000001,10.987));
#23855=CARTESIAN_POINT('',(-15.499999994708,-17.1672595260839,10.4992595260838));
#23856=CARTESIAN_POINT('Ctrl Pts',(-13.5949999999992,-15.5000000000296,
10.7370000000007));
#23857=CARTESIAN_POINT('Ctrl Pts',(-13.6008497881007,-15.2564355648758,
10.7311502118955));
#23858=CARTESIAN_POINT('Ctrl Pts',(-13.650944651317,-15.0667953438396,10.7259167101349));
#23859=CARTESIAN_POINT('Ctrl Pts',(-13.7548661865755,-14.7648541062214,
10.7172082071437));
#23860=CARTESIAN_POINT('Ctrl Pts',(-13.8368618391017,-14.6050214267038,
10.7121852577521));
#23861=CARTESIAN_POINT('Ctrl Pts',(-14.073970488167,-14.2704423655218,10.7006604618175));
#23862=CARTESIAN_POINT('Ctrl Pts',(-14.2414766707786,-14.1080191324474,
10.6942562020715));
#23863=CARTESIAN_POINT('Ctrl Pts',(-14.6374778586095,-13.8453173047647,
10.681998762105));
#23864=CARTESIAN_POINT('Ctrl Pts',(-14.8639328565342,-13.7520840601426,
10.6760021091648));
#23865=CARTESIAN_POINT('Ctrl Pts',(-15.3364039021795,-13.6614771916233,
10.6624990364387));
#23866=CARTESIAN_POINT('Ctrl Pts',(-15.5758065143609,-13.6626363666899,
10.655582285966));
#23867=CARTESIAN_POINT('Ctrl Pts',(-16.062912999776,-13.7609513162477,10.6413472559504));
#23868=CARTESIAN_POINT('Ctrl Pts',(-16.2635040620812,-13.8578641877347,
10.6354098660481));
#23869=CARTESIAN_POINT('Ctrl Pts',(-16.6035611311394,-14.0672823720547,
10.6252403230972));
#23870=CARTESIAN_POINT('Ctrl Pts',(-16.7766690301586,-14.2283948798923,
10.6186368111943));
#23871=CARTESIAN_POINT('Ctrl Pts',(-17.0457728351311,-14.6023972130674,
10.6050799280797));
#23872=CARTESIAN_POINT('Ctrl Pts',(-17.1416118806701,-14.8099919664234,
10.5982690748888));
#23873=CARTESIAN_POINT('Ctrl Pts',(-17.2495576082356,-15.2485979049578,
10.5851458477462));
#23874=CARTESIAN_POINT('Ctrl Pts',(-17.2617643752449,-15.4776646621072,
10.5793320921415));
#23875=CARTESIAN_POINT('Ctrl Pts',(-17.1990672566599,-15.9104000162702,
10.567155287325));
#23876=CARTESIAN_POINT('Ctrl Pts',(-17.1306302329843,-16.1118828633918,
10.5608366679581));
#23877=CARTESIAN_POINT('Ctrl Pts',(-16.9166251729184,-16.4935678846234,
10.5474332016197));
#23878=CARTESIAN_POINT('Ctrl Pts',(-16.7678269425302,-16.6673647634593,
10.5404564545235));
#23879=CARTESIAN_POINT('Ctrl Pts',(-16.4380554775456,-16.9263243699996,
10.5282450923036));
#23880=CARTESIAN_POINT('Ctrl Pts',(-16.2402954425981,-17.0406955315939,
10.5224302623227));
#23881=CARTESIAN_POINT('Ctrl Pts',(-15.8342695060709,-17.1526817172524,
10.5098001955615));
#23882=CARTESIAN_POINT('Ctrl Pts',(-15.6670883208016,-17.1725541316431,
10.5045541305823));
#23883=CARTESIAN_POINT('Ctrl Pts',(-15.4999999894162,-17.1672595260839,
10.4992595260838));
#23884=CARTESIAN_POINT('',(-14.5577749122402,-14.2313898004749,10.4122404735808));
#23885=CARTESIAN_POINT('Ctrl Pts',(-14.5577749122402,-14.2313898004749,
10.4122404735809));
#23886=CARTESIAN_POINT('Ctrl Pts',(-14.3868051820039,-14.3303760686904,
10.4347161538326));
#23887=CARTESIAN_POINT('Ctrl Pts',(-14.235113371322,-14.4592007076174,10.4582727675319));
#23888=CARTESIAN_POINT('Ctrl Pts',(-13.98017849664,-14.7697452365794,10.5059067908485));
#23889=CARTESIAN_POINT('Ctrl Pts',(-13.8810021159392,-14.9504857681989,
10.5295757840843));
#23890=CARTESIAN_POINT('Ctrl Pts',(-13.7335179124492,-15.400735819956,10.5809089218014));
#23891=CARTESIAN_POINT('Ctrl Pts',(-13.7252310950464,-15.6393119361012,
10.6025326156877));
#23892=CARTESIAN_POINT('Ctrl Pts',(-13.7544578969404,-16.0071202507761,
10.6406359197722));
#23893=CARTESIAN_POINT('Ctrl Pts',(-13.7957662195545,-16.1857710732841,
10.6600613989279));
#23894=CARTESIAN_POINT('Ctrl Pts',(-13.9306559184097,-16.5282411322908,
10.6990893282686));
#23895=CARTESIAN_POINT('Ctrl Pts',(-14.0244109493983,-16.6897880532903,
10.7184707369832));
#23896=CARTESIAN_POINT('Ctrl Pts',(-14.1407339385554,-16.8346987578457,
10.7369999999972));
#23897=CARTESIAN_POINT('',(-13.9406917842496,-15.2436450846258,10.4122404735808));
#23898=CARTESIAN_POINT('Origin',(-15.5,-15.5000000000001,10.4122404735808));
#23899=CARTESIAN_POINT('Ctrl Pts',(-15.4999999894162,-17.1672595260839,
10.4992595260838));
#23900=CARTESIAN_POINT('Ctrl Pts',(-15.4589933982957,-17.1659601311859,
10.4979601314461));
#23901=CARTESIAN_POINT('Ctrl Pts',(-15.4179923936843,-17.1631450533092,
10.4966578716341));
#23902=CARTESIAN_POINT('Ctrl Pts',(-15.1578207074785,-17.1355603869698,
10.4883749005524));
#23903=CARTESIAN_POINT('Ctrl Pts',(-14.9453351143306,-17.0690262279152,
10.4815187112078));
#23904=CARTESIAN_POINT('Ctrl Pts',(-14.5384028688187,-16.8460543494088,
10.468240993816));
#23905=CARTESIAN_POINT('Ctrl Pts',(-14.384838579944,-16.7012184908713,10.4620910771073));
#23906=CARTESIAN_POINT('Ctrl Pts',(-14.1456891975424,-16.4090783981286,
10.4500509032653));
#23907=CARTESIAN_POINT('Ctrl Pts',(-14.046850578254,-16.2259194616222,10.4432455275598));
#23908=CARTESIAN_POINT('Ctrl Pts',(-13.9464878894178,-15.9056854194768,
10.4323954781049));
#23909=CARTESIAN_POINT('Ctrl Pts',(-13.9227846102421,-15.7780439261845,
10.4283074238932));
#23910=CARTESIAN_POINT('Ctrl Pts',(-13.9059874790046,-15.513966292252,10.4203309872474));
#23911=CARTESIAN_POINT('Ctrl Pts',(-13.914345653721,-15.3775884074119,10.4165086268911));
#23912=CARTESIAN_POINT('Ctrl Pts',(-13.94069178425,-15.2436450846239,10.4122404735808));
#23913=CARTESIAN_POINT('',(-15.4999999999999,-17.6550000000001,10.987));
#23914=CARTESIAN_POINT('',(-15.4999999999999,-17.6550000000001,10.987));
#23915=CARTESIAN_POINT('Origin',(-15.5,-15.5,10.987));
#23916=CARTESIAN_POINT('Origin',(15.5,-15.5,10.987));
#23917=CARTESIAN_POINT('',(17.1672595260838,-15.4999999947082,10.4992595260838));
#23918=CARTESIAN_POINT('Ctrl Pts',(15.5000000000296,-13.5949999999993,10.7370000000007));
#23919=CARTESIAN_POINT('Ctrl Pts',(15.2564355648662,-13.600849788101,10.7311502118952));
#23920=CARTESIAN_POINT('Ctrl Pts',(15.0667953438228,-13.6509446513211,10.7259167101345));
#23921=CARTESIAN_POINT('Ctrl Pts',(14.7648541061942,-13.7548661865872,10.7172082071429));
#23922=CARTESIAN_POINT('Ctrl Pts',(14.6050214266715,-13.8368618391195,10.712185257751));
#23923=CARTESIAN_POINT('Ctrl Pts',(14.27044236549,-14.0739704881962,10.7006604618163));
#23924=CARTESIAN_POINT('Ctrl Pts',(14.1080191324201,-14.2414766708108,10.6942562020704));
#23925=CARTESIAN_POINT('Ctrl Pts',(13.8453173047464,-14.6374778586467,10.681998762104));
#23926=CARTESIAN_POINT('Ctrl Pts',(13.7520840601298,-14.8639328565725,10.6760021091637));
#23927=CARTESIAN_POINT('Ctrl Pts',(13.661477191621,-15.336403902218,10.6624990364376));
#23928=CARTESIAN_POINT('Ctrl Pts',(13.6626363666926,-15.5758065143984,10.6555822859649));
#23929=CARTESIAN_POINT('Ctrl Pts',(13.7609513162606,-16.0629129998141,10.6413472559492));
#23930=CARTESIAN_POINT('Ctrl Pts',(13.8578641877541,-16.2635040621222,10.635409866047));
#23931=CARTESIAN_POINT('Ctrl Pts',(14.0672823720874,-16.6035611311796,10.6252403230958));
#23932=CARTESIAN_POINT('Ctrl Pts',(14.2283948799295,-16.7766690301937,10.6186368111928));
#23933=CARTESIAN_POINT('Ctrl Pts',(14.6023972131106,-17.0457728351544,10.6050799280782));
#23934=CARTESIAN_POINT('Ctrl Pts',(14.8099919664681,-17.1416118806874,10.5982690748874));
#23935=CARTESIAN_POINT('Ctrl Pts',(15.2485979050077,-17.2495576082419,10.5851458477448));
#23936=CARTESIAN_POINT('Ctrl Pts',(15.4776646621617,-17.2617643752449,10.57933209214));
#23937=CARTESIAN_POINT('Ctrl Pts',(15.9104000163284,-17.1990672566442,10.5671552873232));
#23938=CARTESIAN_POINT('Ctrl Pts',(16.1118828634489,-17.1306302329612,10.5608366679562));
#23939=CARTESIAN_POINT('Ctrl Pts',(16.4935678846754,-16.9166251728798,10.5474332016177));
#23940=CARTESIAN_POINT('Ctrl Pts',(16.667364763507,-16.767826942484,10.5404564545215));
#23941=CARTESIAN_POINT('Ctrl Pts',(16.9263243700374,-16.4380554774851,10.5282450923016));
#23942=CARTESIAN_POINT('Ctrl Pts',(17.0406955316219,-16.2402954425337,10.5224302623207));
#23943=CARTESIAN_POINT('Ctrl Pts',(17.1526817172575,-15.8342695060273,10.5098001955601));
#23944=CARTESIAN_POINT('Ctrl Pts',(17.1725541316423,-15.6670883207797,10.5045541305816));
#23945=CARTESIAN_POINT('Ctrl Pts',(17.1672595260838,-15.4999999894163,10.4992595260838));
#23946=CARTESIAN_POINT('',(14.2313898004749,-14.5577749122403,10.4122404735808));
#23947=CARTESIAN_POINT('Ctrl Pts',(14.2313898004748,-14.5577749122403,10.4122404735809));
#23948=CARTESIAN_POINT('Ctrl Pts',(14.330374396146,-14.3868080708335,10.4347157740671));
#23949=CARTESIAN_POINT('Ctrl Pts',(14.4592032863654,-14.2351112543341,10.4582731630844));
#23950=CARTESIAN_POINT('Ctrl Pts',(14.7697452366637,-13.9801784965913,10.5059067908598));
#23951=CARTESIAN_POINT('Ctrl Pts',(14.9504857682593,-13.8810021159152,10.5295757840915));
#23952=CARTESIAN_POINT('Ctrl Pts',(15.400735820047,-13.7335179124251,10.5809089218113));
#23953=CARTESIAN_POINT('Ctrl Pts',(15.6393119362485,-13.72523109504,10.6025326157022));
#23954=CARTESIAN_POINT('Ctrl Pts',(16.0071202509296,-13.7544578969706,10.6406359197886));
#23955=CARTESIAN_POINT('Ctrl Pts',(16.1857710734102,-13.7957662195931,10.6600613989418));
#23956=CARTESIAN_POINT('Ctrl Pts',(16.5282411323567,-13.9306559184475,10.6990893282765));
#23957=CARTESIAN_POINT('Ctrl Pts',(16.689788053325,-14.0244109494249,10.7184707369876));
#23958=CARTESIAN_POINT('Ctrl Pts',(16.8346987578547,-14.140733938563,10.7369999999983));
#23959=CARTESIAN_POINT('',(15.2436450846258,-13.9406917842497,10.4122404735808));
#23960=CARTESIAN_POINT('Origin',(15.5,-15.5,10.4122404735808));
#23961=CARTESIAN_POINT('Ctrl Pts',(17.1672595260838,-15.4999999894163,10.4992595260838));
#23962=CARTESIAN_POINT('Ctrl Pts',(17.1659601311851,-15.4589933982724,10.4979601314454));
#23963=CARTESIAN_POINT('Ctrl Pts',(17.1631450533059,-15.4179923936375,10.4966578716326));
#23964=CARTESIAN_POINT('Ctrl Pts',(17.135560386953,-15.1578207074097,10.4883749005502));
#23965=CARTESIAN_POINT('Ctrl Pts',(17.0690262278895,-14.9453351142648,10.4815187112057));
#23966=CARTESIAN_POINT('Ctrl Pts',(16.8460543493517,-14.5384028687359,10.4682409938133));
#23967=CARTESIAN_POINT('Ctrl Pts',(16.7012184908016,-14.3848385798802,10.4620910771043));
#23968=CARTESIAN_POINT('Ctrl Pts',(16.4090783980845,-14.1456891975148,10.4500509032636));
#23969=CARTESIAN_POINT('Ctrl Pts',(16.2259194615737,-14.0468505782317,10.4432455275581));
#23970=CARTESIAN_POINT('Ctrl Pts',(15.9056854194317,-13.9464878894083,10.4323954781035));
#23971=CARTESIAN_POINT('Ctrl Pts',(15.7780439261473,-13.9227846102375,10.428307423892));
#23972=CARTESIAN_POINT('Ctrl Pts',(15.5139662922323,-13.9059874790058,10.4203309872468));
#23973=CARTESIAN_POINT('Ctrl Pts',(15.3775884074022,-13.914345653723,10.4165086268908));
#23974=CARTESIAN_POINT('Ctrl Pts',(15.2436450846239,-13.9406917842501,10.4122404735808));
#23975=CARTESIAN_POINT('',(17.655,-15.5,10.987));
#23976=CARTESIAN_POINT('',(17.655,-15.5,10.987));
#23977=CARTESIAN_POINT('Origin',(15.5,-15.5,10.987));
#23978=CARTESIAN_POINT('Origin',(15.4999999999998,15.5000000000002,10.987));
#23979=CARTESIAN_POINT('',(15.4999999947079,17.167259526084,10.4992595260838));
#23980=CARTESIAN_POINT('Ctrl Pts',(13.5949999999991,15.5000000000298,10.7370000000007));
#23981=CARTESIAN_POINT('Ctrl Pts',(13.600849788101,15.2564355648587,10.731150211895));
#23982=CARTESIAN_POINT('Ctrl Pts',(13.6509446513241,15.0667953438098,10.7259167101341));
#23983=CARTESIAN_POINT('Ctrl Pts',(13.7548661865961,14.7648541061731,10.7172082071422));
#23984=CARTESIAN_POINT('Ctrl Pts',(13.8368618391331,14.6050214266467,10.7121852577502));
#23985=CARTESIAN_POINT('Ctrl Pts',(14.0739704882185,14.2704423654658,10.7006604618154));
#23986=CARTESIAN_POINT('Ctrl Pts',(14.2414766708351,14.1080191323993,10.6942562020695));
#23987=CARTESIAN_POINT('Ctrl Pts',(14.6374778586748,13.8453173047327,10.6819987621032));
#23988=CARTESIAN_POINT('Ctrl Pts',(14.8639328566015,13.7520840601203,10.6760021091628));
#23989=CARTESIAN_POINT('Ctrl Pts',(15.3364039022473,13.6614771916195,10.6624990364368));
#23990=CARTESIAN_POINT('Ctrl Pts',(15.5758065144269,13.6626363666949,10.655582285964));
#23991=CARTESIAN_POINT('Ctrl Pts',(16.0629129998439,13.7609513162709,10.6413472559484));
#23992=CARTESIAN_POINT('Ctrl Pts',(16.2635040621546,13.8578641877698,10.6354098660461));
#23993=CARTESIAN_POINT('Ctrl Pts',(16.6035611312114,14.0672823721137,10.6252403230947));
#23994=CARTESIAN_POINT('Ctrl Pts',(16.7766690302213,14.2283948799594,10.6186368111917));
#23995=CARTESIAN_POINT('Ctrl Pts',(17.0457728351728,14.6023972131454,10.605079928077));
#23996=CARTESIAN_POINT('Ctrl Pts',(17.1416118807008,14.8099919665041,10.5982690748862));
#23997=CARTESIAN_POINT('Ctrl Pts',(17.2495576082467,15.2485979050477,10.5851458477437));
#23998=CARTESIAN_POINT('Ctrl Pts',(17.2617643752446,15.4776646622055,10.5793320921389));
#23999=CARTESIAN_POINT('Ctrl Pts',(17.1990672566315,15.9104000163754,10.5671552873218));
#24000=CARTESIAN_POINT('Ctrl Pts',(17.1306302329423,16.111882863495,10.5608366679547));
#24001=CARTESIAN_POINT('Ctrl Pts',(16.9166251728486,16.4935678847174,10.5474332016161));
#24002=CARTESIAN_POINT('Ctrl Pts',(16.7678269424465,16.6673647635456,10.5404564545199));
#24003=CARTESIAN_POINT('Ctrl Pts',(16.4380554774367,16.9263243700677,10.5282450923));
#24004=CARTESIAN_POINT('Ctrl Pts',(16.2402954424824,17.0406955316445,10.5224302623191));
#24005=CARTESIAN_POINT('Ctrl Pts',(15.8342695059919,17.1526817172619,10.509800195559));
#24006=CARTESIAN_POINT('Ctrl Pts',(15.6670883207619,17.1725541316419,10.504554130581));
#24007=CARTESIAN_POINT('Ctrl Pts',(15.4999999894161,17.167259526084,10.4992595260838));
#24008=CARTESIAN_POINT('',(14.5577835109666,14.2313848221087,10.4122393431954));
#24009=CARTESIAN_POINT('Ctrl Pts',(14.5577835109666,14.2313848221087,10.4122393431954));
#24010=CARTESIAN_POINT('Ctrl Pts',(14.3868137807237,14.3303710903281,10.434715023448));
#24011=CARTESIAN_POINT('Ctrl Pts',(14.2351133713102,14.4592007076274,10.4582727675337));
#24012=CARTESIAN_POINT('Ctrl Pts',(13.9801784966279,14.7697452365986,10.5059067908511));
#24013=CARTESIAN_POINT('Ctrl Pts',(13.8810021159297,14.9504857682191,10.5295757840868));
#24014=CARTESIAN_POINT('Ctrl Pts',(13.7335179124459,15.4007358199769,10.5809089218035));
#24015=CARTESIAN_POINT('Ctrl Pts',(13.725231095046,15.6393119361218,10.6025326156897));
#24016=CARTESIAN_POINT('Ctrl Pts',(13.7544578969435,16.0071202507932,10.640635919774));
#24017=CARTESIAN_POINT('Ctrl Pts',(13.7957662195588,16.185771073299,10.6600613989296));
#24018=CARTESIAN_POINT('Ctrl Pts',(13.9306559184154,16.5282411323019,10.69908932827));
#24019=CARTESIAN_POINT('Ctrl Pts',(14.0244109494044,16.6897880532997,10.7184707369844));
#24020=CARTESIAN_POINT('Ctrl Pts',(14.1407339385614,16.8346987578534,10.7369999999982));
#24021=CARTESIAN_POINT('',(13.9406937133188,15.2436352774332,10.4122401610704));
#24022=CARTESIAN_POINT('Origin',(15.4999999999998,15.5000000000002,10.4122404735808));
#24023=CARTESIAN_POINT('Ctrl Pts',(15.4999999894161,17.167259526084,10.4992595260838));
#24024=CARTESIAN_POINT('Ctrl Pts',(15.4589933982536,17.1659601311847,10.4979601314448));
#24025=CARTESIAN_POINT('Ctrl Pts',(15.4179923936001,17.1631450533035,10.4966578716315));
#24026=CARTESIAN_POINT('Ctrl Pts',(15.1578207073548,17.1355603869399,10.4883749005484));
#24027=CARTESIAN_POINT('Ctrl Pts',(14.9453351142122,17.0690262278694,10.481518711204));
#24028=CARTESIAN_POINT('Ctrl Pts',(14.5384028686677,16.8460543493053,10.468240993811));
#24029=CARTESIAN_POINT('Ctrl Pts',(14.3848385798272,16.7012184907442,10.4620910771019));
#24030=CARTESIAN_POINT('Ctrl Pts',(14.1456891974921,16.4090783980489,10.4500509032622));
#24031=CARTESIAN_POINT('Ctrl Pts',(14.0468505782134,16.2259194615347,10.4432455275567));
#24032=CARTESIAN_POINT('Ctrl Pts',(13.9464878894004,15.9056854193956,10.4323954781023));
#24033=CARTESIAN_POINT('Ctrl Pts',(13.9227846102335,15.7780439261173,10.4283074238911));
#24034=CARTESIAN_POINT('Ctrl Pts',(13.9059874790066,15.5139662922165,10.4203309872464));
#24035=CARTESIAN_POINT('Ctrl Pts',(13.9143467252667,15.3775784311783,10.4165083253794));
#24036=CARTESIAN_POINT('Ctrl Pts',(13.9406937133188,15.2436352774332,10.4122401610704));
#24037=CARTESIAN_POINT('',(15.4999999999998,17.6550000000003,10.9870000000001));
#24038=CARTESIAN_POINT('',(15.4999999999998,17.6550000000002,10.987));
#24039=CARTESIAN_POINT('Origin',(15.5,15.5,10.987));
#24040=CARTESIAN_POINT('Origin',(-15.5,15.5,10.987));
#24041=CARTESIAN_POINT('',(-17.1672595260838,15.4999999947082,10.4992595260838));
#24042=CARTESIAN_POINT('Ctrl Pts',(-15.5000000000296,13.5949999999993,10.7370000000007));
#24043=CARTESIAN_POINT('Ctrl Pts',(-15.2564355648662,13.600849788101,10.7311502118952));
#24044=CARTESIAN_POINT('Ctrl Pts',(-15.0667953438228,13.6509446513211,10.7259167101345));
#24045=CARTESIAN_POINT('Ctrl Pts',(-14.7648541061942,13.7548661865872,10.7172082071429));
#24046=CARTESIAN_POINT('Ctrl Pts',(-14.6050214266715,13.8368618391195,10.712185257751));
#24047=CARTESIAN_POINT('Ctrl Pts',(-14.27044236549,14.0739704881962,10.7006604618163));
#24048=CARTESIAN_POINT('Ctrl Pts',(-14.1080191324201,14.2414766708108,10.6942562020704));
#24049=CARTESIAN_POINT('Ctrl Pts',(-13.8453173047464,14.6374778586467,10.681998762104));
#24050=CARTESIAN_POINT('Ctrl Pts',(-13.7520840601298,14.8639328565725,10.6760021091637));
#24051=CARTESIAN_POINT('Ctrl Pts',(-13.661477191621,15.336403902218,10.6624990364376));
#24052=CARTESIAN_POINT('Ctrl Pts',(-13.6626363666926,15.5758065143984,10.6555822859649));
#24053=CARTESIAN_POINT('Ctrl Pts',(-13.7609513162606,16.0629129998141,10.6413472559492));
#24054=CARTESIAN_POINT('Ctrl Pts',(-13.8578641877541,16.2635040621222,10.635409866047));
#24055=CARTESIAN_POINT('Ctrl Pts',(-14.0672823720874,16.6035611311796,10.6252403230958));
#24056=CARTESIAN_POINT('Ctrl Pts',(-14.2283948799295,16.7766690301937,10.6186368111928));
#24057=CARTESIAN_POINT('Ctrl Pts',(-14.6023972131106,17.0457728351544,10.6050799280782));
#24058=CARTESIAN_POINT('Ctrl Pts',(-14.8099919664681,17.1416118806874,10.5982690748874));
#24059=CARTESIAN_POINT('Ctrl Pts',(-15.2485979050077,17.2495576082419,10.5851458477448));
#24060=CARTESIAN_POINT('Ctrl Pts',(-15.4776646621617,17.2617643752449,10.57933209214));
#24061=CARTESIAN_POINT('Ctrl Pts',(-15.9104000163284,17.1990672566442,10.5671552873232));
#24062=CARTESIAN_POINT('Ctrl Pts',(-16.1118828634489,17.1306302329612,10.5608366679562));
#24063=CARTESIAN_POINT('Ctrl Pts',(-16.4935678846754,16.9166251728798,10.5474332016177));
#24064=CARTESIAN_POINT('Ctrl Pts',(-16.667364763507,16.767826942484,10.5404564545215));
#24065=CARTESIAN_POINT('Ctrl Pts',(-16.9263243700374,16.4380554774851,10.5282450923016));
#24066=CARTESIAN_POINT('Ctrl Pts',(-17.0406955316219,16.2402954425337,10.5224302623207));
#24067=CARTESIAN_POINT('Ctrl Pts',(-17.1526817172575,15.8342695060273,10.5098001955601));
#24068=CARTESIAN_POINT('Ctrl Pts',(-17.1725541316423,15.6670883207797,10.5045541305816));
#24069=CARTESIAN_POINT('Ctrl Pts',(-17.1672595260838,15.4999999894163,10.4992595260838));
#24070=CARTESIAN_POINT('',(-14.2313898004749,14.5577749122403,10.4122404735808));
#24071=CARTESIAN_POINT('Ctrl Pts',(-14.2313898004748,14.5577749122403,10.4122404735809));
#24072=CARTESIAN_POINT('Ctrl Pts',(-14.330374396146,14.3868080708335,10.4347157740671));
#24073=CARTESIAN_POINT('Ctrl Pts',(-14.4592032863654,14.2351112543341,10.4582731630844));
#24074=CARTESIAN_POINT('Ctrl Pts',(-14.7697452366637,13.9801784965913,10.5059067908598));
#24075=CARTESIAN_POINT('Ctrl Pts',(-14.9504857682593,13.8810021159152,10.5295757840915));
#24076=CARTESIAN_POINT('Ctrl Pts',(-15.400735820047,13.7335179124251,10.5809089218113));
#24077=CARTESIAN_POINT('Ctrl Pts',(-15.6393119362485,13.72523109504,10.6025326157022));
#24078=CARTESIAN_POINT('Ctrl Pts',(-16.0071202509296,13.7544578969706,10.6406359197886));
#24079=CARTESIAN_POINT('Ctrl Pts',(-16.1857710734102,13.7957662195931,10.6600613989418));
#24080=CARTESIAN_POINT('Ctrl Pts',(-16.5282411323567,13.9306559184475,10.6990893282765));
#24081=CARTESIAN_POINT('Ctrl Pts',(-16.689788053325,14.0244109494249,10.7184707369876));
#24082=CARTESIAN_POINT('Ctrl Pts',(-16.8346987578547,14.140733938563,10.7369999999983));
#24083=CARTESIAN_POINT('',(-15.2436450846258,13.9406917842497,10.4122404735808));
#24084=CARTESIAN_POINT('Origin',(-15.5,15.5,10.4122404735808));
#24085=CARTESIAN_POINT('Ctrl Pts',(-17.1672595260838,15.4999999894163,10.4992595260838));
#24086=CARTESIAN_POINT('Ctrl Pts',(-17.1659601311851,15.4589933982724,10.4979601314454));
#24087=CARTESIAN_POINT('Ctrl Pts',(-17.1631450533059,15.4179923936375,10.4966578716326));
#24088=CARTESIAN_POINT('Ctrl Pts',(-17.135560386953,15.1578207074097,10.4883749005502));
#24089=CARTESIAN_POINT('Ctrl Pts',(-17.0690262278895,14.9453351142648,10.4815187112057));
#24090=CARTESIAN_POINT('Ctrl Pts',(-16.8460543493517,14.5384028687359,10.4682409938133));
#24091=CARTESIAN_POINT('Ctrl Pts',(-16.7012184908016,14.3848385798802,10.4620910771043));
#24092=CARTESIAN_POINT('Ctrl Pts',(-16.4090783980845,14.1456891975148,10.4500509032636));
#24093=CARTESIAN_POINT('Ctrl Pts',(-16.2259194615737,14.0468505782317,10.4432455275581));
#24094=CARTESIAN_POINT('Ctrl Pts',(-15.9056854194317,13.9464878894083,10.4323954781035));
#24095=CARTESIAN_POINT('Ctrl Pts',(-15.7780439261473,13.9227846102375,10.428307423892));
#24096=CARTESIAN_POINT('Ctrl Pts',(-15.5139662922323,13.9059874790058,10.4203309872468));
#24097=CARTESIAN_POINT('Ctrl Pts',(-15.3775884074022,13.914345653723,10.4165086268908));
#24098=CARTESIAN_POINT('Ctrl Pts',(-15.2436450846239,13.9406917842501,10.4122404735808));
#24099=CARTESIAN_POINT('',(-17.655,15.5,10.987));
#24100=CARTESIAN_POINT('',(-17.655,15.5,10.987));
#24101=CARTESIAN_POINT('Origin',(-15.5,15.5,10.987));
#24102=CARTESIAN_POINT('Ctrl Pts',(-15.5,17.0802317716412,11.1745050240672));
#24103=CARTESIAN_POINT('Ctrl Pts',(-16.4123472387391,17.0802317716412,11.1328383574005));
#24104=CARTESIAN_POINT('Ctrl Pts',(-16.8685208581086,16.2901158858206,11.0911716907338));
#24105=CARTESIAN_POINT('Ctrl Pts',(-17.3246944774781,15.5,11.0495050240672));
#24106=CARTESIAN_POINT('Ctrl Pts',(-16.8685208581086,14.7098841141794,11.0078383574005));
#24107=CARTESIAN_POINT('Ctrl Pts',(-16.4123472387391,13.9197682283588,10.9661716907338));
#24108=CARTESIAN_POINT('Ctrl Pts',(-15.5,13.9197682283588,10.9245050240672));
#24109=CARTESIAN_POINT('Ctrl Pts',(-14.5876527612609,13.9197682283588,10.8828383574005));
#24110=CARTESIAN_POINT('Ctrl Pts',(-14.1314791418914,14.7098841141794,10.8411716907338));
#24111=CARTESIAN_POINT('Ctrl Pts',(-13.6753055225219,15.5,10.7995050240672));
#24112=CARTESIAN_POINT('Ctrl Pts',(-14.1314791418914,16.2901158858206,10.7578383574005));
#24113=CARTESIAN_POINT('Ctrl Pts',(-14.5876527612609,17.0802317716412,10.7161716907338));
#24114=CARTESIAN_POINT('Ctrl Pts',(-15.5,17.0802317716412,10.6745050240672));
#24115=CARTESIAN_POINT('Ctrl Pts',(-16.4123472387391,17.0802317716412,10.6328383574005));
#24116=CARTESIAN_POINT('Ctrl Pts',(-16.8685208581086,16.2901158858206,10.5911716907338));
#24117=CARTESIAN_POINT('Ctrl Pts',(-17.3246944774781,15.5,10.5495050240672));
#24118=CARTESIAN_POINT('Ctrl Pts',(-16.8685208581086,14.7098841141794,10.5078383574005));
#24119=CARTESIAN_POINT('Ctrl Pts',(-16.4123472387391,13.9197682283588,10.4661716907338));
#24120=CARTESIAN_POINT('Ctrl Pts',(-15.5,13.9197682283588,10.4245050240672));
#24121=CARTESIAN_POINT('Ctrl Pts',(-14.5876527612609,13.9197682283588,10.3828383574005));
#24122=CARTESIAN_POINT('Ctrl Pts',(-14.1314791418914,14.7098841141794,10.3411716907338));
#24123=CARTESIAN_POINT('Ctrl Pts',(-13.6753055225219,15.5,10.2995050240672));
#24124=CARTESIAN_POINT('Ctrl Pts',(-14.1314791418914,16.2901158858206,10.2578383574005));
#24125=CARTESIAN_POINT('Ctrl Pts',(-14.5876527612609,17.0802317716412,10.2161716907338));
#24126=CARTESIAN_POINT('Ctrl Pts',(-15.5,17.0802317716412,10.1745050240672));
#24127=CARTESIAN_POINT('Ctrl Pts',(-16.4123472387391,17.0802317716412,10.1328383574005));
#24128=CARTESIAN_POINT('Ctrl Pts',(-16.8685208581086,16.2901158858206,10.0911716907338));
#24129=CARTESIAN_POINT('Ctrl Pts',(-17.3246944774781,15.5,10.0495050240672));
#24130=CARTESIAN_POINT('Ctrl Pts',(-16.8685208581086,14.7098841141794,10.0078383574005));
#24131=CARTESIAN_POINT('Ctrl Pts',(-16.4123472387391,13.9197682283588,9.96617169073382));
#24132=CARTESIAN_POINT('Ctrl Pts',(-15.5,13.9197682283588,9.92450502406715));
#24133=CARTESIAN_POINT('Ctrl Pts',(-14.5876527612609,13.9197682283588,9.88283835740048));
#24134=CARTESIAN_POINT('Ctrl Pts',(-14.1314791418914,14.7098841141794,9.84117169073382));
#24135=CARTESIAN_POINT('Ctrl Pts',(-13.6753055225219,15.5,9.79950502406715));
#24136=CARTESIAN_POINT('Ctrl Pts',(-14.1314791418914,16.2901158858206,9.75783835740048));
#24137=CARTESIAN_POINT('Ctrl Pts',(-14.5876527612609,17.0802317716412,9.71617169073381));
#24138=CARTESIAN_POINT('Ctrl Pts',(-15.5,17.0802317716412,9.67450502406715));
#24139=CARTESIAN_POINT('Ctrl Pts',(-16.4123472387391,17.0802317716412,9.63283835740048));
#24140=CARTESIAN_POINT('Ctrl Pts',(-16.8685208581086,16.2901158858206,9.59117169073381));
#24141=CARTESIAN_POINT('Ctrl Pts',(-17.3246944774781,15.5,9.54950502406714));
#24142=CARTESIAN_POINT('Ctrl Pts',(-16.8685208581086,14.7098841141794,9.50783835740048));
#24143=CARTESIAN_POINT('Ctrl Pts',(-16.4123472387391,13.9197682283588,9.46617169073381));
#24144=CARTESIAN_POINT('Ctrl Pts',(-15.5,13.9197682283588,9.42450502406714));
#24145=CARTESIAN_POINT('Ctrl Pts',(-14.5876527612609,13.9197682283588,9.38283835740048));
#24146=CARTESIAN_POINT('Ctrl Pts',(-14.1314791418914,14.7098841141794,9.34117169073381));
#24147=CARTESIAN_POINT('Ctrl Pts',(-13.6753055225219,15.5,9.29950502406714));
#24148=CARTESIAN_POINT('Ctrl Pts',(-14.1314791418914,16.2901158858206,9.25783835740048));
#24149=CARTESIAN_POINT('Ctrl Pts',(-14.5876527612609,17.0802317716412,9.21617169073381));
#24150=CARTESIAN_POINT('Ctrl Pts',(-15.5,17.0802317716412,9.17450502406714));
#24151=CARTESIAN_POINT('Ctrl Pts',(-16.4123472387391,17.0802317716412,9.13283835740047));
#24152=CARTESIAN_POINT('Ctrl Pts',(-16.8685208581086,16.2901158858206,9.09117169073381));
#24153=CARTESIAN_POINT('Ctrl Pts',(-17.3246944774781,15.5,9.04950502406714));
#24154=CARTESIAN_POINT('Ctrl Pts',(-16.8685208581086,14.7098841141794,9.00783835740047));
#24155=CARTESIAN_POINT('Ctrl Pts',(-16.4123472387391,13.9197682283588,8.9661716907338));
#24156=CARTESIAN_POINT('Ctrl Pts',(-15.5,13.9197682283588,8.92450502406714));
#24157=CARTESIAN_POINT('Ctrl Pts',(-14.5876527612609,13.9197682283588,8.88283835740047));
#24158=CARTESIAN_POINT('Ctrl Pts',(-14.1314791418914,14.7098841141794,8.8411716907338));
#24159=CARTESIAN_POINT('Ctrl Pts',(-13.6753055225219,15.5,8.79950502406713));
#24160=CARTESIAN_POINT('Ctrl Pts',(-14.1314791418914,16.2901158858206,8.75783835740047));
#24161=CARTESIAN_POINT('Ctrl Pts',(-14.5876527612609,17.0802317716412,8.7161716907338));
#24162=CARTESIAN_POINT('Ctrl Pts',(-15.5,17.0802317716412,8.67450502406713));
#24163=CARTESIAN_POINT('Ctrl Pts',(-16.4123472387391,17.0802317716412,8.63283835740047));
#24164=CARTESIAN_POINT('Ctrl Pts',(-16.8685208581086,16.2901158858206,8.5911716907338));
#24165=CARTESIAN_POINT('Ctrl Pts',(-17.3246944774781,15.5,8.54950502406713));
#24166=CARTESIAN_POINT('Ctrl Pts',(-16.8685208581086,14.7098841141794,8.50783835740046));
#24167=CARTESIAN_POINT('Ctrl Pts',(-16.4123472387391,13.9197682283588,8.4661716907338));
#24168=CARTESIAN_POINT('Ctrl Pts',(-15.5,13.9197682283588,8.42450502406713));
#24169=CARTESIAN_POINT('Ctrl Pts',(-14.5876527612609,13.9197682283588,8.38283835740046));
#24170=CARTESIAN_POINT('Ctrl Pts',(-14.1314791418914,14.7098841141794,8.3411716907338));
#24171=CARTESIAN_POINT('Ctrl Pts',(-13.6753055225219,15.5,8.29950502406713));
#24172=CARTESIAN_POINT('Ctrl Pts',(-14.1314791418914,16.2901158858206,8.25783835740046));
#24173=CARTESIAN_POINT('Ctrl Pts',(-14.5876527612609,17.0802317716412,8.21617169073379));
#24174=CARTESIAN_POINT('Ctrl Pts',(-15.5,17.0802317716412,8.17450502406713));
#24175=CARTESIAN_POINT('Ctrl Pts',(-16.4123472387391,17.0802317716412,8.13283835740046));
#24176=CARTESIAN_POINT('Ctrl Pts',(-16.8685208581086,16.2901158858206,8.09117169073379));
#24177=CARTESIAN_POINT('Ctrl Pts',(-17.3246944774781,15.5,8.04950502406713));
#24178=CARTESIAN_POINT('Ctrl Pts',(-16.8685208581086,14.7098841141794,8.00783835740046));
#24179=CARTESIAN_POINT('Ctrl Pts',(-16.4123472387391,13.9197682283588,7.96617169073379));
#24180=CARTESIAN_POINT('Ctrl Pts',(-15.5,13.9197682283588,7.92450502406712));
#24181=CARTESIAN_POINT('Ctrl Pts',(-14.5876527612609,13.9197682283588,7.88283835740046));
#24182=CARTESIAN_POINT('Ctrl Pts',(-14.1314791418914,14.7098841141794,7.84117169073379));
#24183=CARTESIAN_POINT('Ctrl Pts',(-13.6753055225219,15.5,7.79950502406712));
#24184=CARTESIAN_POINT('Ctrl Pts',(-14.1314791418914,16.2901158858206,7.75783835740046));
#24185=CARTESIAN_POINT('Ctrl Pts',(-14.5876527612609,17.0802317716412,7.71617169073378));
#24186=CARTESIAN_POINT('Ctrl Pts',(-15.5,17.0802317716412,7.67450502406712));
#24187=CARTESIAN_POINT('Ctrl Pts',(-16.4123472387391,17.0802317716412,7.63283835740045));
#24188=CARTESIAN_POINT('Ctrl Pts',(-16.8685208581086,16.2901158858206,7.59117169073379));
#24189=CARTESIAN_POINT('Ctrl Pts',(-17.3246944774781,15.5,7.54950502406712));
#24190=CARTESIAN_POINT('Ctrl Pts',(-16.8685208581086,14.7098841141794,7.50783835740045));
#24191=CARTESIAN_POINT('Ctrl Pts',(-16.4123472387391,13.9197682283588,7.46617169073379));
#24192=CARTESIAN_POINT('Ctrl Pts',(-15.5,13.9197682283588,7.42450502406712));
#24193=CARTESIAN_POINT('Ctrl Pts',(-14.5876527612609,13.9197682283588,7.38283835740045));
#24194=CARTESIAN_POINT('Ctrl Pts',(-14.1314791418914,14.7098841141794,7.34117169073378));
#24195=CARTESIAN_POINT('Ctrl Pts',(-13.6753055225219,15.5,7.29950502406711));
#24196=CARTESIAN_POINT('Ctrl Pts',(-14.1314791418914,16.2901158858206,7.25783835740045));
#24197=CARTESIAN_POINT('Ctrl Pts',(-14.5876527612609,17.0802317716412,7.21617169073378));
#24198=CARTESIAN_POINT('Ctrl Pts',(-15.5,17.0802317716412,7.17450502406711));
#24199=CARTESIAN_POINT('Ctrl Pts',(-16.4123472387391,17.0802317716412,7.13283835740044));
#24200=CARTESIAN_POINT('Ctrl Pts',(-16.8685208581086,16.2901158858206,7.09117169073378));
#24201=CARTESIAN_POINT('Ctrl Pts',(-17.3246944774781,15.5,7.04950502406711));
#24202=CARTESIAN_POINT('Ctrl Pts',(-16.8685208581086,14.7098841141794,7.00783835740045));
#24203=CARTESIAN_POINT('Ctrl Pts',(-16.4123472387391,13.9197682283588,6.96617169073378));
#24204=CARTESIAN_POINT('Ctrl Pts',(-15.5,13.9197682283588,6.92450502406711));
#24205=CARTESIAN_POINT('Ctrl Pts',(-14.5876527612609,13.9197682283588,6.88283835740044));
#24206=CARTESIAN_POINT('Ctrl Pts',(-14.1314791418914,14.7098841141794,6.84117169073378));
#24207=CARTESIAN_POINT('Ctrl Pts',(-13.6753055225219,15.5,6.79950502406711));
#24208=CARTESIAN_POINT('Ctrl Pts',(-14.1314791418914,16.2901158858206,6.75783835740044));
#24209=CARTESIAN_POINT('Ctrl Pts',(-14.5876527612609,17.0802317716412,6.71617169073377));
#24210=CARTESIAN_POINT('Ctrl Pts',(-15.5,17.0802317716412,6.67450502406711));
#24211=CARTESIAN_POINT('Ctrl Pts',(-16.4123472387391,17.0802317716412,6.63283835740044));
#24212=CARTESIAN_POINT('Ctrl Pts',(-16.8685208581086,16.2901158858206,6.59117169073377));
#24213=CARTESIAN_POINT('Ctrl Pts',(-17.3246944774781,15.5,6.54950502406711));
#24214=CARTESIAN_POINT('Ctrl Pts',(-16.8685208581086,14.7098841141794,6.50783835740044));
#24215=CARTESIAN_POINT('Ctrl Pts',(-16.4123472387391,13.9197682283588,6.46617169073377));
#24216=CARTESIAN_POINT('Ctrl Pts',(-15.5,13.9197682283588,6.4245050240671));
#24217=CARTESIAN_POINT('Ctrl Pts',(-14.5876527612609,13.9197682283588,6.38283835740044));
#24218=CARTESIAN_POINT('Ctrl Pts',(-14.1314791418914,14.7098841141794,6.34117169073377));
#24219=CARTESIAN_POINT('Ctrl Pts',(-13.6753055225219,15.5,6.2995050240671));
#24220=CARTESIAN_POINT('Ctrl Pts',(-14.1314791418914,16.2901158858206,6.25783835740044));
#24221=CARTESIAN_POINT('Ctrl Pts',(-14.5876527612609,17.0802317716412,6.21617169073377));
#24222=CARTESIAN_POINT('Ctrl Pts',(-15.5,17.0802317716412,6.1745050240671));
#24223=CARTESIAN_POINT('Ctrl Pts',(-16.4123472387391,17.0802317716412,6.13283835740043));
#24224=CARTESIAN_POINT('Ctrl Pts',(-16.8685208581086,16.2901158858206,6.09117169073377));
#24225=CARTESIAN_POINT('Ctrl Pts',(-17.3246944774781,15.5,6.0495050240671));
#24226=CARTESIAN_POINT('Ctrl Pts',(-16.8685208581086,14.7098841141794,6.00783835740043));
#24227=CARTESIAN_POINT('Ctrl Pts',(-16.4123472387391,13.9197682283588,5.96617169073376));
#24228=CARTESIAN_POINT('Ctrl Pts',(-15.5,13.9197682283588,5.9245050240671));
#24229=CARTESIAN_POINT('Ctrl Pts',(-14.5876527612609,13.9197682283588,5.88283835740043));
#24230=CARTESIAN_POINT('Ctrl Pts',(-14.1314791418914,14.7098841141794,5.84117169073376));
#24231=CARTESIAN_POINT('Ctrl Pts',(-13.6753055225219,15.5,5.79950502406709));
#24232=CARTESIAN_POINT('Ctrl Pts',(-14.1314791418914,16.2901158858206,5.75783835740043));
#24233=CARTESIAN_POINT('Ctrl Pts',(-14.5876527612609,17.0802317716412,5.71617169073376));
#24234=CARTESIAN_POINT('Ctrl Pts',(-15.5,17.0802317716412,5.67450502406709));
#24235=CARTESIAN_POINT('Ctrl Pts',(-16.4123472387391,17.0802317716412,5.63283835740043));
#24236=CARTESIAN_POINT('Ctrl Pts',(-16.8685208581086,16.2901158858206,5.59117169073376));
#24237=CARTESIAN_POINT('Ctrl Pts',(-17.3246944774781,15.5,5.54950502406709));
#24238=CARTESIAN_POINT('Ctrl Pts',(-16.8685208581086,14.7098841141794,5.50783835740043));
#24239=CARTESIAN_POINT('Ctrl Pts',(-16.4123472387391,13.9197682283588,5.46617169073376));
#24240=CARTESIAN_POINT('Ctrl Pts',(-15.5,13.9197682283588,5.42450502406709));
#24241=CARTESIAN_POINT('Ctrl Pts',(-14.5876527612609,13.9197682283588,5.38283835740042));
#24242=CARTESIAN_POINT('Ctrl Pts',(-14.1314791418914,14.7098841141794,5.34117169073376));
#24243=CARTESIAN_POINT('Ctrl Pts',(-13.6753055225219,15.5,5.29950502406709));
#24244=CARTESIAN_POINT('Ctrl Pts',(-14.1314791418914,16.2901158858206,5.25783835740042));
#24245=CARTESIAN_POINT('Ctrl Pts',(-14.5876527612609,17.0802317716412,5.21617169073375));
#24246=CARTESIAN_POINT('Ctrl Pts',(-15.5,17.0802317716412,5.17450502406709));
#24247=CARTESIAN_POINT('Ctrl Pts',(-16.4123472387391,17.0802317716412,5.13283835740042));
#24248=CARTESIAN_POINT('Ctrl Pts',(-16.8685208581086,16.2901158858206,5.09117169073375));
#24249=CARTESIAN_POINT('Ctrl Pts',(-17.3246944774781,15.5,5.04950502406708));
#24250=CARTESIAN_POINT('Ctrl Pts',(-16.8685208581086,14.7098841141794,5.00783835740042));
#24251=CARTESIAN_POINT('Ctrl Pts',(-16.4123472387391,13.9197682283588,4.96617169073375));
#24252=CARTESIAN_POINT('Ctrl Pts',(-15.5,13.9197682283588,4.92450502406708));
#24253=CARTESIAN_POINT('Ctrl Pts',(-14.5876527612609,13.9197682283588,4.88283835740042));
#24254=CARTESIAN_POINT('Ctrl Pts',(-14.1314791418914,14.7098841141794,4.84117169073375));
#24255=CARTESIAN_POINT('Ctrl Pts',(-13.6753055225219,15.5,4.79950502406708));
#24256=CARTESIAN_POINT('Ctrl Pts',(-14.1314791418914,16.2901158858206,4.75783835740041));
#24257=CARTESIAN_POINT('Ctrl Pts',(-14.5876527612609,17.0802317716412,4.71617169073375));
#24258=CARTESIAN_POINT('Ctrl Pts',(-15.5,17.0802317716412,4.67450502406708));
#24259=CARTESIAN_POINT('Ctrl Pts',(-16.4123472387391,17.0802317716412,4.63283835740041));
#24260=CARTESIAN_POINT('Ctrl Pts',(-16.8685208581086,16.2901158858206,4.59117169073375));
#24261=CARTESIAN_POINT('Ctrl Pts',(-17.3246944774781,15.5,4.54950502406708));
#24262=CARTESIAN_POINT('Ctrl Pts',(-16.8685208581086,14.7098841141794,4.50783835740041));
#24263=CARTESIAN_POINT('Ctrl Pts',(-16.4123472387391,13.9197682283588,4.46617169073374));
#24264=CARTESIAN_POINT('Ctrl Pts',(-15.5,13.9197682283588,4.42450502406708));
#24265=CARTESIAN_POINT('Ctrl Pts',(-14.5876527612609,13.9197682283588,4.38283835740041));
#24266=CARTESIAN_POINT('Ctrl Pts',(-14.1314791418914,14.7098841141794,4.34117169073374));
#24267=CARTESIAN_POINT('Ctrl Pts',(-13.6753055225219,15.5,4.29950502406708));
#24268=CARTESIAN_POINT('Ctrl Pts',(-14.1314791418914,16.2901158858206,4.25783835740041));
#24269=CARTESIAN_POINT('Ctrl Pts',(-14.5876527612609,17.0802317716412,4.21617169073374));
#24270=CARTESIAN_POINT('Ctrl Pts',(-15.5,17.0802317716412,4.17450502406707));
#24271=CARTESIAN_POINT('Ctrl Pts',(-16.4123472387391,17.0802317716412,4.13283835740041));
#24272=CARTESIAN_POINT('Ctrl Pts',(-16.8685208581086,16.2901158858206,4.09117169073374));
#24273=CARTESIAN_POINT('Ctrl Pts',(-17.3246944774781,15.5,4.04950502406707));
#24274=CARTESIAN_POINT('Ctrl Pts',(-16.8685208581086,14.7098841141794,4.0078383574004));
#24275=CARTESIAN_POINT('Ctrl Pts',(-16.4123472387391,13.9197682283588,3.96617169073374));
#24276=CARTESIAN_POINT('Ctrl Pts',(-15.5,13.9197682283588,3.92450502406707));
#24277=CARTESIAN_POINT('Ctrl Pts',(-14.5876527612609,13.9197682283588,3.8828383574004));
#24278=CARTESIAN_POINT('Ctrl Pts',(-14.1314791418914,14.7098841141794,3.84117169073374));
#24279=CARTESIAN_POINT('Ctrl Pts',(-13.6753055225219,15.5,3.79950502406707));
#24280=CARTESIAN_POINT('Ctrl Pts',(-14.1314791418914,16.2901158858206,3.7578383574004));
#24281=CARTESIAN_POINT('Ctrl Pts',(-14.5876527612609,17.0802317716412,3.71617169073373));
#24282=CARTESIAN_POINT('Ctrl Pts',(-15.5,17.0802317716412,3.67450502406707));
#24283=CARTESIAN_POINT('Ctrl Pts',(-16.4123472387391,17.0802317716412,3.6328383574004));
#24284=CARTESIAN_POINT('Ctrl Pts',(-16.8685208581086,16.2901158858206,3.59117169073373));
#24285=CARTESIAN_POINT('Ctrl Pts',(-17.3246944774781,15.5,3.54950502406707));
#24286=CARTESIAN_POINT('Ctrl Pts',(-16.8685208581086,14.7098841141794,3.5078383574004));
#24287=CARTESIAN_POINT('Ctrl Pts',(-16.4123472387391,13.9197682283588,3.46617169073373));
#24288=CARTESIAN_POINT('Ctrl Pts',(-15.5,13.9197682283588,3.42450502406706));
#24289=CARTESIAN_POINT('Ctrl Pts',(-14.5876527612609,13.9197682283588,3.3828383574004));
#24290=CARTESIAN_POINT('Ctrl Pts',(-14.1314791418914,14.7098841141794,3.34117169073373));
#24291=CARTESIAN_POINT('Ctrl Pts',(-13.6753055225219,15.5,3.29950502406706));
#24292=CARTESIAN_POINT('Ctrl Pts',(-14.1314791418914,16.2901158858206,3.2578383574004));
#24293=CARTESIAN_POINT('Ctrl Pts',(-14.5876527612609,17.0802317716412,3.21617169073373));
#24294=CARTESIAN_POINT('Ctrl Pts',(-15.5,17.0802317716412,3.17450502406706));
#24295=CARTESIAN_POINT('Ctrl Pts',(-16.4123472387391,17.0802317716412,3.13283835740039));
#24296=CARTESIAN_POINT('Ctrl Pts',(-16.8685208581086,16.2901158858206,3.09117169073373));
#24297=CARTESIAN_POINT('Ctrl Pts',(-17.3246944774781,15.5,3.04950502406706));
#24298=CARTESIAN_POINT('Ctrl Pts',(-16.8685208581086,14.7098841141794,3.00783835740039));
#24299=CARTESIAN_POINT('Ctrl Pts',(-16.4123472387391,13.9197682283588,2.96617169073372));
#24300=CARTESIAN_POINT('Ctrl Pts',(-15.5,13.9197682283588,2.92450502406706));
#24301=CARTESIAN_POINT('Ctrl Pts',(-14.5876527612609,13.9197682283588,2.88283835740039));
#24302=CARTESIAN_POINT('Ctrl Pts',(-14.1314791418914,14.7098841141794,2.84117169073372));
#24303=CARTESIAN_POINT('Ctrl Pts',(-13.6753055225219,15.5,2.79950502406705));
#24304=CARTESIAN_POINT('Ctrl Pts',(-14.1314791418914,16.2901158858206,2.75783835740039));
#24305=CARTESIAN_POINT('Ctrl Pts',(-14.5876527612609,17.0802317716412,2.71617169073372));
#24306=CARTESIAN_POINT('Ctrl Pts',(-15.5,17.0802317716412,2.67450502406705));
#24307=CARTESIAN_POINT('Ctrl Pts',(-16.4123472387391,17.0802317716412,2.63283835740039));
#24308=CARTESIAN_POINT('Ctrl Pts',(-16.8685208581086,16.2901158858206,2.59117169073372));
#24309=CARTESIAN_POINT('Ctrl Pts',(-17.3246944774781,15.5,2.54950502406705));
#24310=CARTESIAN_POINT('Ctrl Pts',(-16.8685208581086,14.7098841141794,2.50783835740038));
#24311=CARTESIAN_POINT('Ctrl Pts',(-16.4123472387391,13.9197682283588,2.46617169073372));
#24312=CARTESIAN_POINT('Ctrl Pts',(-15.5,13.9197682283588,2.42450502406705));
#24313=CARTESIAN_POINT('Ctrl Pts',(-14.5876527612609,13.9197682283588,2.38283835740038));
#24314=CARTESIAN_POINT('Ctrl Pts',(-14.1314791418914,14.7098841141794,2.34117169073371));
#24315=CARTESIAN_POINT('Ctrl Pts',(-13.6753055225219,15.5,2.29950502406705));
#24316=CARTESIAN_POINT('Ctrl Pts',(-14.1314791418914,16.2901158858206,2.25783835740038));
#24317=CARTESIAN_POINT('Ctrl Pts',(-14.5876527612609,17.0802317716412,2.21617169073371));
#24318=CARTESIAN_POINT('Ctrl Pts',(-15.5,17.0802317716412,2.17450502406705));
#24319=CARTESIAN_POINT('Ctrl Pts',(-16.4123472387391,17.0802317716412,2.13283835740038));
#24320=CARTESIAN_POINT('Ctrl Pts',(-16.8685208581086,16.2901158858206,2.09117169073371));
#24321=CARTESIAN_POINT('Ctrl Pts',(-17.3246944774781,15.5,2.04950502406705));
#24322=CARTESIAN_POINT('Ctrl Pts',(-16.8685208581086,14.7098841141794,2.00783835740038));
#24323=CARTESIAN_POINT('Ctrl Pts',(-16.4123472387391,13.9197682283588,1.96617169073371));
#24324=CARTESIAN_POINT('Ctrl Pts',(-15.5,13.9197682283588,1.92450502406704));
#24325=CARTESIAN_POINT('Ctrl Pts',(-14.5876527612609,13.9197682283588,1.88283835740038));
#24326=CARTESIAN_POINT('Ctrl Pts',(-14.1314791418914,14.7098841141794,1.84117169073371));
#24327=CARTESIAN_POINT('Ctrl Pts',(-13.6753055225219,15.5,1.79950502406704));
#24328=CARTESIAN_POINT('Ctrl Pts',(-14.1314791418914,16.2901158858206,1.75783835740037));
#24329=CARTESIAN_POINT('Ctrl Pts',(-14.5876527612609,17.0802317716412,1.71617169073371));
#24330=CARTESIAN_POINT('Ctrl Pts',(-15.5,17.0802317716412,1.67450502406704));
#24331=CARTESIAN_POINT('Ctrl Pts',(-16.4123472387391,17.0802317716412,1.63283835740037));
#24332=CARTESIAN_POINT('Ctrl Pts',(-16.8685208581086,16.2901158858206,1.59117169073371));
#24333=CARTESIAN_POINT('Ctrl Pts',(-17.3246944774781,15.5,1.54950502406704));
#24334=CARTESIAN_POINT('Ctrl Pts',(-16.8685208581086,14.7098841141794,1.50783835740037));
#24335=CARTESIAN_POINT('Ctrl Pts',(-16.4123472387391,13.9197682283588,1.4661716907337));
#24336=CARTESIAN_POINT('Ctrl Pts',(-15.5,13.9197682283588,1.42450502406704));
#24337=CARTESIAN_POINT('Ctrl Pts',(-14.5876527612609,13.9197682283588,1.38283835740037));
#24338=CARTESIAN_POINT('Ctrl Pts',(-14.1314791418914,14.7098841141794,1.3411716907337));
#24339=CARTESIAN_POINT('Ctrl Pts',(-13.6753055225219,15.5,1.29950502406703));
#24340=CARTESIAN_POINT('Ctrl Pts',(-14.1314791418914,16.2901158858206,1.25783835740037));
#24341=CARTESIAN_POINT('Ctrl Pts',(-14.5876527612609,17.0802317716412,1.2161716907337));
#24342=CARTESIAN_POINT('Ctrl Pts',(-15.5,17.0802317716412,1.17450502406703));
#24343=CARTESIAN_POINT('Ctrl Pts',(-16.4123472387391,17.0802317716412,1.13283835740037));
#24344=CARTESIAN_POINT('Ctrl Pts',(-16.8685208581086,16.2901158858206,1.0911716907337));
#24345=CARTESIAN_POINT('Ctrl Pts',(-17.3246944774781,15.5,1.04950502406703));
#24346=CARTESIAN_POINT('Ctrl Pts',(-16.8685208581086,14.7098841141794,1.00783835740037));
#24347=CARTESIAN_POINT('Ctrl Pts',(-16.4123472387391,13.9197682283588,0.966171690733698));
#24348=CARTESIAN_POINT('Ctrl Pts',(-15.5,13.9197682283588,0.924505024067031));
#24349=CARTESIAN_POINT('Ctrl Pts',(-14.5876527612609,13.9197682283588,0.882838357400363));
#24350=CARTESIAN_POINT('Ctrl Pts',(-14.1314791418914,14.7098841141794,0.841171690733696));
#24351=CARTESIAN_POINT('Ctrl Pts',(-13.6753055225219,15.5,0.799505024067029));
#24352=CARTESIAN_POINT('Ctrl Pts',(-14.1314791418914,16.2901158858206,0.757838357400362));
#24353=CARTESIAN_POINT('Ctrl Pts',(-14.5876527612609,17.0802317716412,0.716171690733694));
#24354=CARTESIAN_POINT('Ctrl Pts',(-15.5,17.0802317716412,0.674505024067027));
#24355=CARTESIAN_POINT('Ctrl Pts',(-16.4123472387391,17.0802317716412,0.632838357400359));
#24356=CARTESIAN_POINT('Ctrl Pts',(-16.8685208581086,16.2901158858206,0.591171690733692));
#24357=CARTESIAN_POINT('Ctrl Pts',(-17.3246944774781,15.5,0.549505024067025));
#24358=CARTESIAN_POINT('Ctrl Pts',(-16.8685208581086,14.7098841141794,0.507838357400358));
#24359=CARTESIAN_POINT('Ctrl Pts',(-16.4123472387391,13.9197682283588,0.46617169073369));
#24360=CARTESIAN_POINT('Ctrl Pts',(-15.5,13.9197682283588,0.424505024067023));
#24361=CARTESIAN_POINT('Ctrl Pts',(-14.5876527612609,13.9197682283588,0.382838357400356));
#24362=CARTESIAN_POINT('Ctrl Pts',(-14.1314791418914,14.7098841141794,0.341171690733689));
#24363=CARTESIAN_POINT('Ctrl Pts',(-13.6753055225219,15.5,0.299505024067021));
#24364=CARTESIAN_POINT('Ctrl Pts',(-14.1314791418914,16.2901158858206,0.257838357400354));
#24365=CARTESIAN_POINT('Ctrl Pts',(-14.5876527612609,17.0802317716412,0.216171690733687));
#24366=CARTESIAN_POINT('Ctrl Pts',(-15.5,17.0802317716412,0.174505024067019));
#24367=CARTESIAN_POINT('Ctrl Pts',(-16.4123472387391,17.0802317716412,0.132838357400352));
#24368=CARTESIAN_POINT('Ctrl Pts',(-16.8685208581086,16.2901158858206,0.0911716907336849));
#24369=CARTESIAN_POINT('Ctrl Pts',(-17.3246944774781,15.5,0.0495050240670176));
#24370=CARTESIAN_POINT('Ctrl Pts',(-16.8685208581086,14.7098841141794,0.00783835740035031));
#24371=CARTESIAN_POINT('Ctrl Pts',(-16.4123472387391,13.9197682283588,-0.033828309266317));
#24372=CARTESIAN_POINT('Ctrl Pts',(-15.5,13.9197682283588,-0.0754949759329843));
#24373=CARTESIAN_POINT('Ctrl Pts',(-14.5876527612609,13.9197682283588,-0.11716164259965));
#24374=CARTESIAN_POINT('Ctrl Pts',(-14.1314791418914,14.7098841141794,-0.158828309266317));
#24375=CARTESIAN_POINT('Ctrl Pts',(-13.6753055225219,15.5,-0.200494975932984));
#24376=CARTESIAN_POINT('Ctrl Pts',(-14.1314791418914,16.2901158858206,-0.242161642599652));
#24377=CARTESIAN_POINT('Ctrl Pts',(-14.5876527612609,17.0802317716412,-0.283828309266319));
#24378=CARTESIAN_POINT('Ctrl Pts',(-15.5,17.0802317716412,-0.325494975932986));
#24379=CARTESIAN_POINT('Ctrl Pts',(-16.4123472387391,17.0802317716412,-0.367161642599654));
#24380=CARTESIAN_POINT('Ctrl Pts',(-16.8685208581086,16.2901158858206,-0.408828309266321));
#24381=CARTESIAN_POINT('Ctrl Pts',(-17.3246944774781,15.5,-0.450494975932988));
#24382=CARTESIAN_POINT('Ctrl Pts',(-16.8685208581086,14.7098841141794,-0.492161642599655));
#24383=CARTESIAN_POINT('Ctrl Pts',(-16.4123472387391,13.9197682283588,-0.533828309266323));
#24384=CARTESIAN_POINT('Ctrl Pts',(-15.5,13.9197682283588,-0.57549497593299));
#24385=CARTESIAN_POINT('Ctrl Pts',(-14.5876527612609,13.9197682283588,-0.617161642599657));
#24386=CARTESIAN_POINT('Ctrl Pts',(-14.1314791418914,14.7098841141794,-0.658828309266325));
#24387=CARTESIAN_POINT('Ctrl Pts',(-13.6753055225219,15.5,-0.700494975932992));
#24388=CARTESIAN_POINT('Ctrl Pts',(-14.1314791418914,16.2901158858206,-0.742161642599659));
#24389=CARTESIAN_POINT('Ctrl Pts',(-14.5876527612609,17.0802317716412,-0.783828309266326));
#24390=CARTESIAN_POINT('Ctrl Pts',(-15.5,17.0802317716412,-0.825494975932993));
#24391=CARTESIAN_POINT('Ctrl Pts',(-16.4123472387391,17.0802317716412,-0.867161642599661));
#24392=CARTESIAN_POINT('Ctrl Pts',(-16.8685208581086,16.2901158858206,-0.908828309266328));
#24393=CARTESIAN_POINT('Ctrl Pts',(-17.3246944774781,15.5,-0.950494975932995));
#24394=CARTESIAN_POINT('Ctrl Pts',(-16.8685208581086,14.7098841141794,-0.992161642599663));
#24395=CARTESIAN_POINT('Ctrl Pts',(-16.4123472387391,13.9197682283588,-1.03382830926633));
#24396=CARTESIAN_POINT('Ctrl Pts',(-15.5,13.9197682283588,-1.075494975933));
#24397=CARTESIAN_POINT('Ctrl Pts',(-14.5876527612609,13.9197682283588,-1.11716164259966));
#24398=CARTESIAN_POINT('Ctrl Pts',(-14.1314791418914,14.7098841141794,-1.15882830926633));
#24399=CARTESIAN_POINT('Ctrl Pts',(-13.6753055225219,15.5,-1.200494975933));
#24400=CARTESIAN_POINT('Ctrl Pts',(-14.1314791418914,16.2901158858206,-1.24216164259967));
#24401=CARTESIAN_POINT('Ctrl Pts',(-14.5876527612609,17.0802317716412,-1.28382830926633));
#24402=CARTESIAN_POINT('Ctrl Pts',(-15.5,17.0802317716412,-1.325494975933));
#24403=CARTESIAN_POINT('Ctrl Pts',(-16.4123472387391,17.0802317716412,-1.36716164259967));
#24404=CARTESIAN_POINT('Ctrl Pts',(-16.8685208581086,16.2901158858206,-1.40882830926633));
#24405=CARTESIAN_POINT('Ctrl Pts',(-17.3246944774781,15.5,-1.450494975933));
#24406=CARTESIAN_POINT('Ctrl Pts',(-16.8685208581086,14.7098841141794,-1.49216164259967));
#24407=CARTESIAN_POINT('Ctrl Pts',(-16.4123472387391,13.9197682283588,-1.53382830926634));
#24408=CARTESIAN_POINT('Ctrl Pts',(-15.5,13.9197682283588,-1.575494975933));
#24409=CARTESIAN_POINT('Ctrl Pts',(-14.5876527612609,13.9197682283588,-1.61716164259967));
#24410=CARTESIAN_POINT('Ctrl Pts',(-14.1314791418914,14.7098841141794,-1.65882830926634));
#24411=CARTESIAN_POINT('Ctrl Pts',(-13.6753055225219,15.5,-1.70049497593301));
#24412=CARTESIAN_POINT('Ctrl Pts',(-14.1314791418914,16.2901158858206,-1.74216164259967));
#24413=CARTESIAN_POINT('Ctrl Pts',(-14.5876527612609,17.0802317716412,-1.78382830926634));
#24414=CARTESIAN_POINT('Ctrl Pts',(-15.5,17.0802317716412,-1.82549497593301));
#24415=CARTESIAN_POINT('Ctrl Pts',(-16.4123472387391,17.0802317716412,-1.86716164259967));
#24416=CARTESIAN_POINT('Ctrl Pts',(-16.8685208581086,16.2901158858206,-1.90882830926634));
#24417=CARTESIAN_POINT('Ctrl Pts',(-17.3246944774781,15.5,-1.95049497593301));
#24418=CARTESIAN_POINT('Ctrl Pts',(-16.8685208581086,14.7098841141794,-1.99216164259968));
#24419=CARTESIAN_POINT('Ctrl Pts',(-16.7005726719216,14.4189893226644,-2.00750194461187));
#24420=CARTESIAN_POINT('Ctrl Pts',(-16.4288249477777,14.2215569357652,-2.02511838079831));
#24421=CARTESIAN_POINT('Ctrl Pts',(-15.5,17.4320632938683,10.971375));
#24422=CARTESIAN_POINT('Ctrl Pts',(-16.6154772628062,17.4320632938683,10.9297083333333));
#24423=CARTESIAN_POINT('Ctrl Pts',(-17.1732158942094,16.4660316469341,10.8880416666667));
#24424=CARTESIAN_POINT('Ctrl Pts',(-17.7309545256125,15.5,10.846375));
#24425=CARTESIAN_POINT('Ctrl Pts',(-17.1732158942094,14.5339683530659,10.8047083333333));
#24426=CARTESIAN_POINT('Ctrl Pts',(-16.6154772628062,13.5679367061317,10.7630416666667));
#24427=CARTESIAN_POINT('Ctrl Pts',(-15.5,13.5679367061317,10.721375));
#24428=CARTESIAN_POINT('Ctrl Pts',(-14.3845227371938,13.5679367061317,10.6797083333333));
#24429=CARTESIAN_POINT('Ctrl Pts',(-13.8267841057906,14.5339683530659,10.6380416666667));
#24430=CARTESIAN_POINT('Ctrl Pts',(-13.2690454743875,15.5,10.596375));
#24431=CARTESIAN_POINT('Ctrl Pts',(-13.8267841057906,16.4660316469341,10.5547083333333));
#24432=CARTESIAN_POINT('Ctrl Pts',(-14.3845227371938,17.4320632938683,10.5130416666667));
#24433=CARTESIAN_POINT('Ctrl Pts',(-15.5,17.4320632938683,10.471375));
#24434=CARTESIAN_POINT('Ctrl Pts',(-16.6154772628062,17.4320632938683,10.4297083333333));
#24435=CARTESIAN_POINT('Ctrl Pts',(-17.1732158942094,16.4660316469341,10.3880416666667));
#24436=CARTESIAN_POINT('Ctrl Pts',(-17.7309545256125,15.5,10.346375));
#24437=CARTESIAN_POINT('Ctrl Pts',(-17.1732158942094,14.5339683530659,10.3047083333333));
#24438=CARTESIAN_POINT('Ctrl Pts',(-16.6154772628062,13.5679367061317,10.2630416666667));
#24439=CARTESIAN_POINT('Ctrl Pts',(-15.5,13.5679367061317,10.221375));
#24440=CARTESIAN_POINT('Ctrl Pts',(-14.3845227371938,13.5679367061317,10.1797083333333));
#24441=CARTESIAN_POINT('Ctrl Pts',(-13.8267841057906,14.5339683530659,10.1380416666667));
#24442=CARTESIAN_POINT('Ctrl Pts',(-13.2690454743875,15.5,10.096375));
#24443=CARTESIAN_POINT('Ctrl Pts',(-13.8267841057906,16.4660316469341,10.0547083333333));
#24444=CARTESIAN_POINT('Ctrl Pts',(-14.3845227371938,17.4320632938683,10.0130416666666));
#24445=CARTESIAN_POINT('Ctrl Pts',(-15.5,17.4320632938683,9.97137499999998));
#24446=CARTESIAN_POINT('Ctrl Pts',(-16.6154772628062,17.4320632938683,9.92970833333332));
#24447=CARTESIAN_POINT('Ctrl Pts',(-17.1732158942094,16.4660316469341,9.88804166666665));
#24448=CARTESIAN_POINT('Ctrl Pts',(-17.7309545256125,15.5,9.84637499999998));
#24449=CARTESIAN_POINT('Ctrl Pts',(-17.1732158942094,14.5339683530659,9.80470833333331));
#24450=CARTESIAN_POINT('Ctrl Pts',(-16.6154772628062,13.5679367061317,9.76304166666665));
#24451=CARTESIAN_POINT('Ctrl Pts',(-15.5,13.5679367061317,9.72137499999998));
#24452=CARTESIAN_POINT('Ctrl Pts',(-14.3845227371938,13.5679367061317,9.67970833333331));
#24453=CARTESIAN_POINT('Ctrl Pts',(-13.8267841057906,14.5339683530659,9.63804166666664));
#24454=CARTESIAN_POINT('Ctrl Pts',(-13.2690454743875,15.5,9.59637499999998));
#24455=CARTESIAN_POINT('Ctrl Pts',(-13.8267841057906,16.4660316469341,9.55470833333331));
#24456=CARTESIAN_POINT('Ctrl Pts',(-14.3845227371938,17.4320632938683,9.51304166666664));
#24457=CARTESIAN_POINT('Ctrl Pts',(-15.5,17.4320632938683,9.47137499999998));
#24458=CARTESIAN_POINT('Ctrl Pts',(-16.6154772628062,17.4320632938683,9.42970833333331));
#24459=CARTESIAN_POINT('Ctrl Pts',(-17.1732158942094,16.4660316469341,9.38804166666664));
#24460=CARTESIAN_POINT('Ctrl Pts',(-17.7309545256125,15.5,9.34637499999997));
#24461=CARTESIAN_POINT('Ctrl Pts',(-17.1732158942094,14.5339683530659,9.30470833333331));
#24462=CARTESIAN_POINT('Ctrl Pts',(-16.6154772628062,13.5679367061317,9.26304166666664));
#24463=CARTESIAN_POINT('Ctrl Pts',(-15.5,13.5679367061317,9.22137499999997));
#24464=CARTESIAN_POINT('Ctrl Pts',(-14.3845227371938,13.5679367061317,9.1797083333333));
#24465=CARTESIAN_POINT('Ctrl Pts',(-13.8267841057906,14.5339683530659,9.13804166666664));
#24466=CARTESIAN_POINT('Ctrl Pts',(-13.2690454743875,15.5,9.09637499999997));
#24467=CARTESIAN_POINT('Ctrl Pts',(-13.8267841057906,16.4660316469341,9.0547083333333));
#24468=CARTESIAN_POINT('Ctrl Pts',(-14.3845227371938,17.4320632938683,9.01304166666664));
#24469=CARTESIAN_POINT('Ctrl Pts',(-15.5,17.4320632938683,8.97137499999997));
#24470=CARTESIAN_POINT('Ctrl Pts',(-16.6154772628062,17.4320632938683,8.9297083333333));
#24471=CARTESIAN_POINT('Ctrl Pts',(-17.1732158942094,16.4660316469341,8.88804166666663));
#24472=CARTESIAN_POINT('Ctrl Pts',(-17.7309545256125,15.5,8.84637499999997));
#24473=CARTESIAN_POINT('Ctrl Pts',(-17.1732158942094,14.5339683530659,8.8047083333333));
#24474=CARTESIAN_POINT('Ctrl Pts',(-16.6154772628062,13.5679367061317,8.76304166666663));
#24475=CARTESIAN_POINT('Ctrl Pts',(-15.5,13.5679367061317,8.72137499999997));
#24476=CARTESIAN_POINT('Ctrl Pts',(-14.3845227371938,13.5679367061317,8.6797083333333));
#24477=CARTESIAN_POINT('Ctrl Pts',(-13.8267841057906,14.5339683530659,8.63804166666663));
#24478=CARTESIAN_POINT('Ctrl Pts',(-13.2690454743875,15.5,8.59637499999996));
#24479=CARTESIAN_POINT('Ctrl Pts',(-13.8267841057906,16.4660316469341,8.5547083333333));
#24480=CARTESIAN_POINT('Ctrl Pts',(-14.3845227371938,17.4320632938683,8.51304166666663));
#24481=CARTESIAN_POINT('Ctrl Pts',(-15.5,17.4320632938683,8.47137499999996));
#24482=CARTESIAN_POINT('Ctrl Pts',(-16.6154772628062,17.4320632938683,8.42970833333329));
#24483=CARTESIAN_POINT('Ctrl Pts',(-17.1732158942094,16.4660316469341,8.38804166666663));
#24484=CARTESIAN_POINT('Ctrl Pts',(-17.7309545256125,15.5,8.34637499999996));
#24485=CARTESIAN_POINT('Ctrl Pts',(-17.1732158942094,14.5339683530659,8.30470833333329));
#24486=CARTESIAN_POINT('Ctrl Pts',(-16.6154772628062,13.5679367061317,8.26304166666663));
#24487=CARTESIAN_POINT('Ctrl Pts',(-15.5,13.5679367061317,8.22137499999996));
#24488=CARTESIAN_POINT('Ctrl Pts',(-14.3845227371938,13.5679367061317,8.17970833333329));
#24489=CARTESIAN_POINT('Ctrl Pts',(-13.8267841057906,14.5339683530659,8.13804166666662));
#24490=CARTESIAN_POINT('Ctrl Pts',(-13.2690454743875,15.5,8.09637499999996));
#24491=CARTESIAN_POINT('Ctrl Pts',(-13.8267841057906,16.4660316469341,8.05470833333329));
#24492=CARTESIAN_POINT('Ctrl Pts',(-14.3845227371938,17.4320632938683,8.01304166666662));
#24493=CARTESIAN_POINT('Ctrl Pts',(-15.5,17.4320632938683,7.97137499999995));
#24494=CARTESIAN_POINT('Ctrl Pts',(-16.6154772628062,17.4320632938683,7.92970833333329));
#24495=CARTESIAN_POINT('Ctrl Pts',(-17.1732158942094,16.4660316469341,7.88804166666662));
#24496=CARTESIAN_POINT('Ctrl Pts',(-17.7309545256125,15.5,7.84637499999995));
#24497=CARTESIAN_POINT('Ctrl Pts',(-17.1732158942094,14.5339683530659,7.80470833333329));
#24498=CARTESIAN_POINT('Ctrl Pts',(-16.6154772628062,13.5679367061317,7.76304166666662));
#24499=CARTESIAN_POINT('Ctrl Pts',(-15.5,13.5679367061317,7.72137499999995));
#24500=CARTESIAN_POINT('Ctrl Pts',(-14.3845227371938,13.5679367061317,7.67970833333329));
#24501=CARTESIAN_POINT('Ctrl Pts',(-13.8267841057906,14.5339683530659,7.63804166666662));
#24502=CARTESIAN_POINT('Ctrl Pts',(-13.2690454743875,15.5,7.59637499999995));
#24503=CARTESIAN_POINT('Ctrl Pts',(-13.8267841057906,16.4660316469341,7.55470833333328));
#24504=CARTESIAN_POINT('Ctrl Pts',(-14.3845227371938,17.4320632938683,7.51304166666662));
#24505=CARTESIAN_POINT('Ctrl Pts',(-15.5,17.4320632938683,7.47137499999995));
#24506=CARTESIAN_POINT('Ctrl Pts',(-16.6154772628062,17.4320632938683,7.42970833333328));
#24507=CARTESIAN_POINT('Ctrl Pts',(-17.1732158942094,16.4660316469341,7.38804166666661));
#24508=CARTESIAN_POINT('Ctrl Pts',(-17.7309545256125,15.5,7.34637499999995));
#24509=CARTESIAN_POINT('Ctrl Pts',(-17.1732158942094,14.5339683530659,7.30470833333328));
#24510=CARTESIAN_POINT('Ctrl Pts',(-16.6154772628062,13.5679367061317,7.26304166666661));
#24511=CARTESIAN_POINT('Ctrl Pts',(-15.5,13.5679367061317,7.22137499999994));
#24512=CARTESIAN_POINT('Ctrl Pts',(-14.3845227371938,13.5679367061317,7.17970833333328));
#24513=CARTESIAN_POINT('Ctrl Pts',(-13.8267841057906,14.5339683530659,7.13804166666661));
#24514=CARTESIAN_POINT('Ctrl Pts',(-13.2690454743875,15.5,7.09637499999995));
#24515=CARTESIAN_POINT('Ctrl Pts',(-13.8267841057906,16.4660316469341,7.05470833333328));
#24516=CARTESIAN_POINT('Ctrl Pts',(-14.3845227371938,17.4320632938683,7.01304166666661));
#24517=CARTESIAN_POINT('Ctrl Pts',(-15.5,17.4320632938683,6.97137499999994));
#24518=CARTESIAN_POINT('Ctrl Pts',(-16.6154772628062,17.4320632938683,6.92970833333328));
#24519=CARTESIAN_POINT('Ctrl Pts',(-17.1732158942094,16.4660316469341,6.88804166666661));
#24520=CARTESIAN_POINT('Ctrl Pts',(-17.7309545256125,15.5,6.84637499999994));
#24521=CARTESIAN_POINT('Ctrl Pts',(-17.1732158942094,14.5339683530659,6.80470833333327));
#24522=CARTESIAN_POINT('Ctrl Pts',(-16.6154772628062,13.5679367061317,6.76304166666661));
#24523=CARTESIAN_POINT('Ctrl Pts',(-15.5,13.5679367061317,6.72137499999994));
#24524=CARTESIAN_POINT('Ctrl Pts',(-14.3845227371938,13.5679367061317,6.67970833333327));
#24525=CARTESIAN_POINT('Ctrl Pts',(-13.8267841057906,14.5339683530659,6.6380416666666));
#24526=CARTESIAN_POINT('Ctrl Pts',(-13.2690454743875,15.5,6.59637499999994));
#24527=CARTESIAN_POINT('Ctrl Pts',(-13.8267841057906,16.4660316469341,6.55470833333327));
#24528=CARTESIAN_POINT('Ctrl Pts',(-14.3845227371938,17.4320632938683,6.5130416666666));
#24529=CARTESIAN_POINT('Ctrl Pts',(-15.5,17.4320632938683,6.47137499999994));
#24530=CARTESIAN_POINT('Ctrl Pts',(-16.6154772628062,17.4320632938683,6.42970833333327));
#24531=CARTESIAN_POINT('Ctrl Pts',(-17.1732158942094,16.4660316469341,6.3880416666666));
#24532=CARTESIAN_POINT('Ctrl Pts',(-17.7309545256125,15.5,6.34637499999993));
#24533=CARTESIAN_POINT('Ctrl Pts',(-17.1732158942094,14.5339683530659,6.30470833333327));
#24534=CARTESIAN_POINT('Ctrl Pts',(-16.6154772628062,13.5679367061317,6.2630416666666));
#24535=CARTESIAN_POINT('Ctrl Pts',(-15.5,13.5679367061317,6.22137499999993));
#24536=CARTESIAN_POINT('Ctrl Pts',(-14.3845227371938,13.5679367061317,6.17970833333327));
#24537=CARTESIAN_POINT('Ctrl Pts',(-13.8267841057906,14.5339683530659,6.1380416666666));
#24538=CARTESIAN_POINT('Ctrl Pts',(-13.2690454743875,15.5,6.09637499999993));
#24539=CARTESIAN_POINT('Ctrl Pts',(-13.8267841057906,16.4660316469341,6.05470833333326));
#24540=CARTESIAN_POINT('Ctrl Pts',(-14.3845227371938,17.4320632938683,6.0130416666666));
#24541=CARTESIAN_POINT('Ctrl Pts',(-15.5,17.4320632938683,5.97137499999993));
#24542=CARTESIAN_POINT('Ctrl Pts',(-16.6154772628062,17.4320632938683,5.92970833333326));
#24543=CARTESIAN_POINT('Ctrl Pts',(-17.1732158942094,16.4660316469341,5.8880416666666));
#24544=CARTESIAN_POINT('Ctrl Pts',(-17.7309545256125,15.5,5.84637499999993));
#24545=CARTESIAN_POINT('Ctrl Pts',(-17.1732158942094,14.5339683530659,5.80470833333326));
#24546=CARTESIAN_POINT('Ctrl Pts',(-16.6154772628062,13.5679367061317,5.76304166666659));
#24547=CARTESIAN_POINT('Ctrl Pts',(-15.5,13.5679367061317,5.72137499999993));
#24548=CARTESIAN_POINT('Ctrl Pts',(-14.3845227371938,13.5679367061317,5.67970833333326));
#24549=CARTESIAN_POINT('Ctrl Pts',(-13.8267841057906,14.5339683530659,5.63804166666659));
#24550=CARTESIAN_POINT('Ctrl Pts',(-13.2690454743875,15.5,5.59637499999992));
#24551=CARTESIAN_POINT('Ctrl Pts',(-13.8267841057906,16.4660316469341,5.55470833333326));
#24552=CARTESIAN_POINT('Ctrl Pts',(-14.3845227371938,17.4320632938683,5.51304166666659));
#24553=CARTESIAN_POINT('Ctrl Pts',(-15.5,17.4320632938683,5.47137499999992));
#24554=CARTESIAN_POINT('Ctrl Pts',(-16.6154772628062,17.4320632938683,5.42970833333325));
#24555=CARTESIAN_POINT('Ctrl Pts',(-17.1732158942094,16.4660316469341,5.38804166666659));
#24556=CARTESIAN_POINT('Ctrl Pts',(-17.7309545256125,15.5,5.34637499999992));
#24557=CARTESIAN_POINT('Ctrl Pts',(-17.1732158942094,14.5339683530659,5.30470833333325));
#24558=CARTESIAN_POINT('Ctrl Pts',(-16.6154772628062,13.5679367061317,5.26304166666659));
#24559=CARTESIAN_POINT('Ctrl Pts',(-15.5,13.5679367061317,5.22137499999992));
#24560=CARTESIAN_POINT('Ctrl Pts',(-14.3845227371938,13.5679367061317,5.17970833333325));
#24561=CARTESIAN_POINT('Ctrl Pts',(-13.8267841057906,14.5339683530659,5.13804166666659));
#24562=CARTESIAN_POINT('Ctrl Pts',(-13.2690454743875,15.5,5.09637499999992));
#24563=CARTESIAN_POINT('Ctrl Pts',(-13.8267841057906,16.4660316469341,5.05470833333325));
#24564=CARTESIAN_POINT('Ctrl Pts',(-14.3845227371938,17.4320632938683,5.01304166666658));
#24565=CARTESIAN_POINT('Ctrl Pts',(-15.5,17.4320632938683,4.97137499999991));
#24566=CARTESIAN_POINT('Ctrl Pts',(-16.6154772628062,17.4320632938683,4.92970833333325));
#24567=CARTESIAN_POINT('Ctrl Pts',(-17.1732158942094,16.4660316469341,4.88804166666658));
#24568=CARTESIAN_POINT('Ctrl Pts',(-17.7309545256125,15.5,4.84637499999991));
#24569=CARTESIAN_POINT('Ctrl Pts',(-17.1732158942094,14.5339683530659,4.80470833333325));
#24570=CARTESIAN_POINT('Ctrl Pts',(-16.6154772628062,13.5679367061317,4.76304166666658));
#24571=CARTESIAN_POINT('Ctrl Pts',(-15.5,13.5679367061317,4.72137499999991));
#24572=CARTESIAN_POINT('Ctrl Pts',(-14.3845227371938,13.5679367061317,4.67970833333325));
#24573=CARTESIAN_POINT('Ctrl Pts',(-13.8267841057906,14.5339683530659,4.63804166666658));
#24574=CARTESIAN_POINT('Ctrl Pts',(-13.2690454743875,15.5,4.59637499999991));
#24575=CARTESIAN_POINT('Ctrl Pts',(-13.8267841057906,16.4660316469341,4.55470833333324));
#24576=CARTESIAN_POINT('Ctrl Pts',(-14.3845227371938,17.4320632938683,4.51304166666658));
#24577=CARTESIAN_POINT('Ctrl Pts',(-15.5,17.4320632938683,4.47137499999991));
#24578=CARTESIAN_POINT('Ctrl Pts',(-16.6154772628062,17.4320632938683,4.42970833333324));
#24579=CARTESIAN_POINT('Ctrl Pts',(-17.1732158942094,16.4660316469341,4.38804166666657));
#24580=CARTESIAN_POINT('Ctrl Pts',(-17.7309545256125,15.5,4.34637499999991));
#24581=CARTESIAN_POINT('Ctrl Pts',(-17.1732158942094,14.5339683530659,4.30470833333324));
#24582=CARTESIAN_POINT('Ctrl Pts',(-16.6154772628062,13.5679367061317,4.26304166666657));
#24583=CARTESIAN_POINT('Ctrl Pts',(-15.5,13.5679367061317,4.22137499999991));
#24584=CARTESIAN_POINT('Ctrl Pts',(-14.3845227371938,13.5679367061317,4.17970833333324));
#24585=CARTESIAN_POINT('Ctrl Pts',(-13.8267841057906,14.5339683530659,4.13804166666657));
#24586=CARTESIAN_POINT('Ctrl Pts',(-13.2690454743875,15.5,4.0963749999999));
#24587=CARTESIAN_POINT('Ctrl Pts',(-13.8267841057906,16.4660316469341,4.05470833333324));
#24588=CARTESIAN_POINT('Ctrl Pts',(-14.3845227371938,17.4320632938683,4.01304166666657));
#24589=CARTESIAN_POINT('Ctrl Pts',(-15.5,17.4320632938683,3.9713749999999));
#24590=CARTESIAN_POINT('Ctrl Pts',(-16.6154772628062,17.4320632938683,3.92970833333323));
#24591=CARTESIAN_POINT('Ctrl Pts',(-17.1732158942094,16.4660316469341,3.88804166666657));
#24592=CARTESIAN_POINT('Ctrl Pts',(-17.7309545256125,15.5,3.8463749999999));
#24593=CARTESIAN_POINT('Ctrl Pts',(-17.1732158942094,14.5339683530659,3.80470833333323));
#24594=CARTESIAN_POINT('Ctrl Pts',(-16.6154772628062,13.5679367061317,3.76304166666656));
#24595=CARTESIAN_POINT('Ctrl Pts',(-15.5,13.5679367061317,3.7213749999999));
#24596=CARTESIAN_POINT('Ctrl Pts',(-14.3845227371938,13.5679367061317,3.67970833333323));
#24597=CARTESIAN_POINT('Ctrl Pts',(-13.8267841057906,14.5339683530659,3.63804166666656));
#24598=CARTESIAN_POINT('Ctrl Pts',(-13.2690454743875,15.5,3.5963749999999));
#24599=CARTESIAN_POINT('Ctrl Pts',(-13.8267841057906,16.4660316469341,3.55470833333323));
#24600=CARTESIAN_POINT('Ctrl Pts',(-14.3845227371938,17.4320632938683,3.51304166666656));
#24601=CARTESIAN_POINT('Ctrl Pts',(-15.5,17.4320632938683,3.4713749999999));
#24602=CARTESIAN_POINT('Ctrl Pts',(-16.6154772628062,17.4320632938683,3.42970833333323));
#24603=CARTESIAN_POINT('Ctrl Pts',(-17.1732158942094,16.4660316469341,3.38804166666656));
#24604=CARTESIAN_POINT('Ctrl Pts',(-17.7309545256125,15.5,3.34637499999989));
#24605=CARTESIAN_POINT('Ctrl Pts',(-17.1732158942094,14.5339683530659,3.30470833333323));
#24606=CARTESIAN_POINT('Ctrl Pts',(-16.6154772628062,13.5679367061317,3.26304166666656));
#24607=CARTESIAN_POINT('Ctrl Pts',(-15.5,13.5679367061317,3.22137499999989));
#24608=CARTESIAN_POINT('Ctrl Pts',(-14.3845227371938,13.5679367061317,3.17970833333322));
#24609=CARTESIAN_POINT('Ctrl Pts',(-13.8267841057906,14.5339683530659,3.13804166666656));
#24610=CARTESIAN_POINT('Ctrl Pts',(-13.2690454743875,15.5,3.09637499999989));
#24611=CARTESIAN_POINT('Ctrl Pts',(-13.8267841057906,16.4660316469341,3.05470833333322));
#24612=CARTESIAN_POINT('Ctrl Pts',(-14.3845227371938,17.4320632938683,3.01304166666656));
#24613=CARTESIAN_POINT('Ctrl Pts',(-15.5,17.4320632938683,2.97137499999989));
#24614=CARTESIAN_POINT('Ctrl Pts',(-16.6154772628062,17.4320632938683,2.92970833333322));
#24615=CARTESIAN_POINT('Ctrl Pts',(-17.1732158942094,16.4660316469341,2.88804166666655));
#24616=CARTESIAN_POINT('Ctrl Pts',(-17.7309545256125,15.5,2.84637499999989));
#24617=CARTESIAN_POINT('Ctrl Pts',(-17.1732158942094,14.5339683530659,2.80470833333322));
#24618=CARTESIAN_POINT('Ctrl Pts',(-16.6154772628062,13.5679367061317,2.76304166666655));
#24619=CARTESIAN_POINT('Ctrl Pts',(-15.5,13.5679367061317,2.72137499999989));
#24620=CARTESIAN_POINT('Ctrl Pts',(-14.3845227371938,13.5679367061317,2.67970833333322));
#24621=CARTESIAN_POINT('Ctrl Pts',(-13.8267841057906,14.5339683530659,2.63804166666655));
#24622=CARTESIAN_POINT('Ctrl Pts',(-13.2690454743875,15.5,2.59637499999988));
#24623=CARTESIAN_POINT('Ctrl Pts',(-13.8267841057906,16.4660316469341,2.55470833333322));
#24624=CARTESIAN_POINT('Ctrl Pts',(-14.3845227371938,17.4320632938683,2.51304166666655));
#24625=CARTESIAN_POINT('Ctrl Pts',(-15.5,17.4320632938683,2.47137499999988));
#24626=CARTESIAN_POINT('Ctrl Pts',(-16.6154772628062,17.4320632938683,2.42970833333321));
#24627=CARTESIAN_POINT('Ctrl Pts',(-17.1732158942094,16.4660316469341,2.38804166666655));
#24628=CARTESIAN_POINT('Ctrl Pts',(-17.7309545256125,15.5,2.34637499999988));
#24629=CARTESIAN_POINT('Ctrl Pts',(-17.1732158942094,14.5339683530659,2.30470833333321));
#24630=CARTESIAN_POINT('Ctrl Pts',(-16.6154772628062,13.5679367061317,2.26304166666655));
#24631=CARTESIAN_POINT('Ctrl Pts',(-15.5,13.5679367061317,2.22137499999988));
#24632=CARTESIAN_POINT('Ctrl Pts',(-14.3845227371938,13.5679367061317,2.17970833333321));
#24633=CARTESIAN_POINT('Ctrl Pts',(-13.8267841057906,14.5339683530659,2.13804166666654));
#24634=CARTESIAN_POINT('Ctrl Pts',(-13.2690454743875,15.5,2.09637499999988));
#24635=CARTESIAN_POINT('Ctrl Pts',(-13.8267841057906,16.4660316469341,2.05470833333321));
#24636=CARTESIAN_POINT('Ctrl Pts',(-14.3845227371938,17.4320632938683,2.01304166666654));
#24637=CARTESIAN_POINT('Ctrl Pts',(-15.5,17.4320632938683,1.97137499999988));
#24638=CARTESIAN_POINT('Ctrl Pts',(-16.6154772628062,17.4320632938683,1.92970833333321));
#24639=CARTESIAN_POINT('Ctrl Pts',(-17.1732158942094,16.4660316469341,1.88804166666654));
#24640=CARTESIAN_POINT('Ctrl Pts',(-17.7309545256125,15.5,1.84637499999987));
#24641=CARTESIAN_POINT('Ctrl Pts',(-17.1732158942094,14.5339683530659,1.80470833333321));
#24642=CARTESIAN_POINT('Ctrl Pts',(-16.6154772628062,13.5679367061317,1.76304166666654));
#24643=CARTESIAN_POINT('Ctrl Pts',(-15.5,13.5679367061317,1.72137499999987));
#24644=CARTESIAN_POINT('Ctrl Pts',(-14.3845227371938,13.5679367061317,1.67970833333321));
#24645=CARTESIAN_POINT('Ctrl Pts',(-13.8267841057906,14.5339683530659,1.63804166666654));
#24646=CARTESIAN_POINT('Ctrl Pts',(-13.2690454743875,15.5,1.59637499999987));
#24647=CARTESIAN_POINT('Ctrl Pts',(-13.8267841057906,16.4660316469341,1.5547083333332));
#24648=CARTESIAN_POINT('Ctrl Pts',(-14.3845227371938,17.4320632938683,1.51304166666654));
#24649=CARTESIAN_POINT('Ctrl Pts',(-15.5,17.4320632938683,1.47137499999987));
#24650=CARTESIAN_POINT('Ctrl Pts',(-16.6154772628062,17.4320632938683,1.4297083333332));
#24651=CARTESIAN_POINT('Ctrl Pts',(-17.1732158942094,16.4660316469341,1.38804166666653));
#24652=CARTESIAN_POINT('Ctrl Pts',(-17.7309545256125,15.5,1.34637499999987));
#24653=CARTESIAN_POINT('Ctrl Pts',(-17.1732158942094,14.5339683530659,1.3047083333332));
#24654=CARTESIAN_POINT('Ctrl Pts',(-16.6154772628062,13.5679367061317,1.26304166666653));
#24655=CARTESIAN_POINT('Ctrl Pts',(-15.5,13.5679367061317,1.22137499999987));
#24656=CARTESIAN_POINT('Ctrl Pts',(-14.3845227371938,13.5679367061317,1.1797083333332));
#24657=CARTESIAN_POINT('Ctrl Pts',(-13.8267841057906,14.5339683530659,1.13804166666653));
#24658=CARTESIAN_POINT('Ctrl Pts',(-13.2690454743875,15.5,1.09637499999986));
#24659=CARTESIAN_POINT('Ctrl Pts',(-13.8267841057906,16.4660316469341,1.0547083333332));
#24660=CARTESIAN_POINT('Ctrl Pts',(-14.3845227371938,17.4320632938683,1.01304166666653));
#24661=CARTESIAN_POINT('Ctrl Pts',(-15.5,17.4320632938683,0.971374999999861));
#24662=CARTESIAN_POINT('Ctrl Pts',(-16.6154772628062,17.4320632938683,0.929708333333194));
#24663=CARTESIAN_POINT('Ctrl Pts',(-17.1732158942094,16.4660316469341,0.888041666666528));
#24664=CARTESIAN_POINT('Ctrl Pts',(-17.7309545256125,15.5,0.846374999999861));
#24665=CARTESIAN_POINT('Ctrl Pts',(-17.1732158942094,14.5339683530659,0.804708333333194));
#24666=CARTESIAN_POINT('Ctrl Pts',(-16.6154772628062,13.5679367061317,0.763041666666526));
#24667=CARTESIAN_POINT('Ctrl Pts',(-15.5,13.5679367061317,0.721374999999859));
#24668=CARTESIAN_POINT('Ctrl Pts',(-14.3845227371938,13.5679367061317,0.679708333333192));
#24669=CARTESIAN_POINT('Ctrl Pts',(-13.8267841057906,14.5339683530659,0.638041666666525));
#24670=CARTESIAN_POINT('Ctrl Pts',(-13.2690454743875,15.5,0.596374999999858));
#24671=CARTESIAN_POINT('Ctrl Pts',(-13.8267841057906,16.4660316469341,0.55470833333319));
#24672=CARTESIAN_POINT('Ctrl Pts',(-14.3845227371938,17.4320632938683,0.513041666666523));
#24673=CARTESIAN_POINT('Ctrl Pts',(-15.5,17.4320632938683,0.471374999999856));
#24674=CARTESIAN_POINT('Ctrl Pts',(-16.6154772628062,17.4320632938683,0.429708333333188));
#24675=CARTESIAN_POINT('Ctrl Pts',(-17.1732158942094,16.4660316469341,0.388041666666521));
#24676=CARTESIAN_POINT('Ctrl Pts',(-17.7309545256125,15.5,0.346374999999854));
#24677=CARTESIAN_POINT('Ctrl Pts',(-17.1732158942094,14.5339683530659,0.304708333333186));
#24678=CARTESIAN_POINT('Ctrl Pts',(-16.6154772628062,13.5679367061317,0.263041666666519));
#24679=CARTESIAN_POINT('Ctrl Pts',(-15.5,13.5679367061317,0.221374999999852));
#24680=CARTESIAN_POINT('Ctrl Pts',(-14.3845227371938,13.5679367061317,0.179708333333185));
#24681=CARTESIAN_POINT('Ctrl Pts',(-13.8267841057906,14.5339683530659,0.138041666666517));
#24682=CARTESIAN_POINT('Ctrl Pts',(-13.2690454743875,15.5,0.0963749999998501));
#24683=CARTESIAN_POINT('Ctrl Pts',(-13.8267841057906,16.4660316469341,0.0547083333331828));
#24684=CARTESIAN_POINT('Ctrl Pts',(-14.3845227371938,17.4320632938683,0.0130416666665155));
#24685=CARTESIAN_POINT('Ctrl Pts',(-15.5,17.4320632938683,-0.0286250000001518));
#24686=CARTESIAN_POINT('Ctrl Pts',(-16.6154772628062,17.4320632938683,-0.0702916666668191));
#24687=CARTESIAN_POINT('Ctrl Pts',(-17.1732158942094,16.4660316469341,-0.111958333333486));
#24688=CARTESIAN_POINT('Ctrl Pts',(-17.7309545256125,15.5,-0.153625000000154));
#24689=CARTESIAN_POINT('Ctrl Pts',(-17.1732158942094,14.5339683530659,-0.195291666666821));
#24690=CARTESIAN_POINT('Ctrl Pts',(-16.6154772628062,13.5679367061317,-0.236958333333488));
#24691=CARTESIAN_POINT('Ctrl Pts',(-15.5,13.5679367061317,-0.278625000000155));
#24692=CARTESIAN_POINT('Ctrl Pts',(-14.3845227371938,13.5679367061317,-0.320291666666821));
#24693=CARTESIAN_POINT('Ctrl Pts',(-13.8267841057906,14.5339683530659,-0.361958333333488));
#24694=CARTESIAN_POINT('Ctrl Pts',(-13.2690454743875,15.5,-0.403625000000156));
#24695=CARTESIAN_POINT('Ctrl Pts',(-13.8267841057906,16.4660316469341,-0.445291666666823));
#24696=CARTESIAN_POINT('Ctrl Pts',(-14.3845227371938,17.4320632938683,-0.48695833333349));
#24697=CARTESIAN_POINT('Ctrl Pts',(-15.5,17.4320632938683,-0.528625000000157));
#24698=CARTESIAN_POINT('Ctrl Pts',(-16.6154772628062,17.4320632938683,-0.570291666666825));
#24699=CARTESIAN_POINT('Ctrl Pts',(-17.1732158942094,16.4660316469341,-0.611958333333492));
#24700=CARTESIAN_POINT('Ctrl Pts',(-17.7309545256125,15.5,-0.653625000000159));
#24701=CARTESIAN_POINT('Ctrl Pts',(-17.1732158942094,14.5339683530659,-0.695291666666827));
#24702=CARTESIAN_POINT('Ctrl Pts',(-16.6154772628062,13.5679367061317,-0.736958333333494));
#24703=CARTESIAN_POINT('Ctrl Pts',(-15.5,13.5679367061317,-0.778625000000161));
#24704=CARTESIAN_POINT('Ctrl Pts',(-14.3845227371938,13.5679367061317,-0.820291666666829));
#24705=CARTESIAN_POINT('Ctrl Pts',(-13.8267841057906,14.5339683530659,-0.861958333333496));
#24706=CARTESIAN_POINT('Ctrl Pts',(-13.2690454743875,15.5,-0.903625000000163));
#24707=CARTESIAN_POINT('Ctrl Pts',(-13.8267841057906,16.4660316469341,-0.94529166666683));
#24708=CARTESIAN_POINT('Ctrl Pts',(-14.3845227371938,17.4320632938683,-0.986958333333498));
#24709=CARTESIAN_POINT('Ctrl Pts',(-15.5,17.4320632938683,-1.02862500000016));
#24710=CARTESIAN_POINT('Ctrl Pts',(-16.6154772628062,17.4320632938683,-1.07029166666683));
#24711=CARTESIAN_POINT('Ctrl Pts',(-17.1732158942094,16.4660316469341,-1.1119583333335));
#24712=CARTESIAN_POINT('Ctrl Pts',(-17.7309545256125,15.5,-1.15362500000017));
#24713=CARTESIAN_POINT('Ctrl Pts',(-17.1732158942094,14.5339683530659,-1.19529166666683));
#24714=CARTESIAN_POINT('Ctrl Pts',(-16.6154772628062,13.5679367061317,-1.2369583333335));
#24715=CARTESIAN_POINT('Ctrl Pts',(-15.5,13.5679367061317,-1.27862500000017));
#24716=CARTESIAN_POINT('Ctrl Pts',(-14.3845227371938,13.5679367061317,-1.32029166666684));
#24717=CARTESIAN_POINT('Ctrl Pts',(-13.8267841057906,14.5339683530659,-1.3619583333335));
#24718=CARTESIAN_POINT('Ctrl Pts',(-13.2690454743875,15.5,-1.40362500000017));
#24719=CARTESIAN_POINT('Ctrl Pts',(-13.8267841057906,16.4660316469341,-1.44529166666684));
#24720=CARTESIAN_POINT('Ctrl Pts',(-14.3845227371938,17.4320632938683,-1.4869583333335));
#24721=CARTESIAN_POINT('Ctrl Pts',(-15.5,17.4320632938683,-1.52862500000017));
#24722=CARTESIAN_POINT('Ctrl Pts',(-16.6154772628062,17.4320632938683,-1.57029166666684));
#24723=CARTESIAN_POINT('Ctrl Pts',(-17.1732158942094,16.4660316469341,-1.61195833333351));
#24724=CARTESIAN_POINT('Ctrl Pts',(-17.7309545256125,15.5,-1.65362500000017));
#24725=CARTESIAN_POINT('Ctrl Pts',(-17.1732158942094,14.5339683530659,-1.69529166666684));
#24726=CARTESIAN_POINT('Ctrl Pts',(-16.6154772628062,13.5679367061317,-1.73695833333351));
#24727=CARTESIAN_POINT('Ctrl Pts',(-15.5,13.5679367061317,-1.77862500000017));
#24728=CARTESIAN_POINT('Ctrl Pts',(-14.3845227371938,13.5679367061317,-1.82029166666684));
#24729=CARTESIAN_POINT('Ctrl Pts',(-13.8267841057906,14.5339683530659,-1.86195833333351));
#24730=CARTESIAN_POINT('Ctrl Pts',(-13.2690454743875,15.5,-1.90362500000018));
#24731=CARTESIAN_POINT('Ctrl Pts',(-13.8267841057906,16.4660316469341,-1.94529166666684));
#24732=CARTESIAN_POINT('Ctrl Pts',(-14.3845227371938,17.4320632938683,-1.98695833333351));
#24733=CARTESIAN_POINT('Ctrl Pts',(-15.5,17.4320632938683,-2.02862500000018));
#24734=CARTESIAN_POINT('Ctrl Pts',(-16.6154772628062,17.4320632938683,-2.07029166666685));
#24735=CARTESIAN_POINT('Ctrl Pts',(-17.1732158942094,16.4660316469341,-2.11195833333351));
#24736=CARTESIAN_POINT('Ctrl Pts',(-17.7309545256125,15.5,-2.15362500000018));
#24737=CARTESIAN_POINT('Ctrl Pts',(-17.1732158942094,14.5339683530659,-2.19529166666685));
#24738=CARTESIAN_POINT('Ctrl Pts',(-16.9678747970191,14.1783071398504,-2.21063196867905));
#24739=CARTESIAN_POINT('Ctrl Pts',(-16.6356236599184,13.9369173167914,-2.22824840486548));
#24740=CARTESIAN_POINT('Origin',(-15.5080107655896,15.6430062215135,1.38580563032467));
#24741=CARTESIAN_POINT('',(-16.4288320706156,14.2215513317122,-2.02512305032214));
#24742=CARTESIAN_POINT('Ctrl Pts',(-15.2436450846258,13.9406917842497,10.4122404735808));
#24743=CARTESIAN_POINT('Ctrl Pts',(-14.5054990725557,14.0620451873462,10.3753299573543));
#24744=CARTESIAN_POINT('Ctrl Pts',(-14.1314716057906,14.7098797632096,10.3411666666667));
#24745=CARTESIAN_POINT('Ctrl Pts',(-13.6752954743875,15.5,10.2995));
#24746=CARTESIAN_POINT('Ctrl Pts',(-14.1314716057906,16.2901202367904,10.2578333333333));
#24747=CARTESIAN_POINT('Ctrl Pts',(-14.5876477371938,17.0802404735808,10.2161666666667));
#24748=CARTESIAN_POINT('Ctrl Pts',(-15.5,17.0802404735808,10.1745));
#24749=CARTESIAN_POINT('Ctrl Pts',(-16.4123522628062,17.0802404735808,10.1328333333333));
#24750=CARTESIAN_POINT('Ctrl Pts',(-16.8685283942094,16.2901202367904,10.0911666666667));
#24751=CARTESIAN_POINT('Ctrl Pts',(-17.3247045256125,15.5,10.0495));
#24752=CARTESIAN_POINT('Ctrl Pts',(-16.8685283942094,14.7098797632096,10.0078333333333));
#24753=CARTESIAN_POINT('Ctrl Pts',(-16.4123522628062,13.9197595264192,9.96616666666665));
#24754=CARTESIAN_POINT('Ctrl Pts',(-15.5,13.9197595264192,9.92449999999998));
#24755=CARTESIAN_POINT('Ctrl Pts',(-14.5876477371938,13.9197595264192,9.88283333333331));
#24756=CARTESIAN_POINT('Ctrl Pts',(-14.1314716057906,14.7098797632096,9.84116666666665));
#24757=CARTESIAN_POINT('Ctrl Pts',(-13.6752954743875,15.5,9.79949999999998));
#24758=CARTESIAN_POINT('Ctrl Pts',(-14.1314716057906,16.2901202367904,9.75783333333331));
#24759=CARTESIAN_POINT('Ctrl Pts',(-14.5876477371938,17.0802404735808,9.71616666666665));
#24760=CARTESIAN_POINT('Ctrl Pts',(-15.5,17.0802404735808,9.67449999999998));
#24761=CARTESIAN_POINT('Ctrl Pts',(-16.4123522628062,17.0802404735808,9.63283333333331));
#24762=CARTESIAN_POINT('Ctrl Pts',(-16.8685283942094,16.2901202367904,9.59116666666664));
#24763=CARTESIAN_POINT('Ctrl Pts',(-17.3247045256125,15.5,9.54949999999998));
#24764=CARTESIAN_POINT('Ctrl Pts',(-16.8685283942094,14.7098797632096,9.50783333333331));
#24765=CARTESIAN_POINT('Ctrl Pts',(-16.4123522628062,13.9197595264192,9.46616666666664));
#24766=CARTESIAN_POINT('Ctrl Pts',(-15.5,13.9197595264192,9.42449999999998));
#24767=CARTESIAN_POINT('Ctrl Pts',(-14.5876477371938,13.9197595264192,9.38283333333331));
#24768=CARTESIAN_POINT('Ctrl Pts',(-14.1314716057906,14.7098797632096,9.34116666666664));
#24769=CARTESIAN_POINT('Ctrl Pts',(-13.6752954743875,15.5,9.29949999999997));
#24770=CARTESIAN_POINT('Ctrl Pts',(-14.1314716057906,16.2901202367904,9.25783333333331));
#24771=CARTESIAN_POINT('Ctrl Pts',(-14.5876477371938,17.0802404735808,9.21616666666664));
#24772=CARTESIAN_POINT('Ctrl Pts',(-15.5,17.0802404735808,9.17449999999997));
#24773=CARTESIAN_POINT('Ctrl Pts',(-16.4123522628062,17.0802404735808,9.13283333333331));
#24774=CARTESIAN_POINT('Ctrl Pts',(-16.8685283942094,16.2901202367904,9.09116666666664));
#24775=CARTESIAN_POINT('Ctrl Pts',(-17.3247045256125,15.5,9.04949999999997));
#24776=CARTESIAN_POINT('Ctrl Pts',(-16.8685283942094,14.7098797632096,9.0078333333333));
#24777=CARTESIAN_POINT('Ctrl Pts',(-16.4123522628062,13.9197595264192,8.96616666666664));
#24778=CARTESIAN_POINT('Ctrl Pts',(-15.5,13.9197595264192,8.92449999999997));
#24779=CARTESIAN_POINT('Ctrl Pts',(-14.5876477371938,13.9197595264192,8.8828333333333));
#24780=CARTESIAN_POINT('Ctrl Pts',(-14.1314716057906,14.7098797632096,8.84116666666664));
#24781=CARTESIAN_POINT('Ctrl Pts',(-13.6752954743875,15.5,8.79949999999997));
#24782=CARTESIAN_POINT('Ctrl Pts',(-14.1314716057906,16.2901202367904,8.7578333333333));
#24783=CARTESIAN_POINT('Ctrl Pts',(-14.5876477371938,17.0802404735808,8.71616666666663));
#24784=CARTESIAN_POINT('Ctrl Pts',(-15.5,17.0802404735808,8.67449999999997));
#24785=CARTESIAN_POINT('Ctrl Pts',(-16.4123522628062,17.0802404735808,8.6328333333333));
#24786=CARTESIAN_POINT('Ctrl Pts',(-16.8685283942094,16.2901202367904,8.59116666666663));
#24787=CARTESIAN_POINT('Ctrl Pts',(-17.3247045256125,15.5,8.54949999999996));
#24788=CARTESIAN_POINT('Ctrl Pts',(-16.8685283942094,14.7098797632096,8.50783333333329));
#24789=CARTESIAN_POINT('Ctrl Pts',(-16.4123522628062,13.9197595264192,8.46616666666663));
#24790=CARTESIAN_POINT('Ctrl Pts',(-15.5,13.9197595264192,8.42449999999996));
#24791=CARTESIAN_POINT('Ctrl Pts',(-14.5876477371938,13.9197595264192,8.38283333333329));
#24792=CARTESIAN_POINT('Ctrl Pts',(-14.1314716057906,14.7098797632096,8.34116666666663));
#24793=CARTESIAN_POINT('Ctrl Pts',(-13.6752954743875,15.5,8.29949999999996));
#24794=CARTESIAN_POINT('Ctrl Pts',(-14.1314716057906,16.2901202367904,8.25783333333329));
#24795=CARTESIAN_POINT('Ctrl Pts',(-14.5876477371938,17.0802404735808,8.21616666666663));
#24796=CARTESIAN_POINT('Ctrl Pts',(-15.5,17.0802404735808,8.17449999999996));
#24797=CARTESIAN_POINT('Ctrl Pts',(-16.4123522628062,17.0802404735808,8.13283333333329));
#24798=CARTESIAN_POINT('Ctrl Pts',(-16.8685283942094,16.2901202367904,8.09116666666663));
#24799=CARTESIAN_POINT('Ctrl Pts',(-17.3247045256125,15.5,8.04949999999996));
#24800=CARTESIAN_POINT('Ctrl Pts',(-16.8685283942094,14.7098797632096,8.00783333333329));
#24801=CARTESIAN_POINT('Ctrl Pts',(-16.4123522628062,13.9197595264192,7.96616666666662));
#24802=CARTESIAN_POINT('Ctrl Pts',(-15.5,13.9197595264192,7.92449999999996));
#24803=CARTESIAN_POINT('Ctrl Pts',(-14.5876477371938,13.9197595264192,7.88283333333329));
#24804=CARTESIAN_POINT('Ctrl Pts',(-14.1314716057906,14.7098797632096,7.84116666666662));
#24805=CARTESIAN_POINT('Ctrl Pts',(-13.6752954743875,15.5,7.79949999999995));
#24806=CARTESIAN_POINT('Ctrl Pts',(-14.1314716057906,16.2901202367904,7.75783333333329));
#24807=CARTESIAN_POINT('Ctrl Pts',(-14.5876477371938,17.0802404735808,7.71616666666662));
#24808=CARTESIAN_POINT('Ctrl Pts',(-15.5,17.0802404735808,7.67449999999995));
#24809=CARTESIAN_POINT('Ctrl Pts',(-16.4123522628062,17.0802404735808,7.63283333333328));
#24810=CARTESIAN_POINT('Ctrl Pts',(-16.8685283942094,16.2901202367904,7.59116666666662));
#24811=CARTESIAN_POINT('Ctrl Pts',(-17.3247045256125,15.5,7.54949999999995));
#24812=CARTESIAN_POINT('Ctrl Pts',(-16.8685283942094,14.7098797632096,7.50783333333328));
#24813=CARTESIAN_POINT('Ctrl Pts',(-16.4123522628062,13.9197595264192,7.46616666666662));
#24814=CARTESIAN_POINT('Ctrl Pts',(-15.5,13.9197595264192,7.42449999999995));
#24815=CARTESIAN_POINT('Ctrl Pts',(-14.5876477371938,13.9197595264192,7.38283333333328));
#24816=CARTESIAN_POINT('Ctrl Pts',(-14.1314716057906,14.7098797632096,7.34116666666661));
#24817=CARTESIAN_POINT('Ctrl Pts',(-13.6752954743875,15.5,7.29949999999995));
#24818=CARTESIAN_POINT('Ctrl Pts',(-14.1314716057906,16.2901202367904,7.25783333333328));
#24819=CARTESIAN_POINT('Ctrl Pts',(-14.5876477371938,17.0802404735808,7.21616666666661));
#24820=CARTESIAN_POINT('Ctrl Pts',(-15.5,17.0802404735808,7.17449999999995));
#24821=CARTESIAN_POINT('Ctrl Pts',(-16.4123522628062,17.0802404735808,7.13283333333328));
#24822=CARTESIAN_POINT('Ctrl Pts',(-16.8685283942094,16.2901202367904,7.09116666666661));
#24823=CARTESIAN_POINT('Ctrl Pts',(-17.3247045256125,15.5,7.04949999999994));
#24824=CARTESIAN_POINT('Ctrl Pts',(-16.8685283942094,14.7098797632096,7.00783333333328));
#24825=CARTESIAN_POINT('Ctrl Pts',(-16.4123522628062,13.9197595264192,6.96616666666661));
#24826=CARTESIAN_POINT('Ctrl Pts',(-15.5,13.9197595264192,6.92449999999994));
#24827=CARTESIAN_POINT('Ctrl Pts',(-14.5876477371938,13.9197595264192,6.88283333333327));
#24828=CARTESIAN_POINT('Ctrl Pts',(-14.1314716057906,14.7098797632096,6.84116666666661));
#24829=CARTESIAN_POINT('Ctrl Pts',(-13.6752954743875,15.5,6.79949999999994));
#24830=CARTESIAN_POINT('Ctrl Pts',(-14.1314716057906,16.2901202367904,6.75783333333327));
#24831=CARTESIAN_POINT('Ctrl Pts',(-14.5876477371938,17.0802404735808,6.71616666666661));
#24832=CARTESIAN_POINT('Ctrl Pts',(-15.5,17.0802404735808,6.67449999999994));
#24833=CARTESIAN_POINT('Ctrl Pts',(-16.4123522628062,17.0802404735808,6.63283333333327));
#24834=CARTESIAN_POINT('Ctrl Pts',(-16.8685283942094,16.2901202367904,6.59116666666661));
#24835=CARTESIAN_POINT('Ctrl Pts',(-17.3247045256125,15.5,6.54949999999994));
#24836=CARTESIAN_POINT('Ctrl Pts',(-16.8685283942094,14.7098797632096,6.50783333333327));
#24837=CARTESIAN_POINT('Ctrl Pts',(-16.4123522628062,13.9197595264192,6.4661666666666));
#24838=CARTESIAN_POINT('Ctrl Pts',(-15.5,13.9197595264192,6.42449999999994));
#24839=CARTESIAN_POINT('Ctrl Pts',(-14.5876477371938,13.9197595264192,6.38283333333327));
#24840=CARTESIAN_POINT('Ctrl Pts',(-14.1314716057906,14.7098797632096,6.3411666666666));
#24841=CARTESIAN_POINT('Ctrl Pts',(-13.6752954743875,15.5,6.29949999999993));
#24842=CARTESIAN_POINT('Ctrl Pts',(-14.1314716057906,16.2901202367904,6.25783333333327));
#24843=CARTESIAN_POINT('Ctrl Pts',(-14.5876477371938,17.0802404735808,6.2161666666666));
#24844=CARTESIAN_POINT('Ctrl Pts',(-15.5,17.0802404735808,6.17449999999993));
#24845=CARTESIAN_POINT('Ctrl Pts',(-16.4123522628062,17.0802404735808,6.13283333333326));
#24846=CARTESIAN_POINT('Ctrl Pts',(-16.8685283942094,16.2901202367904,6.0911666666666));
#24847=CARTESIAN_POINT('Ctrl Pts',(-17.3247045256125,15.5,6.04949999999993));
#24848=CARTESIAN_POINT('Ctrl Pts',(-16.8685283942094,14.7098797632096,6.00783333333326));
#24849=CARTESIAN_POINT('Ctrl Pts',(-16.4123522628062,13.9197595264192,5.9661666666666));
#24850=CARTESIAN_POINT('Ctrl Pts',(-15.5,13.9197595264192,5.92449999999993));
#24851=CARTESIAN_POINT('Ctrl Pts',(-14.5876477371938,13.9197595264192,5.88283333333326));
#24852=CARTESIAN_POINT('Ctrl Pts',(-14.1314716057906,14.7098797632096,5.8411666666666));
#24853=CARTESIAN_POINT('Ctrl Pts',(-13.6752954743875,15.5,5.79949999999993));
#24854=CARTESIAN_POINT('Ctrl Pts',(-14.1314716057906,16.2901202367904,5.75783333333326));
#24855=CARTESIAN_POINT('Ctrl Pts',(-14.5876477371938,17.0802404735808,5.71616666666659));
#24856=CARTESIAN_POINT('Ctrl Pts',(-15.5,17.0802404735808,5.67449999999993));
#24857=CARTESIAN_POINT('Ctrl Pts',(-16.4123522628062,17.0802404735808,5.63283333333326));
#24858=CARTESIAN_POINT('Ctrl Pts',(-16.8685283942094,16.2901202367904,5.59116666666659));
#24859=CARTESIAN_POINT('Ctrl Pts',(-17.3247045256125,15.5,5.54949999999992));
#24860=CARTESIAN_POINT('Ctrl Pts',(-16.8685283942094,14.7098797632096,5.50783333333326));
#24861=CARTESIAN_POINT('Ctrl Pts',(-16.4123522628062,13.9197595264192,5.46616666666659));
#24862=CARTESIAN_POINT('Ctrl Pts',(-15.5,13.9197595264192,5.42449999999992));
#24863=CARTESIAN_POINT('Ctrl Pts',(-14.5876477371938,13.9197595264192,5.38283333333326));
#24864=CARTESIAN_POINT('Ctrl Pts',(-14.1314716057906,14.7098797632096,5.34116666666659));
#24865=CARTESIAN_POINT('Ctrl Pts',(-13.6752954743875,15.5,5.29949999999992));
#24866=CARTESIAN_POINT('Ctrl Pts',(-14.1314716057906,16.2901202367904,5.25783333333325));
#24867=CARTESIAN_POINT('Ctrl Pts',(-14.5876477371938,17.0802404735808,5.21616666666659));
#24868=CARTESIAN_POINT('Ctrl Pts',(-15.5,17.0802404735808,5.17449999999992));
#24869=CARTESIAN_POINT('Ctrl Pts',(-16.4123522628062,17.0802404735808,5.13283333333325));
#24870=CARTESIAN_POINT('Ctrl Pts',(-16.8685283942094,16.2901202367904,5.09116666666658));
#24871=CARTESIAN_POINT('Ctrl Pts',(-17.3247045256125,15.5,5.04949999999992));
#24872=CARTESIAN_POINT('Ctrl Pts',(-16.8685283942094,14.7098797632096,5.00783333333325));
#24873=CARTESIAN_POINT('Ctrl Pts',(-16.4123522628062,13.9197595264192,4.96616666666658));
#24874=CARTESIAN_POINT('Ctrl Pts',(-15.5,13.9197595264192,4.92449999999992));
#24875=CARTESIAN_POINT('Ctrl Pts',(-14.5876477371938,13.9197595264192,4.88283333333325));
#24876=CARTESIAN_POINT('Ctrl Pts',(-14.1314716057906,14.7098797632096,4.84116666666658));
#24877=CARTESIAN_POINT('Ctrl Pts',(-13.6752954743875,15.5,4.79949999999991));
#24878=CARTESIAN_POINT('Ctrl Pts',(-14.1314716057906,16.2901202367904,4.75783333333325));
#24879=CARTESIAN_POINT('Ctrl Pts',(-14.5876477371938,17.0802404735808,4.71616666666658));
#24880=CARTESIAN_POINT('Ctrl Pts',(-15.5,17.0802404735808,4.67449999999991));
#24881=CARTESIAN_POINT('Ctrl Pts',(-16.4123522628062,17.0802404735808,4.63283333333325));
#24882=CARTESIAN_POINT('Ctrl Pts',(-16.8685283942094,16.2901202367904,4.59116666666658));
#24883=CARTESIAN_POINT('Ctrl Pts',(-17.3247045256125,15.5,4.54949999999991));
#24884=CARTESIAN_POINT('Ctrl Pts',(-16.8685283942094,14.7098797632096,4.50783333333324));
#24885=CARTESIAN_POINT('Ctrl Pts',(-16.4123522628062,13.9197595264192,4.46616666666658));
#24886=CARTESIAN_POINT('Ctrl Pts',(-15.5,13.9197595264192,4.42449999999991));
#24887=CARTESIAN_POINT('Ctrl Pts',(-14.5876477371938,13.9197595264192,4.38283333333324));
#24888=CARTESIAN_POINT('Ctrl Pts',(-14.1314716057906,14.7098797632096,4.34116666666657));
#24889=CARTESIAN_POINT('Ctrl Pts',(-13.6752954743875,15.5,4.29949999999991));
#24890=CARTESIAN_POINT('Ctrl Pts',(-14.1314716057906,16.2901202367904,4.25783333333324));
#24891=CARTESIAN_POINT('Ctrl Pts',(-14.5876477371938,17.0802404735808,4.21616666666657));
#24892=CARTESIAN_POINT('Ctrl Pts',(-15.5,17.0802404735808,4.17449999999991));
#24893=CARTESIAN_POINT('Ctrl Pts',(-16.4123522628062,17.0802404735808,4.13283333333324));
#24894=CARTESIAN_POINT('Ctrl Pts',(-16.8685283942094,16.2901202367904,4.09116666666657));
#24895=CARTESIAN_POINT('Ctrl Pts',(-17.3247045256125,15.5,4.0494999999999));
#24896=CARTESIAN_POINT('Ctrl Pts',(-16.8685283942094,14.7098797632096,4.00783333333324));
#24897=CARTESIAN_POINT('Ctrl Pts',(-16.4123522628062,13.9197595264192,3.96616666666657));
#24898=CARTESIAN_POINT('Ctrl Pts',(-15.5,13.9197595264192,3.9244999999999));
#24899=CARTESIAN_POINT('Ctrl Pts',(-14.5876477371938,13.9197595264192,3.88283333333323));
#24900=CARTESIAN_POINT('Ctrl Pts',(-14.1314716057906,14.7098797632096,3.84116666666657));
#24901=CARTESIAN_POINT('Ctrl Pts',(-13.6752954743875,15.5,3.7994999999999));
#24902=CARTESIAN_POINT('Ctrl Pts',(-14.1314716057906,16.2901202367904,3.75783333333323));
#24903=CARTESIAN_POINT('Ctrl Pts',(-14.5876477371938,17.0802404735808,3.71616666666657));
#24904=CARTESIAN_POINT('Ctrl Pts',(-15.5,17.0802404735808,3.6744999999999));
#24905=CARTESIAN_POINT('Ctrl Pts',(-16.4123522628062,17.0802404735808,3.63283333333323));
#24906=CARTESIAN_POINT('Ctrl Pts',(-16.8685283942094,16.2901202367904,3.59116666666656));
#24907=CARTESIAN_POINT('Ctrl Pts',(-17.3247045256125,15.5,3.5494999999999));
#24908=CARTESIAN_POINT('Ctrl Pts',(-16.8685283942094,14.7098797632096,3.50783333333323));
#24909=CARTESIAN_POINT('Ctrl Pts',(-16.4123522628062,13.9197595264192,3.46616666666656));
#24910=CARTESIAN_POINT('Ctrl Pts',(-15.5,13.9197595264192,3.4244999999999));
#24911=CARTESIAN_POINT('Ctrl Pts',(-14.5876477371938,13.9197595264192,3.38283333333323));
#24912=CARTESIAN_POINT('Ctrl Pts',(-14.1314716057906,14.7098797632096,3.34116666666656));
#24913=CARTESIAN_POINT('Ctrl Pts',(-13.6752954743875,15.5,3.29949999999989));
#24914=CARTESIAN_POINT('Ctrl Pts',(-14.1314716057906,16.2901202367904,3.25783333333323));
#24915=CARTESIAN_POINT('Ctrl Pts',(-14.5876477371938,17.0802404735808,3.21616666666656));
#24916=CARTESIAN_POINT('Ctrl Pts',(-15.5,17.0802404735808,3.17449999999989));
#24917=CARTESIAN_POINT('Ctrl Pts',(-16.4123522628062,17.0802404735808,3.13283333333323));
#24918=CARTESIAN_POINT('Ctrl Pts',(-16.8685283942094,16.2901202367904,3.09116666666656));
#24919=CARTESIAN_POINT('Ctrl Pts',(-17.3247045256125,15.5,3.04949999999989));
#24920=CARTESIAN_POINT('Ctrl Pts',(-16.8685283942094,14.7098797632096,3.00783333333322));
#24921=CARTESIAN_POINT('Ctrl Pts',(-16.4123522628062,13.9197595264192,2.96616666666656));
#24922=CARTESIAN_POINT('Ctrl Pts',(-15.5,13.9197595264192,2.92449999999989));
#24923=CARTESIAN_POINT('Ctrl Pts',(-14.5876477371938,13.9197595264192,2.88283333333322));
#24924=CARTESIAN_POINT('Ctrl Pts',(-14.1314716057906,14.7098797632096,2.84116666666655));
#24925=CARTESIAN_POINT('Ctrl Pts',(-13.6752954743875,15.5,2.79949999999989));
#24926=CARTESIAN_POINT('Ctrl Pts',(-14.1314716057906,16.2901202367904,2.75783333333322));
#24927=CARTESIAN_POINT('Ctrl Pts',(-14.5876477371938,17.0802404735808,2.71616666666655));
#24928=CARTESIAN_POINT('Ctrl Pts',(-15.5,17.0802404735808,2.67449999999989));
#24929=CARTESIAN_POINT('Ctrl Pts',(-16.4123522628062,17.0802404735808,2.63283333333322));
#24930=CARTESIAN_POINT('Ctrl Pts',(-16.8685283942094,16.2901202367904,2.59116666666655));
#24931=CARTESIAN_POINT('Ctrl Pts',(-17.3247045256125,15.5,2.54949999999988));
#24932=CARTESIAN_POINT('Ctrl Pts',(-16.8685283942094,14.7098797632096,2.50783333333322));
#24933=CARTESIAN_POINT('Ctrl Pts',(-16.4123522628062,13.9197595264192,2.46616666666655));
#24934=CARTESIAN_POINT('Ctrl Pts',(-15.5,13.9197595264192,2.42449999999988));
#24935=CARTESIAN_POINT('Ctrl Pts',(-14.5876477371938,13.9197595264192,2.38283333333321));
#24936=CARTESIAN_POINT('Ctrl Pts',(-14.1314716057906,14.7098797632096,2.34116666666655));
#24937=CARTESIAN_POINT('Ctrl Pts',(-13.6752954743875,15.5,2.29949999999988));
#24938=CARTESIAN_POINT('Ctrl Pts',(-14.1314716057906,16.2901202367904,2.25783333333321));
#24939=CARTESIAN_POINT('Ctrl Pts',(-14.5876477371938,17.0802404735808,2.21616666666655));
#24940=CARTESIAN_POINT('Ctrl Pts',(-15.5,17.0802404735808,2.17449999999988));
#24941=CARTESIAN_POINT('Ctrl Pts',(-16.4123522628062,17.0802404735808,2.13283333333321));
#24942=CARTESIAN_POINT('Ctrl Pts',(-16.8685283942094,16.2901202367904,2.09116666666655));
#24943=CARTESIAN_POINT('Ctrl Pts',(-17.3247045256125,15.5,2.04949999999988));
#24944=CARTESIAN_POINT('Ctrl Pts',(-16.8685283942094,14.7098797632096,2.00783333333321));
#24945=CARTESIAN_POINT('Ctrl Pts',(-16.4123522628062,13.9197595264192,1.96616666666654));
#24946=CARTESIAN_POINT('Ctrl Pts',(-15.5,13.9197595264192,1.92449999999988));
#24947=CARTESIAN_POINT('Ctrl Pts',(-14.5876477371938,13.9197595264192,1.88283333333321));
#24948=CARTESIAN_POINT('Ctrl Pts',(-14.1314716057906,14.7098797632096,1.84116666666654));
#24949=CARTESIAN_POINT('Ctrl Pts',(-13.6752954743875,15.5,1.79949999999987));
#24950=CARTESIAN_POINT('Ctrl Pts',(-14.1314716057906,16.2901202367904,1.75783333333321));
#24951=CARTESIAN_POINT('Ctrl Pts',(-14.5876477371938,17.0802404735808,1.71616666666654));
#24952=CARTESIAN_POINT('Ctrl Pts',(-15.5,17.0802404735808,1.67449999999987));
#24953=CARTESIAN_POINT('Ctrl Pts',(-16.4123522628062,17.0802404735808,1.63283333333321));
#24954=CARTESIAN_POINT('Ctrl Pts',(-16.8685283942094,16.2901202367904,1.59116666666654));
#24955=CARTESIAN_POINT('Ctrl Pts',(-17.3247045256125,15.5,1.54949999999987));
#24956=CARTESIAN_POINT('Ctrl Pts',(-16.8685283942094,14.7098797632096,1.5078333333332));
#24957=CARTESIAN_POINT('Ctrl Pts',(-16.4123522628062,13.9197595264192,1.46616666666654));
#24958=CARTESIAN_POINT('Ctrl Pts',(-15.5,13.9197595264192,1.42449999999987));
#24959=CARTESIAN_POINT('Ctrl Pts',(-14.5876477371938,13.9197595264192,1.3828333333332));
#24960=CARTESIAN_POINT('Ctrl Pts',(-14.1314716057906,14.7098797632096,1.34116666666653));
#24961=CARTESIAN_POINT('Ctrl Pts',(-13.6752954743875,15.5,1.29949999999987));
#24962=CARTESIAN_POINT('Ctrl Pts',(-14.1314716057906,16.2901202367904,1.2578333333332));
#24963=CARTESIAN_POINT('Ctrl Pts',(-14.5876477371938,17.0802404735808,1.21616666666653));
#24964=CARTESIAN_POINT('Ctrl Pts',(-15.5,17.0802404735808,1.17449999999986));
#24965=CARTESIAN_POINT('Ctrl Pts',(-16.4123522628062,17.0802404735808,1.1328333333332));
#24966=CARTESIAN_POINT('Ctrl Pts',(-16.8685283942094,16.2901202367904,1.09116666666653));
#24967=CARTESIAN_POINT('Ctrl Pts',(-17.3247045256125,15.5,1.04949999999987));
#24968=CARTESIAN_POINT('Ctrl Pts',(-16.8685283942094,14.7098797632096,1.0078333333332));
#24969=CARTESIAN_POINT('Ctrl Pts',(-16.4123522628062,13.9197595264192,0.96616666666653));
#24970=CARTESIAN_POINT('Ctrl Pts',(-15.5,13.9197595264192,0.924499999999863));
#24971=CARTESIAN_POINT('Ctrl Pts',(-14.5876477371938,13.9197595264192,0.882833333333196));
#24972=CARTESIAN_POINT('Ctrl Pts',(-14.1314716057906,14.7098797632096,0.841166666666529));
#24973=CARTESIAN_POINT('Ctrl Pts',(-13.6752954743875,15.5,0.799499999999861));
#24974=CARTESIAN_POINT('Ctrl Pts',(-14.1314716057906,16.2901202367904,0.757833333333194));
#24975=CARTESIAN_POINT('Ctrl Pts',(-14.5876477371938,17.0802404735808,0.716166666666527));
#24976=CARTESIAN_POINT('Ctrl Pts',(-15.5,17.0802404735808,0.674499999999859));
#24977=CARTESIAN_POINT('Ctrl Pts',(-16.4123522628062,17.0802404735808,0.632833333333192));
#24978=CARTESIAN_POINT('Ctrl Pts',(-16.8685283942094,16.2901202367904,0.591166666666525));
#24979=CARTESIAN_POINT('Ctrl Pts',(-17.3247045256125,15.5,0.549499999999857));
#24980=CARTESIAN_POINT('Ctrl Pts',(-16.8685283942094,14.7098797632096,0.50783333333319));
#24981=CARTESIAN_POINT('Ctrl Pts',(-16.4123522628062,13.9197595264192,0.466166666666523));
#24982=CARTESIAN_POINT('Ctrl Pts',(-15.5,13.9197595264192,0.424499999999856));
#24983=CARTESIAN_POINT('Ctrl Pts',(-14.5876477371938,13.9197595264192,0.382833333333188));
#24984=CARTESIAN_POINT('Ctrl Pts',(-14.1314716057906,14.7098797632096,0.341166666666521));
#24985=CARTESIAN_POINT('Ctrl Pts',(-13.6752954743875,15.5,0.299499999999854));
#24986=CARTESIAN_POINT('Ctrl Pts',(-14.1314716057906,16.2901202367904,0.257833333333186));
#24987=CARTESIAN_POINT('Ctrl Pts',(-14.5876477371938,17.0802404735808,0.216166666666519));
#24988=CARTESIAN_POINT('Ctrl Pts',(-15.5,17.0802404735808,0.174499999999852));
#24989=CARTESIAN_POINT('Ctrl Pts',(-16.4123522628062,17.0802404735808,0.132833333333185));
#24990=CARTESIAN_POINT('Ctrl Pts',(-16.8685283942094,16.2901202367904,0.0911666666665173));
#24991=CARTESIAN_POINT('Ctrl Pts',(-17.3247045256125,15.5,0.04949999999985));
#24992=CARTESIAN_POINT('Ctrl Pts',(-16.8685283942094,14.7098797632096,0.00783333333318273));
#24993=CARTESIAN_POINT('Ctrl Pts',(-16.4123522628062,13.9197595264192,-0.0338333333334846));
#24994=CARTESIAN_POINT('Ctrl Pts',(-15.5,13.9197595264192,-0.0755000000001518));
#24995=CARTESIAN_POINT('Ctrl Pts',(-14.5876477371938,13.9197595264192,-0.117166666666817));
#24996=CARTESIAN_POINT('Ctrl Pts',(-14.1314716057906,14.7098797632096,-0.158833333333485));
#24997=CARTESIAN_POINT('Ctrl Pts',(-13.6752954743875,15.5,-0.200500000000152));
#24998=CARTESIAN_POINT('Ctrl Pts',(-14.1314716057906,16.2901202367904,-0.242166666666819));
#24999=CARTESIAN_POINT('Ctrl Pts',(-14.5876477371938,17.0802404735808,-0.283833333333487));
#25000=CARTESIAN_POINT('Ctrl Pts',(-15.5,17.0802404735808,-0.325500000000154));
#25001=CARTESIAN_POINT('Ctrl Pts',(-16.4123522628062,17.0802404735808,-0.367166666666821));
#25002=CARTESIAN_POINT('Ctrl Pts',(-16.8685283942094,16.2901202367904,-0.408833333333488));
#25003=CARTESIAN_POINT('Ctrl Pts',(-17.3247045256125,15.5,-0.450500000000156));
#25004=CARTESIAN_POINT('Ctrl Pts',(-16.8685283942094,14.7098797632096,-0.492166666666823));
#25005=CARTESIAN_POINT('Ctrl Pts',(-16.4123522628062,13.9197595264192,-0.53383333333349));
#25006=CARTESIAN_POINT('Ctrl Pts',(-15.5,13.9197595264192,-0.575500000000157));
#25007=CARTESIAN_POINT('Ctrl Pts',(-14.5876477371938,13.9197595264192,-0.617166666666825));
#25008=CARTESIAN_POINT('Ctrl Pts',(-14.1314716057906,14.7098797632096,-0.658833333333492));
#25009=CARTESIAN_POINT('Ctrl Pts',(-13.6752954743875,15.5,-0.700500000000159));
#25010=CARTESIAN_POINT('Ctrl Pts',(-14.1314716057906,16.2901202367904,-0.742166666666827));
#25011=CARTESIAN_POINT('Ctrl Pts',(-14.5876477371938,17.0802404735808,-0.783833333333494));
#25012=CARTESIAN_POINT('Ctrl Pts',(-15.5,17.0802404735808,-0.825500000000161));
#25013=CARTESIAN_POINT('Ctrl Pts',(-16.4123522628062,17.0802404735808,-0.867166666666829));
#25014=CARTESIAN_POINT('Ctrl Pts',(-16.8685283942094,16.2901202367904,-0.908833333333496));
#25015=CARTESIAN_POINT('Ctrl Pts',(-17.3247045256125,15.5,-0.950500000000163));
#25016=CARTESIAN_POINT('Ctrl Pts',(-16.8685283942094,14.7098797632096,-0.99216666666683));
#25017=CARTESIAN_POINT('Ctrl Pts',(-16.4123522628062,13.9197595264192,-1.0338333333335));
#25018=CARTESIAN_POINT('Ctrl Pts',(-15.5,13.9197595264192,-1.07550000000016));
#25019=CARTESIAN_POINT('Ctrl Pts',(-14.5876477371938,13.9197595264192,-1.11716666666683));
#25020=CARTESIAN_POINT('Ctrl Pts',(-14.1314716057906,14.7098797632096,-1.1588333333335));
#25021=CARTESIAN_POINT('Ctrl Pts',(-13.6752954743875,15.5,-1.20050000000017));
#25022=CARTESIAN_POINT('Ctrl Pts',(-14.1314716057906,16.2901202367904,-1.24216666666683));
#25023=CARTESIAN_POINT('Ctrl Pts',(-14.5876477371938,17.0802404735808,-1.2838333333335));
#25024=CARTESIAN_POINT('Ctrl Pts',(-15.5,17.0802404735808,-1.32550000000017));
#25025=CARTESIAN_POINT('Ctrl Pts',(-16.4123522628062,17.0802404735808,-1.36716666666683));
#25026=CARTESIAN_POINT('Ctrl Pts',(-16.8685283942094,16.2901202367904,-1.4088333333335));
#25027=CARTESIAN_POINT('Ctrl Pts',(-17.3247045256125,15.5,-1.45050000000017));
#25028=CARTESIAN_POINT('Ctrl Pts',(-16.8685283942094,14.7098797632096,-1.49216666666684));
#25029=CARTESIAN_POINT('Ctrl Pts',(-16.4123522628062,13.9197595264192,-1.5338333333335));
#25030=CARTESIAN_POINT('Ctrl Pts',(-15.5,13.9197595264192,-1.57550000000017));
#25031=CARTESIAN_POINT('Ctrl Pts',(-14.5876477371938,13.9197595264192,-1.61716666666684));
#25032=CARTESIAN_POINT('Ctrl Pts',(-14.1314716057906,14.7098797632096,-1.65883333333351));
#25033=CARTESIAN_POINT('Ctrl Pts',(-13.6752954743875,15.5,-1.70050000000017));
#25034=CARTESIAN_POINT('Ctrl Pts',(-14.1314716057906,16.2901202367904,-1.74216666666684));
#25035=CARTESIAN_POINT('Ctrl Pts',(-14.5876477371938,17.0802404735808,-1.78383333333351));
#25036=CARTESIAN_POINT('Ctrl Pts',(-15.5,17.0802404735808,-1.82550000000017));
#25037=CARTESIAN_POINT('Ctrl Pts',(-16.4123522628062,17.0802404735808,-1.86716666666684));
#25038=CARTESIAN_POINT('Ctrl Pts',(-16.8685283942094,16.2901202367904,-1.90883333333351));
#25039=CARTESIAN_POINT('Ctrl Pts',(-17.3247045256125,15.5,-1.95050000000018));
#25040=CARTESIAN_POINT('Ctrl Pts',(-16.8685283942094,14.7098797632096,-1.99216666666684));
#25041=CARTESIAN_POINT('Ctrl Pts',(-16.7005831533691,14.4189900731849,-2.00750661517932));
#25042=CARTESIAN_POINT('Ctrl Pts',(-16.4288360540161,14.2215542486879,-2.02512301646327));
#25043=CARTESIAN_POINT('',(-16.6356236599184,13.9369173167914,-2.22824840486548));
#25044=CARTESIAN_POINT('Ctrl Pts',(-15.5,17.4320632938683,11.440125));
#25045=CARTESIAN_POINT('Ctrl Pts',(-16.6154772628062,17.4320632938683,11.3984583333333));
#25046=CARTESIAN_POINT('Ctrl Pts',(-17.1732158942094,16.4660316469341,11.3567916666667));
#25047=CARTESIAN_POINT('Ctrl Pts',(-17.7309545256125,15.5,11.315125));
#25048=CARTESIAN_POINT('Ctrl Pts',(-17.1732158942094,14.5339683530659,11.2734583333333));
#25049=CARTESIAN_POINT('Ctrl Pts',(-16.6154772628062,13.5679367061317,11.2317916666667));
#25050=CARTESIAN_POINT('Ctrl Pts',(-15.5,13.5679367061317,11.190125));
#25051=CARTESIAN_POINT('Ctrl Pts',(-14.3845227371938,13.5679367061317,11.1484583333333));
#25052=CARTESIAN_POINT('Ctrl Pts',(-13.8267841057906,14.5339683530659,11.1067916666667));
#25053=CARTESIAN_POINT('Ctrl Pts',(-13.2690454743875,15.5,11.065125));
#25054=CARTESIAN_POINT('Ctrl Pts',(-13.8267841057906,16.4660316469341,11.0234583333333));
#25055=CARTESIAN_POINT('Ctrl Pts',(-14.3845227371938,17.4320632938683,10.9817916666667));
#25056=CARTESIAN_POINT('Ctrl Pts',(-15.5,17.4320632938683,10.940125));
#25057=CARTESIAN_POINT('Ctrl Pts',(-16.6154772628062,17.4320632938683,10.8984583333333));
#25058=CARTESIAN_POINT('Ctrl Pts',(-17.1732158942094,16.4660316469341,10.8567916666667));
#25059=CARTESIAN_POINT('Ctrl Pts',(-17.7309545256125,15.5,10.815125));
#25060=CARTESIAN_POINT('Ctrl Pts',(-17.1732158942094,14.5339683530659,10.7734583333333));
#25061=CARTESIAN_POINT('Ctrl Pts',(-16.6154772628062,13.5679367061317,10.7317916666667));
#25062=CARTESIAN_POINT('Ctrl Pts',(-15.5,13.5679367061317,10.690125));
#25063=CARTESIAN_POINT('Ctrl Pts',(-14.3845227371938,13.5679367061317,10.6484583333333));
#25064=CARTESIAN_POINT('Ctrl Pts',(-13.8267841057906,14.5339683530659,10.6067916666667));
#25065=CARTESIAN_POINT('Ctrl Pts',(-13.2690454743875,15.5,10.565125));
#25066=CARTESIAN_POINT('Ctrl Pts',(-13.8267841057906,16.4660316469341,10.5234583333333));
#25067=CARTESIAN_POINT('Ctrl Pts',(-14.3845227371938,17.4320632938683,10.4817916666667));
#25068=CARTESIAN_POINT('Ctrl Pts',(-15.5,17.4320632938683,10.440125));
#25069=CARTESIAN_POINT('Ctrl Pts',(-16.6154772628062,17.4320632938683,10.3984583333333));
#25070=CARTESIAN_POINT('Ctrl Pts',(-17.1732158942094,16.4660316469341,10.3567916666667));
#25071=CARTESIAN_POINT('Ctrl Pts',(-17.7309545256125,15.5,10.315125));
#25072=CARTESIAN_POINT('Ctrl Pts',(-17.1732158942094,14.5339683530659,10.2734583333333));
#25073=CARTESIAN_POINT('Ctrl Pts',(-16.6154772628062,13.5679367061317,10.2317916666667));
#25074=CARTESIAN_POINT('Ctrl Pts',(-15.5,13.5679367061317,10.190125));
#25075=CARTESIAN_POINT('Ctrl Pts',(-14.3845227371938,13.5679367061317,10.1484583333333));
#25076=CARTESIAN_POINT('Ctrl Pts',(-13.8267841057906,14.5339683530659,10.1067916666666));
#25077=CARTESIAN_POINT('Ctrl Pts',(-13.2690454743875,15.5,10.065125));
#25078=CARTESIAN_POINT('Ctrl Pts',(-13.8267841057906,16.4660316469341,10.0234583333333));
#25079=CARTESIAN_POINT('Ctrl Pts',(-14.3845227371938,17.4320632938683,9.98179166666664));
#25080=CARTESIAN_POINT('Ctrl Pts',(-15.5,17.4320632938683,9.94012499999998));
#25081=CARTESIAN_POINT('Ctrl Pts',(-16.6154772628062,17.4320632938683,9.89845833333331));
#25082=CARTESIAN_POINT('Ctrl Pts',(-17.1732158942094,16.4660316469341,9.85679166666664));
#25083=CARTESIAN_POINT('Ctrl Pts',(-17.7309545256125,15.5,9.81512499999998));
#25084=CARTESIAN_POINT('Ctrl Pts',(-17.1732158942094,14.5339683530659,9.77345833333331));
#25085=CARTESIAN_POINT('Ctrl Pts',(-16.6154772628062,13.5679367061317,9.73179166666664));
#25086=CARTESIAN_POINT('Ctrl Pts',(-15.5,13.5679367061317,9.69012499999998));
#25087=CARTESIAN_POINT('Ctrl Pts',(-14.3845227371938,13.5679367061317,9.64845833333331));
#25088=CARTESIAN_POINT('Ctrl Pts',(-13.8267841057906,14.5339683530659,9.60679166666664));
#25089=CARTESIAN_POINT('Ctrl Pts',(-13.2690454743875,15.5,9.56512499999998));
#25090=CARTESIAN_POINT('Ctrl Pts',(-13.8267841057906,16.4660316469341,9.52345833333331));
#25091=CARTESIAN_POINT('Ctrl Pts',(-14.3845227371938,17.4320632938683,9.48179166666664));
#25092=CARTESIAN_POINT('Ctrl Pts',(-15.5,17.4320632938683,9.44012499999997));
#25093=CARTESIAN_POINT('Ctrl Pts',(-16.6154772628062,17.4320632938683,9.39845833333331));
#25094=CARTESIAN_POINT('Ctrl Pts',(-17.1732158942094,16.4660316469341,9.35679166666664));
#25095=CARTESIAN_POINT('Ctrl Pts',(-17.7309545256125,15.5,9.31512499999997));
#25096=CARTESIAN_POINT('Ctrl Pts',(-17.1732158942094,14.5339683530659,9.2734583333333));
#25097=CARTESIAN_POINT('Ctrl Pts',(-16.6154772628062,13.5679367061317,9.23179166666664));
#25098=CARTESIAN_POINT('Ctrl Pts',(-15.5,13.5679367061317,9.19012499999997));
#25099=CARTESIAN_POINT('Ctrl Pts',(-14.3845227371938,13.5679367061317,9.1484583333333));
#25100=CARTESIAN_POINT('Ctrl Pts',(-13.8267841057906,14.5339683530659,9.10679166666664));
#25101=CARTESIAN_POINT('Ctrl Pts',(-13.2690454743875,15.5,9.06512499999997));
#25102=CARTESIAN_POINT('Ctrl Pts',(-13.8267841057906,16.4660316469341,9.0234583333333));
#25103=CARTESIAN_POINT('Ctrl Pts',(-14.3845227371938,17.4320632938683,8.98179166666663));
#25104=CARTESIAN_POINT('Ctrl Pts',(-15.5,17.4320632938683,8.94012499999997));
#25105=CARTESIAN_POINT('Ctrl Pts',(-16.6154772628062,17.4320632938683,8.8984583333333));
#25106=CARTESIAN_POINT('Ctrl Pts',(-17.1732158942094,16.4660316469341,8.85679166666663));
#25107=CARTESIAN_POINT('Ctrl Pts',(-17.7309545256125,15.5,8.81512499999996));
#25108=CARTESIAN_POINT('Ctrl Pts',(-17.1732158942094,14.5339683530659,8.7734583333333));
#25109=CARTESIAN_POINT('Ctrl Pts',(-16.6154772628062,13.5679367061317,8.73179166666663));
#25110=CARTESIAN_POINT('Ctrl Pts',(-15.5,13.5679367061317,8.69012499999996));
#25111=CARTESIAN_POINT('Ctrl Pts',(-14.3845227371938,13.5679367061317,8.64845833333329));
#25112=CARTESIAN_POINT('Ctrl Pts',(-13.8267841057906,14.5339683530659,8.60679166666663));
#25113=CARTESIAN_POINT('Ctrl Pts',(-13.2690454743875,15.5,8.56512499999996));
#25114=CARTESIAN_POINT('Ctrl Pts',(-13.8267841057906,16.4660316469341,8.52345833333329));
#25115=CARTESIAN_POINT('Ctrl Pts',(-14.3845227371938,17.4320632938683,8.48179166666663));
#25116=CARTESIAN_POINT('Ctrl Pts',(-15.5,17.4320632938683,8.44012499999996));
#25117=CARTESIAN_POINT('Ctrl Pts',(-16.6154772628062,17.4320632938683,8.39845833333329));
#25118=CARTESIAN_POINT('Ctrl Pts',(-17.1732158942094,16.4660316469341,8.35679166666662));
#25119=CARTESIAN_POINT('Ctrl Pts',(-17.7309545256125,15.5,8.31512499999996));
#25120=CARTESIAN_POINT('Ctrl Pts',(-17.1732158942094,14.5339683530659,8.27345833333329));
#25121=CARTESIAN_POINT('Ctrl Pts',(-16.6154772628062,13.5679367061317,8.23179166666662));
#25122=CARTESIAN_POINT('Ctrl Pts',(-15.5,13.5679367061317,8.19012499999996));
#25123=CARTESIAN_POINT('Ctrl Pts',(-14.3845227371938,13.5679367061317,8.14845833333329));
#25124=CARTESIAN_POINT('Ctrl Pts',(-13.8267841057906,14.5339683530659,8.10679166666662));
#25125=CARTESIAN_POINT('Ctrl Pts',(-13.2690454743875,15.5,8.06512499999995));
#25126=CARTESIAN_POINT('Ctrl Pts',(-13.8267841057906,16.4660316469341,8.02345833333329));
#25127=CARTESIAN_POINT('Ctrl Pts',(-14.3845227371938,17.4320632938683,7.98179166666662));
#25128=CARTESIAN_POINT('Ctrl Pts',(-15.5,17.4320632938683,7.94012499999995));
#25129=CARTESIAN_POINT('Ctrl Pts',(-16.6154772628062,17.4320632938683,7.89845833333329));
#25130=CARTESIAN_POINT('Ctrl Pts',(-17.1732158942094,16.4660316469341,7.85679166666662));
#25131=CARTESIAN_POINT('Ctrl Pts',(-17.7309545256125,15.5,7.81512499999995));
#25132=CARTESIAN_POINT('Ctrl Pts',(-17.1732158942094,14.5339683530659,7.77345833333328));
#25133=CARTESIAN_POINT('Ctrl Pts',(-16.6154772628062,13.5679367061317,7.73179166666662));
#25134=CARTESIAN_POINT('Ctrl Pts',(-15.5,13.5679367061317,7.69012499999995));
#25135=CARTESIAN_POINT('Ctrl Pts',(-14.3845227371938,13.5679367061317,7.64845833333328));
#25136=CARTESIAN_POINT('Ctrl Pts',(-13.8267841057906,14.5339683530659,7.60679166666661));
#25137=CARTESIAN_POINT('Ctrl Pts',(-13.2690454743875,15.5,7.56512499999995));
#25138=CARTESIAN_POINT('Ctrl Pts',(-13.8267841057906,16.4660316469341,7.52345833333328));
#25139=CARTESIAN_POINT('Ctrl Pts',(-14.3845227371938,17.4320632938683,7.48179166666661));
#25140=CARTESIAN_POINT('Ctrl Pts',(-15.5,17.4320632938683,7.44012499999995));
#25141=CARTESIAN_POINT('Ctrl Pts',(-16.6154772628062,17.4320632938683,7.39845833333328));
#25142=CARTESIAN_POINT('Ctrl Pts',(-17.1732158942094,16.4660316469341,7.35679166666661));
#25143=CARTESIAN_POINT('Ctrl Pts',(-17.7309545256125,15.5,7.31512499999995));
#25144=CARTESIAN_POINT('Ctrl Pts',(-17.1732158942094,14.5339683530659,7.27345833333328));
#25145=CARTESIAN_POINT('Ctrl Pts',(-16.6154772628062,13.5679367061317,7.23179166666661));
#25146=CARTESIAN_POINT('Ctrl Pts',(-15.5,13.5679367061317,7.19012499999994));
#25147=CARTESIAN_POINT('Ctrl Pts',(-14.3845227371938,13.5679367061317,7.14845833333328));
#25148=CARTESIAN_POINT('Ctrl Pts',(-13.8267841057906,14.5339683530659,7.10679166666661));
#25149=CARTESIAN_POINT('Ctrl Pts',(-13.2690454743875,15.5,7.06512499999994));
#25150=CARTESIAN_POINT('Ctrl Pts',(-13.8267841057906,16.4660316469341,7.02345833333327));
#25151=CARTESIAN_POINT('Ctrl Pts',(-14.3845227371938,17.4320632938683,6.98179166666661));
#25152=CARTESIAN_POINT('Ctrl Pts',(-15.5,17.4320632938683,6.94012499999994));
#25153=CARTESIAN_POINT('Ctrl Pts',(-16.6154772628062,17.4320632938683,6.89845833333327));
#25154=CARTESIAN_POINT('Ctrl Pts',(-17.1732158942094,16.4660316469341,6.8567916666666));
#25155=CARTESIAN_POINT('Ctrl Pts',(-17.7309545256125,15.5,6.81512499999994));
#25156=CARTESIAN_POINT('Ctrl Pts',(-17.1732158942094,14.5339683530659,6.77345833333327));
#25157=CARTESIAN_POINT('Ctrl Pts',(-16.6154772628062,13.5679367061317,6.7317916666666));
#25158=CARTESIAN_POINT('Ctrl Pts',(-15.5,13.5679367061317,6.69012499999994));
#25159=CARTESIAN_POINT('Ctrl Pts',(-14.3845227371938,13.5679367061317,6.64845833333327));
#25160=CARTESIAN_POINT('Ctrl Pts',(-13.8267841057906,14.5339683530659,6.6067916666666));
#25161=CARTESIAN_POINT('Ctrl Pts',(-13.2690454743875,15.5,6.56512499999993));
#25162=CARTESIAN_POINT('Ctrl Pts',(-13.8267841057906,16.4660316469341,6.52345833333327));
#25163=CARTESIAN_POINT('Ctrl Pts',(-14.3845227371938,17.4320632938683,6.4817916666666));
#25164=CARTESIAN_POINT('Ctrl Pts',(-15.5,17.4320632938683,6.44012499999993));
#25165=CARTESIAN_POINT('Ctrl Pts',(-16.6154772628062,17.4320632938683,6.39845833333327));
#25166=CARTESIAN_POINT('Ctrl Pts',(-17.1732158942094,16.4660316469341,6.3567916666666));
#25167=CARTESIAN_POINT('Ctrl Pts',(-17.7309545256125,15.5,6.31512499999993));
#25168=CARTESIAN_POINT('Ctrl Pts',(-17.1732158942094,14.5339683530659,6.27345833333326));
#25169=CARTESIAN_POINT('Ctrl Pts',(-16.6154772628062,13.5679367061317,6.2317916666666));
#25170=CARTESIAN_POINT('Ctrl Pts',(-15.5,13.5679367061317,6.19012499999993));
#25171=CARTESIAN_POINT('Ctrl Pts',(-14.3845227371938,13.5679367061317,6.14845833333326));
#25172=CARTESIAN_POINT('Ctrl Pts',(-13.8267841057906,14.5339683530659,6.10679166666659));
#25173=CARTESIAN_POINT('Ctrl Pts',(-13.2690454743875,15.5,6.06512499999993));
#25174=CARTESIAN_POINT('Ctrl Pts',(-13.8267841057906,16.4660316469341,6.02345833333326));
#25175=CARTESIAN_POINT('Ctrl Pts',(-14.3845227371938,17.4320632938683,5.98179166666659));
#25176=CARTESIAN_POINT('Ctrl Pts',(-15.5,17.4320632938683,5.94012499999993));
#25177=CARTESIAN_POINT('Ctrl Pts',(-16.6154772628062,17.4320632938683,5.89845833333326));
#25178=CARTESIAN_POINT('Ctrl Pts',(-17.1732158942094,16.4660316469341,5.85679166666659));
#25179=CARTESIAN_POINT('Ctrl Pts',(-17.7309545256125,15.5,5.81512499999992));
#25180=CARTESIAN_POINT('Ctrl Pts',(-17.1732158942094,14.5339683530659,5.77345833333326));
#25181=CARTESIAN_POINT('Ctrl Pts',(-16.6154772628062,13.5679367061317,5.73179166666659));
#25182=CARTESIAN_POINT('Ctrl Pts',(-15.5,13.5679367061317,5.69012499999992));
#25183=CARTESIAN_POINT('Ctrl Pts',(-14.3845227371938,13.5679367061317,5.64845833333326));
#25184=CARTESIAN_POINT('Ctrl Pts',(-13.8267841057906,14.5339683530659,5.60679166666659));
#25185=CARTESIAN_POINT('Ctrl Pts',(-13.2690454743875,15.5,5.56512499999992));
#25186=CARTESIAN_POINT('Ctrl Pts',(-13.8267841057906,16.4660316469341,5.52345833333325));
#25187=CARTESIAN_POINT('Ctrl Pts',(-14.3845227371938,17.4320632938683,5.48179166666659));
#25188=CARTESIAN_POINT('Ctrl Pts',(-15.5,17.4320632938683,5.44012499999992));
#25189=CARTESIAN_POINT('Ctrl Pts',(-16.6154772628062,17.4320632938683,5.39845833333325));
#25190=CARTESIAN_POINT('Ctrl Pts',(-17.1732158942094,16.4660316469341,5.35679166666658));
#25191=CARTESIAN_POINT('Ctrl Pts',(-17.7309545256125,15.5,5.31512499999992));
#25192=CARTESIAN_POINT('Ctrl Pts',(-17.1732158942094,14.5339683530659,5.27345833333325));
#25193=CARTESIAN_POINT('Ctrl Pts',(-16.6154772628062,13.5679367061317,5.23179166666658));
#25194=CARTESIAN_POINT('Ctrl Pts',(-15.5,13.5679367061317,5.19012499999992));
#25195=CARTESIAN_POINT('Ctrl Pts',(-14.3845227371938,13.5679367061317,5.14845833333325));
#25196=CARTESIAN_POINT('Ctrl Pts',(-13.8267841057906,14.5339683530659,5.10679166666658));
#25197=CARTESIAN_POINT('Ctrl Pts',(-13.2690454743875,15.5,5.06512499999991));
#25198=CARTESIAN_POINT('Ctrl Pts',(-13.8267841057906,16.4660316469341,5.02345833333325));
#25199=CARTESIAN_POINT('Ctrl Pts',(-14.3845227371938,17.4320632938683,4.98179166666658));
#25200=CARTESIAN_POINT('Ctrl Pts',(-15.5,17.4320632938683,4.94012499999991));
#25201=CARTESIAN_POINT('Ctrl Pts',(-16.6154772628062,17.4320632938683,4.89845833333325));
#25202=CARTESIAN_POINT('Ctrl Pts',(-17.1732158942094,16.4660316469341,4.85679166666658));
#25203=CARTESIAN_POINT('Ctrl Pts',(-17.7309545256125,15.5,4.81512499999991));
#25204=CARTESIAN_POINT('Ctrl Pts',(-17.1732158942094,14.5339683530659,4.77345833333324));
#25205=CARTESIAN_POINT('Ctrl Pts',(-16.6154772628062,13.5679367061317,4.73179166666658));
#25206=CARTESIAN_POINT('Ctrl Pts',(-15.5,13.5679367061317,4.69012499999991));
#25207=CARTESIAN_POINT('Ctrl Pts',(-14.3845227371938,13.5679367061317,4.64845833333324));
#25208=CARTESIAN_POINT('Ctrl Pts',(-13.8267841057906,14.5339683530659,4.60679166666657));
#25209=CARTESIAN_POINT('Ctrl Pts',(-13.2690454743875,15.5,4.56512499999991));
#25210=CARTESIAN_POINT('Ctrl Pts',(-13.8267841057906,16.4660316469341,4.52345833333324));
#25211=CARTESIAN_POINT('Ctrl Pts',(-14.3845227371938,17.4320632938683,4.48179166666657));
#25212=CARTESIAN_POINT('Ctrl Pts',(-15.5,17.4320632938683,4.44012499999991));
#25213=CARTESIAN_POINT('Ctrl Pts',(-16.6154772628062,17.4320632938683,4.39845833333324));
#25214=CARTESIAN_POINT('Ctrl Pts',(-17.1732158942094,16.4660316469341,4.35679166666657));
#25215=CARTESIAN_POINT('Ctrl Pts',(-17.7309545256125,15.5,4.31512499999991));
#25216=CARTESIAN_POINT('Ctrl Pts',(-17.1732158942094,14.5339683530659,4.27345833333324));
#25217=CARTESIAN_POINT('Ctrl Pts',(-16.6154772628062,13.5679367061317,4.23179166666657));
#25218=CARTESIAN_POINT('Ctrl Pts',(-15.5,13.5679367061317,4.1901249999999));
#25219=CARTESIAN_POINT('Ctrl Pts',(-14.3845227371938,13.5679367061317,4.14845833333324));
#25220=CARTESIAN_POINT('Ctrl Pts',(-13.8267841057906,14.5339683530659,4.10679166666657));
#25221=CARTESIAN_POINT('Ctrl Pts',(-13.2690454743875,15.5,4.0651249999999));
#25222=CARTESIAN_POINT('Ctrl Pts',(-13.8267841057906,16.4660316469341,4.02345833333323));
#25223=CARTESIAN_POINT('Ctrl Pts',(-14.3845227371938,17.4320632938683,3.98179166666657));
#25224=CARTESIAN_POINT('Ctrl Pts',(-15.5,17.4320632938683,3.9401249999999));
#25225=CARTESIAN_POINT('Ctrl Pts',(-16.6154772628062,17.4320632938683,3.89845833333323));
#25226=CARTESIAN_POINT('Ctrl Pts',(-17.1732158942094,16.4660316469341,3.85679166666657));
#25227=CARTESIAN_POINT('Ctrl Pts',(-17.7309545256125,15.5,3.8151249999999));
#25228=CARTESIAN_POINT('Ctrl Pts',(-17.1732158942094,14.5339683530659,3.77345833333323));
#25229=CARTESIAN_POINT('Ctrl Pts',(-16.6154772628062,13.5679367061317,3.73179166666656));
#25230=CARTESIAN_POINT('Ctrl Pts',(-15.5,13.5679367061317,3.6901249999999));
#25231=CARTESIAN_POINT('Ctrl Pts',(-14.3845227371938,13.5679367061317,3.64845833333323));
#25232=CARTESIAN_POINT('Ctrl Pts',(-13.8267841057906,14.5339683530659,3.60679166666656));
#25233=CARTESIAN_POINT('Ctrl Pts',(-13.2690454743875,15.5,3.5651249999999));
#25234=CARTESIAN_POINT('Ctrl Pts',(-13.8267841057906,16.4660316469341,3.52345833333323));
#25235=CARTESIAN_POINT('Ctrl Pts',(-14.3845227371938,17.4320632938683,3.48179166666656));
#25236=CARTESIAN_POINT('Ctrl Pts',(-15.5,17.4320632938683,3.44012499999989));
#25237=CARTESIAN_POINT('Ctrl Pts',(-16.6154772628062,17.4320632938683,3.39845833333323));
#25238=CARTESIAN_POINT('Ctrl Pts',(-17.1732158942094,16.4660316469341,3.35679166666656));
#25239=CARTESIAN_POINT('Ctrl Pts',(-17.7309545256125,15.5,3.31512499999989));
#25240=CARTESIAN_POINT('Ctrl Pts',(-17.1732158942094,14.5339683530659,3.27345833333322));
#25241=CARTESIAN_POINT('Ctrl Pts',(-16.6154772628062,13.5679367061317,3.23179166666656));
#25242=CARTESIAN_POINT('Ctrl Pts',(-15.5,13.5679367061317,3.19012499999989));
#25243=CARTESIAN_POINT('Ctrl Pts',(-14.3845227371938,13.5679367061317,3.14845833333322));
#25244=CARTESIAN_POINT('Ctrl Pts',(-13.8267841057906,14.5339683530659,3.10679166666655));
#25245=CARTESIAN_POINT('Ctrl Pts',(-13.2690454743875,15.5,3.06512499999989));
#25246=CARTESIAN_POINT('Ctrl Pts',(-13.8267841057906,16.4660316469341,3.02345833333322));
#25247=CARTESIAN_POINT('Ctrl Pts',(-14.3845227371938,17.4320632938683,2.98179166666655));
#25248=CARTESIAN_POINT('Ctrl Pts',(-15.5,17.4320632938683,2.94012499999989));
#25249=CARTESIAN_POINT('Ctrl Pts',(-16.6154772628062,17.4320632938683,2.89845833333322));
#25250=CARTESIAN_POINT('Ctrl Pts',(-17.1732158942094,16.4660316469341,2.85679166666655));
#25251=CARTESIAN_POINT('Ctrl Pts',(-17.7309545256125,15.5,2.81512499999988));
#25252=CARTESIAN_POINT('Ctrl Pts',(-17.1732158942094,14.5339683530659,2.77345833333322));
#25253=CARTESIAN_POINT('Ctrl Pts',(-16.6154772628062,13.5679367061317,2.73179166666655));
#25254=CARTESIAN_POINT('Ctrl Pts',(-15.5,13.5679367061317,2.69012499999988));
#25255=CARTESIAN_POINT('Ctrl Pts',(-14.3845227371938,13.5679367061317,2.64845833333321));
#25256=CARTESIAN_POINT('Ctrl Pts',(-13.8267841057906,14.5339683530659,2.60679166666655));
#25257=CARTESIAN_POINT('Ctrl Pts',(-13.2690454743875,15.5,2.56512499999988));
#25258=CARTESIAN_POINT('Ctrl Pts',(-13.8267841057906,16.4660316469341,2.52345833333321));
#25259=CARTESIAN_POINT('Ctrl Pts',(-14.3845227371938,17.4320632938683,2.48179166666655));
#25260=CARTESIAN_POINT('Ctrl Pts',(-15.5,17.4320632938683,2.44012499999988));
#25261=CARTESIAN_POINT('Ctrl Pts',(-16.6154772628062,17.4320632938683,2.39845833333321));
#25262=CARTESIAN_POINT('Ctrl Pts',(-17.1732158942094,16.4660316469341,2.35679166666655));
#25263=CARTESIAN_POINT('Ctrl Pts',(-17.7309545256125,15.5,2.31512499999988));
#25264=CARTESIAN_POINT('Ctrl Pts',(-17.1732158942094,14.5339683530659,2.27345833333321));
#25265=CARTESIAN_POINT('Ctrl Pts',(-16.6154772628062,13.5679367061317,2.23179166666654));
#25266=CARTESIAN_POINT('Ctrl Pts',(-15.5,13.5679367061317,2.19012499999988));
#25267=CARTESIAN_POINT('Ctrl Pts',(-14.3845227371938,13.5679367061317,2.14845833333321));
#25268=CARTESIAN_POINT('Ctrl Pts',(-13.8267841057906,14.5339683530659,2.10679166666654));
#25269=CARTESIAN_POINT('Ctrl Pts',(-13.2690454743875,15.5,2.06512499999987));
#25270=CARTESIAN_POINT('Ctrl Pts',(-13.8267841057906,16.4660316469341,2.02345833333321));
#25271=CARTESIAN_POINT('Ctrl Pts',(-14.3845227371938,17.4320632938683,1.98179166666654));
#25272=CARTESIAN_POINT('Ctrl Pts',(-15.5,17.4320632938683,1.94012499999987));
#25273=CARTESIAN_POINT('Ctrl Pts',(-16.6154772628062,17.4320632938683,1.89845833333321));
#25274=CARTESIAN_POINT('Ctrl Pts',(-17.1732158942094,16.4660316469341,1.85679166666654));
#25275=CARTESIAN_POINT('Ctrl Pts',(-17.7309545256125,15.5,1.81512499999987));
#25276=CARTESIAN_POINT('Ctrl Pts',(-17.1732158942094,14.5339683530659,1.7734583333332));
#25277=CARTESIAN_POINT('Ctrl Pts',(-16.6154772628062,13.5679367061317,1.73179166666654));
#25278=CARTESIAN_POINT('Ctrl Pts',(-15.5,13.5679367061317,1.69012499999987));
#25279=CARTESIAN_POINT('Ctrl Pts',(-14.3845227371938,13.5679367061317,1.6484583333332));
#25280=CARTESIAN_POINT('Ctrl Pts',(-13.8267841057906,14.5339683530659,1.60679166666653));
#25281=CARTESIAN_POINT('Ctrl Pts',(-13.2690454743875,15.5,1.56512499999987));
#25282=CARTESIAN_POINT('Ctrl Pts',(-13.8267841057906,16.4660316469341,1.5234583333332));
#25283=CARTESIAN_POINT('Ctrl Pts',(-14.3845227371938,17.4320632938683,1.48179166666653));
#25284=CARTESIAN_POINT('Ctrl Pts',(-15.5,17.4320632938683,1.44012499999987));
#25285=CARTESIAN_POINT('Ctrl Pts',(-16.6154772628062,17.4320632938683,1.3984583333332));
#25286=CARTESIAN_POINT('Ctrl Pts',(-17.1732158942094,16.4660316469341,1.35679166666653));
#25287=CARTESIAN_POINT('Ctrl Pts',(-17.7309545256125,15.5,1.31512499999987));
#25288=CARTESIAN_POINT('Ctrl Pts',(-17.1732158942094,14.5339683530659,1.2734583333332));
#25289=CARTESIAN_POINT('Ctrl Pts',(-16.6154772628062,13.5679367061317,1.23179166666653));
#25290=CARTESIAN_POINT('Ctrl Pts',(-15.5,13.5679367061317,1.19012499999986));
#25291=CARTESIAN_POINT('Ctrl Pts',(-14.3845227371938,13.5679367061317,1.1484583333332));
#25292=CARTESIAN_POINT('Ctrl Pts',(-13.8267841057906,14.5339683530659,1.10679166666653));
#25293=CARTESIAN_POINT('Ctrl Pts',(-13.2690454743875,15.5,1.06512499999986));
#25294=CARTESIAN_POINT('Ctrl Pts',(-13.8267841057906,16.4660316469341,1.02345833333319));
#25295=CARTESIAN_POINT('Ctrl Pts',(-14.3845227371938,17.4320632938683,0.981791666666527));
#25296=CARTESIAN_POINT('Ctrl Pts',(-15.5,17.4320632938683,0.94012499999986));
#25297=CARTESIAN_POINT('Ctrl Pts',(-16.6154772628062,17.4320632938683,0.898458333333192));
#25298=CARTESIAN_POINT('Ctrl Pts',(-17.1732158942094,16.4660316469341,0.856791666666525));
#25299=CARTESIAN_POINT('Ctrl Pts',(-17.7309545256125,15.5,0.815124999999858));
#25300=CARTESIAN_POINT('Ctrl Pts',(-17.1732158942094,14.5339683530659,0.77345833333319));
#25301=CARTESIAN_POINT('Ctrl Pts',(-16.6154772628062,13.5679367061317,0.731791666666523));
#25302=CARTESIAN_POINT('Ctrl Pts',(-15.5,13.5679367061317,0.690124999999856));
#25303=CARTESIAN_POINT('Ctrl Pts',(-14.3845227371938,13.5679367061317,0.648458333333188));
#25304=CARTESIAN_POINT('Ctrl Pts',(-13.8267841057906,14.5339683530659,0.606791666666521));
#25305=CARTESIAN_POINT('Ctrl Pts',(-13.2690454743875,15.5,0.565124999999854));
#25306=CARTESIAN_POINT('Ctrl Pts',(-13.8267841057906,16.4660316469341,0.523458333333187));
#25307=CARTESIAN_POINT('Ctrl Pts',(-14.3845227371938,17.4320632938683,0.481791666666519));
#25308=CARTESIAN_POINT('Ctrl Pts',(-15.5,17.4320632938683,0.440124999999852));
#25309=CARTESIAN_POINT('Ctrl Pts',(-16.6154772628062,17.4320632938683,0.398458333333185));
#25310=CARTESIAN_POINT('Ctrl Pts',(-17.1732158942094,16.4660316469341,0.356791666666518));
#25311=CARTESIAN_POINT('Ctrl Pts',(-17.7309545256125,15.5,0.31512499999985));
#25312=CARTESIAN_POINT('Ctrl Pts',(-17.1732158942094,14.5339683530659,0.273458333333183));
#25313=CARTESIAN_POINT('Ctrl Pts',(-16.6154772628062,13.5679367061317,0.231791666666516));
#25314=CARTESIAN_POINT('Ctrl Pts',(-15.5,13.5679367061317,0.190124999999848));
#25315=CARTESIAN_POINT('Ctrl Pts',(-14.3845227371938,13.5679367061317,0.148458333333183));
#25316=CARTESIAN_POINT('Ctrl Pts',(-13.8267841057906,14.5339683530659,0.106791666666516));
#25317=CARTESIAN_POINT('Ctrl Pts',(-13.2690454743875,15.5,0.0651249999998483));
#25318=CARTESIAN_POINT('Ctrl Pts',(-13.8267841057906,16.4660316469341,0.023458333333181));
#25319=CARTESIAN_POINT('Ctrl Pts',(-14.3845227371938,17.4320632938683,-0.0182083333334863));
#25320=CARTESIAN_POINT('Ctrl Pts',(-15.5,17.4320632938683,-0.0598750000001536));
#25321=CARTESIAN_POINT('Ctrl Pts',(-16.6154772628062,17.4320632938683,-0.101541666666821));
#25322=CARTESIAN_POINT('Ctrl Pts',(-17.1732158942094,16.4660316469341,-0.143208333333488));
#25323=CARTESIAN_POINT('Ctrl Pts',(-17.7309545256125,15.5,-0.184875000000155));
#25324=CARTESIAN_POINT('Ctrl Pts',(-17.1732158942094,14.5339683530659,-0.226541666666823));
#25325=CARTESIAN_POINT('Ctrl Pts',(-16.6154772628062,13.5679367061317,-0.26820833333349));
#25326=CARTESIAN_POINT('Ctrl Pts',(-15.5,13.5679367061317,-0.309875000000157));
#25327=CARTESIAN_POINT('Ctrl Pts',(-14.3845227371938,13.5679367061317,-0.351541666666825));
#25328=CARTESIAN_POINT('Ctrl Pts',(-13.8267841057906,14.5339683530659,-0.393208333333492));
#25329=CARTESIAN_POINT('Ctrl Pts',(-13.2690454743875,15.5,-0.434875000000159));
#25330=CARTESIAN_POINT('Ctrl Pts',(-13.8267841057906,16.4660316469341,-0.476541666666826));
#25331=CARTESIAN_POINT('Ctrl Pts',(-14.3845227371938,17.4320632938683,-0.518208333333494));
#25332=CARTESIAN_POINT('Ctrl Pts',(-15.5,17.4320632938683,-0.559875000000161));
#25333=CARTESIAN_POINT('Ctrl Pts',(-16.6154772628062,17.4320632938683,-0.601541666666828));
#25334=CARTESIAN_POINT('Ctrl Pts',(-17.1732158942094,16.4660316469341,-0.643208333333495));
#25335=CARTESIAN_POINT('Ctrl Pts',(-17.7309545256125,15.5,-0.684875000000163));
#25336=CARTESIAN_POINT('Ctrl Pts',(-17.1732158942094,14.5339683530659,-0.72654166666683));
#25337=CARTESIAN_POINT('Ctrl Pts',(-16.6154772628062,13.5679367061317,-0.768208333333497));
#25338=CARTESIAN_POINT('Ctrl Pts',(-15.5,13.5679367061317,-0.809875000000165));
#25339=CARTESIAN_POINT('Ctrl Pts',(-14.3845227371938,13.5679367061317,-0.851541666666832));
#25340=CARTESIAN_POINT('Ctrl Pts',(-13.8267841057906,14.5339683530659,-0.893208333333499));
#25341=CARTESIAN_POINT('Ctrl Pts',(-13.2690454743875,15.5,-0.934875000000167));
#25342=CARTESIAN_POINT('Ctrl Pts',(-13.8267841057906,16.4660316469341,-0.976541666666834));
#25343=CARTESIAN_POINT('Ctrl Pts',(-14.3845227371938,17.4320632938683,-1.0182083333335));
#25344=CARTESIAN_POINT('Ctrl Pts',(-15.5,17.4320632938683,-1.05987500000017));
#25345=CARTESIAN_POINT('Ctrl Pts',(-16.6154772628062,17.4320632938683,-1.10154166666683));
#25346=CARTESIAN_POINT('Ctrl Pts',(-17.1732158942094,16.4660316469341,-1.1432083333335));
#25347=CARTESIAN_POINT('Ctrl Pts',(-17.7309545256125,15.5,-1.18487500000017));
#25348=CARTESIAN_POINT('Ctrl Pts',(-17.1732158942094,14.5339683530659,-1.22654166666684));
#25349=CARTESIAN_POINT('Ctrl Pts',(-16.6154772628062,13.5679367061317,-1.2682083333335));
#25350=CARTESIAN_POINT('Ctrl Pts',(-15.5,13.5679367061317,-1.30987500000017));
#25351=CARTESIAN_POINT('Ctrl Pts',(-14.3845227371938,13.5679367061317,-1.35154166666684));
#25352=CARTESIAN_POINT('Ctrl Pts',(-13.8267841057906,14.5339683530659,-1.3932083333335));
#25353=CARTESIAN_POINT('Ctrl Pts',(-13.2690454743875,15.5,-1.43487500000017));
#25354=CARTESIAN_POINT('Ctrl Pts',(-13.8267841057906,16.4660316469341,-1.47654166666684));
#25355=CARTESIAN_POINT('Ctrl Pts',(-14.3845227371938,17.4320632938683,-1.51820833333351));
#25356=CARTESIAN_POINT('Ctrl Pts',(-15.5,17.4320632938683,-1.55987500000017));
#25357=CARTESIAN_POINT('Ctrl Pts',(-16.6154772628062,17.4320632938683,-1.60154166666684));
#25358=CARTESIAN_POINT('Ctrl Pts',(-17.1732158942094,16.4660316469341,-1.64320833333351));
#25359=CARTESIAN_POINT('Ctrl Pts',(-17.7309545256125,15.5,-1.68487500000018));
#25360=CARTESIAN_POINT('Ctrl Pts',(-17.1732158942094,14.5339683530659,-1.72654166666684));
#25361=CARTESIAN_POINT('Ctrl Pts',(-16.9678753992805,14.1783081829978,-1.74188192368624));
#25362=CARTESIAN_POINT('Ctrl Pts',(-16.6356255246375,13.9369186715641,-1.75949830599533));
#25363=CARTESIAN_POINT('Ctrl Pts',(-15.5,17.0802404735808,11.237));
#25364=CARTESIAN_POINT('Ctrl Pts',(-16.4123522628062,17.0802404735808,11.1953333333333));
#25365=CARTESIAN_POINT('Ctrl Pts',(-16.8685283942094,16.2901202367904,11.1536666666667));
#25366=CARTESIAN_POINT('Ctrl Pts',(-17.3247045256125,15.5,11.112));
#25367=CARTESIAN_POINT('Ctrl Pts',(-16.8685283942094,14.7098797632096,11.0703333333333));
#25368=CARTESIAN_POINT('Ctrl Pts',(-16.4123522628062,13.9197595264192,11.0286666666667));
#25369=CARTESIAN_POINT('Ctrl Pts',(-15.5,13.9197595264192,10.987));
#25370=CARTESIAN_POINT('Ctrl Pts',(-14.5876477371938,13.9197595264192,10.9453333333333));
#25371=CARTESIAN_POINT('Ctrl Pts',(-14.1314716057906,14.7098797632096,10.9036666666667));
#25372=CARTESIAN_POINT('Ctrl Pts',(-13.6752954743875,15.5,10.862));
#25373=CARTESIAN_POINT('Ctrl Pts',(-14.1314716057906,16.2901202367904,10.8203333333333));
#25374=CARTESIAN_POINT('Ctrl Pts',(-14.5876477371938,17.0802404735808,10.7786666666667));
#25375=CARTESIAN_POINT('Ctrl Pts',(-15.5,17.0802404735808,10.737));
#25376=CARTESIAN_POINT('Ctrl Pts',(-16.4123522628062,17.0802404735808,10.6953333333333));
#25377=CARTESIAN_POINT('Ctrl Pts',(-16.8685283942094,16.2901202367904,10.6536666666667));
#25378=CARTESIAN_POINT('Ctrl Pts',(-17.3247045256125,15.5,10.612));
#25379=CARTESIAN_POINT('Ctrl Pts',(-16.8685283942094,14.7098797632096,10.5703333333333));
#25380=CARTESIAN_POINT('Ctrl Pts',(-16.4123522628062,13.9197595264192,10.5286666666667));
#25381=CARTESIAN_POINT('Ctrl Pts',(-15.5,13.9197595264192,10.487));
#25382=CARTESIAN_POINT('Ctrl Pts',(-14.5876477371938,13.9197595264192,10.4453333333333));
#25383=CARTESIAN_POINT('Ctrl Pts',(-14.1314716057906,14.7098797632096,10.4036666666667));
#25384=CARTESIAN_POINT('Ctrl Pts',(-13.6752954743875,15.5,10.362));
#25385=CARTESIAN_POINT('Ctrl Pts',(-14.1314716057906,16.2901202367904,10.3203333333333));
#25386=CARTESIAN_POINT('Ctrl Pts',(-14.5876477371938,17.0802404735808,10.2786666666667));
#25387=CARTESIAN_POINT('Ctrl Pts',(-15.5,17.0802404735808,10.237));
#25388=CARTESIAN_POINT('Ctrl Pts',(-16.4123522628062,17.0802404735808,10.1953333333333));
#25389=CARTESIAN_POINT('Ctrl Pts',(-16.8685283942094,16.2901202367904,10.1536666666667));
#25390=CARTESIAN_POINT('Ctrl Pts',(-17.3247045256125,15.5,10.112));
#25391=CARTESIAN_POINT('Ctrl Pts',(-16.8685283942094,14.7098797632096,10.0703333333333));
#25392=CARTESIAN_POINT('Ctrl Pts',(-16.4123522628062,13.9197595264192,10.0286666666667));
#25393=CARTESIAN_POINT('Ctrl Pts',(-15.5,13.9197595264192,9.98699999999998));
#25394=CARTESIAN_POINT('Ctrl Pts',(-14.5876477371938,13.9197595264192,9.94533333333332));
#25395=CARTESIAN_POINT('Ctrl Pts',(-14.1314716057906,14.7098797632096,9.90366666666665));
#25396=CARTESIAN_POINT('Ctrl Pts',(-13.6752954743875,15.5,9.86199999999998));
#25397=CARTESIAN_POINT('Ctrl Pts',(-14.1314716057906,16.2901202367904,9.82033333333331));
#25398=CARTESIAN_POINT('Ctrl Pts',(-14.5876477371938,17.0802404735808,9.77866666666665));
#25399=CARTESIAN_POINT('Ctrl Pts',(-15.5,17.0802404735808,9.73699999999998));
#25400=CARTESIAN_POINT('Ctrl Pts',(-16.4123522628062,17.0802404735808,9.69533333333331));
#25401=CARTESIAN_POINT('Ctrl Pts',(-16.8685283942094,16.2901202367904,9.65366666666664));
#25402=CARTESIAN_POINT('Ctrl Pts',(-17.3247045256125,15.5,9.61199999999998));
#25403=CARTESIAN_POINT('Ctrl Pts',(-16.8685283942094,14.7098797632096,9.57033333333331));
#25404=CARTESIAN_POINT('Ctrl Pts',(-16.4123522628062,13.9197595264192,9.52866666666664));
#25405=CARTESIAN_POINT('Ctrl Pts',(-15.5,13.9197595264192,9.48699999999998));
#25406=CARTESIAN_POINT('Ctrl Pts',(-14.5876477371938,13.9197595264192,9.44533333333331));
#25407=CARTESIAN_POINT('Ctrl Pts',(-14.1314716057906,14.7098797632096,9.40366666666664));
#25408=CARTESIAN_POINT('Ctrl Pts',(-13.6752954743875,15.5,9.36199999999997));
#25409=CARTESIAN_POINT('Ctrl Pts',(-14.1314716057906,16.2901202367904,9.32033333333331));
#25410=CARTESIAN_POINT('Ctrl Pts',(-14.5876477371938,17.0802404735808,9.27866666666664));
#25411=CARTESIAN_POINT('Ctrl Pts',(-15.5,17.0802404735808,9.23699999999997));
#25412=CARTESIAN_POINT('Ctrl Pts',(-16.4123522628062,17.0802404735808,9.19533333333331));
#25413=CARTESIAN_POINT('Ctrl Pts',(-16.8685283942094,16.2901202367904,9.15366666666664));
#25414=CARTESIAN_POINT('Ctrl Pts',(-17.3247045256125,15.5,9.11199999999997));
#25415=CARTESIAN_POINT('Ctrl Pts',(-16.8685283942094,14.7098797632096,9.0703333333333));
#25416=CARTESIAN_POINT('Ctrl Pts',(-16.4123522628062,13.9197595264192,9.02866666666664));
#25417=CARTESIAN_POINT('Ctrl Pts',(-15.5,13.9197595264192,8.98699999999997));
#25418=CARTESIAN_POINT('Ctrl Pts',(-14.5876477371938,13.9197595264192,8.9453333333333));
#25419=CARTESIAN_POINT('Ctrl Pts',(-14.1314716057906,14.7098797632096,8.90366666666664));
#25420=CARTESIAN_POINT('Ctrl Pts',(-13.6752954743875,15.5,8.86199999999997));
#25421=CARTESIAN_POINT('Ctrl Pts',(-14.1314716057906,16.2901202367904,8.8203333333333));
#25422=CARTESIAN_POINT('Ctrl Pts',(-14.5876477371938,17.0802404735808,8.77866666666663));
#25423=CARTESIAN_POINT('Ctrl Pts',(-15.5,17.0802404735808,8.73699999999997));
#25424=CARTESIAN_POINT('Ctrl Pts',(-16.4123522628062,17.0802404735808,8.6953333333333));
#25425=CARTESIAN_POINT('Ctrl Pts',(-16.8685283942094,16.2901202367904,8.65366666666663));
#25426=CARTESIAN_POINT('Ctrl Pts',(-17.3247045256125,15.5,8.61199999999996));
#25427=CARTESIAN_POINT('Ctrl Pts',(-16.8685283942094,14.7098797632096,8.57033333333329));
#25428=CARTESIAN_POINT('Ctrl Pts',(-16.4123522628062,13.9197595264192,8.52866666666663));
#25429=CARTESIAN_POINT('Ctrl Pts',(-15.5,13.9197595264192,8.48699999999996));
#25430=CARTESIAN_POINT('Ctrl Pts',(-14.5876477371938,13.9197595264192,8.44533333333329));
#25431=CARTESIAN_POINT('Ctrl Pts',(-14.1314716057906,14.7098797632096,8.40366666666663));
#25432=CARTESIAN_POINT('Ctrl Pts',(-13.6752954743875,15.5,8.36199999999996));
#25433=CARTESIAN_POINT('Ctrl Pts',(-14.1314716057906,16.2901202367904,8.32033333333329));
#25434=CARTESIAN_POINT('Ctrl Pts',(-14.5876477371938,17.0802404735808,8.27866666666663));
#25435=CARTESIAN_POINT('Ctrl Pts',(-15.5,17.0802404735808,8.23699999999996));
#25436=CARTESIAN_POINT('Ctrl Pts',(-16.4123522628062,17.0802404735808,8.19533333333329));
#25437=CARTESIAN_POINT('Ctrl Pts',(-16.8685283942094,16.2901202367904,8.15366666666663));
#25438=CARTESIAN_POINT('Ctrl Pts',(-17.3247045256125,15.5,8.11199999999996));
#25439=CARTESIAN_POINT('Ctrl Pts',(-16.8685283942094,14.7098797632096,8.07033333333329));
#25440=CARTESIAN_POINT('Ctrl Pts',(-16.4123522628062,13.9197595264192,8.02866666666662));
#25441=CARTESIAN_POINT('Ctrl Pts',(-15.5,13.9197595264192,7.98699999999996));
#25442=CARTESIAN_POINT('Ctrl Pts',(-14.5876477371938,13.9197595264192,7.94533333333329));
#25443=CARTESIAN_POINT('Ctrl Pts',(-14.1314716057906,14.7098797632096,7.90366666666662));
#25444=CARTESIAN_POINT('Ctrl Pts',(-13.6752954743875,15.5,7.86199999999995));
#25445=CARTESIAN_POINT('Ctrl Pts',(-14.1314716057906,16.2901202367904,7.82033333333329));
#25446=CARTESIAN_POINT('Ctrl Pts',(-14.5876477371938,17.0802404735808,7.77866666666662));
#25447=CARTESIAN_POINT('Ctrl Pts',(-15.5,17.0802404735808,7.73699999999995));
#25448=CARTESIAN_POINT('Ctrl Pts',(-16.4123522628062,17.0802404735808,7.69533333333329));
#25449=CARTESIAN_POINT('Ctrl Pts',(-16.8685283942094,16.2901202367904,7.65366666666662));
#25450=CARTESIAN_POINT('Ctrl Pts',(-17.3247045256125,15.5,7.61199999999995));
#25451=CARTESIAN_POINT('Ctrl Pts',(-16.8685283942094,14.7098797632096,7.57033333333328));
#25452=CARTESIAN_POINT('Ctrl Pts',(-16.4123522628062,13.9197595264192,7.52866666666661));
#25453=CARTESIAN_POINT('Ctrl Pts',(-15.5,13.9197595264192,7.48699999999995));
#25454=CARTESIAN_POINT('Ctrl Pts',(-14.5876477371938,13.9197595264192,7.44533333333328));
#25455=CARTESIAN_POINT('Ctrl Pts',(-14.1314716057906,14.7098797632096,7.40366666666661));
#25456=CARTESIAN_POINT('Ctrl Pts',(-13.6752954743875,15.5,7.36199999999995));
#25457=CARTESIAN_POINT('Ctrl Pts',(-14.1314716057906,16.2901202367904,7.32033333333328));
#25458=CARTESIAN_POINT('Ctrl Pts',(-14.5876477371938,17.0802404735808,7.27866666666661));
#25459=CARTESIAN_POINT('Ctrl Pts',(-15.5,17.0802404735808,7.23699999999995));
#25460=CARTESIAN_POINT('Ctrl Pts',(-16.4123522628062,17.0802404735808,7.19533333333328));
#25461=CARTESIAN_POINT('Ctrl Pts',(-16.8685283942094,16.2901202367904,7.15366666666661));
#25462=CARTESIAN_POINT('Ctrl Pts',(-17.3247045256125,15.5,7.11199999999994));
#25463=CARTESIAN_POINT('Ctrl Pts',(-16.8685283942094,14.7098797632096,7.07033333333328));
#25464=CARTESIAN_POINT('Ctrl Pts',(-16.4123522628062,13.9197595264192,7.02866666666661));
#25465=CARTESIAN_POINT('Ctrl Pts',(-15.5,13.9197595264192,6.98699999999994));
#25466=CARTESIAN_POINT('Ctrl Pts',(-14.5876477371938,13.9197595264192,6.94533333333327));
#25467=CARTESIAN_POINT('Ctrl Pts',(-14.1314716057906,14.7098797632096,6.90366666666661));
#25468=CARTESIAN_POINT('Ctrl Pts',(-13.6752954743875,15.5,6.86199999999994));
#25469=CARTESIAN_POINT('Ctrl Pts',(-14.1314716057906,16.2901202367904,6.82033333333327));
#25470=CARTESIAN_POINT('Ctrl Pts',(-14.5876477371938,17.0802404735808,6.77866666666661));
#25471=CARTESIAN_POINT('Ctrl Pts',(-15.5,17.0802404735808,6.73699999999994));
#25472=CARTESIAN_POINT('Ctrl Pts',(-16.4123522628062,17.0802404735808,6.69533333333327));
#25473=CARTESIAN_POINT('Ctrl Pts',(-16.8685283942094,16.2901202367904,6.65366666666661));
#25474=CARTESIAN_POINT('Ctrl Pts',(-17.3247045256125,15.5,6.61199999999994));
#25475=CARTESIAN_POINT('Ctrl Pts',(-16.8685283942094,14.7098797632096,6.57033333333327));
#25476=CARTESIAN_POINT('Ctrl Pts',(-16.4123522628062,13.9197595264192,6.5286666666666));
#25477=CARTESIAN_POINT('Ctrl Pts',(-15.5,13.9197595264192,6.48699999999994));
#25478=CARTESIAN_POINT('Ctrl Pts',(-14.5876477371938,13.9197595264192,6.44533333333327));
#25479=CARTESIAN_POINT('Ctrl Pts',(-14.1314716057906,14.7098797632096,6.4036666666666));
#25480=CARTESIAN_POINT('Ctrl Pts',(-13.6752954743875,15.5,6.36199999999993));
#25481=CARTESIAN_POINT('Ctrl Pts',(-14.1314716057906,16.2901202367904,6.32033333333327));
#25482=CARTESIAN_POINT('Ctrl Pts',(-14.5876477371938,17.0802404735808,6.2786666666666));
#25483=CARTESIAN_POINT('Ctrl Pts',(-15.5,17.0802404735808,6.23699999999993));
#25484=CARTESIAN_POINT('Ctrl Pts',(-16.4123522628062,17.0802404735808,6.19533333333326));
#25485=CARTESIAN_POINT('Ctrl Pts',(-16.8685283942094,16.2901202367904,6.1536666666666));
#25486=CARTESIAN_POINT('Ctrl Pts',(-17.3247045256125,15.5,6.11199999999993));
#25487=CARTESIAN_POINT('Ctrl Pts',(-16.8685283942094,14.7098797632096,6.07033333333326));
#25488=CARTESIAN_POINT('Ctrl Pts',(-16.4123522628062,13.9197595264192,6.0286666666666));
#25489=CARTESIAN_POINT('Ctrl Pts',(-15.5,13.9197595264192,5.98699999999993));
#25490=CARTESIAN_POINT('Ctrl Pts',(-14.5876477371938,13.9197595264192,5.94533333333326));
#25491=CARTESIAN_POINT('Ctrl Pts',(-14.1314716057906,14.7098797632096,5.9036666666666));
#25492=CARTESIAN_POINT('Ctrl Pts',(-13.6752954743875,15.5,5.86199999999993));
#25493=CARTESIAN_POINT('Ctrl Pts',(-14.1314716057906,16.2901202367904,5.82033333333326));
#25494=CARTESIAN_POINT('Ctrl Pts',(-14.5876477371938,17.0802404735808,5.77866666666659));
#25495=CARTESIAN_POINT('Ctrl Pts',(-15.5,17.0802404735808,5.73699999999993));
#25496=CARTESIAN_POINT('Ctrl Pts',(-16.4123522628062,17.0802404735808,5.69533333333326));
#25497=CARTESIAN_POINT('Ctrl Pts',(-16.8685283942094,16.2901202367904,5.65366666666659));
#25498=CARTESIAN_POINT('Ctrl Pts',(-17.3247045256125,15.5,5.61199999999992));
#25499=CARTESIAN_POINT('Ctrl Pts',(-16.8685283942094,14.7098797632096,5.57033333333326));
#25500=CARTESIAN_POINT('Ctrl Pts',(-16.4123522628062,13.9197595264192,5.52866666666659));
#25501=CARTESIAN_POINT('Ctrl Pts',(-15.5,13.9197595264192,5.48699999999992));
#25502=CARTESIAN_POINT('Ctrl Pts',(-14.5876477371938,13.9197595264192,5.44533333333326));
#25503=CARTESIAN_POINT('Ctrl Pts',(-14.1314716057906,14.7098797632096,5.40366666666659));
#25504=CARTESIAN_POINT('Ctrl Pts',(-13.6752954743875,15.5,5.36199999999992));
#25505=CARTESIAN_POINT('Ctrl Pts',(-14.1314716057906,16.2901202367904,5.32033333333325));
#25506=CARTESIAN_POINT('Ctrl Pts',(-14.5876477371938,17.0802404735808,5.27866666666659));
#25507=CARTESIAN_POINT('Ctrl Pts',(-15.5,17.0802404735808,5.23699999999992));
#25508=CARTESIAN_POINT('Ctrl Pts',(-16.4123522628062,17.0802404735808,5.19533333333325));
#25509=CARTESIAN_POINT('Ctrl Pts',(-16.8685283942094,16.2901202367904,5.15366666666658));
#25510=CARTESIAN_POINT('Ctrl Pts',(-17.3247045256125,15.5,5.11199999999992));
#25511=CARTESIAN_POINT('Ctrl Pts',(-16.8685283942094,14.7098797632096,5.07033333333325));
#25512=CARTESIAN_POINT('Ctrl Pts',(-16.4123522628062,13.9197595264192,5.02866666666658));
#25513=CARTESIAN_POINT('Ctrl Pts',(-15.5,13.9197595264192,4.98699999999992));
#25514=CARTESIAN_POINT('Ctrl Pts',(-14.5876477371938,13.9197595264192,4.94533333333325));
#25515=CARTESIAN_POINT('Ctrl Pts',(-14.1314716057906,14.7098797632096,4.90366666666658));
#25516=CARTESIAN_POINT('Ctrl Pts',(-13.6752954743875,15.5,4.86199999999991));
#25517=CARTESIAN_POINT('Ctrl Pts',(-14.1314716057906,16.2901202367904,4.82033333333325));
#25518=CARTESIAN_POINT('Ctrl Pts',(-14.5876477371938,17.0802404735808,4.77866666666658));
#25519=CARTESIAN_POINT('Ctrl Pts',(-15.5,17.0802404735808,4.73699999999991));
#25520=CARTESIAN_POINT('Ctrl Pts',(-16.4123522628062,17.0802404735808,4.69533333333325));
#25521=CARTESIAN_POINT('Ctrl Pts',(-16.8685283942094,16.2901202367904,4.65366666666658));
#25522=CARTESIAN_POINT('Ctrl Pts',(-17.3247045256125,15.5,4.61199999999991));
#25523=CARTESIAN_POINT('Ctrl Pts',(-16.8685283942094,14.7098797632096,4.57033333333324));
#25524=CARTESIAN_POINT('Ctrl Pts',(-16.4123522628062,13.9197595264192,4.52866666666658));
#25525=CARTESIAN_POINT('Ctrl Pts',(-15.5,13.9197595264192,4.48699999999991));
#25526=CARTESIAN_POINT('Ctrl Pts',(-14.5876477371938,13.9197595264192,4.44533333333324));
#25527=CARTESIAN_POINT('Ctrl Pts',(-14.1314716057906,14.7098797632096,4.40366666666658));
#25528=CARTESIAN_POINT('Ctrl Pts',(-13.6752954743875,15.5,4.36199999999991));
#25529=CARTESIAN_POINT('Ctrl Pts',(-14.1314716057906,16.2901202367904,4.32033333333324));
#25530=CARTESIAN_POINT('Ctrl Pts',(-14.5876477371938,17.0802404735808,4.27866666666657));
#25531=CARTESIAN_POINT('Ctrl Pts',(-15.5,17.0802404735808,4.23699999999991));
#25532=CARTESIAN_POINT('Ctrl Pts',(-16.4123522628062,17.0802404735808,4.19533333333324));
#25533=CARTESIAN_POINT('Ctrl Pts',(-16.8685283942094,16.2901202367904,4.15366666666657));
#25534=CARTESIAN_POINT('Ctrl Pts',(-17.3247045256125,15.5,4.1119999999999));
#25535=CARTESIAN_POINT('Ctrl Pts',(-16.8685283942094,14.7098797632096,4.07033333333324));
#25536=CARTESIAN_POINT('Ctrl Pts',(-16.4123522628062,13.9197595264192,4.02866666666657));
#25537=CARTESIAN_POINT('Ctrl Pts',(-15.5,13.9197595264192,3.9869999999999));
#25538=CARTESIAN_POINT('Ctrl Pts',(-14.5876477371938,13.9197595264192,3.94533333333323));
#25539=CARTESIAN_POINT('Ctrl Pts',(-14.1314716057906,14.7098797632096,3.90366666666657));
#25540=CARTESIAN_POINT('Ctrl Pts',(-13.6752954743875,15.5,3.8619999999999));
#25541=CARTESIAN_POINT('Ctrl Pts',(-14.1314716057906,16.2901202367904,3.82033333333323));
#25542=CARTESIAN_POINT('Ctrl Pts',(-14.5876477371938,17.0802404735808,3.77866666666657));
#25543=CARTESIAN_POINT('Ctrl Pts',(-15.5,17.0802404735808,3.7369999999999));
#25544=CARTESIAN_POINT('Ctrl Pts',(-16.4123522628062,17.0802404735808,3.69533333333323));
#25545=CARTESIAN_POINT('Ctrl Pts',(-16.8685283942094,16.2901202367904,3.65366666666656));
#25546=CARTESIAN_POINT('Ctrl Pts',(-17.3247045256125,15.5,3.6119999999999));
#25547=CARTESIAN_POINT('Ctrl Pts',(-16.8685283942094,14.7098797632096,3.57033333333323));
#25548=CARTESIAN_POINT('Ctrl Pts',(-16.4123522628062,13.9197595264192,3.52866666666656));
#25549=CARTESIAN_POINT('Ctrl Pts',(-15.5,13.9197595264192,3.4869999999999));
#25550=CARTESIAN_POINT('Ctrl Pts',(-14.5876477371938,13.9197595264192,3.44533333333323));
#25551=CARTESIAN_POINT('Ctrl Pts',(-14.1314716057906,14.7098797632096,3.40366666666656));
#25552=CARTESIAN_POINT('Ctrl Pts',(-13.6752954743875,15.5,3.36199999999989));
#25553=CARTESIAN_POINT('Ctrl Pts',(-14.1314716057906,16.2901202367904,3.32033333333323));
#25554=CARTESIAN_POINT('Ctrl Pts',(-14.5876477371938,17.0802404735808,3.27866666666656));
#25555=CARTESIAN_POINT('Ctrl Pts',(-15.5,17.0802404735808,3.23699999999989));
#25556=CARTESIAN_POINT('Ctrl Pts',(-16.4123522628062,17.0802404735808,3.19533333333323));
#25557=CARTESIAN_POINT('Ctrl Pts',(-16.8685283942094,16.2901202367904,3.15366666666656));
#25558=CARTESIAN_POINT('Ctrl Pts',(-17.3247045256125,15.5,3.11199999999989));
#25559=CARTESIAN_POINT('Ctrl Pts',(-16.8685283942094,14.7098797632096,3.07033333333322));
#25560=CARTESIAN_POINT('Ctrl Pts',(-16.4123522628062,13.9197595264192,3.02866666666656));
#25561=CARTESIAN_POINT('Ctrl Pts',(-15.5,13.9197595264192,2.98699999999989));
#25562=CARTESIAN_POINT('Ctrl Pts',(-14.5876477371938,13.9197595264192,2.94533333333322));
#25563=CARTESIAN_POINT('Ctrl Pts',(-14.1314716057906,14.7098797632096,2.90366666666656));
#25564=CARTESIAN_POINT('Ctrl Pts',(-13.6752954743875,15.5,2.86199999999989));
#25565=CARTESIAN_POINT('Ctrl Pts',(-14.1314716057906,16.2901202367904,2.82033333333322));
#25566=CARTESIAN_POINT('Ctrl Pts',(-14.5876477371938,17.0802404735808,2.77866666666655));
#25567=CARTESIAN_POINT('Ctrl Pts',(-15.5,17.0802404735808,2.73699999999989));
#25568=CARTESIAN_POINT('Ctrl Pts',(-16.4123522628062,17.0802404735808,2.69533333333322));
#25569=CARTESIAN_POINT('Ctrl Pts',(-16.8685283942094,16.2901202367904,2.65366666666655));
#25570=CARTESIAN_POINT('Ctrl Pts',(-17.3247045256125,15.5,2.61199999999988));
#25571=CARTESIAN_POINT('Ctrl Pts',(-16.8685283942094,14.7098797632096,2.57033333333322));
#25572=CARTESIAN_POINT('Ctrl Pts',(-16.4123522628062,13.9197595264192,2.52866666666655));
#25573=CARTESIAN_POINT('Ctrl Pts',(-15.5,13.9197595264192,2.48699999999988));
#25574=CARTESIAN_POINT('Ctrl Pts',(-14.5876477371938,13.9197595264192,2.44533333333321));
#25575=CARTESIAN_POINT('Ctrl Pts',(-14.1314716057906,14.7098797632096,2.40366666666655));
#25576=CARTESIAN_POINT('Ctrl Pts',(-13.6752954743875,15.5,2.36199999999988));
#25577=CARTESIAN_POINT('Ctrl Pts',(-14.1314716057906,16.2901202367904,2.32033333333321));
#25578=CARTESIAN_POINT('Ctrl Pts',(-14.5876477371938,17.0802404735808,2.27866666666655));
#25579=CARTESIAN_POINT('Ctrl Pts',(-15.5,17.0802404735808,2.23699999999988));
#25580=CARTESIAN_POINT('Ctrl Pts',(-16.4123522628062,17.0802404735808,2.19533333333321));
#25581=CARTESIAN_POINT('Ctrl Pts',(-16.8685283942094,16.2901202367904,2.15366666666655));
#25582=CARTESIAN_POINT('Ctrl Pts',(-17.3247045256125,15.5,2.11199999999988));
#25583=CARTESIAN_POINT('Ctrl Pts',(-16.8685283942094,14.7098797632096,2.07033333333321));
#25584=CARTESIAN_POINT('Ctrl Pts',(-16.4123522628062,13.9197595264192,2.02866666666654));
#25585=CARTESIAN_POINT('Ctrl Pts',(-15.5,13.9197595264192,1.98699999999988));
#25586=CARTESIAN_POINT('Ctrl Pts',(-14.5876477371938,13.9197595264192,1.94533333333321));
#25587=CARTESIAN_POINT('Ctrl Pts',(-14.1314716057906,14.7098797632096,1.90366666666654));
#25588=CARTESIAN_POINT('Ctrl Pts',(-13.6752954743875,15.5,1.86199999999987));
#25589=CARTESIAN_POINT('Ctrl Pts',(-14.1314716057906,16.2901202367904,1.82033333333321));
#25590=CARTESIAN_POINT('Ctrl Pts',(-14.5876477371938,17.0802404735808,1.77866666666654));
#25591=CARTESIAN_POINT('Ctrl Pts',(-15.5,17.0802404735808,1.73699999999987));
#25592=CARTESIAN_POINT('Ctrl Pts',(-16.4123522628062,17.0802404735808,1.6953333333332));
#25593=CARTESIAN_POINT('Ctrl Pts',(-16.8685283942094,16.2901202367904,1.65366666666654));
#25594=CARTESIAN_POINT('Ctrl Pts',(-17.3247045256125,15.5,1.61199999999987));
#25595=CARTESIAN_POINT('Ctrl Pts',(-16.8685283942094,14.7098797632096,1.5703333333332));
#25596=CARTESIAN_POINT('Ctrl Pts',(-16.4123522628062,13.9197595264192,1.52866666666654));
#25597=CARTESIAN_POINT('Ctrl Pts',(-15.5,13.9197595264192,1.48699999999987));
#25598=CARTESIAN_POINT('Ctrl Pts',(-14.5876477371938,13.9197595264192,1.4453333333332));
#25599=CARTESIAN_POINT('Ctrl Pts',(-14.1314716057906,14.7098797632096,1.40366666666653));
#25600=CARTESIAN_POINT('Ctrl Pts',(-13.6752954743875,15.5,1.36199999999987));
#25601=CARTESIAN_POINT('Ctrl Pts',(-14.1314716057906,16.2901202367904,1.3203333333332));
#25602=CARTESIAN_POINT('Ctrl Pts',(-14.5876477371938,17.0802404735808,1.27866666666653));
#25603=CARTESIAN_POINT('Ctrl Pts',(-15.5,17.0802404735808,1.23699999999987));
#25604=CARTESIAN_POINT('Ctrl Pts',(-16.4123522628062,17.0802404735808,1.1953333333332));
#25605=CARTESIAN_POINT('Ctrl Pts',(-16.8685283942094,16.2901202367904,1.15366666666653));
#25606=CARTESIAN_POINT('Ctrl Pts',(-17.3247045256125,15.5,1.11199999999986));
#25607=CARTESIAN_POINT('Ctrl Pts',(-16.8685283942094,14.7098797632096,1.0703333333332));
#25608=CARTESIAN_POINT('Ctrl Pts',(-16.4123522628062,13.9197595264192,1.02866666666653));
#25609=CARTESIAN_POINT('Ctrl Pts',(-15.5,13.9197595264192,0.986999999999863));
#25610=CARTESIAN_POINT('Ctrl Pts',(-14.5876477371938,13.9197595264192,0.945333333333196));
#25611=CARTESIAN_POINT('Ctrl Pts',(-14.1314716057906,14.7098797632096,0.903666666666529));
#25612=CARTESIAN_POINT('Ctrl Pts',(-13.6752954743875,15.5,0.861999999999861));
#25613=CARTESIAN_POINT('Ctrl Pts',(-14.1314716057906,16.2901202367904,0.820333333333194));
#25614=CARTESIAN_POINT('Ctrl Pts',(-14.5876477371938,17.0802404735808,0.778666666666527));
#25615=CARTESIAN_POINT('Ctrl Pts',(-15.5,17.0802404735808,0.736999999999859));
#25616=CARTESIAN_POINT('Ctrl Pts',(-16.4123522628062,17.0802404735808,0.695333333333192));
#25617=CARTESIAN_POINT('Ctrl Pts',(-16.8685283942094,16.2901202367904,0.653666666666525));
#25618=CARTESIAN_POINT('Ctrl Pts',(-17.3247045256125,15.5,0.611999999999857));
#25619=CARTESIAN_POINT('Ctrl Pts',(-16.8685283942094,14.7098797632096,0.57033333333319));
#25620=CARTESIAN_POINT('Ctrl Pts',(-16.4123522628062,13.9197595264192,0.528666666666523));
#25621=CARTESIAN_POINT('Ctrl Pts',(-15.5,13.9197595264192,0.486999999999856));
#25622=CARTESIAN_POINT('Ctrl Pts',(-14.5876477371938,13.9197595264192,0.445333333333188));
#25623=CARTESIAN_POINT('Ctrl Pts',(-14.1314716057906,14.7098797632096,0.403666666666521));
#25624=CARTESIAN_POINT('Ctrl Pts',(-13.6752954743875,15.5,0.361999999999854));
#25625=CARTESIAN_POINT('Ctrl Pts',(-14.1314716057906,16.2901202367904,0.320333333333186));
#25626=CARTESIAN_POINT('Ctrl Pts',(-14.5876477371938,17.0802404735808,0.278666666666519));
#25627=CARTESIAN_POINT('Ctrl Pts',(-15.5,17.0802404735808,0.236999999999852));
#25628=CARTESIAN_POINT('Ctrl Pts',(-16.4123522628062,17.0802404735808,0.195333333333185));
#25629=CARTESIAN_POINT('Ctrl Pts',(-16.8685283942094,16.2901202367904,0.153666666666517));
#25630=CARTESIAN_POINT('Ctrl Pts',(-17.3247045256125,15.5,0.11199999999985));
#25631=CARTESIAN_POINT('Ctrl Pts',(-16.8685283942094,14.7098797632096,0.0703333333331828));
#25632=CARTESIAN_POINT('Ctrl Pts',(-16.4123522628062,13.9197595264192,0.0286666666665155));
#25633=CARTESIAN_POINT('Ctrl Pts',(-15.5,13.9197595264192,-0.0130000000001518));
#25634=CARTESIAN_POINT('Ctrl Pts',(-14.5876477371938,13.9197595264192,-0.0546666666668173));
#25635=CARTESIAN_POINT('Ctrl Pts',(-14.1314716057906,14.7098797632096,-0.0963333333334846));
#25636=CARTESIAN_POINT('Ctrl Pts',(-13.6752954743875,15.5,-0.138000000000152));
#25637=CARTESIAN_POINT('Ctrl Pts',(-14.1314716057906,16.2901202367904,-0.179666666666819));
#25638=CARTESIAN_POINT('Ctrl Pts',(-14.5876477371938,17.0802404735808,-0.221333333333486));
#25639=CARTESIAN_POINT('Ctrl Pts',(-15.5,17.0802404735808,-0.263000000000154));
#25640=CARTESIAN_POINT('Ctrl Pts',(-16.4123522628062,17.0802404735808,-0.304666666666821));
#25641=CARTESIAN_POINT('Ctrl Pts',(-16.8685283942094,16.2901202367904,-0.346333333333488));
#25642=CARTESIAN_POINT('Ctrl Pts',(-17.3247045256125,15.5,-0.388000000000156));
#25643=CARTESIAN_POINT('Ctrl Pts',(-16.8685283942094,14.7098797632096,-0.429666666666823));
#25644=CARTESIAN_POINT('Ctrl Pts',(-16.4123522628062,13.9197595264192,-0.47133333333349));
#25645=CARTESIAN_POINT('Ctrl Pts',(-15.5,13.9197595264192,-0.513000000000157));
#25646=CARTESIAN_POINT('Ctrl Pts',(-14.5876477371938,13.9197595264192,-0.554666666666825));
#25647=CARTESIAN_POINT('Ctrl Pts',(-14.1314716057906,14.7098797632096,-0.596333333333492));
#25648=CARTESIAN_POINT('Ctrl Pts',(-13.6752954743875,15.5,-0.638000000000159));
#25649=CARTESIAN_POINT('Ctrl Pts',(-14.1314716057906,16.2901202367904,-0.679666666666827));
#25650=CARTESIAN_POINT('Ctrl Pts',(-14.5876477371938,17.0802404735808,-0.721333333333494));
#25651=CARTESIAN_POINT('Ctrl Pts',(-15.5,17.0802404735808,-0.763000000000161));
#25652=CARTESIAN_POINT('Ctrl Pts',(-16.4123522628062,17.0802404735808,-0.804666666666829));
#25653=CARTESIAN_POINT('Ctrl Pts',(-16.8685283942094,16.2901202367904,-0.846333333333496));
#25654=CARTESIAN_POINT('Ctrl Pts',(-17.3247045256125,15.5,-0.888000000000163));
#25655=CARTESIAN_POINT('Ctrl Pts',(-16.8685283942094,14.7098797632096,-0.92966666666683));
#25656=CARTESIAN_POINT('Ctrl Pts',(-16.4123522628062,13.9197595264192,-0.971333333333497));
#25657=CARTESIAN_POINT('Ctrl Pts',(-15.5,13.9197595264192,-1.01300000000016));
#25658=CARTESIAN_POINT('Ctrl Pts',(-14.5876477371938,13.9197595264192,-1.05466666666683));
#25659=CARTESIAN_POINT('Ctrl Pts',(-14.1314716057906,14.7098797632096,-1.0963333333335));
#25660=CARTESIAN_POINT('Ctrl Pts',(-13.6752954743875,15.5,-1.13800000000017));
#25661=CARTESIAN_POINT('Ctrl Pts',(-14.1314716057906,16.2901202367904,-1.17966666666683));
#25662=CARTESIAN_POINT('Ctrl Pts',(-14.5876477371938,17.0802404735808,-1.2213333333335));
#25663=CARTESIAN_POINT('Ctrl Pts',(-15.5,17.0802404735808,-1.26300000000017));
#25664=CARTESIAN_POINT('Ctrl Pts',(-16.4123522628062,17.0802404735808,-1.30466666666683));
#25665=CARTESIAN_POINT('Ctrl Pts',(-16.8685283942094,16.2901202367904,-1.3463333333335));
#25666=CARTESIAN_POINT('Ctrl Pts',(-17.3247045256125,15.5,-1.38800000000017));
#25667=CARTESIAN_POINT('Ctrl Pts',(-16.8685283942094,14.7098797632096,-1.42966666666684));
#25668=CARTESIAN_POINT('Ctrl Pts',(-16.4123522628062,13.9197595264192,-1.4713333333335));
#25669=CARTESIAN_POINT('Ctrl Pts',(-15.5,13.9197595264192,-1.51300000000017));
#25670=CARTESIAN_POINT('Ctrl Pts',(-14.5876477371938,13.9197595264192,-1.55466666666684));
#25671=CARTESIAN_POINT('Ctrl Pts',(-14.1314716057906,14.7098797632096,-1.59633333333351));
#25672=CARTESIAN_POINT('Ctrl Pts',(-13.6752954743875,15.5,-1.63800000000017));
#25673=CARTESIAN_POINT('Ctrl Pts',(-14.1314716057906,16.2901202367904,-1.67966666666684));
#25674=CARTESIAN_POINT('Ctrl Pts',(-14.5876477371938,17.0802404735808,-1.72133333333351));
#25675=CARTESIAN_POINT('Ctrl Pts',(-15.5,17.0802404735808,-1.76300000000017));
#25676=CARTESIAN_POINT('Ctrl Pts',(-16.4123522628062,17.0802404735808,-1.80466666666684));
#25677=CARTESIAN_POINT('Ctrl Pts',(-16.8685283942094,16.2901202367904,-1.84633333333351));
#25678=CARTESIAN_POINT('Ctrl Pts',(-17.3247045256125,15.5,-1.88800000000018));
#25679=CARTESIAN_POINT('Ctrl Pts',(-16.8685283942094,14.7098797632096,-1.92966666666684));
#25680=CARTESIAN_POINT('Ctrl Pts',(-16.7005797757653,14.4189842230035,-1.94500692368624));
#25681=CARTESIAN_POINT('Ctrl Pts',(-16.428831587743,14.221551003773,-1.96262330599533));
#25682=CARTESIAN_POINT('Origin',(-15.6296099418937,15.4374167911874,1.3857776251332));
#25683=CARTESIAN_POINT('',(-16.4288315898516,14.2215509627457,-1.96262324188451));
#25684=CARTESIAN_POINT('',(-16.4288304039466,14.2215500160357,-1.96262332703658));
#25685=CARTESIAN_POINT('Ctrl Pts',(-14.2313898004749,14.5577749122403,10.4122404735808));
#25686=CARTESIAN_POINT('Ctrl Pts',(-14.1770441521709,14.6309457974488,10.407829216981));
#25687=CARTESIAN_POINT('Ctrl Pts',(-14.1314716057906,14.7098797632096,10.4036666666667));
#25688=CARTESIAN_POINT('Ctrl Pts',(-13.6752954743875,15.5,10.362));
#25689=CARTESIAN_POINT('Ctrl Pts',(-14.1314716057906,16.2901202367904,10.3203333333333));
#25690=CARTESIAN_POINT('Ctrl Pts',(-14.5876477371938,17.0802404735808,10.2786666666667));
#25691=CARTESIAN_POINT('Ctrl Pts',(-15.5,17.0802404735808,10.237));
#25692=CARTESIAN_POINT('Ctrl Pts',(-16.4123522628062,17.0802404735808,10.1953333333333));
#25693=CARTESIAN_POINT('Ctrl Pts',(-16.8685283942094,16.2901202367904,10.1536666666667));
#25694=CARTESIAN_POINT('Ctrl Pts',(-17.3247045256125,15.5,10.112));
#25695=CARTESIAN_POINT('Ctrl Pts',(-16.8685283942094,14.7098797632096,10.0703333333333));
#25696=CARTESIAN_POINT('Ctrl Pts',(-16.4123522628062,13.9197595264192,10.0286666666667));
#25697=CARTESIAN_POINT('Ctrl Pts',(-15.5,13.9197595264192,9.98699999999998));
#25698=CARTESIAN_POINT('Ctrl Pts',(-14.5876477371938,13.9197595264192,9.94533333333331));
#25699=CARTESIAN_POINT('Ctrl Pts',(-14.1314716057906,14.7098797632096,9.90366666666665));
#25700=CARTESIAN_POINT('Ctrl Pts',(-13.6752954743875,15.5,9.86199999999998));
#25701=CARTESIAN_POINT('Ctrl Pts',(-14.1314716057906,16.2901202367904,9.82033333333331));
#25702=CARTESIAN_POINT('Ctrl Pts',(-14.5876477371938,17.0802404735808,9.77866666666665));
#25703=CARTESIAN_POINT('Ctrl Pts',(-15.5,17.0802404735808,9.73699999999998));
#25704=CARTESIAN_POINT('Ctrl Pts',(-16.4123522628062,17.0802404735808,9.69533333333331));
#25705=CARTESIAN_POINT('Ctrl Pts',(-16.8685283942094,16.2901202367904,9.65366666666664));
#25706=CARTESIAN_POINT('Ctrl Pts',(-17.3247045256125,15.5,9.61199999999998));
#25707=CARTESIAN_POINT('Ctrl Pts',(-16.8685283942094,14.7098797632096,9.57033333333331));
#25708=CARTESIAN_POINT('Ctrl Pts',(-16.4123522628062,13.9197595264192,9.52866666666664));
#25709=CARTESIAN_POINT('Ctrl Pts',(-15.5,13.9197595264192,9.48699999999998));
#25710=CARTESIAN_POINT('Ctrl Pts',(-14.5876477371938,13.9197595264192,9.44533333333331));
#25711=CARTESIAN_POINT('Ctrl Pts',(-14.1314716057906,14.7098797632096,9.40366666666664));
#25712=CARTESIAN_POINT('Ctrl Pts',(-13.6752954743875,15.5,9.36199999999998));
#25713=CARTESIAN_POINT('Ctrl Pts',(-14.1314716057906,16.2901202367904,9.32033333333331));
#25714=CARTESIAN_POINT('Ctrl Pts',(-14.5876477371938,17.0802404735808,9.27866666666664));
#25715=CARTESIAN_POINT('Ctrl Pts',(-15.5,17.0802404735808,9.23699999999997));
#25716=CARTESIAN_POINT('Ctrl Pts',(-16.4123522628062,17.0802404735808,9.19533333333331));
#25717=CARTESIAN_POINT('Ctrl Pts',(-16.8685283942094,16.2901202367904,9.15366666666664));
#25718=CARTESIAN_POINT('Ctrl Pts',(-17.3247045256125,15.5,9.11199999999997));
#25719=CARTESIAN_POINT('Ctrl Pts',(-16.8685283942094,14.7098797632096,9.0703333333333));
#25720=CARTESIAN_POINT('Ctrl Pts',(-16.4123522628062,13.9197595264192,9.02866666666664));
#25721=CARTESIAN_POINT('Ctrl Pts',(-15.5,13.9197595264192,8.98699999999997));
#25722=CARTESIAN_POINT('Ctrl Pts',(-14.5876477371938,13.9197595264192,8.9453333333333));
#25723=CARTESIAN_POINT('Ctrl Pts',(-14.1314716057906,14.7098797632096,8.90366666666664));
#25724=CARTESIAN_POINT('Ctrl Pts',(-13.6752954743875,15.5,8.86199999999997));
#25725=CARTESIAN_POINT('Ctrl Pts',(-14.1314716057906,16.2901202367904,8.8203333333333));
#25726=CARTESIAN_POINT('Ctrl Pts',(-14.5876477371938,17.0802404735808,8.77866666666663));
#25727=CARTESIAN_POINT('Ctrl Pts',(-15.5,17.0802404735808,8.73699999999997));
#25728=CARTESIAN_POINT('Ctrl Pts',(-16.4123522628062,17.0802404735808,8.6953333333333));
#25729=CARTESIAN_POINT('Ctrl Pts',(-16.8685283942094,16.2901202367904,8.65366666666663));
#25730=CARTESIAN_POINT('Ctrl Pts',(-17.3247045256125,15.5,8.61199999999996));
#25731=CARTESIAN_POINT('Ctrl Pts',(-16.8685283942094,14.7098797632096,8.57033333333329));
#25732=CARTESIAN_POINT('Ctrl Pts',(-16.4123522628062,13.9197595264192,8.52866666666663));
#25733=CARTESIAN_POINT('Ctrl Pts',(-15.5,13.9197595264192,8.48699999999996));
#25734=CARTESIAN_POINT('Ctrl Pts',(-14.5876477371938,13.9197595264192,8.44533333333329));
#25735=CARTESIAN_POINT('Ctrl Pts',(-14.1314716057906,14.7098797632096,8.40366666666663));
#25736=CARTESIAN_POINT('Ctrl Pts',(-13.6752954743875,15.5,8.36199999999996));
#25737=CARTESIAN_POINT('Ctrl Pts',(-14.1314716057906,16.2901202367904,8.32033333333329));
#25738=CARTESIAN_POINT('Ctrl Pts',(-14.5876477371938,17.0802404735808,8.27866666666663));
#25739=CARTESIAN_POINT('Ctrl Pts',(-15.5,17.0802404735808,8.23699999999996));
#25740=CARTESIAN_POINT('Ctrl Pts',(-16.4123522628062,17.0802404735808,8.19533333333329));
#25741=CARTESIAN_POINT('Ctrl Pts',(-16.8685283942094,16.2901202367904,8.15366666666663));
#25742=CARTESIAN_POINT('Ctrl Pts',(-17.3247045256125,15.5,8.11199999999996));
#25743=CARTESIAN_POINT('Ctrl Pts',(-16.8685283942094,14.7098797632096,8.07033333333329));
#25744=CARTESIAN_POINT('Ctrl Pts',(-16.4123522628062,13.9197595264192,8.02866666666662));
#25745=CARTESIAN_POINT('Ctrl Pts',(-15.5,13.9197595264192,7.98699999999996));
#25746=CARTESIAN_POINT('Ctrl Pts',(-14.5876477371938,13.9197595264192,7.94533333333329));
#25747=CARTESIAN_POINT('Ctrl Pts',(-14.1314716057906,14.7098797632096,7.90366666666662));
#25748=CARTESIAN_POINT('Ctrl Pts',(-13.6752954743875,15.5,7.86199999999995));
#25749=CARTESIAN_POINT('Ctrl Pts',(-14.1314716057906,16.2901202367904,7.82033333333329));
#25750=CARTESIAN_POINT('Ctrl Pts',(-14.5876477371938,17.0802404735808,7.77866666666662));
#25751=CARTESIAN_POINT('Ctrl Pts',(-15.5,17.0802404735808,7.73699999999995));
#25752=CARTESIAN_POINT('Ctrl Pts',(-16.4123522628062,17.0802404735808,7.69533333333329));
#25753=CARTESIAN_POINT('Ctrl Pts',(-16.8685283942094,16.2901202367904,7.65366666666662));
#25754=CARTESIAN_POINT('Ctrl Pts',(-17.3247045256125,15.5,7.61199999999995));
#25755=CARTESIAN_POINT('Ctrl Pts',(-16.8685283942094,14.7098797632096,7.57033333333328));
#25756=CARTESIAN_POINT('Ctrl Pts',(-16.4123522628062,13.9197595264192,7.52866666666662));
#25757=CARTESIAN_POINT('Ctrl Pts',(-15.5,13.9197595264192,7.48699999999995));
#25758=CARTESIAN_POINT('Ctrl Pts',(-14.5876477371938,13.9197595264192,7.44533333333328));
#25759=CARTESIAN_POINT('Ctrl Pts',(-14.1314716057906,14.7098797632096,7.40366666666661));
#25760=CARTESIAN_POINT('Ctrl Pts',(-13.6752954743875,15.5,7.36199999999995));
#25761=CARTESIAN_POINT('Ctrl Pts',(-14.1314716057906,16.2901202367904,7.32033333333328));
#25762=CARTESIAN_POINT('Ctrl Pts',(-14.5876477371938,17.0802404735808,7.27866666666661));
#25763=CARTESIAN_POINT('Ctrl Pts',(-15.5,17.0802404735808,7.23699999999995));
#25764=CARTESIAN_POINT('Ctrl Pts',(-16.4123522628062,17.0802404735808,7.19533333333328));
#25765=CARTESIAN_POINT('Ctrl Pts',(-16.8685283942094,16.2901202367904,7.15366666666661));
#25766=CARTESIAN_POINT('Ctrl Pts',(-17.3247045256125,15.5,7.11199999999994));
#25767=CARTESIAN_POINT('Ctrl Pts',(-16.8685283942094,14.7098797632096,7.07033333333328));
#25768=CARTESIAN_POINT('Ctrl Pts',(-16.4123522628062,13.9197595264192,7.02866666666661));
#25769=CARTESIAN_POINT('Ctrl Pts',(-15.5,13.9197595264192,6.98699999999994));
#25770=CARTESIAN_POINT('Ctrl Pts',(-14.5876477371938,13.9197595264192,6.94533333333327));
#25771=CARTESIAN_POINT('Ctrl Pts',(-14.1314716057906,14.7098797632096,6.90366666666661));
#25772=CARTESIAN_POINT('Ctrl Pts',(-13.6752954743875,15.5,6.86199999999994));
#25773=CARTESIAN_POINT('Ctrl Pts',(-14.1314716057906,16.2901202367904,6.82033333333327));
#25774=CARTESIAN_POINT('Ctrl Pts',(-14.5876477371938,17.0802404735808,6.77866666666661));
#25775=CARTESIAN_POINT('Ctrl Pts',(-15.5,17.0802404735808,6.73699999999994));
#25776=CARTESIAN_POINT('Ctrl Pts',(-16.4123522628062,17.0802404735808,6.69533333333327));
#25777=CARTESIAN_POINT('Ctrl Pts',(-16.8685283942094,16.2901202367904,6.65366666666661));
#25778=CARTESIAN_POINT('Ctrl Pts',(-17.3247045256125,15.5,6.61199999999994));
#25779=CARTESIAN_POINT('Ctrl Pts',(-16.8685283942094,14.7098797632096,6.57033333333327));
#25780=CARTESIAN_POINT('Ctrl Pts',(-16.4123522628062,13.9197595264192,6.5286666666666));
#25781=CARTESIAN_POINT('Ctrl Pts',(-15.5,13.9197595264192,6.48699999999994));
#25782=CARTESIAN_POINT('Ctrl Pts',(-14.5876477371938,13.9197595264192,6.44533333333327));
#25783=CARTESIAN_POINT('Ctrl Pts',(-14.1314716057906,14.7098797632096,6.4036666666666));
#25784=CARTESIAN_POINT('Ctrl Pts',(-13.6752954743875,15.5,6.36199999999993));
#25785=CARTESIAN_POINT('Ctrl Pts',(-14.1314716057906,16.2901202367904,6.32033333333327));
#25786=CARTESIAN_POINT('Ctrl Pts',(-14.5876477371938,17.0802404735808,6.2786666666666));
#25787=CARTESIAN_POINT('Ctrl Pts',(-15.5,17.0802404735808,6.23699999999993));
#25788=CARTESIAN_POINT('Ctrl Pts',(-16.4123522628062,17.0802404735808,6.19533333333326));
#25789=CARTESIAN_POINT('Ctrl Pts',(-16.8685283942094,16.2901202367904,6.1536666666666));
#25790=CARTESIAN_POINT('Ctrl Pts',(-17.3247045256125,15.5,6.11199999999993));
#25791=CARTESIAN_POINT('Ctrl Pts',(-16.8685283942094,14.7098797632096,6.07033333333326));
#25792=CARTESIAN_POINT('Ctrl Pts',(-16.4123522628062,13.9197595264192,6.0286666666666));
#25793=CARTESIAN_POINT('Ctrl Pts',(-15.5,13.9197595264192,5.98699999999993));
#25794=CARTESIAN_POINT('Ctrl Pts',(-14.5876477371938,13.9197595264192,5.94533333333326));
#25795=CARTESIAN_POINT('Ctrl Pts',(-14.1314716057906,14.7098797632096,5.9036666666666));
#25796=CARTESIAN_POINT('Ctrl Pts',(-13.6752954743875,15.5,5.86199999999993));
#25797=CARTESIAN_POINT('Ctrl Pts',(-14.1314716057906,16.2901202367904,5.82033333333326));
#25798=CARTESIAN_POINT('Ctrl Pts',(-14.5876477371938,17.0802404735808,5.77866666666659));
#25799=CARTESIAN_POINT('Ctrl Pts',(-15.5,17.0802404735808,5.73699999999993));
#25800=CARTESIAN_POINT('Ctrl Pts',(-16.4123522628062,17.0802404735808,5.69533333333326));
#25801=CARTESIAN_POINT('Ctrl Pts',(-16.8685283942094,16.2901202367904,5.65366666666659));
#25802=CARTESIAN_POINT('Ctrl Pts',(-17.3247045256125,15.5,5.61199999999992));
#25803=CARTESIAN_POINT('Ctrl Pts',(-16.8685283942094,14.7098797632096,5.57033333333326));
#25804=CARTESIAN_POINT('Ctrl Pts',(-16.4123522628062,13.9197595264192,5.52866666666659));
#25805=CARTESIAN_POINT('Ctrl Pts',(-15.5,13.9197595264192,5.48699999999992));
#25806=CARTESIAN_POINT('Ctrl Pts',(-14.5876477371938,13.9197595264192,5.44533333333326));
#25807=CARTESIAN_POINT('Ctrl Pts',(-14.1314716057906,14.7098797632096,5.40366666666659));
#25808=CARTESIAN_POINT('Ctrl Pts',(-13.6752954743875,15.5,5.36199999999992));
#25809=CARTESIAN_POINT('Ctrl Pts',(-14.1314716057906,16.2901202367904,5.32033333333325));
#25810=CARTESIAN_POINT('Ctrl Pts',(-14.5876477371938,17.0802404735808,5.27866666666659));
#25811=CARTESIAN_POINT('Ctrl Pts',(-15.5,17.0802404735808,5.23699999999992));
#25812=CARTESIAN_POINT('Ctrl Pts',(-16.4123522628062,17.0802404735808,5.19533333333325));
#25813=CARTESIAN_POINT('Ctrl Pts',(-16.8685283942094,16.2901202367904,5.15366666666658));
#25814=CARTESIAN_POINT('Ctrl Pts',(-17.3247045256125,15.5,5.11199999999992));
#25815=CARTESIAN_POINT('Ctrl Pts',(-16.8685283942094,14.7098797632096,5.07033333333325));
#25816=CARTESIAN_POINT('Ctrl Pts',(-16.4123522628062,13.9197595264192,5.02866666666658));
#25817=CARTESIAN_POINT('Ctrl Pts',(-15.5,13.9197595264192,4.98699999999992));
#25818=CARTESIAN_POINT('Ctrl Pts',(-14.5876477371938,13.9197595264192,4.94533333333325));
#25819=CARTESIAN_POINT('Ctrl Pts',(-14.1314716057906,14.7098797632096,4.90366666666658));
#25820=CARTESIAN_POINT('Ctrl Pts',(-13.6752954743875,15.5,4.86199999999991));
#25821=CARTESIAN_POINT('Ctrl Pts',(-14.1314716057906,16.2901202367904,4.82033333333325));
#25822=CARTESIAN_POINT('Ctrl Pts',(-14.5876477371938,17.0802404735808,4.77866666666658));
#25823=CARTESIAN_POINT('Ctrl Pts',(-15.5,17.0802404735808,4.73699999999991));
#25824=CARTESIAN_POINT('Ctrl Pts',(-16.4123522628062,17.0802404735808,4.69533333333325));
#25825=CARTESIAN_POINT('Ctrl Pts',(-16.8685283942094,16.2901202367904,4.65366666666658));
#25826=CARTESIAN_POINT('Ctrl Pts',(-17.3247045256125,15.5,4.61199999999991));
#25827=CARTESIAN_POINT('Ctrl Pts',(-16.8685283942094,14.7098797632096,4.57033333333324));
#25828=CARTESIAN_POINT('Ctrl Pts',(-16.4123522628062,13.9197595264192,4.52866666666658));
#25829=CARTESIAN_POINT('Ctrl Pts',(-15.5,13.9197595264192,4.48699999999991));
#25830=CARTESIAN_POINT('Ctrl Pts',(-14.5876477371938,13.9197595264192,4.44533333333324));
#25831=CARTESIAN_POINT('Ctrl Pts',(-14.1314716057906,14.7098797632096,4.40366666666658));
#25832=CARTESIAN_POINT('Ctrl Pts',(-13.6752954743875,15.5,4.36199999999991));
#25833=CARTESIAN_POINT('Ctrl Pts',(-14.1314716057906,16.2901202367904,4.32033333333324));
#25834=CARTESIAN_POINT('Ctrl Pts',(-14.5876477371938,17.0802404735808,4.27866666666657));
#25835=CARTESIAN_POINT('Ctrl Pts',(-15.5,17.0802404735808,4.23699999999991));
#25836=CARTESIAN_POINT('Ctrl Pts',(-16.4123522628062,17.0802404735808,4.19533333333324));
#25837=CARTESIAN_POINT('Ctrl Pts',(-16.8685283942094,16.2901202367904,4.15366666666657));
#25838=CARTESIAN_POINT('Ctrl Pts',(-17.3247045256125,15.5,4.1119999999999));
#25839=CARTESIAN_POINT('Ctrl Pts',(-16.8685283942094,14.7098797632096,4.07033333333324));
#25840=CARTESIAN_POINT('Ctrl Pts',(-16.4123522628062,13.9197595264192,4.02866666666657));
#25841=CARTESIAN_POINT('Ctrl Pts',(-15.5,13.9197595264192,3.9869999999999));
#25842=CARTESIAN_POINT('Ctrl Pts',(-14.5876477371938,13.9197595264192,3.94533333333323));
#25843=CARTESIAN_POINT('Ctrl Pts',(-14.1314716057906,14.7098797632096,3.90366666666657));
#25844=CARTESIAN_POINT('Ctrl Pts',(-13.6752954743875,15.5,3.8619999999999));
#25845=CARTESIAN_POINT('Ctrl Pts',(-14.1314716057906,16.2901202367904,3.82033333333323));
#25846=CARTESIAN_POINT('Ctrl Pts',(-14.5876477371938,17.0802404735808,3.77866666666657));
#25847=CARTESIAN_POINT('Ctrl Pts',(-15.5,17.0802404735808,3.7369999999999));
#25848=CARTESIAN_POINT('Ctrl Pts',(-16.4123522628062,17.0802404735808,3.69533333333323));
#25849=CARTESIAN_POINT('Ctrl Pts',(-16.8685283942094,16.2901202367904,3.65366666666656));
#25850=CARTESIAN_POINT('Ctrl Pts',(-17.3247045256125,15.5,3.6119999999999));
#25851=CARTESIAN_POINT('Ctrl Pts',(-16.8685283942094,14.7098797632096,3.57033333333323));
#25852=CARTESIAN_POINT('Ctrl Pts',(-16.4123522628062,13.9197595264192,3.52866666666656));
#25853=CARTESIAN_POINT('Ctrl Pts',(-15.5,13.9197595264192,3.4869999999999));
#25854=CARTESIAN_POINT('Ctrl Pts',(-14.5876477371938,13.9197595264192,3.44533333333323));
#25855=CARTESIAN_POINT('Ctrl Pts',(-14.1314716057906,14.7098797632096,3.40366666666656));
#25856=CARTESIAN_POINT('Ctrl Pts',(-13.6752954743875,15.5,3.36199999999989));
#25857=CARTESIAN_POINT('Ctrl Pts',(-14.1314716057906,16.2901202367904,3.32033333333323));
#25858=CARTESIAN_POINT('Ctrl Pts',(-14.5876477371938,17.0802404735808,3.27866666666656));
#25859=CARTESIAN_POINT('Ctrl Pts',(-15.5,17.0802404735808,3.23699999999989));
#25860=CARTESIAN_POINT('Ctrl Pts',(-16.4123522628062,17.0802404735808,3.19533333333323));
#25861=CARTESIAN_POINT('Ctrl Pts',(-16.8685283942094,16.2901202367904,3.15366666666656));
#25862=CARTESIAN_POINT('Ctrl Pts',(-17.3247045256125,15.5,3.11199999999989));
#25863=CARTESIAN_POINT('Ctrl Pts',(-16.8685283942094,14.7098797632096,3.07033333333322));
#25864=CARTESIAN_POINT('Ctrl Pts',(-16.4123522628062,13.9197595264192,3.02866666666656));
#25865=CARTESIAN_POINT('Ctrl Pts',(-15.5,13.9197595264192,2.98699999999989));
#25866=CARTESIAN_POINT('Ctrl Pts',(-14.5876477371938,13.9197595264192,2.94533333333322));
#25867=CARTESIAN_POINT('Ctrl Pts',(-14.1314716057906,14.7098797632096,2.90366666666656));
#25868=CARTESIAN_POINT('Ctrl Pts',(-13.6752954743875,15.5,2.86199999999989));
#25869=CARTESIAN_POINT('Ctrl Pts',(-14.1314716057906,16.2901202367904,2.82033333333322));
#25870=CARTESIAN_POINT('Ctrl Pts',(-14.5876477371938,17.0802404735808,2.77866666666655));
#25871=CARTESIAN_POINT('Ctrl Pts',(-15.5,17.0802404735808,2.73699999999989));
#25872=CARTESIAN_POINT('Ctrl Pts',(-16.4123522628062,17.0802404735808,2.69533333333322));
#25873=CARTESIAN_POINT('Ctrl Pts',(-16.8685283942094,16.2901202367904,2.65366666666655));
#25874=CARTESIAN_POINT('Ctrl Pts',(-17.3247045256125,15.5,2.61199999999988));
#25875=CARTESIAN_POINT('Ctrl Pts',(-16.8685283942094,14.7098797632096,2.57033333333322));
#25876=CARTESIAN_POINT('Ctrl Pts',(-16.4123522628062,13.9197595264192,2.52866666666655));
#25877=CARTESIAN_POINT('Ctrl Pts',(-15.5,13.9197595264192,2.48699999999988));
#25878=CARTESIAN_POINT('Ctrl Pts',(-14.5876477371938,13.9197595264192,2.44533333333321));
#25879=CARTESIAN_POINT('Ctrl Pts',(-14.1314716057906,14.7098797632096,2.40366666666655));
#25880=CARTESIAN_POINT('Ctrl Pts',(-13.6752954743875,15.5,2.36199999999988));
#25881=CARTESIAN_POINT('Ctrl Pts',(-14.1314716057906,16.2901202367904,2.32033333333321));
#25882=CARTESIAN_POINT('Ctrl Pts',(-14.5876477371938,17.0802404735808,2.27866666666655));
#25883=CARTESIAN_POINT('Ctrl Pts',(-15.5,17.0802404735808,2.23699999999988));
#25884=CARTESIAN_POINT('Ctrl Pts',(-16.4123522628062,17.0802404735808,2.19533333333321));
#25885=CARTESIAN_POINT('Ctrl Pts',(-16.8685283942094,16.2901202367904,2.15366666666655));
#25886=CARTESIAN_POINT('Ctrl Pts',(-17.3247045256125,15.5,2.11199999999988));
#25887=CARTESIAN_POINT('Ctrl Pts',(-16.8685283942094,14.7098797632096,2.07033333333321));
#25888=CARTESIAN_POINT('Ctrl Pts',(-16.4123522628062,13.9197595264192,2.02866666666654));
#25889=CARTESIAN_POINT('Ctrl Pts',(-15.5,13.9197595264192,1.98699999999988));
#25890=CARTESIAN_POINT('Ctrl Pts',(-14.5876477371938,13.9197595264192,1.94533333333321));
#25891=CARTESIAN_POINT('Ctrl Pts',(-14.1314716057906,14.7098797632096,1.90366666666654));
#25892=CARTESIAN_POINT('Ctrl Pts',(-13.6752954743875,15.5,1.86199999999987));
#25893=CARTESIAN_POINT('Ctrl Pts',(-14.1314716057906,16.2901202367904,1.82033333333321));
#25894=CARTESIAN_POINT('Ctrl Pts',(-14.5876477371938,17.0802404735808,1.77866666666654));
#25895=CARTESIAN_POINT('Ctrl Pts',(-15.5,17.0802404735808,1.73699999999987));
#25896=CARTESIAN_POINT('Ctrl Pts',(-16.4123522628062,17.0802404735808,1.6953333333332));
#25897=CARTESIAN_POINT('Ctrl Pts',(-16.8685283942094,16.2901202367904,1.65366666666654));
#25898=CARTESIAN_POINT('Ctrl Pts',(-17.3247045256125,15.5,1.61199999999987));
#25899=CARTESIAN_POINT('Ctrl Pts',(-16.8685283942094,14.7098797632096,1.5703333333332));
#25900=CARTESIAN_POINT('Ctrl Pts',(-16.4123522628062,13.9197595264192,1.52866666666654));
#25901=CARTESIAN_POINT('Ctrl Pts',(-15.5,13.9197595264192,1.48699999999987));
#25902=CARTESIAN_POINT('Ctrl Pts',(-14.5876477371938,13.9197595264192,1.4453333333332));
#25903=CARTESIAN_POINT('Ctrl Pts',(-14.1314716057906,14.7098797632096,1.40366666666653));
#25904=CARTESIAN_POINT('Ctrl Pts',(-13.6752954743875,15.5,1.36199999999987));
#25905=CARTESIAN_POINT('Ctrl Pts',(-14.1314716057906,16.2901202367904,1.3203333333332));
#25906=CARTESIAN_POINT('Ctrl Pts',(-14.5876477371938,17.0802404735808,1.27866666666653));
#25907=CARTESIAN_POINT('Ctrl Pts',(-15.5,17.0802404735808,1.23699999999987));
#25908=CARTESIAN_POINT('Ctrl Pts',(-16.4123522628062,17.0802404735808,1.1953333333332));
#25909=CARTESIAN_POINT('Ctrl Pts',(-16.8685283942094,16.2901202367904,1.15366666666653));
#25910=CARTESIAN_POINT('Ctrl Pts',(-17.3247045256125,15.5,1.11199999999986));
#25911=CARTESIAN_POINT('Ctrl Pts',(-16.8685283942094,14.7098797632096,1.0703333333332));
#25912=CARTESIAN_POINT('Ctrl Pts',(-16.4123522628062,13.9197595264192,1.02866666666653));
#25913=CARTESIAN_POINT('Ctrl Pts',(-15.5,13.9197595264192,0.986999999999863));
#25914=CARTESIAN_POINT('Ctrl Pts',(-14.5876477371938,13.9197595264192,0.945333333333196));
#25915=CARTESIAN_POINT('Ctrl Pts',(-14.1314716057906,14.7098797632096,0.903666666666529));
#25916=CARTESIAN_POINT('Ctrl Pts',(-13.6752954743875,15.5,0.861999999999861));
#25917=CARTESIAN_POINT('Ctrl Pts',(-14.1314716057906,16.2901202367904,0.820333333333194));
#25918=CARTESIAN_POINT('Ctrl Pts',(-14.5876477371938,17.0802404735808,0.778666666666527));
#25919=CARTESIAN_POINT('Ctrl Pts',(-15.5,17.0802404735808,0.736999999999859));
#25920=CARTESIAN_POINT('Ctrl Pts',(-16.4123522628062,17.0802404735808,0.695333333333192));
#25921=CARTESIAN_POINT('Ctrl Pts',(-16.8685283942094,16.2901202367904,0.653666666666525));
#25922=CARTESIAN_POINT('Ctrl Pts',(-17.3247045256125,15.5,0.611999999999858));
#25923=CARTESIAN_POINT('Ctrl Pts',(-16.8685283942094,14.7098797632096,0.57033333333319));
#25924=CARTESIAN_POINT('Ctrl Pts',(-16.4123522628062,13.9197595264192,0.528666666666523));
#25925=CARTESIAN_POINT('Ctrl Pts',(-15.5,13.9197595264192,0.486999999999856));
#25926=CARTESIAN_POINT('Ctrl Pts',(-14.5876477371938,13.9197595264192,0.445333333333188));
#25927=CARTESIAN_POINT('Ctrl Pts',(-14.1314716057906,14.7098797632096,0.403666666666521));
#25928=CARTESIAN_POINT('Ctrl Pts',(-13.6752954743875,15.5,0.361999999999854));
#25929=CARTESIAN_POINT('Ctrl Pts',(-14.1314716057906,16.2901202367904,0.320333333333186));
#25930=CARTESIAN_POINT('Ctrl Pts',(-14.5876477371938,17.0802404735808,0.278666666666519));
#25931=CARTESIAN_POINT('Ctrl Pts',(-15.5,17.0802404735808,0.236999999999852));
#25932=CARTESIAN_POINT('Ctrl Pts',(-16.4123522628062,17.0802404735808,0.195333333333185));
#25933=CARTESIAN_POINT('Ctrl Pts',(-16.8685283942094,16.2901202367904,0.153666666666517));
#25934=CARTESIAN_POINT('Ctrl Pts',(-17.3247045256125,15.5,0.11199999999985));
#25935=CARTESIAN_POINT('Ctrl Pts',(-16.8685283942094,14.7098797632096,0.0703333333331828));
#25936=CARTESIAN_POINT('Ctrl Pts',(-16.4123522628062,13.9197595264192,0.0286666666665155));
#25937=CARTESIAN_POINT('Ctrl Pts',(-15.5,13.9197595264192,-0.0130000000001518));
#25938=CARTESIAN_POINT('Ctrl Pts',(-14.5876477371938,13.9197595264192,-0.0546666666668173));
#25939=CARTESIAN_POINT('Ctrl Pts',(-14.1314716057906,14.7098797632096,-0.0963333333334846));
#25940=CARTESIAN_POINT('Ctrl Pts',(-13.6752954743875,15.5,-0.138000000000152));
#25941=CARTESIAN_POINT('Ctrl Pts',(-14.1314716057906,16.2901202367904,-0.179666666666819));
#25942=CARTESIAN_POINT('Ctrl Pts',(-14.5876477371938,17.0802404735808,-0.221333333333486));
#25943=CARTESIAN_POINT('Ctrl Pts',(-15.5,17.0802404735808,-0.263000000000154));
#25944=CARTESIAN_POINT('Ctrl Pts',(-16.4123522628062,17.0802404735808,-0.304666666666821));
#25945=CARTESIAN_POINT('Ctrl Pts',(-16.8685283942094,16.2901202367904,-0.346333333333488));
#25946=CARTESIAN_POINT('Ctrl Pts',(-17.3247045256125,15.5,-0.388000000000156));
#25947=CARTESIAN_POINT('Ctrl Pts',(-16.8685283942094,14.7098797632096,-0.429666666666823));
#25948=CARTESIAN_POINT('Ctrl Pts',(-16.4123522628062,13.9197595264192,-0.47133333333349));
#25949=CARTESIAN_POINT('Ctrl Pts',(-15.5,13.9197595264192,-0.513000000000157));
#25950=CARTESIAN_POINT('Ctrl Pts',(-14.5876477371938,13.9197595264192,-0.554666666666825));
#25951=CARTESIAN_POINT('Ctrl Pts',(-14.1314716057906,14.7098797632096,-0.596333333333492));
#25952=CARTESIAN_POINT('Ctrl Pts',(-13.6752954743875,15.5,-0.638000000000159));
#25953=CARTESIAN_POINT('Ctrl Pts',(-14.1314716057906,16.2901202367904,-0.679666666666827));
#25954=CARTESIAN_POINT('Ctrl Pts',(-14.5876477371938,17.0802404735808,-0.721333333333494));
#25955=CARTESIAN_POINT('Ctrl Pts',(-15.5,17.0802404735808,-0.763000000000161));
#25956=CARTESIAN_POINT('Ctrl Pts',(-16.4123522628062,17.0802404735808,-0.804666666666829));
#25957=CARTESIAN_POINT('Ctrl Pts',(-16.8685283942094,16.2901202367904,-0.846333333333496));
#25958=CARTESIAN_POINT('Ctrl Pts',(-17.3247045256125,15.5,-0.888000000000163));
#25959=CARTESIAN_POINT('Ctrl Pts',(-16.8685283942094,14.7098797632096,-0.92966666666683));
#25960=CARTESIAN_POINT('Ctrl Pts',(-16.4123522628062,13.9197595264192,-0.971333333333498));
#25961=CARTESIAN_POINT('Ctrl Pts',(-15.5,13.9197595264192,-1.01300000000016));
#25962=CARTESIAN_POINT('Ctrl Pts',(-14.5876477371938,13.9197595264192,-1.05466666666683));
#25963=CARTESIAN_POINT('Ctrl Pts',(-14.1314716057906,14.7098797632096,-1.0963333333335));
#25964=CARTESIAN_POINT('Ctrl Pts',(-13.6752954743875,15.5,-1.13800000000017));
#25965=CARTESIAN_POINT('Ctrl Pts',(-14.1314716057906,16.2901202367904,-1.17966666666683));
#25966=CARTESIAN_POINT('Ctrl Pts',(-14.5876477371938,17.0802404735808,-1.2213333333335));
#25967=CARTESIAN_POINT('Ctrl Pts',(-15.5,17.0802404735808,-1.26300000000017));
#25968=CARTESIAN_POINT('Ctrl Pts',(-16.4123522628062,17.0802404735808,-1.30466666666683));
#25969=CARTESIAN_POINT('Ctrl Pts',(-16.8685283942094,16.2901202367904,-1.3463333333335));
#25970=CARTESIAN_POINT('Ctrl Pts',(-17.3247045256125,15.5,-1.38800000000017));
#25971=CARTESIAN_POINT('Ctrl Pts',(-16.8685283942094,14.7098797632096,-1.42966666666684));
#25972=CARTESIAN_POINT('Ctrl Pts',(-16.4123522628062,13.9197595264192,-1.4713333333335));
#25973=CARTESIAN_POINT('Ctrl Pts',(-15.5,13.9197595264192,-1.51300000000017));
#25974=CARTESIAN_POINT('Ctrl Pts',(-14.5876477371938,13.9197595264192,-1.55466666666684));
#25975=CARTESIAN_POINT('Ctrl Pts',(-14.1314716057906,14.7098797632096,-1.59633333333351));
#25976=CARTESIAN_POINT('Ctrl Pts',(-13.6752954743875,15.5,-1.63800000000017));
#25977=CARTESIAN_POINT('Ctrl Pts',(-14.1314716057906,16.2901202367904,-1.67966666666684));
#25978=CARTESIAN_POINT('Ctrl Pts',(-14.5876477371938,17.0802404735808,-1.72133333333351));
#25979=CARTESIAN_POINT('Ctrl Pts',(-15.5,17.0802404735808,-1.76300000000017));
#25980=CARTESIAN_POINT('Ctrl Pts',(-16.4123522628062,17.0802404735808,-1.80466666666684));
#25981=CARTESIAN_POINT('Ctrl Pts',(-16.8685283942094,16.2901202367904,-1.84633333333351));
#25982=CARTESIAN_POINT('Ctrl Pts',(-17.3247045256125,15.5,-1.88800000000018));
#25983=CARTESIAN_POINT('Ctrl Pts',(-16.8685283942094,14.7098797632096,-1.92966666666684));
#25984=CARTESIAN_POINT('Ctrl Pts',(-16.700583153372,14.4189900731899,-1.94500661517905));
#25985=CARTESIAN_POINT('Ctrl Pts',(-16.4288340223699,14.2215527726061,-1.96262314816781));
#25986=CARTESIAN_POINT('Origin',(-16.5839252605846,14.0080754615186,-2.17746715486548));
#25987=CARTESIAN_POINT('',(-16.4288300625788,14.2215498957104,-2.02512301642216));
#25988=CARTESIAN_POINT('Ctrl Pts',(-15.5,17.0802404735808,11.2370201234482));
#25989=CARTESIAN_POINT('Ctrl Pts',(-16.4123522628062,17.0802404735808,11.1953534567815));
#25990=CARTESIAN_POINT('Ctrl Pts',(-16.8685283942094,16.2901202367904,11.1536867901149));
#25991=CARTESIAN_POINT('Ctrl Pts',(-17.3247045256125,15.5,11.1120201234482));
#25992=CARTESIAN_POINT('Ctrl Pts',(-16.8685283942094,14.7098797632096,11.0703534567815));
#25993=CARTESIAN_POINT('Ctrl Pts',(-16.4123522628062,13.9197595264192,11.0286867901149));
#25994=CARTESIAN_POINT('Ctrl Pts',(-15.5,13.9197595264192,10.9870201234482));
#25995=CARTESIAN_POINT('Ctrl Pts',(-14.5876477371938,13.9197595264192,10.9453534567815));
#25996=CARTESIAN_POINT('Ctrl Pts',(-14.1314716057906,14.7098797632096,10.9036867901149));
#25997=CARTESIAN_POINT('Ctrl Pts',(-13.6752954743875,15.5,10.8620201234482));
#25998=CARTESIAN_POINT('Ctrl Pts',(-14.1314716057906,16.2901202367904,10.8203534567815));
#25999=CARTESIAN_POINT('Ctrl Pts',(-14.5876477371938,17.0802404735808,10.7786867901149));
#26000=CARTESIAN_POINT('Ctrl Pts',(-15.5,17.0802404735808,10.7370201234482));
#26001=CARTESIAN_POINT('Ctrl Pts',(-16.4123522628062,17.0802404735808,10.6953534567815));
#26002=CARTESIAN_POINT('Ctrl Pts',(-16.8685283942094,16.2901202367904,10.6536867901149));
#26003=CARTESIAN_POINT('Ctrl Pts',(-17.3247045256125,15.5,10.6120201234482));
#26004=CARTESIAN_POINT('Ctrl Pts',(-16.8685283942094,14.7098797632096,10.5703534567815));
#26005=CARTESIAN_POINT('Ctrl Pts',(-16.4123522628062,13.9197595264192,10.5286867901149));
#26006=CARTESIAN_POINT('Ctrl Pts',(-15.5,13.9197595264192,10.4870201234482));
#26007=CARTESIAN_POINT('Ctrl Pts',(-14.5876477371938,13.9197595264192,10.4453534567815));
#26008=CARTESIAN_POINT('Ctrl Pts',(-14.1314716057906,14.7098797632096,10.4036867901149));
#26009=CARTESIAN_POINT('Ctrl Pts',(-13.6752954743875,15.5,10.3620201234482));
#26010=CARTESIAN_POINT('Ctrl Pts',(-14.1314716057906,16.2901202367904,10.3203534567815));
#26011=CARTESIAN_POINT('Ctrl Pts',(-14.5876477371938,17.0802404735808,10.2786867901149));
#26012=CARTESIAN_POINT('Ctrl Pts',(-15.5,17.0802404735808,10.2370201234482));
#26013=CARTESIAN_POINT('Ctrl Pts',(-16.4123522628062,17.0802404735808,10.1953534567815));
#26014=CARTESIAN_POINT('Ctrl Pts',(-16.8685283942094,16.2901202367904,10.1536867901149));
#26015=CARTESIAN_POINT('Ctrl Pts',(-17.3247045256125,15.5,10.1120201234482));
#26016=CARTESIAN_POINT('Ctrl Pts',(-16.8685283942094,14.7098797632096,10.0703534567815));
#26017=CARTESIAN_POINT('Ctrl Pts',(-16.4123522628062,13.9197595264192,10.0286867901149));
#26018=CARTESIAN_POINT('Ctrl Pts',(-15.5,13.9197595264192,9.98702012344818));
#26019=CARTESIAN_POINT('Ctrl Pts',(-14.5876477371938,13.9197595264192,9.94535345678152));
#26020=CARTESIAN_POINT('Ctrl Pts',(-14.1314716057906,14.7098797632096,9.90368679011485));
#26021=CARTESIAN_POINT('Ctrl Pts',(-13.6752954743875,15.5,9.86202012344818));
#26022=CARTESIAN_POINT('Ctrl Pts',(-14.1314716057906,16.2901202367904,9.82035345678152));
#26023=CARTESIAN_POINT('Ctrl Pts',(-14.5876477371938,17.0802404735808,9.77868679011485));
#26024=CARTESIAN_POINT('Ctrl Pts',(-15.5,17.0802404735808,9.73702012344818));
#26025=CARTESIAN_POINT('Ctrl Pts',(-16.4123522628062,17.0802404735808,9.69535345678152));
#26026=CARTESIAN_POINT('Ctrl Pts',(-16.8685283942094,16.2901202367904,9.65368679011485));
#26027=CARTESIAN_POINT('Ctrl Pts',(-17.3247045256125,15.5,9.61202012344818));
#26028=CARTESIAN_POINT('Ctrl Pts',(-16.8685283942094,14.7098797632096,9.57035345678151));
#26029=CARTESIAN_POINT('Ctrl Pts',(-16.4123522628062,13.9197595264192,9.52868679011484));
#26030=CARTESIAN_POINT('Ctrl Pts',(-15.5,13.9197595264192,9.48702012344818));
#26031=CARTESIAN_POINT('Ctrl Pts',(-14.5876477371938,13.9197595264192,9.44535345678151));
#26032=CARTESIAN_POINT('Ctrl Pts',(-14.1314716057906,14.7098797632096,9.40368679011484));
#26033=CARTESIAN_POINT('Ctrl Pts',(-13.6752954743875,15.5,9.36202012344818));
#26034=CARTESIAN_POINT('Ctrl Pts',(-14.1314716057906,16.2901202367904,9.32035345678151));
#26035=CARTESIAN_POINT('Ctrl Pts',(-14.5876477371938,17.0802404735808,9.27868679011484));
#26036=CARTESIAN_POINT('Ctrl Pts',(-15.5,17.0802404735808,9.23702012344818));
#26037=CARTESIAN_POINT('Ctrl Pts',(-16.4123522628062,17.0802404735808,9.19535345678151));
#26038=CARTESIAN_POINT('Ctrl Pts',(-16.8685283942094,16.2901202367904,9.15368679011484));
#26039=CARTESIAN_POINT('Ctrl Pts',(-17.3247045256125,15.5,9.11202012344818));
#26040=CARTESIAN_POINT('Ctrl Pts',(-16.8685283942094,14.7098797632096,9.07035345678151));
#26041=CARTESIAN_POINT('Ctrl Pts',(-16.4123522628062,13.9197595264192,9.02868679011484));
#26042=CARTESIAN_POINT('Ctrl Pts',(-15.5,13.9197595264192,8.98702012344817));
#26043=CARTESIAN_POINT('Ctrl Pts',(-14.5876477371938,13.9197595264192,8.9453534567815));
#26044=CARTESIAN_POINT('Ctrl Pts',(-14.1314716057906,14.7098797632096,8.90368679011484));
#26045=CARTESIAN_POINT('Ctrl Pts',(-13.6752954743875,15.5,8.86202012344817));
#26046=CARTESIAN_POINT('Ctrl Pts',(-14.1314716057906,16.2901202367904,8.8203534567815));
#26047=CARTESIAN_POINT('Ctrl Pts',(-14.5876477371938,17.0802404735808,8.77868679011483));
#26048=CARTESIAN_POINT('Ctrl Pts',(-15.5,17.0802404735808,8.73702012344817));
#26049=CARTESIAN_POINT('Ctrl Pts',(-16.4123522628062,17.0802404735808,8.6953534567815));
#26050=CARTESIAN_POINT('Ctrl Pts',(-16.8685283942094,16.2901202367904,8.65368679011483));
#26051=CARTESIAN_POINT('Ctrl Pts',(-17.3247045256125,15.5,8.61202012344817));
#26052=CARTESIAN_POINT('Ctrl Pts',(-16.8685283942094,14.7098797632096,8.5703534567815));
#26053=CARTESIAN_POINT('Ctrl Pts',(-16.4123522628062,13.9197595264192,8.52868679011483));
#26054=CARTESIAN_POINT('Ctrl Pts',(-15.5,13.9197595264192,8.48702012344816));
#26055=CARTESIAN_POINT('Ctrl Pts',(-14.5876477371938,13.9197595264192,8.4453534567815));
#26056=CARTESIAN_POINT('Ctrl Pts',(-14.1314716057906,14.7098797632096,8.40368679011483));
#26057=CARTESIAN_POINT('Ctrl Pts',(-13.6752954743875,15.5,8.36202012344816));
#26058=CARTESIAN_POINT('Ctrl Pts',(-14.1314716057906,16.2901202367904,8.3203534567815));
#26059=CARTESIAN_POINT('Ctrl Pts',(-14.5876477371938,17.0802404735808,8.27868679011483));
#26060=CARTESIAN_POINT('Ctrl Pts',(-15.5,17.0802404735808,8.23702012344816));
#26061=CARTESIAN_POINT('Ctrl Pts',(-16.4123522628062,17.0802404735808,8.19535345678149));
#26062=CARTESIAN_POINT('Ctrl Pts',(-16.8685283942094,16.2901202367904,8.15368679011483));
#26063=CARTESIAN_POINT('Ctrl Pts',(-17.3247045256125,15.5,8.11202012344816));
#26064=CARTESIAN_POINT('Ctrl Pts',(-16.8685283942094,14.7098797632096,8.0703534567815));
#26065=CARTESIAN_POINT('Ctrl Pts',(-16.4123522628062,13.9197595264192,8.02868679011483));
#26066=CARTESIAN_POINT('Ctrl Pts',(-15.5,13.9197595264192,7.98702012344816));
#26067=CARTESIAN_POINT('Ctrl Pts',(-14.5876477371938,13.9197595264192,7.94535345678149));
#26068=CARTESIAN_POINT('Ctrl Pts',(-14.1314716057906,14.7098797632096,7.90368679011482));
#26069=CARTESIAN_POINT('Ctrl Pts',(-13.6752954743875,15.5,7.86202012344816));
#26070=CARTESIAN_POINT('Ctrl Pts',(-14.1314716057906,16.2901202367904,7.82035345678149));
#26071=CARTESIAN_POINT('Ctrl Pts',(-14.5876477371938,17.0802404735808,7.77868679011482));
#26072=CARTESIAN_POINT('Ctrl Pts',(-15.5,17.0802404735808,7.73702012344816));
#26073=CARTESIAN_POINT('Ctrl Pts',(-16.4123522628062,17.0802404735808,7.69535345678149));
#26074=CARTESIAN_POINT('Ctrl Pts',(-16.8685283942094,16.2901202367904,7.65368679011482));
#26075=CARTESIAN_POINT('Ctrl Pts',(-17.3247045256125,15.5,7.61202012344815));
#26076=CARTESIAN_POINT('Ctrl Pts',(-16.8685283942094,14.7098797632096,7.57035345678149));
#26077=CARTESIAN_POINT('Ctrl Pts',(-16.4123522628062,13.9197595264192,7.52868679011482));
#26078=CARTESIAN_POINT('Ctrl Pts',(-15.5,13.9197595264192,7.48702012344815));
#26079=CARTESIAN_POINT('Ctrl Pts',(-14.5876477371938,13.9197595264192,7.44535345678149));
#26080=CARTESIAN_POINT('Ctrl Pts',(-14.1314716057906,14.7098797632096,7.40368679011482));
#26081=CARTESIAN_POINT('Ctrl Pts',(-13.6752954743875,15.5,7.36202012344815));
#26082=CARTESIAN_POINT('Ctrl Pts',(-14.1314716057906,16.2901202367904,7.32035345678148));
#26083=CARTESIAN_POINT('Ctrl Pts',(-14.5876477371938,17.0802404735808,7.27868679011482));
#26084=CARTESIAN_POINT('Ctrl Pts',(-15.5,17.0802404735808,7.23702012344815));
#26085=CARTESIAN_POINT('Ctrl Pts',(-16.4123522628062,17.0802404735808,7.19535345678148));
#26086=CARTESIAN_POINT('Ctrl Pts',(-16.8685283942094,16.2901202367904,7.15368679011481));
#26087=CARTESIAN_POINT('Ctrl Pts',(-17.3247045256125,15.5,7.11202012344815));
#26088=CARTESIAN_POINT('Ctrl Pts',(-16.8685283942094,14.7098797632096,7.07035345678148));
#26089=CARTESIAN_POINT('Ctrl Pts',(-16.4123522628062,13.9197595264192,7.02868679011481));
#26090=CARTESIAN_POINT('Ctrl Pts',(-15.5,13.9197595264192,6.98702012344814));
#26091=CARTESIAN_POINT('Ctrl Pts',(-14.5876477371938,13.9197595264192,6.94535345678148));
#26092=CARTESIAN_POINT('Ctrl Pts',(-14.1314716057906,14.7098797632096,6.90368679011481));
#26093=CARTESIAN_POINT('Ctrl Pts',(-13.6752954743875,15.5,6.86202012344814));
#26094=CARTESIAN_POINT('Ctrl Pts',(-14.1314716057906,16.2901202367904,6.82035345678148));
#26095=CARTESIAN_POINT('Ctrl Pts',(-14.5876477371938,17.0802404735808,6.77868679011481));
#26096=CARTESIAN_POINT('Ctrl Pts',(-15.5,17.0802404735808,6.73702012344814));
#26097=CARTESIAN_POINT('Ctrl Pts',(-16.4123522628062,17.0802404735808,6.69535345678147));
#26098=CARTESIAN_POINT('Ctrl Pts',(-16.8685283942094,16.2901202367904,6.65368679011481));
#26099=CARTESIAN_POINT('Ctrl Pts',(-17.3247045256125,15.5,6.61202012344814));
#26100=CARTESIAN_POINT('Ctrl Pts',(-16.8685283942094,14.7098797632096,6.57035345678147));
#26101=CARTESIAN_POINT('Ctrl Pts',(-16.4123522628062,13.9197595264192,6.52868679011481));
#26102=CARTESIAN_POINT('Ctrl Pts',(-15.5,13.9197595264192,6.48702012344814));
#26103=CARTESIAN_POINT('Ctrl Pts',(-14.5876477371938,13.9197595264192,6.44535345678147));
#26104=CARTESIAN_POINT('Ctrl Pts',(-14.1314716057906,14.7098797632096,6.40368679011481));
#26105=CARTESIAN_POINT('Ctrl Pts',(-13.6752954743875,15.5,6.36202012344814));
#26106=CARTESIAN_POINT('Ctrl Pts',(-14.1314716057906,16.2901202367904,6.32035345678147));
#26107=CARTESIAN_POINT('Ctrl Pts',(-14.5876477371938,17.0802404735808,6.2786867901148));
#26108=CARTESIAN_POINT('Ctrl Pts',(-15.5,17.0802404735808,6.23702012344813));
#26109=CARTESIAN_POINT('Ctrl Pts',(-16.4123522628062,17.0802404735808,6.19535345678147));
#26110=CARTESIAN_POINT('Ctrl Pts',(-16.8685283942094,16.2901202367904,6.1536867901148));
#26111=CARTESIAN_POINT('Ctrl Pts',(-17.3247045256125,15.5,6.11202012344813));
#26112=CARTESIAN_POINT('Ctrl Pts',(-16.8685283942094,14.7098797632096,6.07035345678146));
#26113=CARTESIAN_POINT('Ctrl Pts',(-16.4123522628062,13.9197595264192,6.0286867901148));
#26114=CARTESIAN_POINT('Ctrl Pts',(-15.5,13.9197595264192,5.98702012344813));
#26115=CARTESIAN_POINT('Ctrl Pts',(-14.5876477371938,13.9197595264192,5.94535345678146));
#26116=CARTESIAN_POINT('Ctrl Pts',(-14.1314716057906,14.7098797632096,5.9036867901148));
#26117=CARTESIAN_POINT('Ctrl Pts',(-13.6752954743875,15.5,5.86202012344813));
#26118=CARTESIAN_POINT('Ctrl Pts',(-14.1314716057906,16.2901202367904,5.82035345678146));
#26119=CARTESIAN_POINT('Ctrl Pts',(-14.5876477371938,17.0802404735808,5.77868679011479));
#26120=CARTESIAN_POINT('Ctrl Pts',(-15.5,17.0802404735808,5.73702012344813));
#26121=CARTESIAN_POINT('Ctrl Pts',(-16.4123522628062,17.0802404735808,5.69535345678146));
#26122=CARTESIAN_POINT('Ctrl Pts',(-16.8685283942094,16.2901202367904,5.65368679011479));
#26123=CARTESIAN_POINT('Ctrl Pts',(-17.3247045256125,15.5,5.61202012344813));
#26124=CARTESIAN_POINT('Ctrl Pts',(-16.8685283942094,14.7098797632096,5.57035345678146));
#26125=CARTESIAN_POINT('Ctrl Pts',(-16.4123522628062,13.9197595264192,5.52868679011479));
#26126=CARTESIAN_POINT('Ctrl Pts',(-15.5,13.9197595264192,5.48702012344813));
#26127=CARTESIAN_POINT('Ctrl Pts',(-14.5876477371938,13.9197595264192,5.44535345678146));
#26128=CARTESIAN_POINT('Ctrl Pts',(-14.1314716057906,14.7098797632096,5.40368679011479));
#26129=CARTESIAN_POINT('Ctrl Pts',(-13.6752954743875,15.5,5.36202012344812));
#26130=CARTESIAN_POINT('Ctrl Pts',(-14.1314716057906,16.2901202367904,5.32035345678146));
#26131=CARTESIAN_POINT('Ctrl Pts',(-14.5876477371938,17.0802404735808,5.27868679011479));
#26132=CARTESIAN_POINT('Ctrl Pts',(-15.5,17.0802404735808,5.23702012344812));
#26133=CARTESIAN_POINT('Ctrl Pts',(-16.4123522628062,17.0802404735808,5.19535345678145));
#26134=CARTESIAN_POINT('Ctrl Pts',(-16.8685283942094,16.2901202367904,5.15368679011479));
#26135=CARTESIAN_POINT('Ctrl Pts',(-17.3247045256125,15.5,5.11202012344812));
#26136=CARTESIAN_POINT('Ctrl Pts',(-16.8685283942094,14.7098797632096,5.07035345678145));
#26137=CARTESIAN_POINT('Ctrl Pts',(-16.4123522628062,13.9197595264192,5.02868679011478));
#26138=CARTESIAN_POINT('Ctrl Pts',(-15.5,13.9197595264192,4.98702012344812));
#26139=CARTESIAN_POINT('Ctrl Pts',(-14.5876477371938,13.9197595264192,4.94535345678145));
#26140=CARTESIAN_POINT('Ctrl Pts',(-14.1314716057906,14.7098797632096,4.90368679011478));
#26141=CARTESIAN_POINT('Ctrl Pts',(-13.6752954743875,15.5,4.86202012344812));
#26142=CARTESIAN_POINT('Ctrl Pts',(-14.1314716057906,16.2901202367904,4.82035345678145));
#26143=CARTESIAN_POINT('Ctrl Pts',(-14.5876477371938,17.0802404735808,4.77868679011478));
#26144=CARTESIAN_POINT('Ctrl Pts',(-15.5,17.0802404735808,4.73702012344812));
#26145=CARTESIAN_POINT('Ctrl Pts',(-16.4123522628062,17.0802404735808,4.69535345678145));
#26146=CARTESIAN_POINT('Ctrl Pts',(-16.8685283942094,16.2901202367904,4.65368679011478));
#26147=CARTESIAN_POINT('Ctrl Pts',(-17.3247045256125,15.5,4.61202012344811));
#26148=CARTESIAN_POINT('Ctrl Pts',(-16.8685283942094,14.7098797632096,4.57035345678145));
#26149=CARTESIAN_POINT('Ctrl Pts',(-16.4123522628062,13.9197595264192,4.52868679011478));
#26150=CARTESIAN_POINT('Ctrl Pts',(-15.5,13.9197595264192,4.48702012344811));
#26151=CARTESIAN_POINT('Ctrl Pts',(-14.5876477371938,13.9197595264192,4.44535345678144));
#26152=CARTESIAN_POINT('Ctrl Pts',(-14.1314716057906,14.7098797632096,4.40368679011478));
#26153=CARTESIAN_POINT('Ctrl Pts',(-13.6752954743875,15.5,4.36202012344811));
#26154=CARTESIAN_POINT('Ctrl Pts',(-14.1314716057906,16.2901202367904,4.32035345678144));
#26155=CARTESIAN_POINT('Ctrl Pts',(-14.5876477371938,17.0802404735808,4.27868679011477));
#26156=CARTESIAN_POINT('Ctrl Pts',(-15.5,17.0802404735808,4.23702012344811));
#26157=CARTESIAN_POINT('Ctrl Pts',(-16.4123522628062,17.0802404735808,4.19535345678144));
#26158=CARTESIAN_POINT('Ctrl Pts',(-16.8685283942094,16.2901202367904,4.15368679011477));
#26159=CARTESIAN_POINT('Ctrl Pts',(-17.3247045256125,15.5,4.11202012344811));
#26160=CARTESIAN_POINT('Ctrl Pts',(-16.8685283942094,14.7098797632096,4.07035345678144));
#26161=CARTESIAN_POINT('Ctrl Pts',(-16.4123522628062,13.9197595264192,4.02868679011477));
#26162=CARTESIAN_POINT('Ctrl Pts',(-15.5,13.9197595264192,3.9870201234481));
#26163=CARTESIAN_POINT('Ctrl Pts',(-14.5876477371938,13.9197595264192,3.94535345678144));
#26164=CARTESIAN_POINT('Ctrl Pts',(-14.1314716057906,14.7098797632096,3.90368679011477));
#26165=CARTESIAN_POINT('Ctrl Pts',(-13.6752954743875,15.5,3.8620201234481));
#26166=CARTESIAN_POINT('Ctrl Pts',(-14.1314716057906,16.2901202367904,3.82035345678144));
#26167=CARTESIAN_POINT('Ctrl Pts',(-14.5876477371938,17.0802404735808,3.77868679011477));
#26168=CARTESIAN_POINT('Ctrl Pts',(-15.5,17.0802404735808,3.7370201234481));
#26169=CARTESIAN_POINT('Ctrl Pts',(-16.4123522628062,17.0802404735808,3.69535345678143));
#26170=CARTESIAN_POINT('Ctrl Pts',(-16.8685283942094,16.2901202367904,3.65368679011477));
#26171=CARTESIAN_POINT('Ctrl Pts',(-17.3247045256125,15.5,3.6120201234481));
#26172=CARTESIAN_POINT('Ctrl Pts',(-16.8685283942094,14.7098797632096,3.57035345678143));
#26173=CARTESIAN_POINT('Ctrl Pts',(-16.4123522628062,13.9197595264192,3.52868679011477));
#26174=CARTESIAN_POINT('Ctrl Pts',(-15.5,13.9197595264192,3.4870201234481));
#26175=CARTESIAN_POINT('Ctrl Pts',(-14.5876477371938,13.9197595264192,3.44535345678143));
#26176=CARTESIAN_POINT('Ctrl Pts',(-14.1314716057906,14.7098797632096,3.40368679011476));
#26177=CARTESIAN_POINT('Ctrl Pts',(-13.6752954743875,15.5,3.3620201234481));
#26178=CARTESIAN_POINT('Ctrl Pts',(-14.1314716057906,16.2901202367904,3.32035345678143));
#26179=CARTESIAN_POINT('Ctrl Pts',(-14.5876477371938,17.0802404735808,3.27868679011476));
#26180=CARTESIAN_POINT('Ctrl Pts',(-15.5,17.0802404735808,3.2370201234481));
#26181=CARTESIAN_POINT('Ctrl Pts',(-16.4123522628062,17.0802404735808,3.19535345678143));
#26182=CARTESIAN_POINT('Ctrl Pts',(-16.8685283942094,16.2901202367904,3.15368679011476));
#26183=CARTESIAN_POINT('Ctrl Pts',(-17.3247045256125,15.5,3.11202012344809));
#26184=CARTESIAN_POINT('Ctrl Pts',(-16.8685283942094,14.7098797632096,3.07035345678143));
#26185=CARTESIAN_POINT('Ctrl Pts',(-16.4123522628062,13.9197595264192,3.02868679011476));
#26186=CARTESIAN_POINT('Ctrl Pts',(-15.5,13.9197595264192,2.98702012344809));
#26187=CARTESIAN_POINT('Ctrl Pts',(-14.5876477371938,13.9197595264192,2.94535345678142));
#26188=CARTESIAN_POINT('Ctrl Pts',(-14.1314716057906,14.7098797632096,2.90368679011476));
#26189=CARTESIAN_POINT('Ctrl Pts',(-13.6752954743875,15.5,2.86202012344809));
#26190=CARTESIAN_POINT('Ctrl Pts',(-14.1314716057906,16.2901202367904,2.82035345678142));
#26191=CARTESIAN_POINT('Ctrl Pts',(-14.5876477371938,17.0802404735808,2.77868679011475));
#26192=CARTESIAN_POINT('Ctrl Pts',(-15.5,17.0802404735808,2.73702012344809));
#26193=CARTESIAN_POINT('Ctrl Pts',(-16.4123522628062,17.0802404735808,2.69535345678142));
#26194=CARTESIAN_POINT('Ctrl Pts',(-16.8685283942094,16.2901202367904,2.65368679011475));
#26195=CARTESIAN_POINT('Ctrl Pts',(-17.3247045256125,15.5,2.61202012344809));
#26196=CARTESIAN_POINT('Ctrl Pts',(-16.8685283942094,14.7098797632096,2.57035345678142));
#26197=CARTESIAN_POINT('Ctrl Pts',(-16.4123522628062,13.9197595264192,2.52868679011475));
#26198=CARTESIAN_POINT('Ctrl Pts',(-15.5,13.9197595264192,2.48702012344808));
#26199=CARTESIAN_POINT('Ctrl Pts',(-14.5876477371938,13.9197595264192,2.44535345678142));
#26200=CARTESIAN_POINT('Ctrl Pts',(-14.1314716057906,14.7098797632096,2.40368679011475));
#26201=CARTESIAN_POINT('Ctrl Pts',(-13.6752954743875,15.5,2.36202012344808));
#26202=CARTESIAN_POINT('Ctrl Pts',(-14.1314716057906,16.2901202367904,2.32035345678142));
#26203=CARTESIAN_POINT('Ctrl Pts',(-14.5876477371938,17.0802404735808,2.27868679011475));
#26204=CARTESIAN_POINT('Ctrl Pts',(-15.5,17.0802404735808,2.23702012344808));
#26205=CARTESIAN_POINT('Ctrl Pts',(-16.4123522628062,17.0802404735808,2.19535345678141));
#26206=CARTESIAN_POINT('Ctrl Pts',(-16.8685283942094,16.2901202367904,2.15368679011475));
#26207=CARTESIAN_POINT('Ctrl Pts',(-17.3247045256125,15.5,2.11202012344808));
#26208=CARTESIAN_POINT('Ctrl Pts',(-16.8685283942094,14.7098797632096,2.07035345678141));
#26209=CARTESIAN_POINT('Ctrl Pts',(-16.4123522628062,13.9197595264192,2.02868679011475));
#26210=CARTESIAN_POINT('Ctrl Pts',(-15.5,13.9197595264192,1.98702012344808));
#26211=CARTESIAN_POINT('Ctrl Pts',(-14.5876477371938,13.9197595264192,1.94535345678141));
#26212=CARTESIAN_POINT('Ctrl Pts',(-14.1314716057906,14.7098797632096,1.90368679011474));
#26213=CARTESIAN_POINT('Ctrl Pts',(-13.6752954743875,15.5,1.86202012344808));
#26214=CARTESIAN_POINT('Ctrl Pts',(-14.1314716057906,16.2901202367904,1.82035345678141));
#26215=CARTESIAN_POINT('Ctrl Pts',(-14.5876477371938,17.0802404735808,1.77868679011474));
#26216=CARTESIAN_POINT('Ctrl Pts',(-15.5,17.0802404735808,1.73702012344807));
#26217=CARTESIAN_POINT('Ctrl Pts',(-16.4123522628062,17.0802404735808,1.69535345678141));
#26218=CARTESIAN_POINT('Ctrl Pts',(-16.8685283942094,16.2901202367904,1.65368679011474));
#26219=CARTESIAN_POINT('Ctrl Pts',(-17.3247045256125,15.5,1.61202012344807));
#26220=CARTESIAN_POINT('Ctrl Pts',(-16.8685283942094,14.7098797632096,1.57035345678141));
#26221=CARTESIAN_POINT('Ctrl Pts',(-16.4123522628062,13.9197595264192,1.52868679011474));
#26222=CARTESIAN_POINT('Ctrl Pts',(-15.5,13.9197595264192,1.48702012344807));
#26223=CARTESIAN_POINT('Ctrl Pts',(-14.5876477371938,13.9197595264192,1.4453534567814));
#26224=CARTESIAN_POINT('Ctrl Pts',(-14.1314716057906,14.7098797632096,1.40368679011474));
#26225=CARTESIAN_POINT('Ctrl Pts',(-13.6752954743875,15.5,1.36202012344807));
#26226=CARTESIAN_POINT('Ctrl Pts',(-14.1314716057906,16.2901202367904,1.3203534567814));
#26227=CARTESIAN_POINT('Ctrl Pts',(-14.5876477371938,17.0802404735808,1.27868679011473));
#26228=CARTESIAN_POINT('Ctrl Pts',(-15.5,17.0802404735808,1.23702012344807));
#26229=CARTESIAN_POINT('Ctrl Pts',(-16.4123522628062,17.0802404735808,1.1953534567814));
#26230=CARTESIAN_POINT('Ctrl Pts',(-16.8685283942094,16.2901202367904,1.15368679011473));
#26231=CARTESIAN_POINT('Ctrl Pts',(-17.3247045256125,15.5,1.11202012344807));
#26232=CARTESIAN_POINT('Ctrl Pts',(-16.8685283942094,14.7098797632096,1.0703534567814));
#26233=CARTESIAN_POINT('Ctrl Pts',(-16.4123522628062,13.9197595264192,1.02868679011473));
#26234=CARTESIAN_POINT('Ctrl Pts',(-15.5,13.9197595264192,0.987020123448065));
#26235=CARTESIAN_POINT('Ctrl Pts',(-14.5876477371938,13.9197595264192,0.945353456781398));
#26236=CARTESIAN_POINT('Ctrl Pts',(-14.1314716057906,14.7098797632096,0.903686790114731));
#26237=CARTESIAN_POINT('Ctrl Pts',(-13.6752954743875,15.5,0.862020123448063));
#26238=CARTESIAN_POINT('Ctrl Pts',(-14.1314716057906,16.2901202367904,0.820353456781396));
#26239=CARTESIAN_POINT('Ctrl Pts',(-14.5876477371938,17.0802404735808,0.778686790114729));
#26240=CARTESIAN_POINT('Ctrl Pts',(-15.5,17.0802404735808,0.737020123448061));
#26241=CARTESIAN_POINT('Ctrl Pts',(-16.4123522628062,17.0802404735808,0.695353456781394));
#26242=CARTESIAN_POINT('Ctrl Pts',(-16.8685283942094,16.2901202367904,0.653686790114727));
#26243=CARTESIAN_POINT('Ctrl Pts',(-17.3247045256125,15.5,0.61202012344806));
#26244=CARTESIAN_POINT('Ctrl Pts',(-16.8685283942094,14.7098797632096,0.570353456781392));
#26245=CARTESIAN_POINT('Ctrl Pts',(-16.4123522628062,13.9197595264192,0.528686790114725));
#26246=CARTESIAN_POINT('Ctrl Pts',(-15.5,13.9197595264192,0.487020123448058));
#26247=CARTESIAN_POINT('Ctrl Pts',(-14.5876477371938,13.9197595264192,0.44535345678139));
#26248=CARTESIAN_POINT('Ctrl Pts',(-14.1314716057906,14.7098797632096,0.403686790114723));
#26249=CARTESIAN_POINT('Ctrl Pts',(-13.6752954743875,15.5,0.362020123448056));
#26250=CARTESIAN_POINT('Ctrl Pts',(-14.1314716057906,16.2901202367904,0.320353456781388));
#26251=CARTESIAN_POINT('Ctrl Pts',(-14.5876477371938,17.0802404735808,0.278686790114721));
#26252=CARTESIAN_POINT('Ctrl Pts',(-15.5,17.0802404735808,0.237020123448054));
#26253=CARTESIAN_POINT('Ctrl Pts',(-16.4123522628062,17.0802404735808,0.195353456781387));
#26254=CARTESIAN_POINT('Ctrl Pts',(-16.8685283942094,16.2901202367904,0.153686790114719));
#26255=CARTESIAN_POINT('Ctrl Pts',(-17.3247045256125,15.5,0.112020123448052));
#26256=CARTESIAN_POINT('Ctrl Pts',(-16.8685283942094,14.7098797632096,0.0703534567813848));
#26257=CARTESIAN_POINT('Ctrl Pts',(-16.4123522628062,13.9197595264192,0.0286867901147175));
#26258=CARTESIAN_POINT('Ctrl Pts',(-15.5,13.9197595264192,-0.0129798765519497));
#26259=CARTESIAN_POINT('Ctrl Pts',(-14.5876477371938,13.9197595264192,-0.0546465432186153));
#26260=CARTESIAN_POINT('Ctrl Pts',(-14.1314716057906,14.7098797632096,-0.0963132098852826));
#26261=CARTESIAN_POINT('Ctrl Pts',(-13.6752954743875,15.5,-0.13797987655195));
#26262=CARTESIAN_POINT('Ctrl Pts',(-14.1314716057906,16.2901202367904,-0.179646543218617));
#26263=CARTESIAN_POINT('Ctrl Pts',(-14.5876477371938,17.0802404735808,-0.221313209885284));
#26264=CARTESIAN_POINT('Ctrl Pts',(-15.5,17.0802404735808,-0.262979876551952));
#26265=CARTESIAN_POINT('Ctrl Pts',(-16.4123522628062,17.0802404735808,-0.304646543218619));
#26266=CARTESIAN_POINT('Ctrl Pts',(-16.8685283942094,16.2901202367904,-0.346313209885286));
#26267=CARTESIAN_POINT('Ctrl Pts',(-17.3247045256125,15.5,-0.387979876551954));
#26268=CARTESIAN_POINT('Ctrl Pts',(-16.8685283942094,14.7098797632096,-0.429646543218621));
#26269=CARTESIAN_POINT('Ctrl Pts',(-16.4123522628062,13.9197595264192,-0.471313209885288));
#26270=CARTESIAN_POINT('Ctrl Pts',(-15.5,13.9197595264192,-0.512979876551955));
#26271=CARTESIAN_POINT('Ctrl Pts',(-14.5876477371938,13.9197595264192,-0.554646543218623));
#26272=CARTESIAN_POINT('Ctrl Pts',(-14.1314716057906,14.7098797632096,-0.59631320988529));
#26273=CARTESIAN_POINT('Ctrl Pts',(-13.6752954743875,15.5,-0.637979876551957));
#26274=CARTESIAN_POINT('Ctrl Pts',(-14.1314716057906,16.2901202367904,-0.679646543218624));
#26275=CARTESIAN_POINT('Ctrl Pts',(-14.5876477371938,17.0802404735808,-0.721313209885292));
#26276=CARTESIAN_POINT('Ctrl Pts',(-15.5,17.0802404735808,-0.762979876551959));
#26277=CARTESIAN_POINT('Ctrl Pts',(-16.4123522628062,17.0802404735808,-0.804646543218627));
#26278=CARTESIAN_POINT('Ctrl Pts',(-16.8685283942094,16.2901202367904,-0.846313209885294));
#26279=CARTESIAN_POINT('Ctrl Pts',(-17.3247045256125,15.5,-0.887979876551961));
#26280=CARTESIAN_POINT('Ctrl Pts',(-16.8685283942094,14.7098797632096,-0.929646543218628));
#26281=CARTESIAN_POINT('Ctrl Pts',(-16.4123522628062,13.9197595264192,-0.971313209885295));
#26282=CARTESIAN_POINT('Ctrl Pts',(-15.5,13.9197595264192,-1.01297987655196));
#26283=CARTESIAN_POINT('Ctrl Pts',(-14.5876477371938,13.9197595264192,-1.05464654321863));
#26284=CARTESIAN_POINT('Ctrl Pts',(-14.1314716057906,14.7098797632096,-1.0963132098853));
#26285=CARTESIAN_POINT('Ctrl Pts',(-13.6752954743875,15.5,-1.13797987655196));
#26286=CARTESIAN_POINT('Ctrl Pts',(-14.1314716057906,16.2901202367904,-1.17964654321863));
#26287=CARTESIAN_POINT('Ctrl Pts',(-14.5876477371938,17.0802404735808,-1.2213132098853));
#26288=CARTESIAN_POINT('Ctrl Pts',(-15.5,17.0802404735808,-1.26297987655196));
#26289=CARTESIAN_POINT('Ctrl Pts',(-16.4123522628062,17.0802404735808,-1.30464654321863));
#26290=CARTESIAN_POINT('Ctrl Pts',(-16.8685283942094,16.2901202367904,-1.3463132098853));
#26291=CARTESIAN_POINT('Ctrl Pts',(-17.3247045256125,15.5,-1.38797987655197));
#26292=CARTESIAN_POINT('Ctrl Pts',(-16.8685283942094,14.7098797632096,-1.42964654321863));
#26293=CARTESIAN_POINT('Ctrl Pts',(-16.4123522628062,13.9197595264192,-1.4713132098853));
#26294=CARTESIAN_POINT('Ctrl Pts',(-15.5,13.9197595264192,-1.51297987655197));
#26295=CARTESIAN_POINT('Ctrl Pts',(-14.5876477371938,13.9197595264192,-1.55464654321864));
#26296=CARTESIAN_POINT('Ctrl Pts',(-14.1314716057906,14.7098797632096,-1.5963132098853));
#26297=CARTESIAN_POINT('Ctrl Pts',(-13.6752954743875,15.5,-1.63797987655197));
#26298=CARTESIAN_POINT('Ctrl Pts',(-14.1314716057906,16.2901202367904,-1.67964654321864));
#26299=CARTESIAN_POINT('Ctrl Pts',(-14.5876477371938,17.0802404735808,-1.7213132098853));
#26300=CARTESIAN_POINT('Ctrl Pts',(-15.5,17.0802404735808,-1.76297987655197));
#26301=CARTESIAN_POINT('Ctrl Pts',(-16.4123522628062,17.0802404735808,-1.80464654321864));
#26302=CARTESIAN_POINT('Ctrl Pts',(-16.8685283942094,16.2901202367904,-1.84631320988531));
#26303=CARTESIAN_POINT('Ctrl Pts',(-17.3247045256125,15.5,-1.88797987655197));
#26304=CARTESIAN_POINT('Ctrl Pts',(-16.8685283942094,14.7098797632096,-1.92964654321864));
#26305=CARTESIAN_POINT('Ctrl Pts',(-16.700583153372,14.4189900731899,-1.94498649173085));
#26306=CARTESIAN_POINT('Ctrl Pts',(-16.4288420454487,14.2215586016756,-1.96260250461286));
#26307=CARTESIAN_POINT('Ctrl Pts',(-15.3465777998745,13.4352476007234,-2.03276185973389));
#26308=CARTESIAN_POINT('Ctrl Pts',(-14.2643135543003,12.6489365997713,-2.10292121485492));
#26309=CARTESIAN_POINT('Ctrl Pts',(-15.5,17.0802404735808,11.1745));
#26310=CARTESIAN_POINT('Ctrl Pts',(-16.4123522628062,17.0802404735808,11.1328333333333));
#26311=CARTESIAN_POINT('Ctrl Pts',(-16.8685283942094,16.2901202367904,11.0911666666667));
#26312=CARTESIAN_POINT('Ctrl Pts',(-17.3247045256125,15.5,11.0495));
#26313=CARTESIAN_POINT('Ctrl Pts',(-16.8685283942094,14.7098797632096,11.0078333333333));
#26314=CARTESIAN_POINT('Ctrl Pts',(-16.4123522628062,13.9197595264192,10.9661666666667));
#26315=CARTESIAN_POINT('Ctrl Pts',(-15.5,13.9197595264192,10.9245));
#26316=CARTESIAN_POINT('Ctrl Pts',(-14.5876477371938,13.9197595264192,10.8828333333333));
#26317=CARTESIAN_POINT('Ctrl Pts',(-14.1314716057906,14.7098797632096,10.8411666666667));
#26318=CARTESIAN_POINT('Ctrl Pts',(-13.6752954743875,15.5,10.7995));
#26319=CARTESIAN_POINT('Ctrl Pts',(-14.1314716057906,16.2901202367904,10.7578333333333));
#26320=CARTESIAN_POINT('Ctrl Pts',(-14.5876477371938,17.0802404735808,10.7161666666667));
#26321=CARTESIAN_POINT('Ctrl Pts',(-15.5,17.0802404735808,10.6745));
#26322=CARTESIAN_POINT('Ctrl Pts',(-16.4123522628062,17.0802404735808,10.6328333333333));
#26323=CARTESIAN_POINT('Ctrl Pts',(-16.8685283942094,16.2901202367904,10.5911666666667));
#26324=CARTESIAN_POINT('Ctrl Pts',(-17.3247045256125,15.5,10.5495));
#26325=CARTESIAN_POINT('Ctrl Pts',(-16.8685283942094,14.7098797632096,10.5078333333333));
#26326=CARTESIAN_POINT('Ctrl Pts',(-16.4123522628062,13.9197595264192,10.4661666666667));
#26327=CARTESIAN_POINT('Ctrl Pts',(-15.5,13.9197595264192,10.4245));
#26328=CARTESIAN_POINT('Ctrl Pts',(-14.5876477371938,13.9197595264192,10.3828333333333));
#26329=CARTESIAN_POINT('Ctrl Pts',(-14.1314716057906,14.7098797632096,10.3411666666667));
#26330=CARTESIAN_POINT('Ctrl Pts',(-13.6752954743875,15.5,10.2995));
#26331=CARTESIAN_POINT('Ctrl Pts',(-14.1314716057906,16.2901202367904,10.2578333333333));
#26332=CARTESIAN_POINT('Ctrl Pts',(-14.5876477371938,17.0802404735808,10.2161666666667));
#26333=CARTESIAN_POINT('Ctrl Pts',(-15.5,17.0802404735808,10.1745));
#26334=CARTESIAN_POINT('Ctrl Pts',(-16.4123522628062,17.0802404735808,10.1328333333333));
#26335=CARTESIAN_POINT('Ctrl Pts',(-16.8685283942094,16.2901202367904,10.0911666666667));
#26336=CARTESIAN_POINT('Ctrl Pts',(-17.3247045256125,15.5,10.0495));
#26337=CARTESIAN_POINT('Ctrl Pts',(-16.8685283942094,14.7098797632096,10.0078333333333));
#26338=CARTESIAN_POINT('Ctrl Pts',(-16.4123522628062,13.9197595264192,9.96616666666665));
#26339=CARTESIAN_POINT('Ctrl Pts',(-15.5,13.9197595264192,9.92449999999998));
#26340=CARTESIAN_POINT('Ctrl Pts',(-14.5876477371938,13.9197595264192,9.88283333333331));
#26341=CARTESIAN_POINT('Ctrl Pts',(-14.1314716057906,14.7098797632096,9.84116666666665));
#26342=CARTESIAN_POINT('Ctrl Pts',(-13.6752954743875,15.5,9.79949999999998));
#26343=CARTESIAN_POINT('Ctrl Pts',(-14.1314716057906,16.2901202367904,9.75783333333331));
#26344=CARTESIAN_POINT('Ctrl Pts',(-14.5876477371938,17.0802404735808,9.71616666666665));
#26345=CARTESIAN_POINT('Ctrl Pts',(-15.5,17.0802404735808,9.67449999999998));
#26346=CARTESIAN_POINT('Ctrl Pts',(-16.4123522628062,17.0802404735808,9.63283333333331));
#26347=CARTESIAN_POINT('Ctrl Pts',(-16.8685283942094,16.2901202367904,9.59116666666664));
#26348=CARTESIAN_POINT('Ctrl Pts',(-17.3247045256125,15.5,9.54949999999998));
#26349=CARTESIAN_POINT('Ctrl Pts',(-16.8685283942094,14.7098797632096,9.50783333333331));
#26350=CARTESIAN_POINT('Ctrl Pts',(-16.4123522628062,13.9197595264192,9.46616666666664));
#26351=CARTESIAN_POINT('Ctrl Pts',(-15.5,13.9197595264192,9.42449999999998));
#26352=CARTESIAN_POINT('Ctrl Pts',(-14.5876477371938,13.9197595264192,9.38283333333331));
#26353=CARTESIAN_POINT('Ctrl Pts',(-14.1314716057906,14.7098797632096,9.34116666666664));
#26354=CARTESIAN_POINT('Ctrl Pts',(-13.6752954743875,15.5,9.29949999999998));
#26355=CARTESIAN_POINT('Ctrl Pts',(-14.1314716057906,16.2901202367904,9.25783333333331));
#26356=CARTESIAN_POINT('Ctrl Pts',(-14.5876477371938,17.0802404735808,9.21616666666664));
#26357=CARTESIAN_POINT('Ctrl Pts',(-15.5,17.0802404735808,9.17449999999997));
#26358=CARTESIAN_POINT('Ctrl Pts',(-16.4123522628062,17.0802404735808,9.13283333333331));
#26359=CARTESIAN_POINT('Ctrl Pts',(-16.8685283942094,16.2901202367904,9.09116666666664));
#26360=CARTESIAN_POINT('Ctrl Pts',(-17.3247045256125,15.5,9.04949999999997));
#26361=CARTESIAN_POINT('Ctrl Pts',(-16.8685283942094,14.7098797632096,9.0078333333333));
#26362=CARTESIAN_POINT('Ctrl Pts',(-16.4123522628062,13.9197595264192,8.96616666666664));
#26363=CARTESIAN_POINT('Ctrl Pts',(-15.5,13.9197595264192,8.92449999999997));
#26364=CARTESIAN_POINT('Ctrl Pts',(-14.5876477371938,13.9197595264192,8.8828333333333));
#26365=CARTESIAN_POINT('Ctrl Pts',(-14.1314716057906,14.7098797632096,8.84116666666664));
#26366=CARTESIAN_POINT('Ctrl Pts',(-13.6752954743875,15.5,8.79949999999997));
#26367=CARTESIAN_POINT('Ctrl Pts',(-14.1314716057906,16.2901202367904,8.7578333333333));
#26368=CARTESIAN_POINT('Ctrl Pts',(-14.5876477371938,17.0802404735808,8.71616666666663));
#26369=CARTESIAN_POINT('Ctrl Pts',(-15.5,17.0802404735808,8.67449999999997));
#26370=CARTESIAN_POINT('Ctrl Pts',(-16.4123522628062,17.0802404735808,8.6328333333333));
#26371=CARTESIAN_POINT('Ctrl Pts',(-16.8685283942094,16.2901202367904,8.59116666666663));
#26372=CARTESIAN_POINT('Ctrl Pts',(-17.3247045256125,15.5,8.54949999999996));
#26373=CARTESIAN_POINT('Ctrl Pts',(-16.8685283942094,14.7098797632096,8.50783333333329));
#26374=CARTESIAN_POINT('Ctrl Pts',(-16.4123522628062,13.9197595264192,8.46616666666663));
#26375=CARTESIAN_POINT('Ctrl Pts',(-15.5,13.9197595264192,8.42449999999996));
#26376=CARTESIAN_POINT('Ctrl Pts',(-14.5876477371938,13.9197595264192,8.3828333333333));
#26377=CARTESIAN_POINT('Ctrl Pts',(-14.1314716057906,14.7098797632096,8.34116666666663));
#26378=CARTESIAN_POINT('Ctrl Pts',(-13.6752954743875,15.5,8.29949999999996));
#26379=CARTESIAN_POINT('Ctrl Pts',(-14.1314716057906,16.2901202367904,8.25783333333329));
#26380=CARTESIAN_POINT('Ctrl Pts',(-14.5876477371938,17.0802404735808,8.21616666666663));
#26381=CARTESIAN_POINT('Ctrl Pts',(-15.5,17.0802404735808,8.17449999999996));
#26382=CARTESIAN_POINT('Ctrl Pts',(-16.4123522628062,17.0802404735808,8.13283333333329));
#26383=CARTESIAN_POINT('Ctrl Pts',(-16.8685283942094,16.2901202367904,8.09116666666663));
#26384=CARTESIAN_POINT('Ctrl Pts',(-17.3247045256125,15.5,8.04949999999996));
#26385=CARTESIAN_POINT('Ctrl Pts',(-16.8685283942094,14.7098797632096,8.00783333333329));
#26386=CARTESIAN_POINT('Ctrl Pts',(-16.4123522628062,13.9197595264192,7.96616666666662));
#26387=CARTESIAN_POINT('Ctrl Pts',(-15.5,13.9197595264192,7.92449999999996));
#26388=CARTESIAN_POINT('Ctrl Pts',(-14.5876477371938,13.9197595264192,7.88283333333329));
#26389=CARTESIAN_POINT('Ctrl Pts',(-14.1314716057906,14.7098797632096,7.84116666666662));
#26390=CARTESIAN_POINT('Ctrl Pts',(-13.6752954743875,15.5,7.79949999999995));
#26391=CARTESIAN_POINT('Ctrl Pts',(-14.1314716057906,16.2901202367904,7.75783333333329));
#26392=CARTESIAN_POINT('Ctrl Pts',(-14.5876477371938,17.0802404735808,7.71616666666662));
#26393=CARTESIAN_POINT('Ctrl Pts',(-15.5,17.0802404735808,7.67449999999995));
#26394=CARTESIAN_POINT('Ctrl Pts',(-16.4123522628062,17.0802404735808,7.63283333333328));
#26395=CARTESIAN_POINT('Ctrl Pts',(-16.8685283942094,16.2901202367904,7.59116666666662));
#26396=CARTESIAN_POINT('Ctrl Pts',(-17.3247045256125,15.5,7.54949999999995));
#26397=CARTESIAN_POINT('Ctrl Pts',(-16.8685283942094,14.7098797632096,7.50783333333328));
#26398=CARTESIAN_POINT('Ctrl Pts',(-16.4123522628062,13.9197595264192,7.46616666666662));
#26399=CARTESIAN_POINT('Ctrl Pts',(-15.5,13.9197595264192,7.42449999999995));
#26400=CARTESIAN_POINT('Ctrl Pts',(-14.5876477371938,13.9197595264192,7.38283333333328));
#26401=CARTESIAN_POINT('Ctrl Pts',(-14.1314716057906,14.7098797632096,7.34116666666661));
#26402=CARTESIAN_POINT('Ctrl Pts',(-13.6752954743875,15.5,7.29949999999995));
#26403=CARTESIAN_POINT('Ctrl Pts',(-14.1314716057906,16.2901202367904,7.25783333333328));
#26404=CARTESIAN_POINT('Ctrl Pts',(-14.5876477371938,17.0802404735808,7.21616666666661));
#26405=CARTESIAN_POINT('Ctrl Pts',(-15.5,17.0802404735808,7.17449999999995));
#26406=CARTESIAN_POINT('Ctrl Pts',(-16.4123522628062,17.0802404735808,7.13283333333328));
#26407=CARTESIAN_POINT('Ctrl Pts',(-16.8685283942094,16.2901202367904,7.09116666666661));
#26408=CARTESIAN_POINT('Ctrl Pts',(-17.3247045256125,15.5,7.04949999999994));
#26409=CARTESIAN_POINT('Ctrl Pts',(-16.8685283942094,14.7098797632096,7.00783333333328));
#26410=CARTESIAN_POINT('Ctrl Pts',(-16.4123522628062,13.9197595264192,6.96616666666661));
#26411=CARTESIAN_POINT('Ctrl Pts',(-15.5,13.9197595264192,6.92449999999994));
#26412=CARTESIAN_POINT('Ctrl Pts',(-14.5876477371938,13.9197595264192,6.88283333333327));
#26413=CARTESIAN_POINT('Ctrl Pts',(-14.1314716057906,14.7098797632096,6.84116666666661));
#26414=CARTESIAN_POINT('Ctrl Pts',(-13.6752954743875,15.5,6.79949999999994));
#26415=CARTESIAN_POINT('Ctrl Pts',(-14.1314716057906,16.2901202367904,6.75783333333327));
#26416=CARTESIAN_POINT('Ctrl Pts',(-14.5876477371938,17.0802404735808,6.71616666666661));
#26417=CARTESIAN_POINT('Ctrl Pts',(-15.5,17.0802404735808,6.67449999999994));
#26418=CARTESIAN_POINT('Ctrl Pts',(-16.4123522628062,17.0802404735808,6.63283333333327));
#26419=CARTESIAN_POINT('Ctrl Pts',(-16.8685283942094,16.2901202367904,6.59116666666661));
#26420=CARTESIAN_POINT('Ctrl Pts',(-17.3247045256125,15.5,6.54949999999994));
#26421=CARTESIAN_POINT('Ctrl Pts',(-16.8685283942094,14.7098797632096,6.50783333333327));
#26422=CARTESIAN_POINT('Ctrl Pts',(-16.4123522628062,13.9197595264192,6.4661666666666));
#26423=CARTESIAN_POINT('Ctrl Pts',(-15.5,13.9197595264192,6.42449999999994));
#26424=CARTESIAN_POINT('Ctrl Pts',(-14.5876477371938,13.9197595264192,6.38283333333327));
#26425=CARTESIAN_POINT('Ctrl Pts',(-14.1314716057906,14.7098797632096,6.3411666666666));
#26426=CARTESIAN_POINT('Ctrl Pts',(-13.6752954743875,15.5,6.29949999999993));
#26427=CARTESIAN_POINT('Ctrl Pts',(-14.1314716057906,16.2901202367904,6.25783333333327));
#26428=CARTESIAN_POINT('Ctrl Pts',(-14.5876477371938,17.0802404735808,6.2161666666666));
#26429=CARTESIAN_POINT('Ctrl Pts',(-15.5,17.0802404735808,6.17449999999993));
#26430=CARTESIAN_POINT('Ctrl Pts',(-16.4123522628062,17.0802404735808,6.13283333333326));
#26431=CARTESIAN_POINT('Ctrl Pts',(-16.8685283942094,16.2901202367904,6.0911666666666));
#26432=CARTESIAN_POINT('Ctrl Pts',(-17.3247045256125,15.5,6.04949999999993));
#26433=CARTESIAN_POINT('Ctrl Pts',(-16.8685283942094,14.7098797632096,6.00783333333326));
#26434=CARTESIAN_POINT('Ctrl Pts',(-16.4123522628062,13.9197595264192,5.9661666666666));
#26435=CARTESIAN_POINT('Ctrl Pts',(-15.5,13.9197595264192,5.92449999999993));
#26436=CARTESIAN_POINT('Ctrl Pts',(-14.5876477371938,13.9197595264192,5.88283333333326));
#26437=CARTESIAN_POINT('Ctrl Pts',(-14.1314716057906,14.7098797632096,5.8411666666666));
#26438=CARTESIAN_POINT('Ctrl Pts',(-13.6752954743875,15.5,5.79949999999993));
#26439=CARTESIAN_POINT('Ctrl Pts',(-14.1314716057906,16.2901202367904,5.75783333333326));
#26440=CARTESIAN_POINT('Ctrl Pts',(-14.5876477371938,17.0802404735808,5.71616666666659));
#26441=CARTESIAN_POINT('Ctrl Pts',(-15.5,17.0802404735808,5.67449999999993));
#26442=CARTESIAN_POINT('Ctrl Pts',(-16.4123522628062,17.0802404735808,5.63283333333326));
#26443=CARTESIAN_POINT('Ctrl Pts',(-16.8685283942094,16.2901202367904,5.59116666666659));
#26444=CARTESIAN_POINT('Ctrl Pts',(-17.3247045256125,15.5,5.54949999999992));
#26445=CARTESIAN_POINT('Ctrl Pts',(-16.8685283942094,14.7098797632096,5.50783333333326));
#26446=CARTESIAN_POINT('Ctrl Pts',(-16.4123522628062,13.9197595264192,5.46616666666659));
#26447=CARTESIAN_POINT('Ctrl Pts',(-15.5,13.9197595264192,5.42449999999992));
#26448=CARTESIAN_POINT('Ctrl Pts',(-14.5876477371938,13.9197595264192,5.38283333333326));
#26449=CARTESIAN_POINT('Ctrl Pts',(-14.1314716057906,14.7098797632096,5.34116666666659));
#26450=CARTESIAN_POINT('Ctrl Pts',(-13.6752954743875,15.5,5.29949999999992));
#26451=CARTESIAN_POINT('Ctrl Pts',(-14.1314716057906,16.2901202367904,5.25783333333325));
#26452=CARTESIAN_POINT('Ctrl Pts',(-14.5876477371938,17.0802404735808,5.21616666666659));
#26453=CARTESIAN_POINT('Ctrl Pts',(-15.5,17.0802404735808,5.17449999999992));
#26454=CARTESIAN_POINT('Ctrl Pts',(-16.4123522628062,17.0802404735808,5.13283333333325));
#26455=CARTESIAN_POINT('Ctrl Pts',(-16.8685283942094,16.2901202367904,5.09116666666658));
#26456=CARTESIAN_POINT('Ctrl Pts',(-17.3247045256125,15.5,5.04949999999992));
#26457=CARTESIAN_POINT('Ctrl Pts',(-16.8685283942094,14.7098797632096,5.00783333333325));
#26458=CARTESIAN_POINT('Ctrl Pts',(-16.4123522628062,13.9197595264192,4.96616666666658));
#26459=CARTESIAN_POINT('Ctrl Pts',(-15.5,13.9197595264192,4.92449999999992));
#26460=CARTESIAN_POINT('Ctrl Pts',(-14.5876477371938,13.9197595264192,4.88283333333325));
#26461=CARTESIAN_POINT('Ctrl Pts',(-14.1314716057906,14.7098797632096,4.84116666666658));
#26462=CARTESIAN_POINT('Ctrl Pts',(-13.6752954743875,15.5,4.79949999999991));
#26463=CARTESIAN_POINT('Ctrl Pts',(-14.1314716057906,16.2901202367904,4.75783333333325));
#26464=CARTESIAN_POINT('Ctrl Pts',(-14.5876477371938,17.0802404735808,4.71616666666658));
#26465=CARTESIAN_POINT('Ctrl Pts',(-15.5,17.0802404735808,4.67449999999991));
#26466=CARTESIAN_POINT('Ctrl Pts',(-16.4123522628062,17.0802404735808,4.63283333333324));
#26467=CARTESIAN_POINT('Ctrl Pts',(-16.8685283942094,16.2901202367904,4.59116666666658));
#26468=CARTESIAN_POINT('Ctrl Pts',(-17.3247045256125,15.5,4.54949999999991));
#26469=CARTESIAN_POINT('Ctrl Pts',(-16.8685283942094,14.7098797632096,4.50783333333324));
#26470=CARTESIAN_POINT('Ctrl Pts',(-16.4123522628062,13.9197595264192,4.46616666666658));
#26471=CARTESIAN_POINT('Ctrl Pts',(-15.5,13.9197595264192,4.42449999999991));
#26472=CARTESIAN_POINT('Ctrl Pts',(-14.5876477371938,13.9197595264192,4.38283333333324));
#26473=CARTESIAN_POINT('Ctrl Pts',(-14.1314716057906,14.7098797632096,4.34116666666657));
#26474=CARTESIAN_POINT('Ctrl Pts',(-13.6752954743875,15.5,4.29949999999991));
#26475=CARTESIAN_POINT('Ctrl Pts',(-14.1314716057906,16.2901202367904,4.25783333333324));
#26476=CARTESIAN_POINT('Ctrl Pts',(-14.5876477371938,17.0802404735808,4.21616666666657));
#26477=CARTESIAN_POINT('Ctrl Pts',(-15.5,17.0802404735808,4.17449999999991));
#26478=CARTESIAN_POINT('Ctrl Pts',(-16.4123522628062,17.0802404735808,4.13283333333324));
#26479=CARTESIAN_POINT('Ctrl Pts',(-16.8685283942094,16.2901202367904,4.09116666666657));
#26480=CARTESIAN_POINT('Ctrl Pts',(-17.3247045256125,15.5,4.0494999999999));
#26481=CARTESIAN_POINT('Ctrl Pts',(-16.8685283942094,14.7098797632096,4.00783333333324));
#26482=CARTESIAN_POINT('Ctrl Pts',(-16.4123522628062,13.9197595264192,3.96616666666657));
#26483=CARTESIAN_POINT('Ctrl Pts',(-15.5,13.9197595264192,3.9244999999999));
#26484=CARTESIAN_POINT('Ctrl Pts',(-14.5876477371938,13.9197595264192,3.88283333333323));
#26485=CARTESIAN_POINT('Ctrl Pts',(-14.1314716057906,14.7098797632096,3.84116666666657));
#26486=CARTESIAN_POINT('Ctrl Pts',(-13.6752954743875,15.5,3.7994999999999));
#26487=CARTESIAN_POINT('Ctrl Pts',(-14.1314716057906,16.2901202367904,3.75783333333323));
#26488=CARTESIAN_POINT('Ctrl Pts',(-14.5876477371938,17.0802404735808,3.71616666666657));
#26489=CARTESIAN_POINT('Ctrl Pts',(-15.5,17.0802404735808,3.6744999999999));
#26490=CARTESIAN_POINT('Ctrl Pts',(-16.4123522628062,17.0802404735808,3.63283333333323));
#26491=CARTESIAN_POINT('Ctrl Pts',(-16.8685283942094,16.2901202367904,3.59116666666656));
#26492=CARTESIAN_POINT('Ctrl Pts',(-17.3247045256125,15.5,3.5494999999999));
#26493=CARTESIAN_POINT('Ctrl Pts',(-16.8685283942094,14.7098797632096,3.50783333333323));
#26494=CARTESIAN_POINT('Ctrl Pts',(-16.4123522628062,13.9197595264192,3.46616666666656));
#26495=CARTESIAN_POINT('Ctrl Pts',(-15.5,13.9197595264192,3.4244999999999));
#26496=CARTESIAN_POINT('Ctrl Pts',(-14.5876477371938,13.9197595264192,3.38283333333323));
#26497=CARTESIAN_POINT('Ctrl Pts',(-14.1314716057906,14.7098797632096,3.34116666666656));
#26498=CARTESIAN_POINT('Ctrl Pts',(-13.6752954743875,15.5,3.29949999999989));
#26499=CARTESIAN_POINT('Ctrl Pts',(-14.1314716057906,16.2901202367904,3.25783333333323));
#26500=CARTESIAN_POINT('Ctrl Pts',(-14.5876477371938,17.0802404735808,3.21616666666656));
#26501=CARTESIAN_POINT('Ctrl Pts',(-15.5,17.0802404735808,3.17449999999989));
#26502=CARTESIAN_POINT('Ctrl Pts',(-16.4123522628062,17.0802404735808,3.13283333333323));
#26503=CARTESIAN_POINT('Ctrl Pts',(-16.8685283942094,16.2901202367904,3.09116666666656));
#26504=CARTESIAN_POINT('Ctrl Pts',(-17.3247045256125,15.5,3.04949999999989));
#26505=CARTESIAN_POINT('Ctrl Pts',(-16.8685283942094,14.7098797632096,3.00783333333322));
#26506=CARTESIAN_POINT('Ctrl Pts',(-16.4123522628062,13.9197595264192,2.96616666666656));
#26507=CARTESIAN_POINT('Ctrl Pts',(-15.5,13.9197595264192,2.92449999999989));
#26508=CARTESIAN_POINT('Ctrl Pts',(-14.5876477371938,13.9197595264192,2.88283333333322));
#26509=CARTESIAN_POINT('Ctrl Pts',(-14.1314716057906,14.7098797632096,2.84116666666655));
#26510=CARTESIAN_POINT('Ctrl Pts',(-13.6752954743875,15.5,2.79949999999989));
#26511=CARTESIAN_POINT('Ctrl Pts',(-14.1314716057906,16.2901202367904,2.75783333333322));
#26512=CARTESIAN_POINT('Ctrl Pts',(-14.5876477371938,17.0802404735808,2.71616666666655));
#26513=CARTESIAN_POINT('Ctrl Pts',(-15.5,17.0802404735808,2.67449999999989));
#26514=CARTESIAN_POINT('Ctrl Pts',(-16.4123522628062,17.0802404735808,2.63283333333322));
#26515=CARTESIAN_POINT('Ctrl Pts',(-16.8685283942094,16.2901202367904,2.59116666666655));
#26516=CARTESIAN_POINT('Ctrl Pts',(-17.3247045256125,15.5,2.54949999999988));
#26517=CARTESIAN_POINT('Ctrl Pts',(-16.8685283942094,14.7098797632096,2.50783333333322));
#26518=CARTESIAN_POINT('Ctrl Pts',(-16.4123522628062,13.9197595264192,2.46616666666655));
#26519=CARTESIAN_POINT('Ctrl Pts',(-15.5,13.9197595264192,2.42449999999988));
#26520=CARTESIAN_POINT('Ctrl Pts',(-14.5876477371938,13.9197595264192,2.38283333333321));
#26521=CARTESIAN_POINT('Ctrl Pts',(-14.1314716057906,14.7098797632096,2.34116666666655));
#26522=CARTESIAN_POINT('Ctrl Pts',(-13.6752954743875,15.5,2.29949999999988));
#26523=CARTESIAN_POINT('Ctrl Pts',(-14.1314716057906,16.2901202367904,2.25783333333321));
#26524=CARTESIAN_POINT('Ctrl Pts',(-14.5876477371938,17.0802404735808,2.21616666666655));
#26525=CARTESIAN_POINT('Ctrl Pts',(-15.5,17.0802404735808,2.17449999999988));
#26526=CARTESIAN_POINT('Ctrl Pts',(-16.4123522628062,17.0802404735808,2.13283333333321));
#26527=CARTESIAN_POINT('Ctrl Pts',(-16.8685283942094,16.2901202367904,2.09116666666655));
#26528=CARTESIAN_POINT('Ctrl Pts',(-17.3247045256125,15.5,2.04949999999988));
#26529=CARTESIAN_POINT('Ctrl Pts',(-16.8685283942094,14.7098797632096,2.00783333333321));
#26530=CARTESIAN_POINT('Ctrl Pts',(-16.4123522628062,13.9197595264192,1.96616666666654));
#26531=CARTESIAN_POINT('Ctrl Pts',(-15.5,13.9197595264192,1.92449999999988));
#26532=CARTESIAN_POINT('Ctrl Pts',(-14.5876477371938,13.9197595264192,1.88283333333321));
#26533=CARTESIAN_POINT('Ctrl Pts',(-14.1314716057906,14.7098797632096,1.84116666666654));
#26534=CARTESIAN_POINT('Ctrl Pts',(-13.6752954743875,15.5,1.79949999999987));
#26535=CARTESIAN_POINT('Ctrl Pts',(-14.1314716057906,16.2901202367904,1.75783333333321));
#26536=CARTESIAN_POINT('Ctrl Pts',(-14.5876477371938,17.0802404735808,1.71616666666654));
#26537=CARTESIAN_POINT('Ctrl Pts',(-15.5,17.0802404735808,1.67449999999987));
#26538=CARTESIAN_POINT('Ctrl Pts',(-16.4123522628062,17.0802404735808,1.63283333333321));
#26539=CARTESIAN_POINT('Ctrl Pts',(-16.8685283942094,16.2901202367904,1.59116666666654));
#26540=CARTESIAN_POINT('Ctrl Pts',(-17.3247045256125,15.5,1.54949999999987));
#26541=CARTESIAN_POINT('Ctrl Pts',(-16.8685283942094,14.7098797632096,1.5078333333332));
#26542=CARTESIAN_POINT('Ctrl Pts',(-16.4123522628062,13.9197595264192,1.46616666666654));
#26543=CARTESIAN_POINT('Ctrl Pts',(-15.5,13.9197595264192,1.42449999999987));
#26544=CARTESIAN_POINT('Ctrl Pts',(-14.5876477371938,13.9197595264192,1.3828333333332));
#26545=CARTESIAN_POINT('Ctrl Pts',(-14.1314716057906,14.7098797632096,1.34116666666653));
#26546=CARTESIAN_POINT('Ctrl Pts',(-13.6752954743875,15.5,1.29949999999987));
#26547=CARTESIAN_POINT('Ctrl Pts',(-14.1314716057906,16.2901202367904,1.2578333333332));
#26548=CARTESIAN_POINT('Ctrl Pts',(-14.5876477371938,17.0802404735808,1.21616666666653));
#26549=CARTESIAN_POINT('Ctrl Pts',(-15.5,17.0802404735808,1.17449999999986));
#26550=CARTESIAN_POINT('Ctrl Pts',(-16.4123522628062,17.0802404735808,1.1328333333332));
#26551=CARTESIAN_POINT('Ctrl Pts',(-16.8685283942094,16.2901202367904,1.09116666666653));
#26552=CARTESIAN_POINT('Ctrl Pts',(-17.3247045256125,15.5,1.04949999999986));
#26553=CARTESIAN_POINT('Ctrl Pts',(-16.8685283942094,14.7098797632096,1.0078333333332));
#26554=CARTESIAN_POINT('Ctrl Pts',(-16.4123522628062,13.9197595264192,0.96616666666653));
#26555=CARTESIAN_POINT('Ctrl Pts',(-15.5,13.9197595264192,0.924499999999863));
#26556=CARTESIAN_POINT('Ctrl Pts',(-14.5876477371938,13.9197595264192,0.882833333333196));
#26557=CARTESIAN_POINT('Ctrl Pts',(-14.1314716057906,14.7098797632096,0.841166666666529));
#26558=CARTESIAN_POINT('Ctrl Pts',(-13.6752954743875,15.5,0.799499999999861));
#26559=CARTESIAN_POINT('Ctrl Pts',(-14.1314716057906,16.2901202367904,0.757833333333194));
#26560=CARTESIAN_POINT('Ctrl Pts',(-14.5876477371938,17.0802404735808,0.716166666666527));
#26561=CARTESIAN_POINT('Ctrl Pts',(-15.5,17.0802404735808,0.674499999999859));
#26562=CARTESIAN_POINT('Ctrl Pts',(-16.4123522628062,17.0802404735808,0.632833333333192));
#26563=CARTESIAN_POINT('Ctrl Pts',(-16.8685283942094,16.2901202367904,0.591166666666525));
#26564=CARTESIAN_POINT('Ctrl Pts',(-17.3247045256125,15.5,0.549499999999857));
#26565=CARTESIAN_POINT('Ctrl Pts',(-16.8685283942094,14.7098797632096,0.50783333333319));
#26566=CARTESIAN_POINT('Ctrl Pts',(-16.4123522628062,13.9197595264192,0.466166666666523));
#26567=CARTESIAN_POINT('Ctrl Pts',(-15.5,13.9197595264192,0.424499999999856));
#26568=CARTESIAN_POINT('Ctrl Pts',(-14.5876477371938,13.9197595264192,0.382833333333188));
#26569=CARTESIAN_POINT('Ctrl Pts',(-14.1314716057906,14.7098797632096,0.341166666666521));
#26570=CARTESIAN_POINT('Ctrl Pts',(-13.6752954743875,15.5,0.299499999999854));
#26571=CARTESIAN_POINT('Ctrl Pts',(-14.1314716057906,16.2901202367904,0.257833333333186));
#26572=CARTESIAN_POINT('Ctrl Pts',(-14.5876477371938,17.0802404735808,0.216166666666519));
#26573=CARTESIAN_POINT('Ctrl Pts',(-15.5,17.0802404735808,0.174499999999852));
#26574=CARTESIAN_POINT('Ctrl Pts',(-16.4123522628062,17.0802404735808,0.132833333333185));
#26575=CARTESIAN_POINT('Ctrl Pts',(-16.8685283942094,16.2901202367904,0.0911666666665173));
#26576=CARTESIAN_POINT('Ctrl Pts',(-17.3247045256125,15.5,0.04949999999985));
#26577=CARTESIAN_POINT('Ctrl Pts',(-16.8685283942094,14.7098797632096,0.00783333333318273));
#26578=CARTESIAN_POINT('Ctrl Pts',(-16.4123522628062,13.9197595264192,-0.0338333333334846));
#26579=CARTESIAN_POINT('Ctrl Pts',(-15.5,13.9197595264192,-0.0755000000001518));
#26580=CARTESIAN_POINT('Ctrl Pts',(-14.5876477371938,13.9197595264192,-0.117166666666817));
#26581=CARTESIAN_POINT('Ctrl Pts',(-14.1314716057906,14.7098797632096,-0.158833333333485));
#26582=CARTESIAN_POINT('Ctrl Pts',(-13.6752954743875,15.5,-0.200500000000152));
#26583=CARTESIAN_POINT('Ctrl Pts',(-14.1314716057906,16.2901202367904,-0.242166666666819));
#26584=CARTESIAN_POINT('Ctrl Pts',(-14.5876477371938,17.0802404735808,-0.283833333333486));
#26585=CARTESIAN_POINT('Ctrl Pts',(-15.5,17.0802404735808,-0.325500000000154));
#26586=CARTESIAN_POINT('Ctrl Pts',(-16.4123522628062,17.0802404735808,-0.367166666666821));
#26587=CARTESIAN_POINT('Ctrl Pts',(-16.8685283942094,16.2901202367904,-0.408833333333488));
#26588=CARTESIAN_POINT('Ctrl Pts',(-17.3247045256125,15.5,-0.450500000000156));
#26589=CARTESIAN_POINT('Ctrl Pts',(-16.8685283942094,14.7098797632096,-0.492166666666823));
#26590=CARTESIAN_POINT('Ctrl Pts',(-16.4123522628062,13.9197595264192,-0.53383333333349));
#26591=CARTESIAN_POINT('Ctrl Pts',(-15.5,13.9197595264192,-0.575500000000157));
#26592=CARTESIAN_POINT('Ctrl Pts',(-14.5876477371938,13.9197595264192,-0.617166666666825));
#26593=CARTESIAN_POINT('Ctrl Pts',(-14.1314716057906,14.7098797632096,-0.658833333333492));
#26594=CARTESIAN_POINT('Ctrl Pts',(-13.6752954743875,15.5,-0.700500000000159));
#26595=CARTESIAN_POINT('Ctrl Pts',(-14.1314716057906,16.2901202367904,-0.742166666666827));
#26596=CARTESIAN_POINT('Ctrl Pts',(-14.5876477371938,17.0802404735808,-0.783833333333494));
#26597=CARTESIAN_POINT('Ctrl Pts',(-15.5,17.0802404735808,-0.825500000000161));
#26598=CARTESIAN_POINT('Ctrl Pts',(-16.4123522628062,17.0802404735808,-0.867166666666829));
#26599=CARTESIAN_POINT('Ctrl Pts',(-16.8685283942094,16.2901202367904,-0.908833333333496));
#26600=CARTESIAN_POINT('Ctrl Pts',(-17.3247045256125,15.5,-0.950500000000163));
#26601=CARTESIAN_POINT('Ctrl Pts',(-16.8685283942094,14.7098797632096,-0.99216666666683));
#26602=CARTESIAN_POINT('Ctrl Pts',(-16.4123522628062,13.9197595264192,-1.0338333333335));
#26603=CARTESIAN_POINT('Ctrl Pts',(-15.5,13.9197595264192,-1.07550000000016));
#26604=CARTESIAN_POINT('Ctrl Pts',(-14.5876477371938,13.9197595264192,-1.11716666666683));
#26605=CARTESIAN_POINT('Ctrl Pts',(-14.1314716057906,14.7098797632096,-1.1588333333335));
#26606=CARTESIAN_POINT('Ctrl Pts',(-13.6752954743875,15.5,-1.20050000000017));
#26607=CARTESIAN_POINT('Ctrl Pts',(-14.1314716057906,16.2901202367904,-1.24216666666683));
#26608=CARTESIAN_POINT('Ctrl Pts',(-14.5876477371938,17.0802404735808,-1.2838333333335));
#26609=CARTESIAN_POINT('Ctrl Pts',(-15.5,17.0802404735808,-1.32550000000017));
#26610=CARTESIAN_POINT('Ctrl Pts',(-16.4123522628062,17.0802404735808,-1.36716666666683));
#26611=CARTESIAN_POINT('Ctrl Pts',(-16.8685283942094,16.2901202367904,-1.4088333333335));
#26612=CARTESIAN_POINT('Ctrl Pts',(-17.3247045256125,15.5,-1.45050000000017));
#26613=CARTESIAN_POINT('Ctrl Pts',(-16.8685283942094,14.7098797632096,-1.49216666666684));
#26614=CARTESIAN_POINT('Ctrl Pts',(-16.4123522628062,13.9197595264192,-1.5338333333335));
#26615=CARTESIAN_POINT('Ctrl Pts',(-15.5,13.9197595264192,-1.57550000000017));
#26616=CARTESIAN_POINT('Ctrl Pts',(-14.5876477371938,13.9197595264192,-1.61716666666684));
#26617=CARTESIAN_POINT('Ctrl Pts',(-14.1314716057906,14.7098797632096,-1.65883333333351));
#26618=CARTESIAN_POINT('Ctrl Pts',(-13.6752954743875,15.5,-1.70050000000017));
#26619=CARTESIAN_POINT('Ctrl Pts',(-14.1314716057906,16.2901202367904,-1.74216666666684));
#26620=CARTESIAN_POINT('Ctrl Pts',(-14.5876477371938,17.0802404735808,-1.78383333333351));
#26621=CARTESIAN_POINT('Ctrl Pts',(-15.5,17.0802404735808,-1.82550000000017));
#26622=CARTESIAN_POINT('Ctrl Pts',(-16.4123522628062,17.0802404735808,-1.86716666666684));
#26623=CARTESIAN_POINT('Ctrl Pts',(-16.8685283942094,16.2901202367904,-1.90883333333351));
#26624=CARTESIAN_POINT('Ctrl Pts',(-17.3247045256125,15.5,-1.95050000000018));
#26625=CARTESIAN_POINT('Ctrl Pts',(-16.8685283942094,14.7098797632096,-1.99216666666684));
#26626=CARTESIAN_POINT('Ctrl Pts',(-16.700583153372,14.4189900731899,-2.00750661517905));
#26627=CARTESIAN_POINT('Ctrl Pts',(-16.4288420454487,14.2215586016756,-2.02512262806106));
#26628=CARTESIAN_POINT('Ctrl Pts',(-15.3465777998745,13.4352476007234,-2.09528198318209));
#26629=CARTESIAN_POINT('Ctrl Pts',(-14.2643135543003,12.6489365997713,-2.16544133830312));
#26630=CARTESIAN_POINT('Origin',(0.,0.,1.3858));
#26631=CARTESIAN_POINT('',(16.96,21.2,1.3858));
#26632=CARTESIAN_POINT('',(-16.96,21.2,1.3858));
#26633=CARTESIAN_POINT('',(-21.2,21.2,1.3858));
#26634=CARTESIAN_POINT('',(21.2,16.96,1.3858));
#26635=CARTESIAN_POINT('',(16.96,21.2,1.3858));
#26636=CARTESIAN_POINT('',(21.2,-16.96,1.3858));
#26637=CARTESIAN_POINT('',(21.2,21.2,1.3858));
#26638=CARTESIAN_POINT('',(16.96,-21.2,1.3858));
#26639=CARTESIAN_POINT('',(16.96,-21.2,1.3858));
#26640=CARTESIAN_POINT('',(-16.96,-21.2,1.3858));
#26641=CARTESIAN_POINT('',(-21.2,-21.2,1.3858));
#26642=CARTESIAN_POINT('',(-21.2,-16.96,1.3858));
#26643=CARTESIAN_POINT('',(-16.96,-21.2,1.3858));
#26644=CARTESIAN_POINT('',(-21.2,16.96,1.3858));
#26645=CARTESIAN_POINT('',(-21.2,21.2,1.3858));
#26646=CARTESIAN_POINT('',(-16.96,21.2,1.3858));
#26647=CARTESIAN_POINT('Origin',(-15.6430062215132,-15.5080107655887,1.38580563032454));
#26648=CARTESIAN_POINT('Origin',(-15.4374167911874,-15.6296099418937,1.38577762513339));
#26649=CARTESIAN_POINT('Origin',(15.508010765588,-15.643006221513,1.38580563032419));
#26650=CARTESIAN_POINT('Origin',(15.6296099418937,-15.4374167911875,1.38577762513336));
#26651=CARTESIAN_POINT('Origin',(15.6430062215131,15.5080107655888,1.38580563032457));
#26652=CARTESIAN_POINT('Origin',(15.4374167911878,15.6296099418941,1.38577762513333));
#26653=CARTESIAN_POINT('Ctrl Pts',(17.0802317716411,15.5000000000002,11.1745050240672));
#26654=CARTESIAN_POINT('Ctrl Pts',(17.0802317716411,16.4123472387392,11.1328383574005));
#26655=CARTESIAN_POINT('Ctrl Pts',(16.2901158858204,16.8685208581088,11.0911716907338));
#26656=CARTESIAN_POINT('Ctrl Pts',(15.4999999999998,17.3246944774783,11.0495050240672));
#26657=CARTESIAN_POINT('Ctrl Pts',(14.7098841141792,16.8685208581088,11.0078383574005));
#26658=CARTESIAN_POINT('Ctrl Pts',(13.9197682283586,16.4123472387392,10.9661716907338));
#26659=CARTESIAN_POINT('Ctrl Pts',(13.9197682283586,15.5000000000001,10.9245050240672));
#26660=CARTESIAN_POINT('Ctrl Pts',(13.9197682283586,14.5876527612611,10.8828383574005));
#26661=CARTESIAN_POINT('Ctrl Pts',(14.7098841141792,14.1314791418916,10.8411716907338));
#26662=CARTESIAN_POINT('Ctrl Pts',(15.4999999999999,13.675305522522,10.7995050240672));
#26663=CARTESIAN_POINT('Ctrl Pts',(16.2901158858205,14.1314791418916,10.7578383574005));
#26664=CARTESIAN_POINT('Ctrl Pts',(17.0802317716411,14.5876527612611,10.7161716907338));
#26665=CARTESIAN_POINT('Ctrl Pts',(17.0802317716411,15.5000000000002,10.6745050240672));
#26666=CARTESIAN_POINT('Ctrl Pts',(17.0802317716411,16.4123472387392,10.6328383574005));
#26667=CARTESIAN_POINT('Ctrl Pts',(16.2901158858204,16.8685208581088,10.5911716907338));
#26668=CARTESIAN_POINT('Ctrl Pts',(15.4999999999998,17.3246944774783,10.5495050240672));
#26669=CARTESIAN_POINT('Ctrl Pts',(14.7098841141792,16.8685208581088,10.5078383574005));
#26670=CARTESIAN_POINT('Ctrl Pts',(13.9197682283586,16.4123472387392,10.4661716907338));
#26671=CARTESIAN_POINT('Ctrl Pts',(13.9197682283586,15.5000000000001,10.4245050240672));
#26672=CARTESIAN_POINT('Ctrl Pts',(13.9197682283586,14.5876527612611,10.3828383574005));
#26673=CARTESIAN_POINT('Ctrl Pts',(14.7098841141792,14.1314791418916,10.3411716907338));
#26674=CARTESIAN_POINT('Ctrl Pts',(15.4999999999999,13.675305522522,10.2995050240672));
#26675=CARTESIAN_POINT('Ctrl Pts',(16.2901158858205,14.1314791418916,10.2578383574005));
#26676=CARTESIAN_POINT('Ctrl Pts',(17.0802317716411,14.5876527612611,10.2161716907338));
#26677=CARTESIAN_POINT('Ctrl Pts',(17.0802317716411,15.5000000000002,10.1745050240672));
#26678=CARTESIAN_POINT('Ctrl Pts',(17.0802317716411,16.4123472387392,10.1328383574005));
#26679=CARTESIAN_POINT('Ctrl Pts',(16.2901158858204,16.8685208581088,10.0911716907338));
#26680=CARTESIAN_POINT('Ctrl Pts',(15.4999999999998,17.3246944774783,10.0495050240672));
#26681=CARTESIAN_POINT('Ctrl Pts',(14.7098841141792,16.8685208581088,10.0078383574005));
#26682=CARTESIAN_POINT('Ctrl Pts',(13.9197682283586,16.4123472387392,9.96617169073382));
#26683=CARTESIAN_POINT('Ctrl Pts',(13.9197682283586,15.5000000000001,9.92450502406715));
#26684=CARTESIAN_POINT('Ctrl Pts',(13.9197682283586,14.5876527612611,9.88283835740048));
#26685=CARTESIAN_POINT('Ctrl Pts',(14.7098841141792,14.1314791418916,9.84117169073382));
#26686=CARTESIAN_POINT('Ctrl Pts',(15.4999999999999,13.675305522522,9.79950502406715));
#26687=CARTESIAN_POINT('Ctrl Pts',(16.2901158858205,14.1314791418916,9.75783835740048));
#26688=CARTESIAN_POINT('Ctrl Pts',(17.0802317716411,14.5876527612611,9.71617169073381));
#26689=CARTESIAN_POINT('Ctrl Pts',(17.0802317716411,15.5000000000002,9.67450502406715));
#26690=CARTESIAN_POINT('Ctrl Pts',(17.0802317716411,16.4123472387392,9.63283835740048));
#26691=CARTESIAN_POINT('Ctrl Pts',(16.2901158858204,16.8685208581088,9.59117169073381));
#26692=CARTESIAN_POINT('Ctrl Pts',(15.4999999999998,17.3246944774783,9.54950502406714));
#26693=CARTESIAN_POINT('Ctrl Pts',(14.7098841141792,16.8685208581088,9.50783835740048));
#26694=CARTESIAN_POINT('Ctrl Pts',(13.9197682283586,16.4123472387392,9.46617169073381));
#26695=CARTESIAN_POINT('Ctrl Pts',(13.9197682283586,15.5000000000001,9.42450502406714));
#26696=CARTESIAN_POINT('Ctrl Pts',(13.9197682283586,14.5876527612611,9.38283835740048));
#26697=CARTESIAN_POINT('Ctrl Pts',(14.7098841141792,14.1314791418916,9.34117169073381));
#26698=CARTESIAN_POINT('Ctrl Pts',(15.4999999999999,13.675305522522,9.29950502406714));
#26699=CARTESIAN_POINT('Ctrl Pts',(16.2901158858205,14.1314791418916,9.25783835740048));
#26700=CARTESIAN_POINT('Ctrl Pts',(17.0802317716411,14.5876527612611,9.21617169073381));
#26701=CARTESIAN_POINT('Ctrl Pts',(17.0802317716411,15.5000000000002,9.17450502406714));
#26702=CARTESIAN_POINT('Ctrl Pts',(17.0802317716411,16.4123472387392,9.13283835740048));
#26703=CARTESIAN_POINT('Ctrl Pts',(16.2901158858204,16.8685208581088,9.09117169073381));
#26704=CARTESIAN_POINT('Ctrl Pts',(15.4999999999998,17.3246944774783,9.04950502406714));
#26705=CARTESIAN_POINT('Ctrl Pts',(14.7098841141792,16.8685208581088,9.00783835740047));
#26706=CARTESIAN_POINT('Ctrl Pts',(13.9197682283586,16.4123472387392,8.9661716907338));
#26707=CARTESIAN_POINT('Ctrl Pts',(13.9197682283586,15.5000000000001,8.92450502406714));
#26708=CARTESIAN_POINT('Ctrl Pts',(13.9197682283586,14.5876527612611,8.88283835740047));
#26709=CARTESIAN_POINT('Ctrl Pts',(14.7098841141792,14.1314791418916,8.8411716907338));
#26710=CARTESIAN_POINT('Ctrl Pts',(15.4999999999999,13.675305522522,8.79950502406713));
#26711=CARTESIAN_POINT('Ctrl Pts',(16.2901158858205,14.1314791418916,8.75783835740047));
#26712=CARTESIAN_POINT('Ctrl Pts',(17.0802317716411,14.5876527612611,8.7161716907338));
#26713=CARTESIAN_POINT('Ctrl Pts',(17.0802317716411,15.5000000000002,8.67450502406713));
#26714=CARTESIAN_POINT('Ctrl Pts',(17.0802317716411,16.4123472387392,8.63283835740047));
#26715=CARTESIAN_POINT('Ctrl Pts',(16.2901158858204,16.8685208581088,8.5911716907338));
#26716=CARTESIAN_POINT('Ctrl Pts',(15.4999999999998,17.3246944774783,8.54950502406713));
#26717=CARTESIAN_POINT('Ctrl Pts',(14.7098841141792,16.8685208581088,8.50783835740046));
#26718=CARTESIAN_POINT('Ctrl Pts',(13.9197682283586,16.4123472387392,8.4661716907338));
#26719=CARTESIAN_POINT('Ctrl Pts',(13.9197682283586,15.5000000000001,8.42450502406713));
#26720=CARTESIAN_POINT('Ctrl Pts',(13.9197682283586,14.5876527612611,8.38283835740046));
#26721=CARTESIAN_POINT('Ctrl Pts',(14.7098841141792,14.1314791418916,8.3411716907338));
#26722=CARTESIAN_POINT('Ctrl Pts',(15.4999999999999,13.675305522522,8.29950502406713));
#26723=CARTESIAN_POINT('Ctrl Pts',(16.2901158858205,14.1314791418916,8.25783835740046));
#26724=CARTESIAN_POINT('Ctrl Pts',(17.0802317716411,14.5876527612611,8.21617169073379));
#26725=CARTESIAN_POINT('Ctrl Pts',(17.0802317716411,15.5000000000002,8.17450502406713));
#26726=CARTESIAN_POINT('Ctrl Pts',(17.0802317716411,16.4123472387392,8.13283835740046));
#26727=CARTESIAN_POINT('Ctrl Pts',(16.2901158858204,16.8685208581088,8.09117169073379));
#26728=CARTESIAN_POINT('Ctrl Pts',(15.4999999999998,17.3246944774783,8.04950502406713));
#26729=CARTESIAN_POINT('Ctrl Pts',(14.7098841141792,16.8685208581088,8.00783835740046));
#26730=CARTESIAN_POINT('Ctrl Pts',(13.9197682283586,16.4123472387392,7.96617169073379));
#26731=CARTESIAN_POINT('Ctrl Pts',(13.9197682283586,15.5000000000001,7.92450502406712));
#26732=CARTESIAN_POINT('Ctrl Pts',(13.9197682283586,14.5876527612611,7.88283835740046));
#26733=CARTESIAN_POINT('Ctrl Pts',(14.7098841141792,14.1314791418916,7.84117169073379));
#26734=CARTESIAN_POINT('Ctrl Pts',(15.4999999999999,13.675305522522,7.79950502406712));
#26735=CARTESIAN_POINT('Ctrl Pts',(16.2901158858205,14.1314791418916,7.75783835740046));
#26736=CARTESIAN_POINT('Ctrl Pts',(17.0802317716411,14.5876527612611,7.71617169073379));
#26737=CARTESIAN_POINT('Ctrl Pts',(17.0802317716411,15.5000000000002,7.67450502406712));
#26738=CARTESIAN_POINT('Ctrl Pts',(17.0802317716411,16.4123472387392,7.63283835740045));
#26739=CARTESIAN_POINT('Ctrl Pts',(16.2901158858204,16.8685208581088,7.59117169073379));
#26740=CARTESIAN_POINT('Ctrl Pts',(15.4999999999998,17.3246944774783,7.54950502406712));
#26741=CARTESIAN_POINT('Ctrl Pts',(14.7098841141792,16.8685208581088,7.50783835740045));
#26742=CARTESIAN_POINT('Ctrl Pts',(13.9197682283586,16.4123472387392,7.46617169073379));
#26743=CARTESIAN_POINT('Ctrl Pts',(13.9197682283586,15.5000000000001,7.42450502406712));
#26744=CARTESIAN_POINT('Ctrl Pts',(13.9197682283586,14.5876527612611,7.38283835740045));
#26745=CARTESIAN_POINT('Ctrl Pts',(14.7098841141792,14.1314791418916,7.34117169073378));
#26746=CARTESIAN_POINT('Ctrl Pts',(15.4999999999999,13.675305522522,7.29950502406711));
#26747=CARTESIAN_POINT('Ctrl Pts',(16.2901158858205,14.1314791418916,7.25783835740045));
#26748=CARTESIAN_POINT('Ctrl Pts',(17.0802317716411,14.5876527612611,7.21617169073378));
#26749=CARTESIAN_POINT('Ctrl Pts',(17.0802317716411,15.5000000000002,7.17450502406711));
#26750=CARTESIAN_POINT('Ctrl Pts',(17.0802317716411,16.4123472387392,7.13283835740045));
#26751=CARTESIAN_POINT('Ctrl Pts',(16.2901158858204,16.8685208581088,7.09117169073378));
#26752=CARTESIAN_POINT('Ctrl Pts',(15.4999999999998,17.3246944774783,7.04950502406711));
#26753=CARTESIAN_POINT('Ctrl Pts',(14.7098841141792,16.8685208581088,7.00783835740045));
#26754=CARTESIAN_POINT('Ctrl Pts',(13.9197682283586,16.4123472387392,6.96617169073378));
#26755=CARTESIAN_POINT('Ctrl Pts',(13.9197682283586,15.5000000000001,6.92450502406711));
#26756=CARTESIAN_POINT('Ctrl Pts',(13.9197682283586,14.5876527612611,6.88283835740044));
#26757=CARTESIAN_POINT('Ctrl Pts',(14.7098841141792,14.1314791418916,6.84117169073378));
#26758=CARTESIAN_POINT('Ctrl Pts',(15.4999999999999,13.675305522522,6.79950502406711));
#26759=CARTESIAN_POINT('Ctrl Pts',(16.2901158858205,14.1314791418916,6.75783835740044));
#26760=CARTESIAN_POINT('Ctrl Pts',(17.0802317716411,14.5876527612611,6.71617169073377));
#26761=CARTESIAN_POINT('Ctrl Pts',(17.0802317716411,15.5000000000002,6.67450502406711));
#26762=CARTESIAN_POINT('Ctrl Pts',(17.0802317716411,16.4123472387392,6.63283835740044));
#26763=CARTESIAN_POINT('Ctrl Pts',(16.2901158858204,16.8685208581088,6.59117169073377));
#26764=CARTESIAN_POINT('Ctrl Pts',(15.4999999999998,17.3246944774783,6.54950502406711));
#26765=CARTESIAN_POINT('Ctrl Pts',(14.7098841141792,16.8685208581088,6.50783835740044));
#26766=CARTESIAN_POINT('Ctrl Pts',(13.9197682283586,16.4123472387392,6.46617169073377));
#26767=CARTESIAN_POINT('Ctrl Pts',(13.9197682283586,15.5000000000001,6.4245050240671));
#26768=CARTESIAN_POINT('Ctrl Pts',(13.9197682283586,14.5876527612611,6.38283835740044));
#26769=CARTESIAN_POINT('Ctrl Pts',(14.7098841141792,14.1314791418916,6.34117169073377));
#26770=CARTESIAN_POINT('Ctrl Pts',(15.4999999999999,13.675305522522,6.2995050240671));
#26771=CARTESIAN_POINT('Ctrl Pts',(16.2901158858205,14.1314791418916,6.25783835740044));
#26772=CARTESIAN_POINT('Ctrl Pts',(17.0802317716411,14.5876527612611,6.21617169073377));
#26773=CARTESIAN_POINT('Ctrl Pts',(17.0802317716411,15.5000000000002,6.1745050240671));
#26774=CARTESIAN_POINT('Ctrl Pts',(17.0802317716411,16.4123472387392,6.13283835740043));
#26775=CARTESIAN_POINT('Ctrl Pts',(16.2901158858204,16.8685208581088,6.09117169073377));
#26776=CARTESIAN_POINT('Ctrl Pts',(15.4999999999998,17.3246944774783,6.0495050240671));
#26777=CARTESIAN_POINT('Ctrl Pts',(14.7098841141792,16.8685208581088,6.00783835740043));
#26778=CARTESIAN_POINT('Ctrl Pts',(13.9197682283586,16.4123472387392,5.96617169073376));
#26779=CARTESIAN_POINT('Ctrl Pts',(13.9197682283586,15.5000000000001,5.9245050240671));
#26780=CARTESIAN_POINT('Ctrl Pts',(13.9197682283586,14.5876527612611,5.88283835740043));
#26781=CARTESIAN_POINT('Ctrl Pts',(14.7098841141792,14.1314791418916,5.84117169073376));
#26782=CARTESIAN_POINT('Ctrl Pts',(15.4999999999999,13.675305522522,5.79950502406709));
#26783=CARTESIAN_POINT('Ctrl Pts',(16.2901158858205,14.1314791418916,5.75783835740043));
#26784=CARTESIAN_POINT('Ctrl Pts',(17.0802317716411,14.5876527612611,5.71617169073376));
#26785=CARTESIAN_POINT('Ctrl Pts',(17.0802317716411,15.5000000000002,5.67450502406709));
#26786=CARTESIAN_POINT('Ctrl Pts',(17.0802317716411,16.4123472387392,5.63283835740043));
#26787=CARTESIAN_POINT('Ctrl Pts',(16.2901158858204,16.8685208581088,5.59117169073376));
#26788=CARTESIAN_POINT('Ctrl Pts',(15.4999999999998,17.3246944774783,5.54950502406709));
#26789=CARTESIAN_POINT('Ctrl Pts',(14.7098841141792,16.8685208581088,5.50783835740043));
#26790=CARTESIAN_POINT('Ctrl Pts',(13.9197682283586,16.4123472387392,5.46617169073376));
#26791=CARTESIAN_POINT('Ctrl Pts',(13.9197682283586,15.5000000000001,5.42450502406709));
#26792=CARTESIAN_POINT('Ctrl Pts',(13.9197682283586,14.5876527612611,5.38283835740042));
#26793=CARTESIAN_POINT('Ctrl Pts',(14.7098841141792,14.1314791418916,5.34117169073376));
#26794=CARTESIAN_POINT('Ctrl Pts',(15.4999999999999,13.675305522522,5.29950502406709));
#26795=CARTESIAN_POINT('Ctrl Pts',(16.2901158858205,14.1314791418916,5.25783835740042));
#26796=CARTESIAN_POINT('Ctrl Pts',(17.0802317716411,14.5876527612611,5.21617169073375));
#26797=CARTESIAN_POINT('Ctrl Pts',(17.0802317716411,15.5000000000002,5.17450502406709));
#26798=CARTESIAN_POINT('Ctrl Pts',(17.0802317716411,16.4123472387392,5.13283835740042));
#26799=CARTESIAN_POINT('Ctrl Pts',(16.2901158858204,16.8685208581088,5.09117169073375));
#26800=CARTESIAN_POINT('Ctrl Pts',(15.4999999999998,17.3246944774783,5.04950502406708));
#26801=CARTESIAN_POINT('Ctrl Pts',(14.7098841141792,16.8685208581088,5.00783835740042));
#26802=CARTESIAN_POINT('Ctrl Pts',(13.9197682283586,16.4123472387392,4.96617169073375));
#26803=CARTESIAN_POINT('Ctrl Pts',(13.9197682283586,15.5000000000001,4.92450502406708));
#26804=CARTESIAN_POINT('Ctrl Pts',(13.9197682283586,14.5876527612611,4.88283835740042));
#26805=CARTESIAN_POINT('Ctrl Pts',(14.7098841141792,14.1314791418916,4.84117169073375));
#26806=CARTESIAN_POINT('Ctrl Pts',(15.4999999999999,13.675305522522,4.79950502406708));
#26807=CARTESIAN_POINT('Ctrl Pts',(16.2901158858205,14.1314791418916,4.75783835740041));
#26808=CARTESIAN_POINT('Ctrl Pts',(17.0802317716411,14.5876527612611,4.71617169073375));
#26809=CARTESIAN_POINT('Ctrl Pts',(17.0802317716411,15.5000000000002,4.67450502406708));
#26810=CARTESIAN_POINT('Ctrl Pts',(17.0802317716411,16.4123472387392,4.63283835740041));
#26811=CARTESIAN_POINT('Ctrl Pts',(16.2901158858204,16.8685208581088,4.59117169073375));
#26812=CARTESIAN_POINT('Ctrl Pts',(15.4999999999998,17.3246944774783,4.54950502406708));
#26813=CARTESIAN_POINT('Ctrl Pts',(14.7098841141792,16.8685208581088,4.50783835740041));
#26814=CARTESIAN_POINT('Ctrl Pts',(13.9197682283586,16.4123472387392,4.46617169073374));
#26815=CARTESIAN_POINT('Ctrl Pts',(13.9197682283586,15.5000000000001,4.42450502406708));
#26816=CARTESIAN_POINT('Ctrl Pts',(13.9197682283586,14.5876527612611,4.38283835740041));
#26817=CARTESIAN_POINT('Ctrl Pts',(14.7098841141792,14.1314791418916,4.34117169073374));
#26818=CARTESIAN_POINT('Ctrl Pts',(15.4999999999999,13.675305522522,4.29950502406708));
#26819=CARTESIAN_POINT('Ctrl Pts',(16.2901158858205,14.1314791418916,4.25783835740041));
#26820=CARTESIAN_POINT('Ctrl Pts',(17.0802317716411,14.5876527612611,4.21617169073374));
#26821=CARTESIAN_POINT('Ctrl Pts',(17.0802317716411,15.5000000000002,4.17450502406707));
#26822=CARTESIAN_POINT('Ctrl Pts',(17.0802317716411,16.4123472387392,4.13283835740041));
#26823=CARTESIAN_POINT('Ctrl Pts',(16.2901158858204,16.8685208581088,4.09117169073374));
#26824=CARTESIAN_POINT('Ctrl Pts',(15.4999999999998,17.3246944774783,4.04950502406707));
#26825=CARTESIAN_POINT('Ctrl Pts',(14.7098841141792,16.8685208581088,4.0078383574004));
#26826=CARTESIAN_POINT('Ctrl Pts',(13.9197682283586,16.4123472387392,3.96617169073374));
#26827=CARTESIAN_POINT('Ctrl Pts',(13.9197682283586,15.5000000000001,3.92450502406707));
#26828=CARTESIAN_POINT('Ctrl Pts',(13.9197682283586,14.5876527612611,3.8828383574004));
#26829=CARTESIAN_POINT('Ctrl Pts',(14.7098841141792,14.1314791418916,3.84117169073374));
#26830=CARTESIAN_POINT('Ctrl Pts',(15.4999999999999,13.675305522522,3.79950502406707));
#26831=CARTESIAN_POINT('Ctrl Pts',(16.2901158858205,14.1314791418916,3.7578383574004));
#26832=CARTESIAN_POINT('Ctrl Pts',(17.0802317716411,14.5876527612611,3.71617169073373));
#26833=CARTESIAN_POINT('Ctrl Pts',(17.0802317716411,15.5000000000002,3.67450502406707));
#26834=CARTESIAN_POINT('Ctrl Pts',(17.0802317716411,16.4123472387392,3.6328383574004));
#26835=CARTESIAN_POINT('Ctrl Pts',(16.2901158858204,16.8685208581088,3.59117169073373));
#26836=CARTESIAN_POINT('Ctrl Pts',(15.4999999999998,17.3246944774783,3.54950502406707));
#26837=CARTESIAN_POINT('Ctrl Pts',(14.7098841141792,16.8685208581088,3.5078383574004));
#26838=CARTESIAN_POINT('Ctrl Pts',(13.9197682283586,16.4123472387392,3.46617169073373));
#26839=CARTESIAN_POINT('Ctrl Pts',(13.9197682283586,15.5000000000001,3.42450502406706));
#26840=CARTESIAN_POINT('Ctrl Pts',(13.9197682283586,14.5876527612611,3.3828383574004));
#26841=CARTESIAN_POINT('Ctrl Pts',(14.7098841141792,14.1314791418916,3.34117169073373));
#26842=CARTESIAN_POINT('Ctrl Pts',(15.4999999999999,13.675305522522,3.29950502406706));
#26843=CARTESIAN_POINT('Ctrl Pts',(16.2901158858205,14.1314791418916,3.2578383574004));
#26844=CARTESIAN_POINT('Ctrl Pts',(17.0802317716411,14.5876527612611,3.21617169073373));
#26845=CARTESIAN_POINT('Ctrl Pts',(17.0802317716411,15.5000000000002,3.17450502406706));
#26846=CARTESIAN_POINT('Ctrl Pts',(17.0802317716411,16.4123472387392,3.13283835740039));
#26847=CARTESIAN_POINT('Ctrl Pts',(16.2901158858204,16.8685208581088,3.09117169073373));
#26848=CARTESIAN_POINT('Ctrl Pts',(15.4999999999998,17.3246944774783,3.04950502406706));
#26849=CARTESIAN_POINT('Ctrl Pts',(14.7098841141792,16.8685208581088,3.00783835740039));
#26850=CARTESIAN_POINT('Ctrl Pts',(13.9197682283586,16.4123472387392,2.96617169073372));
#26851=CARTESIAN_POINT('Ctrl Pts',(13.9197682283586,15.5000000000001,2.92450502406706));
#26852=CARTESIAN_POINT('Ctrl Pts',(13.9197682283586,14.5876527612611,2.88283835740039));
#26853=CARTESIAN_POINT('Ctrl Pts',(14.7098841141792,14.1314791418916,2.84117169073372));
#26854=CARTESIAN_POINT('Ctrl Pts',(15.4999999999999,13.675305522522,2.79950502406705));
#26855=CARTESIAN_POINT('Ctrl Pts',(16.2901158858205,14.1314791418916,2.75783835740039));
#26856=CARTESIAN_POINT('Ctrl Pts',(17.0802317716411,14.5876527612611,2.71617169073372));
#26857=CARTESIAN_POINT('Ctrl Pts',(17.0802317716411,15.5000000000002,2.67450502406705));
#26858=CARTESIAN_POINT('Ctrl Pts',(17.0802317716411,16.4123472387392,2.63283835740039));
#26859=CARTESIAN_POINT('Ctrl Pts',(16.2901158858204,16.8685208581088,2.59117169073372));
#26860=CARTESIAN_POINT('Ctrl Pts',(15.4999999999998,17.3246944774783,2.54950502406705));
#26861=CARTESIAN_POINT('Ctrl Pts',(14.7098841141792,16.8685208581088,2.50783835740038));
#26862=CARTESIAN_POINT('Ctrl Pts',(13.9197682283586,16.4123472387392,2.46617169073372));
#26863=CARTESIAN_POINT('Ctrl Pts',(13.9197682283586,15.5000000000001,2.42450502406705));
#26864=CARTESIAN_POINT('Ctrl Pts',(13.9197682283586,14.5876527612611,2.38283835740038));
#26865=CARTESIAN_POINT('Ctrl Pts',(14.7098841141792,14.1314791418916,2.34117169073372));
#26866=CARTESIAN_POINT('Ctrl Pts',(15.4999999999999,13.675305522522,2.29950502406705));
#26867=CARTESIAN_POINT('Ctrl Pts',(16.2901158858205,14.1314791418916,2.25783835740038));
#26868=CARTESIAN_POINT('Ctrl Pts',(17.0802317716411,14.5876527612611,2.21617169073371));
#26869=CARTESIAN_POINT('Ctrl Pts',(17.0802317716411,15.5000000000002,2.17450502406705));
#26870=CARTESIAN_POINT('Ctrl Pts',(17.0802317716411,16.4123472387392,2.13283835740038));
#26871=CARTESIAN_POINT('Ctrl Pts',(16.2901158858204,16.8685208581088,2.09117169073371));
#26872=CARTESIAN_POINT('Ctrl Pts',(15.4999999999998,17.3246944774783,2.04950502406705));
#26873=CARTESIAN_POINT('Ctrl Pts',(14.7098841141792,16.8685208581088,2.00783835740038));
#26874=CARTESIAN_POINT('Ctrl Pts',(13.9197682283586,16.4123472387392,1.96617169073371));
#26875=CARTESIAN_POINT('Ctrl Pts',(13.9197682283586,15.5000000000001,1.92450502406704));
#26876=CARTESIAN_POINT('Ctrl Pts',(13.9197682283586,14.5876527612611,1.88283835740038));
#26877=CARTESIAN_POINT('Ctrl Pts',(14.7098841141792,14.1314791418916,1.84117169073371));
#26878=CARTESIAN_POINT('Ctrl Pts',(15.4999999999999,13.675305522522,1.79950502406704));
#26879=CARTESIAN_POINT('Ctrl Pts',(16.2901158858205,14.1314791418916,1.75783835740037));
#26880=CARTESIAN_POINT('Ctrl Pts',(17.0802317716411,14.5876527612611,1.71617169073371));
#26881=CARTESIAN_POINT('Ctrl Pts',(17.0802317716411,15.5000000000002,1.67450502406704));
#26882=CARTESIAN_POINT('Ctrl Pts',(17.0802317716411,16.4123472387392,1.63283835740037));
#26883=CARTESIAN_POINT('Ctrl Pts',(16.2901158858204,16.8685208581088,1.59117169073371));
#26884=CARTESIAN_POINT('Ctrl Pts',(15.4999999999998,17.3246944774783,1.54950502406704));
#26885=CARTESIAN_POINT('Ctrl Pts',(14.7098841141792,16.8685208581088,1.50783835740037));
#26886=CARTESIAN_POINT('Ctrl Pts',(13.9197682283586,16.4123472387392,1.4661716907337));
#26887=CARTESIAN_POINT('Ctrl Pts',(13.9197682283586,15.5000000000001,1.42450502406704));
#26888=CARTESIAN_POINT('Ctrl Pts',(13.9197682283586,14.5876527612611,1.38283835740037));
#26889=CARTESIAN_POINT('Ctrl Pts',(14.7098841141792,14.1314791418916,1.3411716907337));
#26890=CARTESIAN_POINT('Ctrl Pts',(15.4999999999999,13.675305522522,1.29950502406703));
#26891=CARTESIAN_POINT('Ctrl Pts',(16.2901158858205,14.1314791418916,1.25783835740037));
#26892=CARTESIAN_POINT('Ctrl Pts',(17.0802317716411,14.5876527612611,1.2161716907337));
#26893=CARTESIAN_POINT('Ctrl Pts',(17.0802317716411,15.5000000000002,1.17450502406703));
#26894=CARTESIAN_POINT('Ctrl Pts',(17.0802317716411,16.4123472387392,1.13283835740037));
#26895=CARTESIAN_POINT('Ctrl Pts',(16.2901158858204,16.8685208581088,1.0911716907337));
#26896=CARTESIAN_POINT('Ctrl Pts',(15.4999999999998,17.3246944774783,1.04950502406703));
#26897=CARTESIAN_POINT('Ctrl Pts',(14.7098841141792,16.8685208581088,1.00783835740037));
#26898=CARTESIAN_POINT('Ctrl Pts',(13.9197682283586,16.4123472387392,0.966171690733698));
#26899=CARTESIAN_POINT('Ctrl Pts',(13.9197682283586,15.5000000000001,0.924505024067031));
#26900=CARTESIAN_POINT('Ctrl Pts',(13.9197682283586,14.5876527612611,0.882838357400363));
#26901=CARTESIAN_POINT('Ctrl Pts',(14.7098841141792,14.1314791418916,0.841171690733696));
#26902=CARTESIAN_POINT('Ctrl Pts',(15.4999999999999,13.675305522522,0.799505024067029));
#26903=CARTESIAN_POINT('Ctrl Pts',(16.2901158858205,14.1314791418916,0.757838357400362));
#26904=CARTESIAN_POINT('Ctrl Pts',(17.0802317716411,14.5876527612611,0.716171690733694));
#26905=CARTESIAN_POINT('Ctrl Pts',(17.0802317716411,15.5000000000002,0.674505024067027));
#26906=CARTESIAN_POINT('Ctrl Pts',(17.0802317716411,16.4123472387392,0.632838357400359));
#26907=CARTESIAN_POINT('Ctrl Pts',(16.2901158858204,16.8685208581088,0.591171690733692));
#26908=CARTESIAN_POINT('Ctrl Pts',(15.4999999999998,17.3246944774783,0.549505024067025));
#26909=CARTESIAN_POINT('Ctrl Pts',(14.7098841141792,16.8685208581088,0.507838357400358));
#26910=CARTESIAN_POINT('Ctrl Pts',(13.9197682283586,16.4123472387392,0.46617169073369));
#26911=CARTESIAN_POINT('Ctrl Pts',(13.9197682283586,15.5000000000001,0.424505024067023));
#26912=CARTESIAN_POINT('Ctrl Pts',(13.9197682283586,14.5876527612611,0.382838357400356));
#26913=CARTESIAN_POINT('Ctrl Pts',(14.7098841141792,14.1314791418916,0.341171690733689));
#26914=CARTESIAN_POINT('Ctrl Pts',(15.4999999999999,13.675305522522,0.299505024067021));
#26915=CARTESIAN_POINT('Ctrl Pts',(16.2901158858205,14.1314791418916,0.257838357400354));
#26916=CARTESIAN_POINT('Ctrl Pts',(17.0802317716411,14.5876527612611,0.216171690733687));
#26917=CARTESIAN_POINT('Ctrl Pts',(17.0802317716411,15.5000000000002,0.174505024067019));
#26918=CARTESIAN_POINT('Ctrl Pts',(17.0802317716411,16.4123472387392,0.132838357400352));
#26919=CARTESIAN_POINT('Ctrl Pts',(16.2901158858204,16.8685208581088,0.0911716907336848));
#26920=CARTESIAN_POINT('Ctrl Pts',(15.4999999999998,17.3246944774783,0.0495050240670175));
#26921=CARTESIAN_POINT('Ctrl Pts',(14.7098841141792,16.8685208581088,0.00783835740035027));
#26922=CARTESIAN_POINT('Ctrl Pts',(13.9197682283586,16.4123472387392,-0.033828309266317));
#26923=CARTESIAN_POINT('Ctrl Pts',(13.9197682283586,15.5000000000001,-0.0754949759329843));
#26924=CARTESIAN_POINT('Ctrl Pts',(13.9197682283586,14.5876527612611,-0.11716164259965));
#26925=CARTESIAN_POINT('Ctrl Pts',(14.7098841141792,14.1314791418916,-0.158828309266317));
#26926=CARTESIAN_POINT('Ctrl Pts',(15.4999999999999,13.675305522522,-0.200494975932984));
#26927=CARTESIAN_POINT('Ctrl Pts',(16.2901158858205,14.1314791418916,-0.242161642599652));
#26928=CARTESIAN_POINT('Ctrl Pts',(17.0802317716411,14.5876527612611,-0.283828309266319));
#26929=CARTESIAN_POINT('Ctrl Pts',(17.0802317716411,15.5000000000002,-0.325494975932986));
#26930=CARTESIAN_POINT('Ctrl Pts',(17.0802317716411,16.4123472387392,-0.367161642599654));
#26931=CARTESIAN_POINT('Ctrl Pts',(16.2901158858204,16.8685208581088,-0.408828309266321));
#26932=CARTESIAN_POINT('Ctrl Pts',(15.4999999999998,17.3246944774783,-0.450494975932988));
#26933=CARTESIAN_POINT('Ctrl Pts',(14.7098841141792,16.8685208581088,-0.492161642599655));
#26934=CARTESIAN_POINT('Ctrl Pts',(13.9197682283586,16.4123472387392,-0.533828309266323));
#26935=CARTESIAN_POINT('Ctrl Pts',(13.9197682283586,15.5000000000001,-0.57549497593299));
#26936=CARTESIAN_POINT('Ctrl Pts',(13.9197682283586,14.5876527612611,-0.617161642599657));
#26937=CARTESIAN_POINT('Ctrl Pts',(14.7098841141792,14.1314791418916,-0.658828309266325));
#26938=CARTESIAN_POINT('Ctrl Pts',(15.4999999999999,13.675305522522,-0.700494975932992));
#26939=CARTESIAN_POINT('Ctrl Pts',(16.2901158858205,14.1314791418916,-0.742161642599659));
#26940=CARTESIAN_POINT('Ctrl Pts',(17.0802317716411,14.5876527612611,-0.783828309266326));
#26941=CARTESIAN_POINT('Ctrl Pts',(17.0802317716411,15.5000000000002,-0.825494975932994));
#26942=CARTESIAN_POINT('Ctrl Pts',(17.0802317716411,16.4123472387392,-0.867161642599661));
#26943=CARTESIAN_POINT('Ctrl Pts',(16.2901158858204,16.8685208581088,-0.908828309266328));
#26944=CARTESIAN_POINT('Ctrl Pts',(15.4999999999998,17.3246944774783,-0.950494975932996));
#26945=CARTESIAN_POINT('Ctrl Pts',(14.7098841141792,16.8685208581088,-0.992161642599663));
#26946=CARTESIAN_POINT('Ctrl Pts',(13.9197682283586,16.4123472387392,-1.03382830926633));
#26947=CARTESIAN_POINT('Ctrl Pts',(13.9197682283586,15.5000000000001,-1.075494975933));
#26948=CARTESIAN_POINT('Ctrl Pts',(13.9197682283586,14.5876527612611,-1.11716164259966));
#26949=CARTESIAN_POINT('Ctrl Pts',(14.7098841141792,14.1314791418916,-1.15882830926633));
#26950=CARTESIAN_POINT('Ctrl Pts',(15.4999999999999,13.675305522522,-1.200494975933));
#26951=CARTESIAN_POINT('Ctrl Pts',(16.2901158858205,14.1314791418916,-1.24216164259967));
#26952=CARTESIAN_POINT('Ctrl Pts',(17.0802317716411,14.5876527612611,-1.28382830926633));
#26953=CARTESIAN_POINT('Ctrl Pts',(17.0802317716411,15.5000000000002,-1.325494975933));
#26954=CARTESIAN_POINT('Ctrl Pts',(17.0802317716411,16.4123472387392,-1.36716164259967));
#26955=CARTESIAN_POINT('Ctrl Pts',(16.2901158858204,16.8685208581088,-1.40882830926633));
#26956=CARTESIAN_POINT('Ctrl Pts',(15.4999999999998,17.3246944774783,-1.450494975933));
#26957=CARTESIAN_POINT('Ctrl Pts',(14.7098841141792,16.8685208581088,-1.49216164259967));
#26958=CARTESIAN_POINT('Ctrl Pts',(13.9197682283586,16.4123472387392,-1.53382830926634));
#26959=CARTESIAN_POINT('Ctrl Pts',(13.9197682283586,15.5000000000001,-1.575494975933));
#26960=CARTESIAN_POINT('Ctrl Pts',(13.9197682283586,14.5876527612611,-1.61716164259967));
#26961=CARTESIAN_POINT('Ctrl Pts',(14.7098841141792,14.1314791418916,-1.65882830926634));
#26962=CARTESIAN_POINT('Ctrl Pts',(15.4999999999999,13.675305522522,-1.70049497593301));
#26963=CARTESIAN_POINT('Ctrl Pts',(16.2901158858205,14.1314791418916,-1.74216164259967));
#26964=CARTESIAN_POINT('Ctrl Pts',(17.0802317716411,14.5876527612611,-1.78382830926634));
#26965=CARTESIAN_POINT('Ctrl Pts',(17.0802317716411,15.5000000000002,-1.82549497593301));
#26966=CARTESIAN_POINT('Ctrl Pts',(17.0802317716411,16.4123472387392,-1.86716164259967));
#26967=CARTESIAN_POINT('Ctrl Pts',(16.2901158858204,16.8685208581088,-1.90882830926634));
#26968=CARTESIAN_POINT('Ctrl Pts',(15.4999999999998,17.3246944774783,-1.95049497593301));
#26969=CARTESIAN_POINT('Ctrl Pts',(14.7098841141792,16.8685208581088,-1.99216164259968));
#26970=CARTESIAN_POINT('Ctrl Pts',(14.4189893226642,16.7005726719217,-2.00750194461187));
#26971=CARTESIAN_POINT('Ctrl Pts',(14.221556935765,16.4288249477779,-2.02511838079831));
#26972=CARTESIAN_POINT('Ctrl Pts',(17.4320632938681,15.5000000000002,10.971375));
#26973=CARTESIAN_POINT('Ctrl Pts',(17.4320632938681,16.6154772628064,10.9297083333333));
#26974=CARTESIAN_POINT('Ctrl Pts',(16.466031646934,17.1732158942095,10.8880416666667));
#26975=CARTESIAN_POINT('Ctrl Pts',(15.4999999999998,17.7309545256126,10.846375));
#26976=CARTESIAN_POINT('Ctrl Pts',(14.5339683530657,17.1732158942095,10.8047083333333));
#26977=CARTESIAN_POINT('Ctrl Pts',(13.5679367061316,16.6154772628064,10.7630416666667));
#26978=CARTESIAN_POINT('Ctrl Pts',(13.5679367061316,15.5000000000001,10.721375));
#26979=CARTESIAN_POINT('Ctrl Pts',(13.5679367061316,14.3845227371939,10.6797083333333));
#26980=CARTESIAN_POINT('Ctrl Pts',(14.5339683530657,13.8267841057908,10.6380416666667));
#26981=CARTESIAN_POINT('Ctrl Pts',(15.4999999999999,13.2690454743877,10.596375));
#26982=CARTESIAN_POINT('Ctrl Pts',(16.466031646934,13.8267841057908,10.5547083333333));
#26983=CARTESIAN_POINT('Ctrl Pts',(17.4320632938681,14.3845227371939,10.5130416666667));
#26984=CARTESIAN_POINT('Ctrl Pts',(17.4320632938681,15.5000000000002,10.471375));
#26985=CARTESIAN_POINT('Ctrl Pts',(17.4320632938681,16.6154772628064,10.4297083333333));
#26986=CARTESIAN_POINT('Ctrl Pts',(16.466031646934,17.1732158942095,10.3880416666667));
#26987=CARTESIAN_POINT('Ctrl Pts',(15.4999999999998,17.7309545256126,10.346375));
#26988=CARTESIAN_POINT('Ctrl Pts',(14.5339683530657,17.1732158942095,10.3047083333333));
#26989=CARTESIAN_POINT('Ctrl Pts',(13.5679367061316,16.6154772628064,10.2630416666667));
#26990=CARTESIAN_POINT('Ctrl Pts',(13.5679367061316,15.5000000000001,10.221375));
#26991=CARTESIAN_POINT('Ctrl Pts',(13.5679367061316,14.3845227371939,10.1797083333333));
#26992=CARTESIAN_POINT('Ctrl Pts',(14.5339683530657,13.8267841057908,10.1380416666667));
#26993=CARTESIAN_POINT('Ctrl Pts',(15.4999999999999,13.2690454743877,10.096375));
#26994=CARTESIAN_POINT('Ctrl Pts',(16.466031646934,13.8267841057908,10.0547083333333));
#26995=CARTESIAN_POINT('Ctrl Pts',(17.4320632938681,14.3845227371939,10.0130416666666));
#26996=CARTESIAN_POINT('Ctrl Pts',(17.4320632938681,15.5000000000002,9.97137499999998));
#26997=CARTESIAN_POINT('Ctrl Pts',(17.4320632938681,16.6154772628064,9.92970833333332));
#26998=CARTESIAN_POINT('Ctrl Pts',(16.466031646934,17.1732158942095,9.88804166666665));
#26999=CARTESIAN_POINT('Ctrl Pts',(15.4999999999998,17.7309545256126,9.84637499999998));
#27000=CARTESIAN_POINT('Ctrl Pts',(14.5339683530657,17.1732158942095,9.80470833333331));
#27001=CARTESIAN_POINT('Ctrl Pts',(13.5679367061316,16.6154772628064,9.76304166666665));
#27002=CARTESIAN_POINT('Ctrl Pts',(13.5679367061316,15.5000000000001,9.72137499999998));
#27003=CARTESIAN_POINT('Ctrl Pts',(13.5679367061316,14.3845227371939,9.67970833333331));
#27004=CARTESIAN_POINT('Ctrl Pts',(14.5339683530657,13.8267841057908,9.63804166666664));
#27005=CARTESIAN_POINT('Ctrl Pts',(15.4999999999999,13.2690454743877,9.59637499999998));
#27006=CARTESIAN_POINT('Ctrl Pts',(16.466031646934,13.8267841057908,9.55470833333331));
#27007=CARTESIAN_POINT('Ctrl Pts',(17.4320632938681,14.3845227371939,9.51304166666664));
#27008=CARTESIAN_POINT('Ctrl Pts',(17.4320632938681,15.5000000000002,9.47137499999998));
#27009=CARTESIAN_POINT('Ctrl Pts',(17.4320632938681,16.6154772628064,9.42970833333331));
#27010=CARTESIAN_POINT('Ctrl Pts',(16.466031646934,17.1732158942095,9.38804166666664));
#27011=CARTESIAN_POINT('Ctrl Pts',(15.4999999999998,17.7309545256126,9.34637499999997));
#27012=CARTESIAN_POINT('Ctrl Pts',(14.5339683530657,17.1732158942095,9.30470833333331));
#27013=CARTESIAN_POINT('Ctrl Pts',(13.5679367061316,16.6154772628064,9.26304166666664));
#27014=CARTESIAN_POINT('Ctrl Pts',(13.5679367061316,15.5000000000001,9.22137499999997));
#27015=CARTESIAN_POINT('Ctrl Pts',(13.5679367061316,14.3845227371939,9.1797083333333));
#27016=CARTESIAN_POINT('Ctrl Pts',(14.5339683530657,13.8267841057908,9.13804166666664));
#27017=CARTESIAN_POINT('Ctrl Pts',(15.4999999999999,13.2690454743877,9.09637499999997));
#27018=CARTESIAN_POINT('Ctrl Pts',(16.466031646934,13.8267841057908,9.0547083333333));
#27019=CARTESIAN_POINT('Ctrl Pts',(17.4320632938681,14.3845227371939,9.01304166666664));
#27020=CARTESIAN_POINT('Ctrl Pts',(17.4320632938681,15.5000000000002,8.97137499999997));
#27021=CARTESIAN_POINT('Ctrl Pts',(17.4320632938681,16.6154772628064,8.9297083333333));
#27022=CARTESIAN_POINT('Ctrl Pts',(16.466031646934,17.1732158942095,8.88804166666663));
#27023=CARTESIAN_POINT('Ctrl Pts',(15.4999999999998,17.7309545256126,8.84637499999997));
#27024=CARTESIAN_POINT('Ctrl Pts',(14.5339683530657,17.1732158942095,8.8047083333333));
#27025=CARTESIAN_POINT('Ctrl Pts',(13.5679367061316,16.6154772628064,8.76304166666663));
#27026=CARTESIAN_POINT('Ctrl Pts',(13.5679367061316,15.5000000000001,8.72137499999997));
#27027=CARTESIAN_POINT('Ctrl Pts',(13.5679367061316,14.3845227371939,8.6797083333333));
#27028=CARTESIAN_POINT('Ctrl Pts',(14.5339683530657,13.8267841057908,8.63804166666663));
#27029=CARTESIAN_POINT('Ctrl Pts',(15.4999999999999,13.2690454743877,8.59637499999996));
#27030=CARTESIAN_POINT('Ctrl Pts',(16.466031646934,13.8267841057908,8.5547083333333));
#27031=CARTESIAN_POINT('Ctrl Pts',(17.4320632938681,14.3845227371939,8.51304166666663));
#27032=CARTESIAN_POINT('Ctrl Pts',(17.4320632938681,15.5000000000002,8.47137499999996));
#27033=CARTESIAN_POINT('Ctrl Pts',(17.4320632938681,16.6154772628064,8.42970833333329));
#27034=CARTESIAN_POINT('Ctrl Pts',(16.466031646934,17.1732158942095,8.38804166666663));
#27035=CARTESIAN_POINT('Ctrl Pts',(15.4999999999998,17.7309545256126,8.34637499999996));
#27036=CARTESIAN_POINT('Ctrl Pts',(14.5339683530657,17.1732158942095,8.30470833333329));
#27037=CARTESIAN_POINT('Ctrl Pts',(13.5679367061316,16.6154772628064,8.26304166666663));
#27038=CARTESIAN_POINT('Ctrl Pts',(13.5679367061316,15.5000000000001,8.22137499999996));
#27039=CARTESIAN_POINT('Ctrl Pts',(13.5679367061316,14.3845227371939,8.17970833333329));
#27040=CARTESIAN_POINT('Ctrl Pts',(14.5339683530657,13.8267841057908,8.13804166666662));
#27041=CARTESIAN_POINT('Ctrl Pts',(15.4999999999999,13.2690454743877,8.09637499999996));
#27042=CARTESIAN_POINT('Ctrl Pts',(16.466031646934,13.8267841057908,8.05470833333329));
#27043=CARTESIAN_POINT('Ctrl Pts',(17.4320632938681,14.3845227371939,8.01304166666662));
#27044=CARTESIAN_POINT('Ctrl Pts',(17.4320632938681,15.5000000000002,7.97137499999995));
#27045=CARTESIAN_POINT('Ctrl Pts',(17.4320632938681,16.6154772628064,7.92970833333329));
#27046=CARTESIAN_POINT('Ctrl Pts',(16.466031646934,17.1732158942095,7.88804166666662));
#27047=CARTESIAN_POINT('Ctrl Pts',(15.4999999999998,17.7309545256126,7.84637499999995));
#27048=CARTESIAN_POINT('Ctrl Pts',(14.5339683530657,17.1732158942095,7.80470833333329));
#27049=CARTESIAN_POINT('Ctrl Pts',(13.5679367061316,16.6154772628064,7.76304166666662));
#27050=CARTESIAN_POINT('Ctrl Pts',(13.5679367061316,15.5000000000001,7.72137499999995));
#27051=CARTESIAN_POINT('Ctrl Pts',(13.5679367061316,14.3845227371939,7.67970833333329));
#27052=CARTESIAN_POINT('Ctrl Pts',(14.5339683530657,13.8267841057908,7.63804166666662));
#27053=CARTESIAN_POINT('Ctrl Pts',(15.4999999999999,13.2690454743877,7.59637499999995));
#27054=CARTESIAN_POINT('Ctrl Pts',(16.466031646934,13.8267841057908,7.55470833333328));
#27055=CARTESIAN_POINT('Ctrl Pts',(17.4320632938681,14.3845227371939,7.51304166666662));
#27056=CARTESIAN_POINT('Ctrl Pts',(17.4320632938681,15.5000000000002,7.47137499999995));
#27057=CARTESIAN_POINT('Ctrl Pts',(17.4320632938681,16.6154772628064,7.42970833333328));
#27058=CARTESIAN_POINT('Ctrl Pts',(16.466031646934,17.1732158942095,7.38804166666661));
#27059=CARTESIAN_POINT('Ctrl Pts',(15.4999999999998,17.7309545256126,7.34637499999995));
#27060=CARTESIAN_POINT('Ctrl Pts',(14.5339683530657,17.1732158942095,7.30470833333328));
#27061=CARTESIAN_POINT('Ctrl Pts',(13.5679367061316,16.6154772628064,7.26304166666661));
#27062=CARTESIAN_POINT('Ctrl Pts',(13.5679367061316,15.5000000000001,7.22137499999994));
#27063=CARTESIAN_POINT('Ctrl Pts',(13.5679367061316,14.3845227371939,7.17970833333328));
#27064=CARTESIAN_POINT('Ctrl Pts',(14.5339683530657,13.8267841057908,7.13804166666661));
#27065=CARTESIAN_POINT('Ctrl Pts',(15.4999999999999,13.2690454743877,7.09637499999995));
#27066=CARTESIAN_POINT('Ctrl Pts',(16.466031646934,13.8267841057908,7.05470833333328));
#27067=CARTESIAN_POINT('Ctrl Pts',(17.4320632938681,14.3845227371939,7.01304166666661));
#27068=CARTESIAN_POINT('Ctrl Pts',(17.4320632938681,15.5000000000002,6.97137499999994));
#27069=CARTESIAN_POINT('Ctrl Pts',(17.4320632938681,16.6154772628064,6.92970833333328));
#27070=CARTESIAN_POINT('Ctrl Pts',(16.466031646934,17.1732158942095,6.88804166666661));
#27071=CARTESIAN_POINT('Ctrl Pts',(15.4999999999998,17.7309545256126,6.84637499999994));
#27072=CARTESIAN_POINT('Ctrl Pts',(14.5339683530657,17.1732158942095,6.80470833333327));
#27073=CARTESIAN_POINT('Ctrl Pts',(13.5679367061316,16.6154772628064,6.76304166666661));
#27074=CARTESIAN_POINT('Ctrl Pts',(13.5679367061316,15.5000000000001,6.72137499999994));
#27075=CARTESIAN_POINT('Ctrl Pts',(13.5679367061316,14.3845227371939,6.67970833333327));
#27076=CARTESIAN_POINT('Ctrl Pts',(14.5339683530657,13.8267841057908,6.6380416666666));
#27077=CARTESIAN_POINT('Ctrl Pts',(15.4999999999999,13.2690454743877,6.59637499999994));
#27078=CARTESIAN_POINT('Ctrl Pts',(16.466031646934,13.8267841057908,6.55470833333327));
#27079=CARTESIAN_POINT('Ctrl Pts',(17.4320632938681,14.3845227371939,6.5130416666666));
#27080=CARTESIAN_POINT('Ctrl Pts',(17.4320632938681,15.5000000000002,6.47137499999994));
#27081=CARTESIAN_POINT('Ctrl Pts',(17.4320632938681,16.6154772628064,6.42970833333327));
#27082=CARTESIAN_POINT('Ctrl Pts',(16.466031646934,17.1732158942095,6.3880416666666));
#27083=CARTESIAN_POINT('Ctrl Pts',(15.4999999999998,17.7309545256126,6.34637499999993));
#27084=CARTESIAN_POINT('Ctrl Pts',(14.5339683530657,17.1732158942095,6.30470833333327));
#27085=CARTESIAN_POINT('Ctrl Pts',(13.5679367061316,16.6154772628064,6.2630416666666));
#27086=CARTESIAN_POINT('Ctrl Pts',(13.5679367061316,15.5000000000001,6.22137499999993));
#27087=CARTESIAN_POINT('Ctrl Pts',(13.5679367061316,14.3845227371939,6.17970833333327));
#27088=CARTESIAN_POINT('Ctrl Pts',(14.5339683530657,13.8267841057908,6.1380416666666));
#27089=CARTESIAN_POINT('Ctrl Pts',(15.4999999999999,13.2690454743877,6.09637499999993));
#27090=CARTESIAN_POINT('Ctrl Pts',(16.466031646934,13.8267841057908,6.05470833333326));
#27091=CARTESIAN_POINT('Ctrl Pts',(17.4320632938681,14.3845227371939,6.0130416666666));
#27092=CARTESIAN_POINT('Ctrl Pts',(17.4320632938681,15.5000000000002,5.97137499999993));
#27093=CARTESIAN_POINT('Ctrl Pts',(17.4320632938681,16.6154772628064,5.92970833333326));
#27094=CARTESIAN_POINT('Ctrl Pts',(16.466031646934,17.1732158942095,5.8880416666666));
#27095=CARTESIAN_POINT('Ctrl Pts',(15.4999999999998,17.7309545256126,5.84637499999993));
#27096=CARTESIAN_POINT('Ctrl Pts',(14.5339683530657,17.1732158942095,5.80470833333326));
#27097=CARTESIAN_POINT('Ctrl Pts',(13.5679367061316,16.6154772628064,5.76304166666659));
#27098=CARTESIAN_POINT('Ctrl Pts',(13.5679367061316,15.5000000000001,5.72137499999993));
#27099=CARTESIAN_POINT('Ctrl Pts',(13.5679367061316,14.3845227371939,5.67970833333326));
#27100=CARTESIAN_POINT('Ctrl Pts',(14.5339683530657,13.8267841057908,5.63804166666659));
#27101=CARTESIAN_POINT('Ctrl Pts',(15.4999999999999,13.2690454743877,5.59637499999992));
#27102=CARTESIAN_POINT('Ctrl Pts',(16.466031646934,13.8267841057908,5.55470833333326));
#27103=CARTESIAN_POINT('Ctrl Pts',(17.4320632938681,14.3845227371939,5.51304166666659));
#27104=CARTESIAN_POINT('Ctrl Pts',(17.4320632938681,15.5000000000002,5.47137499999992));
#27105=CARTESIAN_POINT('Ctrl Pts',(17.4320632938681,16.6154772628064,5.42970833333325));
#27106=CARTESIAN_POINT('Ctrl Pts',(16.466031646934,17.1732158942095,5.38804166666659));
#27107=CARTESIAN_POINT('Ctrl Pts',(15.4999999999998,17.7309545256126,5.34637499999992));
#27108=CARTESIAN_POINT('Ctrl Pts',(14.5339683530657,17.1732158942095,5.30470833333325));
#27109=CARTESIAN_POINT('Ctrl Pts',(13.5679367061316,16.6154772628064,5.26304166666659));
#27110=CARTESIAN_POINT('Ctrl Pts',(13.5679367061316,15.5000000000001,5.22137499999992));
#27111=CARTESIAN_POINT('Ctrl Pts',(13.5679367061316,14.3845227371939,5.17970833333325));
#27112=CARTESIAN_POINT('Ctrl Pts',(14.5339683530657,13.8267841057908,5.13804166666659));
#27113=CARTESIAN_POINT('Ctrl Pts',(15.4999999999999,13.2690454743877,5.09637499999992));
#27114=CARTESIAN_POINT('Ctrl Pts',(16.466031646934,13.8267841057908,5.05470833333325));
#27115=CARTESIAN_POINT('Ctrl Pts',(17.4320632938681,14.3845227371939,5.01304166666658));
#27116=CARTESIAN_POINT('Ctrl Pts',(17.4320632938681,15.5000000000002,4.97137499999991));
#27117=CARTESIAN_POINT('Ctrl Pts',(17.4320632938681,16.6154772628064,4.92970833333325));
#27118=CARTESIAN_POINT('Ctrl Pts',(16.466031646934,17.1732158942095,4.88804166666658));
#27119=CARTESIAN_POINT('Ctrl Pts',(15.4999999999998,17.7309545256126,4.84637499999991));
#27120=CARTESIAN_POINT('Ctrl Pts',(14.5339683530657,17.1732158942095,4.80470833333325));
#27121=CARTESIAN_POINT('Ctrl Pts',(13.5679367061316,16.6154772628064,4.76304166666658));
#27122=CARTESIAN_POINT('Ctrl Pts',(13.5679367061316,15.5000000000001,4.72137499999991));
#27123=CARTESIAN_POINT('Ctrl Pts',(13.5679367061316,14.3845227371939,4.67970833333325));
#27124=CARTESIAN_POINT('Ctrl Pts',(14.5339683530657,13.8267841057908,4.63804166666658));
#27125=CARTESIAN_POINT('Ctrl Pts',(15.4999999999999,13.2690454743877,4.59637499999991));
#27126=CARTESIAN_POINT('Ctrl Pts',(16.466031646934,13.8267841057908,4.55470833333324));
#27127=CARTESIAN_POINT('Ctrl Pts',(17.4320632938681,14.3845227371939,4.51304166666658));
#27128=CARTESIAN_POINT('Ctrl Pts',(17.4320632938681,15.5000000000002,4.47137499999991));
#27129=CARTESIAN_POINT('Ctrl Pts',(17.4320632938681,16.6154772628064,4.42970833333324));
#27130=CARTESIAN_POINT('Ctrl Pts',(16.466031646934,17.1732158942095,4.38804166666657));
#27131=CARTESIAN_POINT('Ctrl Pts',(15.4999999999998,17.7309545256126,4.34637499999991));
#27132=CARTESIAN_POINT('Ctrl Pts',(14.5339683530657,17.1732158942095,4.30470833333324));
#27133=CARTESIAN_POINT('Ctrl Pts',(13.5679367061316,16.6154772628064,4.26304166666657));
#27134=CARTESIAN_POINT('Ctrl Pts',(13.5679367061316,15.5000000000001,4.22137499999991));
#27135=CARTESIAN_POINT('Ctrl Pts',(13.5679367061316,14.3845227371939,4.17970833333324));
#27136=CARTESIAN_POINT('Ctrl Pts',(14.5339683530657,13.8267841057908,4.13804166666657));
#27137=CARTESIAN_POINT('Ctrl Pts',(15.4999999999999,13.2690454743877,4.0963749999999));
#27138=CARTESIAN_POINT('Ctrl Pts',(16.466031646934,13.8267841057908,4.05470833333324));
#27139=CARTESIAN_POINT('Ctrl Pts',(17.4320632938681,14.3845227371939,4.01304166666657));
#27140=CARTESIAN_POINT('Ctrl Pts',(17.4320632938681,15.5000000000002,3.9713749999999));
#27141=CARTESIAN_POINT('Ctrl Pts',(17.4320632938681,16.6154772628064,3.92970833333323));
#27142=CARTESIAN_POINT('Ctrl Pts',(16.466031646934,17.1732158942095,3.88804166666657));
#27143=CARTESIAN_POINT('Ctrl Pts',(15.4999999999998,17.7309545256126,3.8463749999999));
#27144=CARTESIAN_POINT('Ctrl Pts',(14.5339683530657,17.1732158942095,3.80470833333323));
#27145=CARTESIAN_POINT('Ctrl Pts',(13.5679367061316,16.6154772628064,3.76304166666656));
#27146=CARTESIAN_POINT('Ctrl Pts',(13.5679367061316,15.5000000000001,3.7213749999999));
#27147=CARTESIAN_POINT('Ctrl Pts',(13.5679367061316,14.3845227371939,3.67970833333323));
#27148=CARTESIAN_POINT('Ctrl Pts',(14.5339683530657,13.8267841057908,3.63804166666656));
#27149=CARTESIAN_POINT('Ctrl Pts',(15.4999999999999,13.2690454743877,3.5963749999999));
#27150=CARTESIAN_POINT('Ctrl Pts',(16.466031646934,13.8267841057908,3.55470833333323));
#27151=CARTESIAN_POINT('Ctrl Pts',(17.4320632938681,14.3845227371939,3.51304166666656));
#27152=CARTESIAN_POINT('Ctrl Pts',(17.4320632938681,15.5000000000002,3.4713749999999));
#27153=CARTESIAN_POINT('Ctrl Pts',(17.4320632938681,16.6154772628064,3.42970833333323));
#27154=CARTESIAN_POINT('Ctrl Pts',(16.466031646934,17.1732158942095,3.38804166666656));
#27155=CARTESIAN_POINT('Ctrl Pts',(15.4999999999998,17.7309545256126,3.34637499999989));
#27156=CARTESIAN_POINT('Ctrl Pts',(14.5339683530657,17.1732158942095,3.30470833333323));
#27157=CARTESIAN_POINT('Ctrl Pts',(13.5679367061316,16.6154772628064,3.26304166666656));
#27158=CARTESIAN_POINT('Ctrl Pts',(13.5679367061316,15.5000000000001,3.22137499999989));
#27159=CARTESIAN_POINT('Ctrl Pts',(13.5679367061316,14.3845227371939,3.17970833333322));
#27160=CARTESIAN_POINT('Ctrl Pts',(14.5339683530657,13.8267841057908,3.13804166666656));
#27161=CARTESIAN_POINT('Ctrl Pts',(15.4999999999999,13.2690454743877,3.09637499999989));
#27162=CARTESIAN_POINT('Ctrl Pts',(16.466031646934,13.8267841057908,3.05470833333322));
#27163=CARTESIAN_POINT('Ctrl Pts',(17.4320632938681,14.3845227371939,3.01304166666656));
#27164=CARTESIAN_POINT('Ctrl Pts',(17.4320632938681,15.5000000000002,2.97137499999989));
#27165=CARTESIAN_POINT('Ctrl Pts',(17.4320632938681,16.6154772628064,2.92970833333322));
#27166=CARTESIAN_POINT('Ctrl Pts',(16.466031646934,17.1732158942095,2.88804166666655));
#27167=CARTESIAN_POINT('Ctrl Pts',(15.4999999999998,17.7309545256126,2.84637499999989));
#27168=CARTESIAN_POINT('Ctrl Pts',(14.5339683530657,17.1732158942095,2.80470833333322));
#27169=CARTESIAN_POINT('Ctrl Pts',(13.5679367061316,16.6154772628064,2.76304166666655));
#27170=CARTESIAN_POINT('Ctrl Pts',(13.5679367061316,15.5000000000001,2.72137499999989));
#27171=CARTESIAN_POINT('Ctrl Pts',(13.5679367061316,14.3845227371939,2.67970833333322));
#27172=CARTESIAN_POINT('Ctrl Pts',(14.5339683530657,13.8267841057908,2.63804166666655));
#27173=CARTESIAN_POINT('Ctrl Pts',(15.4999999999999,13.2690454743877,2.59637499999988));
#27174=CARTESIAN_POINT('Ctrl Pts',(16.466031646934,13.8267841057908,2.55470833333322));
#27175=CARTESIAN_POINT('Ctrl Pts',(17.4320632938681,14.3845227371939,2.51304166666655));
#27176=CARTESIAN_POINT('Ctrl Pts',(17.4320632938681,15.5000000000002,2.47137499999988));
#27177=CARTESIAN_POINT('Ctrl Pts',(17.4320632938681,16.6154772628064,2.42970833333321));
#27178=CARTESIAN_POINT('Ctrl Pts',(16.466031646934,17.1732158942095,2.38804166666655));
#27179=CARTESIAN_POINT('Ctrl Pts',(15.4999999999998,17.7309545256126,2.34637499999988));
#27180=CARTESIAN_POINT('Ctrl Pts',(14.5339683530657,17.1732158942095,2.30470833333321));
#27181=CARTESIAN_POINT('Ctrl Pts',(13.5679367061316,16.6154772628064,2.26304166666655));
#27182=CARTESIAN_POINT('Ctrl Pts',(13.5679367061316,15.5000000000001,2.22137499999988));
#27183=CARTESIAN_POINT('Ctrl Pts',(13.5679367061316,14.3845227371939,2.17970833333321));
#27184=CARTESIAN_POINT('Ctrl Pts',(14.5339683530657,13.8267841057908,2.13804166666654));
#27185=CARTESIAN_POINT('Ctrl Pts',(15.4999999999999,13.2690454743877,2.09637499999988));
#27186=CARTESIAN_POINT('Ctrl Pts',(16.466031646934,13.8267841057908,2.05470833333321));
#27187=CARTESIAN_POINT('Ctrl Pts',(17.4320632938681,14.3845227371939,2.01304166666654));
#27188=CARTESIAN_POINT('Ctrl Pts',(17.4320632938681,15.5000000000002,1.97137499999988));
#27189=CARTESIAN_POINT('Ctrl Pts',(17.4320632938681,16.6154772628064,1.92970833333321));
#27190=CARTESIAN_POINT('Ctrl Pts',(16.466031646934,17.1732158942095,1.88804166666654));
#27191=CARTESIAN_POINT('Ctrl Pts',(15.4999999999998,17.7309545256126,1.84637499999987));
#27192=CARTESIAN_POINT('Ctrl Pts',(14.5339683530657,17.1732158942095,1.80470833333321));
#27193=CARTESIAN_POINT('Ctrl Pts',(13.5679367061316,16.6154772628064,1.76304166666654));
#27194=CARTESIAN_POINT('Ctrl Pts',(13.5679367061316,15.5000000000001,1.72137499999987));
#27195=CARTESIAN_POINT('Ctrl Pts',(13.5679367061316,14.3845227371939,1.67970833333321));
#27196=CARTESIAN_POINT('Ctrl Pts',(14.5339683530657,13.8267841057908,1.63804166666654));
#27197=CARTESIAN_POINT('Ctrl Pts',(15.4999999999999,13.2690454743877,1.59637499999987));
#27198=CARTESIAN_POINT('Ctrl Pts',(16.466031646934,13.8267841057908,1.5547083333332));
#27199=CARTESIAN_POINT('Ctrl Pts',(17.4320632938681,14.3845227371939,1.51304166666654));
#27200=CARTESIAN_POINT('Ctrl Pts',(17.4320632938681,15.5000000000002,1.47137499999987));
#27201=CARTESIAN_POINT('Ctrl Pts',(17.4320632938681,16.6154772628064,1.4297083333332));
#27202=CARTESIAN_POINT('Ctrl Pts',(16.466031646934,17.1732158942095,1.38804166666653));
#27203=CARTESIAN_POINT('Ctrl Pts',(15.4999999999998,17.7309545256126,1.34637499999987));
#27204=CARTESIAN_POINT('Ctrl Pts',(14.5339683530657,17.1732158942095,1.3047083333332));
#27205=CARTESIAN_POINT('Ctrl Pts',(13.5679367061316,16.6154772628064,1.26304166666653));
#27206=CARTESIAN_POINT('Ctrl Pts',(13.5679367061316,15.5000000000001,1.22137499999987));
#27207=CARTESIAN_POINT('Ctrl Pts',(13.5679367061316,14.3845227371939,1.1797083333332));
#27208=CARTESIAN_POINT('Ctrl Pts',(14.5339683530657,13.8267841057908,1.13804166666653));
#27209=CARTESIAN_POINT('Ctrl Pts',(15.4999999999999,13.2690454743877,1.09637499999986));
#27210=CARTESIAN_POINT('Ctrl Pts',(16.466031646934,13.8267841057908,1.0547083333332));
#27211=CARTESIAN_POINT('Ctrl Pts',(17.4320632938681,14.3845227371939,1.01304166666653));
#27212=CARTESIAN_POINT('Ctrl Pts',(17.4320632938681,15.5000000000002,0.971374999999861));
#27213=CARTESIAN_POINT('Ctrl Pts',(17.4320632938681,16.6154772628064,0.929708333333194));
#27214=CARTESIAN_POINT('Ctrl Pts',(16.466031646934,17.1732158942095,0.888041666666528));
#27215=CARTESIAN_POINT('Ctrl Pts',(15.4999999999998,17.7309545256126,0.846374999999861));
#27216=CARTESIAN_POINT('Ctrl Pts',(14.5339683530657,17.1732158942095,0.804708333333194));
#27217=CARTESIAN_POINT('Ctrl Pts',(13.5679367061316,16.6154772628064,0.763041666666526));
#27218=CARTESIAN_POINT('Ctrl Pts',(13.5679367061316,15.5000000000001,0.721374999999859));
#27219=CARTESIAN_POINT('Ctrl Pts',(13.5679367061316,14.3845227371939,0.679708333333192));
#27220=CARTESIAN_POINT('Ctrl Pts',(14.5339683530657,13.8267841057908,0.638041666666525));
#27221=CARTESIAN_POINT('Ctrl Pts',(15.4999999999999,13.2690454743877,0.596374999999858));
#27222=CARTESIAN_POINT('Ctrl Pts',(16.466031646934,13.8267841057908,0.55470833333319));
#27223=CARTESIAN_POINT('Ctrl Pts',(17.4320632938681,14.3845227371939,0.513041666666523));
#27224=CARTESIAN_POINT('Ctrl Pts',(17.4320632938681,15.5000000000002,0.471374999999856));
#27225=CARTESIAN_POINT('Ctrl Pts',(17.4320632938681,16.6154772628064,0.429708333333188));
#27226=CARTESIAN_POINT('Ctrl Pts',(16.466031646934,17.1732158942095,0.388041666666521));
#27227=CARTESIAN_POINT('Ctrl Pts',(15.4999999999998,17.7309545256126,0.346374999999854));
#27228=CARTESIAN_POINT('Ctrl Pts',(14.5339683530657,17.1732158942095,0.304708333333186));
#27229=CARTESIAN_POINT('Ctrl Pts',(13.5679367061316,16.6154772628064,0.263041666666519));
#27230=CARTESIAN_POINT('Ctrl Pts',(13.5679367061316,15.5000000000001,0.221374999999852));
#27231=CARTESIAN_POINT('Ctrl Pts',(13.5679367061316,14.3845227371939,0.179708333333185));
#27232=CARTESIAN_POINT('Ctrl Pts',(14.5339683530657,13.8267841057908,0.138041666666517));
#27233=CARTESIAN_POINT('Ctrl Pts',(15.4999999999999,13.2690454743877,0.0963749999998501));
#27234=CARTESIAN_POINT('Ctrl Pts',(16.466031646934,13.8267841057908,0.0547083333331828));
#27235=CARTESIAN_POINT('Ctrl Pts',(17.4320632938681,14.3845227371939,0.0130416666665155));
#27236=CARTESIAN_POINT('Ctrl Pts',(17.4320632938681,15.5000000000002,-0.0286250000001518));
#27237=CARTESIAN_POINT('Ctrl Pts',(17.4320632938681,16.6154772628064,-0.0702916666668191));
#27238=CARTESIAN_POINT('Ctrl Pts',(16.466031646934,17.1732158942095,-0.111958333333486));
#27239=CARTESIAN_POINT('Ctrl Pts',(15.4999999999998,17.7309545256126,-0.153625000000154));
#27240=CARTESIAN_POINT('Ctrl Pts',(14.5339683530657,17.1732158942095,-0.195291666666821));
#27241=CARTESIAN_POINT('Ctrl Pts',(13.5679367061316,16.6154772628064,-0.236958333333488));
#27242=CARTESIAN_POINT('Ctrl Pts',(13.5679367061316,15.5000000000001,-0.278625000000155));
#27243=CARTESIAN_POINT('Ctrl Pts',(13.5679367061316,14.3845227371939,-0.320291666666821));
#27244=CARTESIAN_POINT('Ctrl Pts',(14.5339683530657,13.8267841057908,-0.361958333333488));
#27245=CARTESIAN_POINT('Ctrl Pts',(15.4999999999999,13.2690454743877,-0.403625000000156));
#27246=CARTESIAN_POINT('Ctrl Pts',(16.466031646934,13.8267841057908,-0.445291666666823));
#27247=CARTESIAN_POINT('Ctrl Pts',(17.4320632938681,14.3845227371939,-0.48695833333349));
#27248=CARTESIAN_POINT('Ctrl Pts',(17.4320632938681,15.5000000000002,-0.528625000000157));
#27249=CARTESIAN_POINT('Ctrl Pts',(17.4320632938681,16.6154772628064,-0.570291666666825));
#27250=CARTESIAN_POINT('Ctrl Pts',(16.466031646934,17.1732158942095,-0.611958333333492));
#27251=CARTESIAN_POINT('Ctrl Pts',(15.4999999999998,17.7309545256126,-0.653625000000159));
#27252=CARTESIAN_POINT('Ctrl Pts',(14.5339683530657,17.1732158942095,-0.695291666666827));
#27253=CARTESIAN_POINT('Ctrl Pts',(13.5679367061316,16.6154772628064,-0.736958333333494));
#27254=CARTESIAN_POINT('Ctrl Pts',(13.5679367061316,15.5000000000001,-0.778625000000161));
#27255=CARTESIAN_POINT('Ctrl Pts',(13.5679367061316,14.3845227371939,-0.820291666666829));
#27256=CARTESIAN_POINT('Ctrl Pts',(14.5339683530657,13.8267841057908,-0.861958333333496));
#27257=CARTESIAN_POINT('Ctrl Pts',(15.4999999999999,13.2690454743877,-0.903625000000163));
#27258=CARTESIAN_POINT('Ctrl Pts',(16.466031646934,13.8267841057908,-0.94529166666683));
#27259=CARTESIAN_POINT('Ctrl Pts',(17.4320632938681,14.3845227371939,-0.986958333333498));
#27260=CARTESIAN_POINT('Ctrl Pts',(17.4320632938681,15.5000000000002,-1.02862500000016));
#27261=CARTESIAN_POINT('Ctrl Pts',(17.4320632938681,16.6154772628064,-1.07029166666683));
#27262=CARTESIAN_POINT('Ctrl Pts',(16.466031646934,17.1732158942095,-1.1119583333335));
#27263=CARTESIAN_POINT('Ctrl Pts',(15.4999999999998,17.7309545256126,-1.15362500000017));
#27264=CARTESIAN_POINT('Ctrl Pts',(14.5339683530657,17.1732158942095,-1.19529166666683));
#27265=CARTESIAN_POINT('Ctrl Pts',(13.5679367061316,16.6154772628064,-1.2369583333335));
#27266=CARTESIAN_POINT('Ctrl Pts',(13.5679367061316,15.5000000000001,-1.27862500000017));
#27267=CARTESIAN_POINT('Ctrl Pts',(13.5679367061316,14.3845227371939,-1.32029166666684));
#27268=CARTESIAN_POINT('Ctrl Pts',(14.5339683530657,13.8267841057908,-1.3619583333335));
#27269=CARTESIAN_POINT('Ctrl Pts',(15.4999999999999,13.2690454743877,-1.40362500000017));
#27270=CARTESIAN_POINT('Ctrl Pts',(16.466031646934,13.8267841057908,-1.44529166666684));
#27271=CARTESIAN_POINT('Ctrl Pts',(17.4320632938681,14.3845227371939,-1.4869583333335));
#27272=CARTESIAN_POINT('Ctrl Pts',(17.4320632938681,15.5000000000002,-1.52862500000017));
#27273=CARTESIAN_POINT('Ctrl Pts',(17.4320632938681,16.6154772628064,-1.57029166666684));
#27274=CARTESIAN_POINT('Ctrl Pts',(16.466031646934,17.1732158942095,-1.61195833333351));
#27275=CARTESIAN_POINT('Ctrl Pts',(15.4999999999998,17.7309545256126,-1.65362500000017));
#27276=CARTESIAN_POINT('Ctrl Pts',(14.5339683530657,17.1732158942095,-1.69529166666684));
#27277=CARTESIAN_POINT('Ctrl Pts',(13.5679367061316,16.6154772628064,-1.73695833333351));
#27278=CARTESIAN_POINT('Ctrl Pts',(13.5679367061316,15.5000000000001,-1.77862500000017));
#27279=CARTESIAN_POINT('Ctrl Pts',(13.5679367061316,14.3845227371939,-1.82029166666684));
#27280=CARTESIAN_POINT('Ctrl Pts',(14.5339683530657,13.8267841057908,-1.86195833333351));
#27281=CARTESIAN_POINT('Ctrl Pts',(15.4999999999999,13.2690454743877,-1.90362500000018));
#27282=CARTESIAN_POINT('Ctrl Pts',(16.466031646934,13.8267841057908,-1.94529166666684));
#27283=CARTESIAN_POINT('Ctrl Pts',(17.4320632938681,14.3845227371939,-1.98695833333351));
#27284=CARTESIAN_POINT('Ctrl Pts',(17.4320632938681,15.5000000000002,-2.02862500000018));
#27285=CARTESIAN_POINT('Ctrl Pts',(17.4320632938681,16.6154772628064,-2.07029166666685));
#27286=CARTESIAN_POINT('Ctrl Pts',(16.466031646934,17.1732158942095,-2.11195833333351));
#27287=CARTESIAN_POINT('Ctrl Pts',(15.4999999999998,17.7309545256126,-2.15362500000018));
#27288=CARTESIAN_POINT('Ctrl Pts',(14.5339683530657,17.1732158942095,-2.19529166666685));
#27289=CARTESIAN_POINT('Ctrl Pts',(14.1783071398502,16.9678747970192,-2.21063196867905));
#27290=CARTESIAN_POINT('Ctrl Pts',(13.9369173167912,16.6356236599185,-2.22824840486548));
#27291=CARTESIAN_POINT('',(14.2215513317124,16.4288320706155,-2.02512305032131));
#27292=CARTESIAN_POINT('Ctrl Pts',(13.9406917842495,15.2436450846259,10.4122404735808));
#27293=CARTESIAN_POINT('Ctrl Pts',(14.0620451873461,14.5054990725559,10.3753299573543));
#27294=CARTESIAN_POINT('Ctrl Pts',(14.7098797632094,14.1314716057908,10.3411666666667));
#27295=CARTESIAN_POINT('Ctrl Pts',(15.4999999999999,13.6752954743877,10.2995));
#27296=CARTESIAN_POINT('Ctrl Pts',(16.2901202367903,14.1314716057908,10.2578333333333));
#27297=CARTESIAN_POINT('Ctrl Pts',(17.0802404735807,14.5876477371939,10.2161666666667));
#27298=CARTESIAN_POINT('Ctrl Pts',(17.0802404735807,15.5000000000002,10.1745));
#27299=CARTESIAN_POINT('Ctrl Pts',(17.0802404735807,16.4123522628064,10.1328333333333));
#27300=CARTESIAN_POINT('Ctrl Pts',(16.2901202367902,16.8685283942095,10.0911666666667));
#27301=CARTESIAN_POINT('Ctrl Pts',(15.4999999999998,17.3247045256126,10.0495));
#27302=CARTESIAN_POINT('Ctrl Pts',(14.7098797632094,16.8685283942095,10.0078333333333));
#27303=CARTESIAN_POINT('Ctrl Pts',(13.919759526419,16.4123522628064,9.96616666666665));
#27304=CARTESIAN_POINT('Ctrl Pts',(13.919759526419,15.5000000000001,9.92449999999998));
#27305=CARTESIAN_POINT('Ctrl Pts',(13.919759526419,14.5876477371939,9.88283333333331));
#27306=CARTESIAN_POINT('Ctrl Pts',(14.7098797632094,14.1314716057908,9.84116666666665));
#27307=CARTESIAN_POINT('Ctrl Pts',(15.4999999999999,13.6752954743877,9.79949999999998));
#27308=CARTESIAN_POINT('Ctrl Pts',(16.2901202367903,14.1314716057908,9.75783333333331));
#27309=CARTESIAN_POINT('Ctrl Pts',(17.0802404735807,14.5876477371939,9.71616666666665));
#27310=CARTESIAN_POINT('Ctrl Pts',(17.0802404735807,15.5000000000002,9.67449999999998));
#27311=CARTESIAN_POINT('Ctrl Pts',(17.0802404735807,16.4123522628064,9.63283333333331));
#27312=CARTESIAN_POINT('Ctrl Pts',(16.2901202367902,16.8685283942095,9.59116666666664));
#27313=CARTESIAN_POINT('Ctrl Pts',(15.4999999999998,17.3247045256126,9.54949999999998));
#27314=CARTESIAN_POINT('Ctrl Pts',(14.7098797632094,16.8685283942095,9.50783333333331));
#27315=CARTESIAN_POINT('Ctrl Pts',(13.919759526419,16.4123522628064,9.46616666666664));
#27316=CARTESIAN_POINT('Ctrl Pts',(13.919759526419,15.5000000000001,9.42449999999998));
#27317=CARTESIAN_POINT('Ctrl Pts',(13.919759526419,14.5876477371939,9.38283333333331));
#27318=CARTESIAN_POINT('Ctrl Pts',(14.7098797632094,14.1314716057908,9.34116666666664));
#27319=CARTESIAN_POINT('Ctrl Pts',(15.4999999999999,13.6752954743877,9.29949999999997));
#27320=CARTESIAN_POINT('Ctrl Pts',(16.2901202367903,14.1314716057908,9.25783333333331));
#27321=CARTESIAN_POINT('Ctrl Pts',(17.0802404735807,14.5876477371939,9.21616666666664));
#27322=CARTESIAN_POINT('Ctrl Pts',(17.0802404735807,15.5000000000002,9.17449999999997));
#27323=CARTESIAN_POINT('Ctrl Pts',(17.0802404735807,16.4123522628064,9.13283333333331));
#27324=CARTESIAN_POINT('Ctrl Pts',(16.2901202367902,16.8685283942095,9.09116666666664));
#27325=CARTESIAN_POINT('Ctrl Pts',(15.4999999999998,17.3247045256126,9.04949999999997));
#27326=CARTESIAN_POINT('Ctrl Pts',(14.7098797632094,16.8685283942095,9.0078333333333));
#27327=CARTESIAN_POINT('Ctrl Pts',(13.919759526419,16.4123522628064,8.96616666666664));
#27328=CARTESIAN_POINT('Ctrl Pts',(13.919759526419,15.5000000000001,8.92449999999997));
#27329=CARTESIAN_POINT('Ctrl Pts',(13.919759526419,14.5876477371939,8.8828333333333));
#27330=CARTESIAN_POINT('Ctrl Pts',(14.7098797632094,14.1314716057908,8.84116666666664));
#27331=CARTESIAN_POINT('Ctrl Pts',(15.4999999999999,13.6752954743877,8.79949999999997));
#27332=CARTESIAN_POINT('Ctrl Pts',(16.2901202367903,14.1314716057908,8.7578333333333));
#27333=CARTESIAN_POINT('Ctrl Pts',(17.0802404735807,14.5876477371939,8.71616666666663));
#27334=CARTESIAN_POINT('Ctrl Pts',(17.0802404735807,15.5000000000002,8.67449999999997));
#27335=CARTESIAN_POINT('Ctrl Pts',(17.0802404735807,16.4123522628064,8.6328333333333));
#27336=CARTESIAN_POINT('Ctrl Pts',(16.2901202367902,16.8685283942095,8.59116666666663));
#27337=CARTESIAN_POINT('Ctrl Pts',(15.4999999999998,17.3247045256126,8.54949999999996));
#27338=CARTESIAN_POINT('Ctrl Pts',(14.7098797632094,16.8685283942095,8.50783333333329));
#27339=CARTESIAN_POINT('Ctrl Pts',(13.919759526419,16.4123522628064,8.46616666666663));
#27340=CARTESIAN_POINT('Ctrl Pts',(13.919759526419,15.5000000000001,8.42449999999996));
#27341=CARTESIAN_POINT('Ctrl Pts',(13.919759526419,14.5876477371939,8.38283333333329));
#27342=CARTESIAN_POINT('Ctrl Pts',(14.7098797632094,14.1314716057908,8.34116666666663));
#27343=CARTESIAN_POINT('Ctrl Pts',(15.4999999999999,13.6752954743877,8.29949999999996));
#27344=CARTESIAN_POINT('Ctrl Pts',(16.2901202367903,14.1314716057908,8.25783333333329));
#27345=CARTESIAN_POINT('Ctrl Pts',(17.0802404735807,14.5876477371939,8.21616666666663));
#27346=CARTESIAN_POINT('Ctrl Pts',(17.0802404735807,15.5000000000002,8.17449999999996));
#27347=CARTESIAN_POINT('Ctrl Pts',(17.0802404735807,16.4123522628064,8.13283333333329));
#27348=CARTESIAN_POINT('Ctrl Pts',(16.2901202367902,16.8685283942095,8.09116666666663));
#27349=CARTESIAN_POINT('Ctrl Pts',(15.4999999999998,17.3247045256126,8.04949999999996));
#27350=CARTESIAN_POINT('Ctrl Pts',(14.7098797632094,16.8685283942095,8.00783333333329));
#27351=CARTESIAN_POINT('Ctrl Pts',(13.919759526419,16.4123522628064,7.96616666666662));
#27352=CARTESIAN_POINT('Ctrl Pts',(13.919759526419,15.5000000000001,7.92449999999996));
#27353=CARTESIAN_POINT('Ctrl Pts',(13.919759526419,14.5876477371939,7.88283333333329));
#27354=CARTESIAN_POINT('Ctrl Pts',(14.7098797632094,14.1314716057908,7.84116666666662));
#27355=CARTESIAN_POINT('Ctrl Pts',(15.4999999999999,13.6752954743877,7.79949999999995));
#27356=CARTESIAN_POINT('Ctrl Pts',(16.2901202367903,14.1314716057908,7.75783333333329));
#27357=CARTESIAN_POINT('Ctrl Pts',(17.0802404735807,14.5876477371939,7.71616666666662));
#27358=CARTESIAN_POINT('Ctrl Pts',(17.0802404735807,15.5000000000002,7.67449999999995));
#27359=CARTESIAN_POINT('Ctrl Pts',(17.0802404735807,16.4123522628064,7.63283333333328));
#27360=CARTESIAN_POINT('Ctrl Pts',(16.2901202367902,16.8685283942095,7.59116666666662));
#27361=CARTESIAN_POINT('Ctrl Pts',(15.4999999999998,17.3247045256126,7.54949999999995));
#27362=CARTESIAN_POINT('Ctrl Pts',(14.7098797632094,16.8685283942095,7.50783333333328));
#27363=CARTESIAN_POINT('Ctrl Pts',(13.919759526419,16.4123522628064,7.46616666666662));
#27364=CARTESIAN_POINT('Ctrl Pts',(13.919759526419,15.5000000000001,7.42449999999995));
#27365=CARTESIAN_POINT('Ctrl Pts',(13.919759526419,14.5876477371939,7.38283333333328));
#27366=CARTESIAN_POINT('Ctrl Pts',(14.7098797632094,14.1314716057908,7.34116666666661));
#27367=CARTESIAN_POINT('Ctrl Pts',(15.4999999999999,13.6752954743877,7.29949999999995));
#27368=CARTESIAN_POINT('Ctrl Pts',(16.2901202367903,14.1314716057908,7.25783333333328));
#27369=CARTESIAN_POINT('Ctrl Pts',(17.0802404735807,14.5876477371939,7.21616666666661));
#27370=CARTESIAN_POINT('Ctrl Pts',(17.0802404735807,15.5000000000002,7.17449999999995));
#27371=CARTESIAN_POINT('Ctrl Pts',(17.0802404735807,16.4123522628064,7.13283333333328));
#27372=CARTESIAN_POINT('Ctrl Pts',(16.2901202367902,16.8685283942095,7.09116666666661));
#27373=CARTESIAN_POINT('Ctrl Pts',(15.4999999999998,17.3247045256126,7.04949999999994));
#27374=CARTESIAN_POINT('Ctrl Pts',(14.7098797632094,16.8685283942095,7.00783333333328));
#27375=CARTESIAN_POINT('Ctrl Pts',(13.919759526419,16.4123522628064,6.96616666666661));
#27376=CARTESIAN_POINT('Ctrl Pts',(13.919759526419,15.5000000000001,6.92449999999994));
#27377=CARTESIAN_POINT('Ctrl Pts',(13.919759526419,14.5876477371939,6.88283333333327));
#27378=CARTESIAN_POINT('Ctrl Pts',(14.7098797632094,14.1314716057908,6.84116666666661));
#27379=CARTESIAN_POINT('Ctrl Pts',(15.4999999999999,13.6752954743877,6.79949999999994));
#27380=CARTESIAN_POINT('Ctrl Pts',(16.2901202367903,14.1314716057908,6.75783333333327));
#27381=CARTESIAN_POINT('Ctrl Pts',(17.0802404735807,14.5876477371939,6.71616666666661));
#27382=CARTESIAN_POINT('Ctrl Pts',(17.0802404735807,15.5000000000002,6.67449999999994));
#27383=CARTESIAN_POINT('Ctrl Pts',(17.0802404735807,16.4123522628064,6.63283333333327));
#27384=CARTESIAN_POINT('Ctrl Pts',(16.2901202367902,16.8685283942095,6.59116666666661));
#27385=CARTESIAN_POINT('Ctrl Pts',(15.4999999999998,17.3247045256126,6.54949999999994));
#27386=CARTESIAN_POINT('Ctrl Pts',(14.7098797632094,16.8685283942095,6.50783333333327));
#27387=CARTESIAN_POINT('Ctrl Pts',(13.919759526419,16.4123522628064,6.4661666666666));
#27388=CARTESIAN_POINT('Ctrl Pts',(13.919759526419,15.5000000000001,6.42449999999994));
#27389=CARTESIAN_POINT('Ctrl Pts',(13.919759526419,14.5876477371939,6.38283333333327));
#27390=CARTESIAN_POINT('Ctrl Pts',(14.7098797632094,14.1314716057908,6.3411666666666));
#27391=CARTESIAN_POINT('Ctrl Pts',(15.4999999999999,13.6752954743877,6.29949999999993));
#27392=CARTESIAN_POINT('Ctrl Pts',(16.2901202367903,14.1314716057908,6.25783333333327));
#27393=CARTESIAN_POINT('Ctrl Pts',(17.0802404735807,14.5876477371939,6.2161666666666));
#27394=CARTESIAN_POINT('Ctrl Pts',(17.0802404735807,15.5000000000002,6.17449999999993));
#27395=CARTESIAN_POINT('Ctrl Pts',(17.0802404735807,16.4123522628064,6.13283333333326));
#27396=CARTESIAN_POINT('Ctrl Pts',(16.2901202367902,16.8685283942095,6.0911666666666));
#27397=CARTESIAN_POINT('Ctrl Pts',(15.4999999999998,17.3247045256126,6.04949999999993));
#27398=CARTESIAN_POINT('Ctrl Pts',(14.7098797632094,16.8685283942095,6.00783333333326));
#27399=CARTESIAN_POINT('Ctrl Pts',(13.919759526419,16.4123522628064,5.9661666666666));
#27400=CARTESIAN_POINT('Ctrl Pts',(13.919759526419,15.5000000000001,5.92449999999993));
#27401=CARTESIAN_POINT('Ctrl Pts',(13.919759526419,14.5876477371939,5.88283333333326));
#27402=CARTESIAN_POINT('Ctrl Pts',(14.7098797632094,14.1314716057908,5.8411666666666));
#27403=CARTESIAN_POINT('Ctrl Pts',(15.4999999999999,13.6752954743877,5.79949999999993));
#27404=CARTESIAN_POINT('Ctrl Pts',(16.2901202367903,14.1314716057908,5.75783333333326));
#27405=CARTESIAN_POINT('Ctrl Pts',(17.0802404735807,14.5876477371939,5.71616666666659));
#27406=CARTESIAN_POINT('Ctrl Pts',(17.0802404735807,15.5000000000002,5.67449999999993));
#27407=CARTESIAN_POINT('Ctrl Pts',(17.0802404735807,16.4123522628064,5.63283333333326));
#27408=CARTESIAN_POINT('Ctrl Pts',(16.2901202367902,16.8685283942095,5.59116666666659));
#27409=CARTESIAN_POINT('Ctrl Pts',(15.4999999999998,17.3247045256126,5.54949999999992));
#27410=CARTESIAN_POINT('Ctrl Pts',(14.7098797632094,16.8685283942095,5.50783333333326));
#27411=CARTESIAN_POINT('Ctrl Pts',(13.919759526419,16.4123522628064,5.46616666666659));
#27412=CARTESIAN_POINT('Ctrl Pts',(13.919759526419,15.5000000000001,5.42449999999992));
#27413=CARTESIAN_POINT('Ctrl Pts',(13.919759526419,14.5876477371939,5.38283333333326));
#27414=CARTESIAN_POINT('Ctrl Pts',(14.7098797632094,14.1314716057908,5.34116666666659));
#27415=CARTESIAN_POINT('Ctrl Pts',(15.4999999999999,13.6752954743877,5.29949999999992));
#27416=CARTESIAN_POINT('Ctrl Pts',(16.2901202367903,14.1314716057908,5.25783333333325));
#27417=CARTESIAN_POINT('Ctrl Pts',(17.0802404735807,14.5876477371939,5.21616666666659));
#27418=CARTESIAN_POINT('Ctrl Pts',(17.0802404735807,15.5000000000002,5.17449999999992));
#27419=CARTESIAN_POINT('Ctrl Pts',(17.0802404735807,16.4123522628064,5.13283333333325));
#27420=CARTESIAN_POINT('Ctrl Pts',(16.2901202367902,16.8685283942095,5.09116666666658));
#27421=CARTESIAN_POINT('Ctrl Pts',(15.4999999999998,17.3247045256126,5.04949999999992));
#27422=CARTESIAN_POINT('Ctrl Pts',(14.7098797632094,16.8685283942095,5.00783333333325));
#27423=CARTESIAN_POINT('Ctrl Pts',(13.919759526419,16.4123522628064,4.96616666666658));
#27424=CARTESIAN_POINT('Ctrl Pts',(13.919759526419,15.5000000000001,4.92449999999992));
#27425=CARTESIAN_POINT('Ctrl Pts',(13.919759526419,14.5876477371939,4.88283333333325));
#27426=CARTESIAN_POINT('Ctrl Pts',(14.7098797632094,14.1314716057908,4.84116666666658));
#27427=CARTESIAN_POINT('Ctrl Pts',(15.4999999999999,13.6752954743877,4.79949999999991));
#27428=CARTESIAN_POINT('Ctrl Pts',(16.2901202367903,14.1314716057908,4.75783333333325));
#27429=CARTESIAN_POINT('Ctrl Pts',(17.0802404735807,14.5876477371939,4.71616666666658));
#27430=CARTESIAN_POINT('Ctrl Pts',(17.0802404735807,15.5000000000002,4.67449999999991));
#27431=CARTESIAN_POINT('Ctrl Pts',(17.0802404735807,16.4123522628064,4.63283333333325));
#27432=CARTESIAN_POINT('Ctrl Pts',(16.2901202367902,16.8685283942095,4.59116666666658));
#27433=CARTESIAN_POINT('Ctrl Pts',(15.4999999999998,17.3247045256126,4.54949999999991));
#27434=CARTESIAN_POINT('Ctrl Pts',(14.7098797632094,16.8685283942095,4.50783333333324));
#27435=CARTESIAN_POINT('Ctrl Pts',(13.919759526419,16.4123522628064,4.46616666666658));
#27436=CARTESIAN_POINT('Ctrl Pts',(13.919759526419,15.5000000000001,4.42449999999991));
#27437=CARTESIAN_POINT('Ctrl Pts',(13.919759526419,14.5876477371939,4.38283333333324));
#27438=CARTESIAN_POINT('Ctrl Pts',(14.7098797632094,14.1314716057908,4.34116666666657));
#27439=CARTESIAN_POINT('Ctrl Pts',(15.4999999999999,13.6752954743877,4.29949999999991));
#27440=CARTESIAN_POINT('Ctrl Pts',(16.2901202367903,14.1314716057908,4.25783333333324));
#27441=CARTESIAN_POINT('Ctrl Pts',(17.0802404735807,14.5876477371939,4.21616666666657));
#27442=CARTESIAN_POINT('Ctrl Pts',(17.0802404735807,15.5000000000002,4.17449999999991));
#27443=CARTESIAN_POINT('Ctrl Pts',(17.0802404735807,16.4123522628064,4.13283333333324));
#27444=CARTESIAN_POINT('Ctrl Pts',(16.2901202367902,16.8685283942095,4.09116666666657));
#27445=CARTESIAN_POINT('Ctrl Pts',(15.4999999999998,17.3247045256126,4.0494999999999));
#27446=CARTESIAN_POINT('Ctrl Pts',(14.7098797632094,16.8685283942095,4.00783333333324));
#27447=CARTESIAN_POINT('Ctrl Pts',(13.919759526419,16.4123522628064,3.96616666666657));
#27448=CARTESIAN_POINT('Ctrl Pts',(13.919759526419,15.5000000000001,3.9244999999999));
#27449=CARTESIAN_POINT('Ctrl Pts',(13.919759526419,14.5876477371939,3.88283333333323));
#27450=CARTESIAN_POINT('Ctrl Pts',(14.7098797632094,14.1314716057908,3.84116666666657));
#27451=CARTESIAN_POINT('Ctrl Pts',(15.4999999999999,13.6752954743877,3.7994999999999));
#27452=CARTESIAN_POINT('Ctrl Pts',(16.2901202367903,14.1314716057908,3.75783333333323));
#27453=CARTESIAN_POINT('Ctrl Pts',(17.0802404735807,14.5876477371939,3.71616666666657));
#27454=CARTESIAN_POINT('Ctrl Pts',(17.0802404735807,15.5000000000002,3.6744999999999));
#27455=CARTESIAN_POINT('Ctrl Pts',(17.0802404735807,16.4123522628064,3.63283333333323));
#27456=CARTESIAN_POINT('Ctrl Pts',(16.2901202367902,16.8685283942095,3.59116666666656));
#27457=CARTESIAN_POINT('Ctrl Pts',(15.4999999999998,17.3247045256126,3.5494999999999));
#27458=CARTESIAN_POINT('Ctrl Pts',(14.7098797632094,16.8685283942095,3.50783333333323));
#27459=CARTESIAN_POINT('Ctrl Pts',(13.919759526419,16.4123522628064,3.46616666666656));
#27460=CARTESIAN_POINT('Ctrl Pts',(13.919759526419,15.5000000000001,3.4244999999999));
#27461=CARTESIAN_POINT('Ctrl Pts',(13.919759526419,14.5876477371939,3.38283333333323));
#27462=CARTESIAN_POINT('Ctrl Pts',(14.7098797632094,14.1314716057908,3.34116666666656));
#27463=CARTESIAN_POINT('Ctrl Pts',(15.4999999999999,13.6752954743877,3.29949999999989));
#27464=CARTESIAN_POINT('Ctrl Pts',(16.2901202367903,14.1314716057908,3.25783333333323));
#27465=CARTESIAN_POINT('Ctrl Pts',(17.0802404735807,14.5876477371939,3.21616666666656));
#27466=CARTESIAN_POINT('Ctrl Pts',(17.0802404735807,15.5000000000002,3.17449999999989));
#27467=CARTESIAN_POINT('Ctrl Pts',(17.0802404735807,16.4123522628064,3.13283333333323));
#27468=CARTESIAN_POINT('Ctrl Pts',(16.2901202367902,16.8685283942095,3.09116666666656));
#27469=CARTESIAN_POINT('Ctrl Pts',(15.4999999999998,17.3247045256126,3.04949999999989));
#27470=CARTESIAN_POINT('Ctrl Pts',(14.7098797632094,16.8685283942095,3.00783333333322));
#27471=CARTESIAN_POINT('Ctrl Pts',(13.919759526419,16.4123522628064,2.96616666666656));
#27472=CARTESIAN_POINT('Ctrl Pts',(13.919759526419,15.5000000000001,2.92449999999989));
#27473=CARTESIAN_POINT('Ctrl Pts',(13.919759526419,14.5876477371939,2.88283333333322));
#27474=CARTESIAN_POINT('Ctrl Pts',(14.7098797632094,14.1314716057908,2.84116666666655));
#27475=CARTESIAN_POINT('Ctrl Pts',(15.4999999999999,13.6752954743877,2.79949999999989));
#27476=CARTESIAN_POINT('Ctrl Pts',(16.2901202367903,14.1314716057908,2.75783333333322));
#27477=CARTESIAN_POINT('Ctrl Pts',(17.0802404735807,14.5876477371939,2.71616666666655));
#27478=CARTESIAN_POINT('Ctrl Pts',(17.0802404735807,15.5000000000002,2.67449999999989));
#27479=CARTESIAN_POINT('Ctrl Pts',(17.0802404735807,16.4123522628064,2.63283333333322));
#27480=CARTESIAN_POINT('Ctrl Pts',(16.2901202367902,16.8685283942095,2.59116666666655));
#27481=CARTESIAN_POINT('Ctrl Pts',(15.4999999999998,17.3247045256126,2.54949999999988));
#27482=CARTESIAN_POINT('Ctrl Pts',(14.7098797632094,16.8685283942095,2.50783333333322));
#27483=CARTESIAN_POINT('Ctrl Pts',(13.919759526419,16.4123522628064,2.46616666666655));
#27484=CARTESIAN_POINT('Ctrl Pts',(13.919759526419,15.5000000000001,2.42449999999988));
#27485=CARTESIAN_POINT('Ctrl Pts',(13.919759526419,14.5876477371939,2.38283333333321));
#27486=CARTESIAN_POINT('Ctrl Pts',(14.7098797632094,14.1314716057908,2.34116666666655));
#27487=CARTESIAN_POINT('Ctrl Pts',(15.4999999999999,13.6752954743877,2.29949999999988));
#27488=CARTESIAN_POINT('Ctrl Pts',(16.2901202367903,14.1314716057908,2.25783333333321));
#27489=CARTESIAN_POINT('Ctrl Pts',(17.0802404735807,14.5876477371939,2.21616666666655));
#27490=CARTESIAN_POINT('Ctrl Pts',(17.0802404735807,15.5000000000002,2.17449999999988));
#27491=CARTESIAN_POINT('Ctrl Pts',(17.0802404735807,16.4123522628064,2.13283333333321));
#27492=CARTESIAN_POINT('Ctrl Pts',(16.2901202367902,16.8685283942095,2.09116666666655));
#27493=CARTESIAN_POINT('Ctrl Pts',(15.4999999999998,17.3247045256126,2.04949999999988));
#27494=CARTESIAN_POINT('Ctrl Pts',(14.7098797632094,16.8685283942095,2.00783333333321));
#27495=CARTESIAN_POINT('Ctrl Pts',(13.919759526419,16.4123522628064,1.96616666666654));
#27496=CARTESIAN_POINT('Ctrl Pts',(13.919759526419,15.5000000000001,1.92449999999988));
#27497=CARTESIAN_POINT('Ctrl Pts',(13.919759526419,14.5876477371939,1.88283333333321));
#27498=CARTESIAN_POINT('Ctrl Pts',(14.7098797632094,14.1314716057908,1.84116666666654));
#27499=CARTESIAN_POINT('Ctrl Pts',(15.4999999999999,13.6752954743877,1.79949999999987));
#27500=CARTESIAN_POINT('Ctrl Pts',(16.2901202367903,14.1314716057908,1.75783333333321));
#27501=CARTESIAN_POINT('Ctrl Pts',(17.0802404735807,14.5876477371939,1.71616666666654));
#27502=CARTESIAN_POINT('Ctrl Pts',(17.0802404735807,15.5000000000002,1.67449999999987));
#27503=CARTESIAN_POINT('Ctrl Pts',(17.0802404735807,16.4123522628064,1.63283333333321));
#27504=CARTESIAN_POINT('Ctrl Pts',(16.2901202367902,16.8685283942095,1.59116666666654));
#27505=CARTESIAN_POINT('Ctrl Pts',(15.4999999999998,17.3247045256126,1.54949999999987));
#27506=CARTESIAN_POINT('Ctrl Pts',(14.7098797632094,16.8685283942095,1.5078333333332));
#27507=CARTESIAN_POINT('Ctrl Pts',(13.919759526419,16.4123522628064,1.46616666666654));
#27508=CARTESIAN_POINT('Ctrl Pts',(13.919759526419,15.5000000000001,1.42449999999987));
#27509=CARTESIAN_POINT('Ctrl Pts',(13.919759526419,14.5876477371939,1.3828333333332));
#27510=CARTESIAN_POINT('Ctrl Pts',(14.7098797632094,14.1314716057908,1.34116666666653));
#27511=CARTESIAN_POINT('Ctrl Pts',(15.4999999999999,13.6752954743877,1.29949999999987));
#27512=CARTESIAN_POINT('Ctrl Pts',(16.2901202367903,14.1314716057908,1.2578333333332));
#27513=CARTESIAN_POINT('Ctrl Pts',(17.0802404735807,14.5876477371939,1.21616666666653));
#27514=CARTESIAN_POINT('Ctrl Pts',(17.0802404735807,15.5000000000002,1.17449999999986));
#27515=CARTESIAN_POINT('Ctrl Pts',(17.0802404735807,16.4123522628064,1.1328333333332));
#27516=CARTESIAN_POINT('Ctrl Pts',(16.2901202367902,16.8685283942095,1.09116666666653));
#27517=CARTESIAN_POINT('Ctrl Pts',(15.4999999999998,17.3247045256126,1.04949999999987));
#27518=CARTESIAN_POINT('Ctrl Pts',(14.7098797632094,16.8685283942095,1.0078333333332));
#27519=CARTESIAN_POINT('Ctrl Pts',(13.919759526419,16.4123522628064,0.96616666666653));
#27520=CARTESIAN_POINT('Ctrl Pts',(13.919759526419,15.5000000000001,0.924499999999863));
#27521=CARTESIAN_POINT('Ctrl Pts',(13.919759526419,14.5876477371939,0.882833333333196));
#27522=CARTESIAN_POINT('Ctrl Pts',(14.7098797632094,14.1314716057908,0.841166666666529));
#27523=CARTESIAN_POINT('Ctrl Pts',(15.4999999999999,13.6752954743877,0.799499999999861));
#27524=CARTESIAN_POINT('Ctrl Pts',(16.2901202367903,14.1314716057908,0.757833333333194));
#27525=CARTESIAN_POINT('Ctrl Pts',(17.0802404735807,14.5876477371939,0.716166666666527));
#27526=CARTESIAN_POINT('Ctrl Pts',(17.0802404735807,15.5000000000002,0.674499999999859));
#27527=CARTESIAN_POINT('Ctrl Pts',(17.0802404735807,16.4123522628064,0.632833333333192));
#27528=CARTESIAN_POINT('Ctrl Pts',(16.2901202367902,16.8685283942095,0.591166666666525));
#27529=CARTESIAN_POINT('Ctrl Pts',(15.4999999999998,17.3247045256126,0.549499999999857));
#27530=CARTESIAN_POINT('Ctrl Pts',(14.7098797632094,16.8685283942095,0.50783333333319));
#27531=CARTESIAN_POINT('Ctrl Pts',(13.919759526419,16.4123522628064,0.466166666666523));
#27532=CARTESIAN_POINT('Ctrl Pts',(13.919759526419,15.5000000000001,0.424499999999856));
#27533=CARTESIAN_POINT('Ctrl Pts',(13.919759526419,14.5876477371939,0.382833333333188));
#27534=CARTESIAN_POINT('Ctrl Pts',(14.7098797632094,14.1314716057908,0.341166666666521));
#27535=CARTESIAN_POINT('Ctrl Pts',(15.4999999999999,13.6752954743877,0.299499999999854));
#27536=CARTESIAN_POINT('Ctrl Pts',(16.2901202367903,14.1314716057908,0.257833333333186));
#27537=CARTESIAN_POINT('Ctrl Pts',(17.0802404735807,14.5876477371939,0.216166666666519));
#27538=CARTESIAN_POINT('Ctrl Pts',(17.0802404735807,15.5000000000002,0.174499999999852));
#27539=CARTESIAN_POINT('Ctrl Pts',(17.0802404735807,16.4123522628064,0.132833333333185));
#27540=CARTESIAN_POINT('Ctrl Pts',(16.2901202367902,16.8685283942095,0.0911666666665173));
#27541=CARTESIAN_POINT('Ctrl Pts',(15.4999999999998,17.3247045256126,0.04949999999985));
#27542=CARTESIAN_POINT('Ctrl Pts',(14.7098797632094,16.8685283942095,0.00783333333318273));
#27543=CARTESIAN_POINT('Ctrl Pts',(13.919759526419,16.4123522628064,-0.0338333333334846));
#27544=CARTESIAN_POINT('Ctrl Pts',(13.919759526419,15.5000000000001,-0.0755000000001518));
#27545=CARTESIAN_POINT('Ctrl Pts',(13.919759526419,14.5876477371939,-0.117166666666817));
#27546=CARTESIAN_POINT('Ctrl Pts',(14.7098797632094,14.1314716057908,-0.158833333333485));
#27547=CARTESIAN_POINT('Ctrl Pts',(15.4999999999999,13.6752954743877,-0.200500000000152));
#27548=CARTESIAN_POINT('Ctrl Pts',(16.2901202367903,14.1314716057908,-0.242166666666819));
#27549=CARTESIAN_POINT('Ctrl Pts',(17.0802404735807,14.5876477371939,-0.283833333333487));
#27550=CARTESIAN_POINT('Ctrl Pts',(17.0802404735807,15.5000000000002,-0.325500000000154));
#27551=CARTESIAN_POINT('Ctrl Pts',(17.0802404735807,16.4123522628064,-0.367166666666821));
#27552=CARTESIAN_POINT('Ctrl Pts',(16.2901202367902,16.8685283942095,-0.408833333333488));
#27553=CARTESIAN_POINT('Ctrl Pts',(15.4999999999998,17.3247045256126,-0.450500000000156));
#27554=CARTESIAN_POINT('Ctrl Pts',(14.7098797632094,16.8685283942095,-0.492166666666823));
#27555=CARTESIAN_POINT('Ctrl Pts',(13.919759526419,16.4123522628064,-0.53383333333349));
#27556=CARTESIAN_POINT('Ctrl Pts',(13.919759526419,15.5000000000001,-0.575500000000157));
#27557=CARTESIAN_POINT('Ctrl Pts',(13.919759526419,14.5876477371939,-0.617166666666825));
#27558=CARTESIAN_POINT('Ctrl Pts',(14.7098797632094,14.1314716057908,-0.658833333333492));
#27559=CARTESIAN_POINT('Ctrl Pts',(15.4999999999999,13.6752954743877,-0.700500000000159));
#27560=CARTESIAN_POINT('Ctrl Pts',(16.2901202367903,14.1314716057908,-0.742166666666827));
#27561=CARTESIAN_POINT('Ctrl Pts',(17.0802404735807,14.5876477371939,-0.783833333333494));
#27562=CARTESIAN_POINT('Ctrl Pts',(17.0802404735807,15.5000000000002,-0.825500000000161));
#27563=CARTESIAN_POINT('Ctrl Pts',(17.0802404735807,16.4123522628064,-0.867166666666829));
#27564=CARTESIAN_POINT('Ctrl Pts',(16.2901202367902,16.8685283942095,-0.908833333333496));
#27565=CARTESIAN_POINT('Ctrl Pts',(15.4999999999998,17.3247045256126,-0.950500000000163));
#27566=CARTESIAN_POINT('Ctrl Pts',(14.7098797632094,16.8685283942095,-0.99216666666683));
#27567=CARTESIAN_POINT('Ctrl Pts',(13.919759526419,16.4123522628064,-1.0338333333335));
#27568=CARTESIAN_POINT('Ctrl Pts',(13.919759526419,15.5000000000001,-1.07550000000016));
#27569=CARTESIAN_POINT('Ctrl Pts',(13.919759526419,14.5876477371939,-1.11716666666683));
#27570=CARTESIAN_POINT('Ctrl Pts',(14.7098797632094,14.1314716057908,-1.1588333333335));
#27571=CARTESIAN_POINT('Ctrl Pts',(15.4999999999999,13.6752954743877,-1.20050000000017));
#27572=CARTESIAN_POINT('Ctrl Pts',(16.2901202367903,14.1314716057908,-1.24216666666683));
#27573=CARTESIAN_POINT('Ctrl Pts',(17.0802404735807,14.5876477371939,-1.2838333333335));
#27574=CARTESIAN_POINT('Ctrl Pts',(17.0802404735807,15.5000000000002,-1.32550000000017));
#27575=CARTESIAN_POINT('Ctrl Pts',(17.0802404735807,16.4123522628064,-1.36716666666683));
#27576=CARTESIAN_POINT('Ctrl Pts',(16.2901202367902,16.8685283942095,-1.4088333333335));
#27577=CARTESIAN_POINT('Ctrl Pts',(15.4999999999998,17.3247045256126,-1.45050000000017));
#27578=CARTESIAN_POINT('Ctrl Pts',(14.7098797632094,16.8685283942095,-1.49216666666684));
#27579=CARTESIAN_POINT('Ctrl Pts',(13.919759526419,16.4123522628064,-1.5338333333335));
#27580=CARTESIAN_POINT('Ctrl Pts',(13.919759526419,15.5000000000001,-1.57550000000017));
#27581=CARTESIAN_POINT('Ctrl Pts',(13.919759526419,14.5876477371939,-1.61716666666684));
#27582=CARTESIAN_POINT('Ctrl Pts',(14.7098797632094,14.1314716057908,-1.65883333333351));
#27583=CARTESIAN_POINT('Ctrl Pts',(15.4999999999999,13.6752954743877,-1.70050000000017));
#27584=CARTESIAN_POINT('Ctrl Pts',(16.2901202367903,14.1314716057908,-1.74216666666684));
#27585=CARTESIAN_POINT('Ctrl Pts',(17.0802404735807,14.5876477371939,-1.78383333333351));
#27586=CARTESIAN_POINT('Ctrl Pts',(17.0802404735807,15.5000000000002,-1.82550000000017));
#27587=CARTESIAN_POINT('Ctrl Pts',(17.0802404735807,16.4123522628064,-1.86716666666684));
#27588=CARTESIAN_POINT('Ctrl Pts',(16.2901202367902,16.8685283942095,-1.90883333333351));
#27589=CARTESIAN_POINT('Ctrl Pts',(15.4999999999998,17.3247045256126,-1.95050000000018));
#27590=CARTESIAN_POINT('Ctrl Pts',(14.7098797632094,16.8685283942095,-1.99216666666684));
#27591=CARTESIAN_POINT('Ctrl Pts',(14.4189900731848,16.7005831533693,-2.00750661517932));
#27592=CARTESIAN_POINT('Ctrl Pts',(14.2215542486878,16.4288360540163,-2.02512301646327));
#27593=CARTESIAN_POINT('',(13.9369173167912,16.6356236599185,-2.22824840486548));
#27594=CARTESIAN_POINT('Ctrl Pts',(17.4320632938681,15.5000000000002,11.440125));
#27595=CARTESIAN_POINT('Ctrl Pts',(17.4320632938681,16.6154772628064,11.3984583333333));
#27596=CARTESIAN_POINT('Ctrl Pts',(16.466031646934,17.1732158942095,11.3567916666667));
#27597=CARTESIAN_POINT('Ctrl Pts',(15.4999999999998,17.7309545256126,11.315125));
#27598=CARTESIAN_POINT('Ctrl Pts',(14.5339683530657,17.1732158942095,11.2734583333333));
#27599=CARTESIAN_POINT('Ctrl Pts',(13.5679367061316,16.6154772628064,11.2317916666667));
#27600=CARTESIAN_POINT('Ctrl Pts',(13.5679367061316,15.5000000000001,11.190125));
#27601=CARTESIAN_POINT('Ctrl Pts',(13.5679367061316,14.3845227371939,11.1484583333333));
#27602=CARTESIAN_POINT('Ctrl Pts',(14.5339683530657,13.8267841057908,11.1067916666667));
#27603=CARTESIAN_POINT('Ctrl Pts',(15.4999999999999,13.2690454743877,11.065125));
#27604=CARTESIAN_POINT('Ctrl Pts',(16.466031646934,13.8267841057908,11.0234583333333));
#27605=CARTESIAN_POINT('Ctrl Pts',(17.4320632938681,14.3845227371939,10.9817916666667));
#27606=CARTESIAN_POINT('Ctrl Pts',(17.4320632938681,15.5000000000002,10.940125));
#27607=CARTESIAN_POINT('Ctrl Pts',(17.4320632938681,16.6154772628064,10.8984583333333));
#27608=CARTESIAN_POINT('Ctrl Pts',(16.466031646934,17.1732158942095,10.8567916666667));
#27609=CARTESIAN_POINT('Ctrl Pts',(15.4999999999998,17.7309545256126,10.815125));
#27610=CARTESIAN_POINT('Ctrl Pts',(14.5339683530657,17.1732158942095,10.7734583333333));
#27611=CARTESIAN_POINT('Ctrl Pts',(13.5679367061316,16.6154772628064,10.7317916666667));
#27612=CARTESIAN_POINT('Ctrl Pts',(13.5679367061316,15.5000000000001,10.690125));
#27613=CARTESIAN_POINT('Ctrl Pts',(13.5679367061316,14.3845227371939,10.6484583333333));
#27614=CARTESIAN_POINT('Ctrl Pts',(14.5339683530657,13.8267841057908,10.6067916666667));
#27615=CARTESIAN_POINT('Ctrl Pts',(15.4999999999999,13.2690454743877,10.565125));
#27616=CARTESIAN_POINT('Ctrl Pts',(16.466031646934,13.8267841057908,10.5234583333333));
#27617=CARTESIAN_POINT('Ctrl Pts',(17.4320632938681,14.3845227371939,10.4817916666667));
#27618=CARTESIAN_POINT('Ctrl Pts',(17.4320632938681,15.5000000000002,10.440125));
#27619=CARTESIAN_POINT('Ctrl Pts',(17.4320632938681,16.6154772628064,10.3984583333333));
#27620=CARTESIAN_POINT('Ctrl Pts',(16.466031646934,17.1732158942095,10.3567916666667));
#27621=CARTESIAN_POINT('Ctrl Pts',(15.4999999999998,17.7309545256126,10.315125));
#27622=CARTESIAN_POINT('Ctrl Pts',(14.5339683530657,17.1732158942095,10.2734583333333));
#27623=CARTESIAN_POINT('Ctrl Pts',(13.5679367061316,16.6154772628064,10.2317916666667));
#27624=CARTESIAN_POINT('Ctrl Pts',(13.5679367061316,15.5000000000001,10.190125));
#27625=CARTESIAN_POINT('Ctrl Pts',(13.5679367061316,14.3845227371939,10.1484583333333));
#27626=CARTESIAN_POINT('Ctrl Pts',(14.5339683530657,13.8267841057908,10.1067916666666));
#27627=CARTESIAN_POINT('Ctrl Pts',(15.4999999999999,13.2690454743877,10.065125));
#27628=CARTESIAN_POINT('Ctrl Pts',(16.466031646934,13.8267841057908,10.0234583333333));
#27629=CARTESIAN_POINT('Ctrl Pts',(17.4320632938681,14.3845227371939,9.98179166666664));
#27630=CARTESIAN_POINT('Ctrl Pts',(17.4320632938681,15.5000000000002,9.94012499999998));
#27631=CARTESIAN_POINT('Ctrl Pts',(17.4320632938681,16.6154772628064,9.89845833333331));
#27632=CARTESIAN_POINT('Ctrl Pts',(16.466031646934,17.1732158942095,9.85679166666664));
#27633=CARTESIAN_POINT('Ctrl Pts',(15.4999999999998,17.7309545256126,9.81512499999998));
#27634=CARTESIAN_POINT('Ctrl Pts',(14.5339683530657,17.1732158942095,9.77345833333331));
#27635=CARTESIAN_POINT('Ctrl Pts',(13.5679367061316,16.6154772628064,9.73179166666664));
#27636=CARTESIAN_POINT('Ctrl Pts',(13.5679367061316,15.5000000000001,9.69012499999998));
#27637=CARTESIAN_POINT('Ctrl Pts',(13.5679367061316,14.3845227371939,9.64845833333331));
#27638=CARTESIAN_POINT('Ctrl Pts',(14.5339683530657,13.8267841057908,9.60679166666664));
#27639=CARTESIAN_POINT('Ctrl Pts',(15.4999999999999,13.2690454743877,9.56512499999998));
#27640=CARTESIAN_POINT('Ctrl Pts',(16.466031646934,13.8267841057908,9.52345833333331));
#27641=CARTESIAN_POINT('Ctrl Pts',(17.4320632938681,14.3845227371939,9.48179166666664));
#27642=CARTESIAN_POINT('Ctrl Pts',(17.4320632938681,15.5000000000002,9.44012499999997));
#27643=CARTESIAN_POINT('Ctrl Pts',(17.4320632938681,16.6154772628064,9.39845833333331));
#27644=CARTESIAN_POINT('Ctrl Pts',(16.466031646934,17.1732158942095,9.35679166666664));
#27645=CARTESIAN_POINT('Ctrl Pts',(15.4999999999998,17.7309545256126,9.31512499999997));
#27646=CARTESIAN_POINT('Ctrl Pts',(14.5339683530657,17.1732158942095,9.2734583333333));
#27647=CARTESIAN_POINT('Ctrl Pts',(13.5679367061316,16.6154772628064,9.23179166666664));
#27648=CARTESIAN_POINT('Ctrl Pts',(13.5679367061316,15.5000000000001,9.19012499999997));
#27649=CARTESIAN_POINT('Ctrl Pts',(13.5679367061316,14.3845227371939,9.1484583333333));
#27650=CARTESIAN_POINT('Ctrl Pts',(14.5339683530657,13.8267841057908,9.10679166666664));
#27651=CARTESIAN_POINT('Ctrl Pts',(15.4999999999999,13.2690454743877,9.06512499999997));
#27652=CARTESIAN_POINT('Ctrl Pts',(16.466031646934,13.8267841057908,9.0234583333333));
#27653=CARTESIAN_POINT('Ctrl Pts',(17.4320632938681,14.3845227371939,8.98179166666663));
#27654=CARTESIAN_POINT('Ctrl Pts',(17.4320632938681,15.5000000000002,8.94012499999997));
#27655=CARTESIAN_POINT('Ctrl Pts',(17.4320632938681,16.6154772628064,8.8984583333333));
#27656=CARTESIAN_POINT('Ctrl Pts',(16.466031646934,17.1732158942095,8.85679166666663));
#27657=CARTESIAN_POINT('Ctrl Pts',(15.4999999999998,17.7309545256126,8.81512499999996));
#27658=CARTESIAN_POINT('Ctrl Pts',(14.5339683530657,17.1732158942095,8.7734583333333));
#27659=CARTESIAN_POINT('Ctrl Pts',(13.5679367061316,16.6154772628064,8.73179166666663));
#27660=CARTESIAN_POINT('Ctrl Pts',(13.5679367061316,15.5000000000001,8.69012499999996));
#27661=CARTESIAN_POINT('Ctrl Pts',(13.5679367061316,14.3845227371939,8.64845833333329));
#27662=CARTESIAN_POINT('Ctrl Pts',(14.5339683530657,13.8267841057908,8.60679166666663));
#27663=CARTESIAN_POINT('Ctrl Pts',(15.4999999999999,13.2690454743877,8.56512499999996));
#27664=CARTESIAN_POINT('Ctrl Pts',(16.466031646934,13.8267841057908,8.52345833333329));
#27665=CARTESIAN_POINT('Ctrl Pts',(17.4320632938681,14.3845227371939,8.48179166666663));
#27666=CARTESIAN_POINT('Ctrl Pts',(17.4320632938681,15.5000000000002,8.44012499999996));
#27667=CARTESIAN_POINT('Ctrl Pts',(17.4320632938681,16.6154772628064,8.39845833333329));
#27668=CARTESIAN_POINT('Ctrl Pts',(16.466031646934,17.1732158942095,8.35679166666662));
#27669=CARTESIAN_POINT('Ctrl Pts',(15.4999999999998,17.7309545256126,8.31512499999996));
#27670=CARTESIAN_POINT('Ctrl Pts',(14.5339683530657,17.1732158942095,8.27345833333329));
#27671=CARTESIAN_POINT('Ctrl Pts',(13.5679367061316,16.6154772628064,8.23179166666662));
#27672=CARTESIAN_POINT('Ctrl Pts',(13.5679367061316,15.5000000000001,8.19012499999996));
#27673=CARTESIAN_POINT('Ctrl Pts',(13.5679367061316,14.3845227371939,8.14845833333329));
#27674=CARTESIAN_POINT('Ctrl Pts',(14.5339683530657,13.8267841057908,8.10679166666662));
#27675=CARTESIAN_POINT('Ctrl Pts',(15.4999999999999,13.2690454743877,8.06512499999995));
#27676=CARTESIAN_POINT('Ctrl Pts',(16.466031646934,13.8267841057908,8.02345833333329));
#27677=CARTESIAN_POINT('Ctrl Pts',(17.4320632938681,14.3845227371939,7.98179166666662));
#27678=CARTESIAN_POINT('Ctrl Pts',(17.4320632938681,15.5000000000002,7.94012499999995));
#27679=CARTESIAN_POINT('Ctrl Pts',(17.4320632938681,16.6154772628064,7.89845833333329));
#27680=CARTESIAN_POINT('Ctrl Pts',(16.466031646934,17.1732158942095,7.85679166666662));
#27681=CARTESIAN_POINT('Ctrl Pts',(15.4999999999998,17.7309545256126,7.81512499999995));
#27682=CARTESIAN_POINT('Ctrl Pts',(14.5339683530657,17.1732158942095,7.77345833333328));
#27683=CARTESIAN_POINT('Ctrl Pts',(13.5679367061316,16.6154772628064,7.73179166666662));
#27684=CARTESIAN_POINT('Ctrl Pts',(13.5679367061316,15.5000000000001,7.69012499999995));
#27685=CARTESIAN_POINT('Ctrl Pts',(13.5679367061316,14.3845227371939,7.64845833333328));
#27686=CARTESIAN_POINT('Ctrl Pts',(14.5339683530657,13.8267841057908,7.60679166666661));
#27687=CARTESIAN_POINT('Ctrl Pts',(15.4999999999999,13.2690454743877,7.56512499999995));
#27688=CARTESIAN_POINT('Ctrl Pts',(16.466031646934,13.8267841057908,7.52345833333328));
#27689=CARTESIAN_POINT('Ctrl Pts',(17.4320632938681,14.3845227371939,7.48179166666661));
#27690=CARTESIAN_POINT('Ctrl Pts',(17.4320632938681,15.5000000000002,7.44012499999995));
#27691=CARTESIAN_POINT('Ctrl Pts',(17.4320632938681,16.6154772628064,7.39845833333328));
#27692=CARTESIAN_POINT('Ctrl Pts',(16.466031646934,17.1732158942095,7.35679166666661));
#27693=CARTESIAN_POINT('Ctrl Pts',(15.4999999999998,17.7309545256126,7.31512499999995));
#27694=CARTESIAN_POINT('Ctrl Pts',(14.5339683530657,17.1732158942095,7.27345833333328));
#27695=CARTESIAN_POINT('Ctrl Pts',(13.5679367061316,16.6154772628064,7.23179166666661));
#27696=CARTESIAN_POINT('Ctrl Pts',(13.5679367061316,15.5000000000001,7.19012499999994));
#27697=CARTESIAN_POINT('Ctrl Pts',(13.5679367061316,14.3845227371939,7.14845833333328));
#27698=CARTESIAN_POINT('Ctrl Pts',(14.5339683530657,13.8267841057908,7.10679166666661));
#27699=CARTESIAN_POINT('Ctrl Pts',(15.4999999999999,13.2690454743877,7.06512499999994));
#27700=CARTESIAN_POINT('Ctrl Pts',(16.466031646934,13.8267841057908,7.02345833333327));
#27701=CARTESIAN_POINT('Ctrl Pts',(17.4320632938681,14.3845227371939,6.98179166666661));
#27702=CARTESIAN_POINT('Ctrl Pts',(17.4320632938681,15.5000000000002,6.94012499999994));
#27703=CARTESIAN_POINT('Ctrl Pts',(17.4320632938681,16.6154772628064,6.89845833333327));
#27704=CARTESIAN_POINT('Ctrl Pts',(16.466031646934,17.1732158942095,6.8567916666666));
#27705=CARTESIAN_POINT('Ctrl Pts',(15.4999999999998,17.7309545256126,6.81512499999994));
#27706=CARTESIAN_POINT('Ctrl Pts',(14.5339683530657,17.1732158942095,6.77345833333327));
#27707=CARTESIAN_POINT('Ctrl Pts',(13.5679367061316,16.6154772628064,6.7317916666666));
#27708=CARTESIAN_POINT('Ctrl Pts',(13.5679367061316,15.5000000000001,6.69012499999994));
#27709=CARTESIAN_POINT('Ctrl Pts',(13.5679367061316,14.3845227371939,6.64845833333327));
#27710=CARTESIAN_POINT('Ctrl Pts',(14.5339683530657,13.8267841057908,6.6067916666666));
#27711=CARTESIAN_POINT('Ctrl Pts',(15.4999999999999,13.2690454743877,6.56512499999993));
#27712=CARTESIAN_POINT('Ctrl Pts',(16.466031646934,13.8267841057908,6.52345833333327));
#27713=CARTESIAN_POINT('Ctrl Pts',(17.4320632938681,14.3845227371939,6.4817916666666));
#27714=CARTESIAN_POINT('Ctrl Pts',(17.4320632938681,15.5000000000002,6.44012499999993));
#27715=CARTESIAN_POINT('Ctrl Pts',(17.4320632938681,16.6154772628064,6.39845833333327));
#27716=CARTESIAN_POINT('Ctrl Pts',(16.466031646934,17.1732158942095,6.3567916666666));
#27717=CARTESIAN_POINT('Ctrl Pts',(15.4999999999998,17.7309545256126,6.31512499999993));
#27718=CARTESIAN_POINT('Ctrl Pts',(14.5339683530657,17.1732158942095,6.27345833333326));
#27719=CARTESIAN_POINT('Ctrl Pts',(13.5679367061316,16.6154772628064,6.2317916666666));
#27720=CARTESIAN_POINT('Ctrl Pts',(13.5679367061316,15.5000000000001,6.19012499999993));
#27721=CARTESIAN_POINT('Ctrl Pts',(13.5679367061316,14.3845227371939,6.14845833333326));
#27722=CARTESIAN_POINT('Ctrl Pts',(14.5339683530657,13.8267841057908,6.10679166666659));
#27723=CARTESIAN_POINT('Ctrl Pts',(15.4999999999999,13.2690454743877,6.06512499999993));
#27724=CARTESIAN_POINT('Ctrl Pts',(16.466031646934,13.8267841057908,6.02345833333326));
#27725=CARTESIAN_POINT('Ctrl Pts',(17.4320632938681,14.3845227371939,5.98179166666659));
#27726=CARTESIAN_POINT('Ctrl Pts',(17.4320632938681,15.5000000000002,5.94012499999993));
#27727=CARTESIAN_POINT('Ctrl Pts',(17.4320632938681,16.6154772628064,5.89845833333326));
#27728=CARTESIAN_POINT('Ctrl Pts',(16.466031646934,17.1732158942095,5.85679166666659));
#27729=CARTESIAN_POINT('Ctrl Pts',(15.4999999999998,17.7309545256126,5.81512499999992));
#27730=CARTESIAN_POINT('Ctrl Pts',(14.5339683530657,17.1732158942095,5.77345833333326));
#27731=CARTESIAN_POINT('Ctrl Pts',(13.5679367061316,16.6154772628064,5.73179166666659));
#27732=CARTESIAN_POINT('Ctrl Pts',(13.5679367061316,15.5000000000001,5.69012499999992));
#27733=CARTESIAN_POINT('Ctrl Pts',(13.5679367061316,14.3845227371939,5.64845833333326));
#27734=CARTESIAN_POINT('Ctrl Pts',(14.5339683530657,13.8267841057908,5.60679166666659));
#27735=CARTESIAN_POINT('Ctrl Pts',(15.4999999999999,13.2690454743877,5.56512499999992));
#27736=CARTESIAN_POINT('Ctrl Pts',(16.466031646934,13.8267841057908,5.52345833333325));
#27737=CARTESIAN_POINT('Ctrl Pts',(17.4320632938681,14.3845227371939,5.48179166666659));
#27738=CARTESIAN_POINT('Ctrl Pts',(17.4320632938681,15.5000000000002,5.44012499999992));
#27739=CARTESIAN_POINT('Ctrl Pts',(17.4320632938681,16.6154772628064,5.39845833333325));
#27740=CARTESIAN_POINT('Ctrl Pts',(16.466031646934,17.1732158942095,5.35679166666658));
#27741=CARTESIAN_POINT('Ctrl Pts',(15.4999999999998,17.7309545256126,5.31512499999992));
#27742=CARTESIAN_POINT('Ctrl Pts',(14.5339683530657,17.1732158942095,5.27345833333325));
#27743=CARTESIAN_POINT('Ctrl Pts',(13.5679367061316,16.6154772628064,5.23179166666658));
#27744=CARTESIAN_POINT('Ctrl Pts',(13.5679367061316,15.5000000000001,5.19012499999992));
#27745=CARTESIAN_POINT('Ctrl Pts',(13.5679367061316,14.3845227371939,5.14845833333325));
#27746=CARTESIAN_POINT('Ctrl Pts',(14.5339683530657,13.8267841057908,5.10679166666658));
#27747=CARTESIAN_POINT('Ctrl Pts',(15.4999999999999,13.2690454743877,5.06512499999991));
#27748=CARTESIAN_POINT('Ctrl Pts',(16.466031646934,13.8267841057908,5.02345833333325));
#27749=CARTESIAN_POINT('Ctrl Pts',(17.4320632938681,14.3845227371939,4.98179166666658));
#27750=CARTESIAN_POINT('Ctrl Pts',(17.4320632938681,15.5000000000002,4.94012499999991));
#27751=CARTESIAN_POINT('Ctrl Pts',(17.4320632938681,16.6154772628064,4.89845833333325));
#27752=CARTESIAN_POINT('Ctrl Pts',(16.466031646934,17.1732158942095,4.85679166666658));
#27753=CARTESIAN_POINT('Ctrl Pts',(15.4999999999998,17.7309545256126,4.81512499999991));
#27754=CARTESIAN_POINT('Ctrl Pts',(14.5339683530657,17.1732158942095,4.77345833333324));
#27755=CARTESIAN_POINT('Ctrl Pts',(13.5679367061316,16.6154772628064,4.73179166666658));
#27756=CARTESIAN_POINT('Ctrl Pts',(13.5679367061316,15.5000000000001,4.69012499999991));
#27757=CARTESIAN_POINT('Ctrl Pts',(13.5679367061316,14.3845227371939,4.64845833333324));
#27758=CARTESIAN_POINT('Ctrl Pts',(14.5339683530657,13.8267841057908,4.60679166666657));
#27759=CARTESIAN_POINT('Ctrl Pts',(15.4999999999999,13.2690454743877,4.56512499999991));
#27760=CARTESIAN_POINT('Ctrl Pts',(16.466031646934,13.8267841057908,4.52345833333324));
#27761=CARTESIAN_POINT('Ctrl Pts',(17.4320632938681,14.3845227371939,4.48179166666657));
#27762=CARTESIAN_POINT('Ctrl Pts',(17.4320632938681,15.5000000000002,4.44012499999991));
#27763=CARTESIAN_POINT('Ctrl Pts',(17.4320632938681,16.6154772628064,4.39845833333324));
#27764=CARTESIAN_POINT('Ctrl Pts',(16.466031646934,17.1732158942095,4.35679166666657));
#27765=CARTESIAN_POINT('Ctrl Pts',(15.4999999999998,17.7309545256126,4.31512499999991));
#27766=CARTESIAN_POINT('Ctrl Pts',(14.5339683530657,17.1732158942095,4.27345833333324));
#27767=CARTESIAN_POINT('Ctrl Pts',(13.5679367061316,16.6154772628064,4.23179166666657));
#27768=CARTESIAN_POINT('Ctrl Pts',(13.5679367061316,15.5000000000001,4.1901249999999));
#27769=CARTESIAN_POINT('Ctrl Pts',(13.5679367061316,14.3845227371939,4.14845833333324));
#27770=CARTESIAN_POINT('Ctrl Pts',(14.5339683530657,13.8267841057908,4.10679166666657));
#27771=CARTESIAN_POINT('Ctrl Pts',(15.4999999999999,13.2690454743877,4.0651249999999));
#27772=CARTESIAN_POINT('Ctrl Pts',(16.466031646934,13.8267841057908,4.02345833333323));
#27773=CARTESIAN_POINT('Ctrl Pts',(17.4320632938681,14.3845227371939,3.98179166666657));
#27774=CARTESIAN_POINT('Ctrl Pts',(17.4320632938681,15.5000000000002,3.9401249999999));
#27775=CARTESIAN_POINT('Ctrl Pts',(17.4320632938681,16.6154772628064,3.89845833333323));
#27776=CARTESIAN_POINT('Ctrl Pts',(16.466031646934,17.1732158942095,3.85679166666657));
#27777=CARTESIAN_POINT('Ctrl Pts',(15.4999999999998,17.7309545256126,3.8151249999999));
#27778=CARTESIAN_POINT('Ctrl Pts',(14.5339683530657,17.1732158942095,3.77345833333323));
#27779=CARTESIAN_POINT('Ctrl Pts',(13.5679367061316,16.6154772628064,3.73179166666656));
#27780=CARTESIAN_POINT('Ctrl Pts',(13.5679367061316,15.5000000000001,3.6901249999999));
#27781=CARTESIAN_POINT('Ctrl Pts',(13.5679367061316,14.3845227371939,3.64845833333323));
#27782=CARTESIAN_POINT('Ctrl Pts',(14.5339683530657,13.8267841057908,3.60679166666656));
#27783=CARTESIAN_POINT('Ctrl Pts',(15.4999999999999,13.2690454743877,3.5651249999999));
#27784=CARTESIAN_POINT('Ctrl Pts',(16.466031646934,13.8267841057908,3.52345833333323));
#27785=CARTESIAN_POINT('Ctrl Pts',(17.4320632938681,14.3845227371939,3.48179166666656));
#27786=CARTESIAN_POINT('Ctrl Pts',(17.4320632938681,15.5000000000002,3.44012499999989));
#27787=CARTESIAN_POINT('Ctrl Pts',(17.4320632938681,16.6154772628064,3.39845833333323));
#27788=CARTESIAN_POINT('Ctrl Pts',(16.466031646934,17.1732158942095,3.35679166666656));
#27789=CARTESIAN_POINT('Ctrl Pts',(15.4999999999998,17.7309545256126,3.31512499999989));
#27790=CARTESIAN_POINT('Ctrl Pts',(14.5339683530657,17.1732158942095,3.27345833333322));
#27791=CARTESIAN_POINT('Ctrl Pts',(13.5679367061316,16.6154772628064,3.23179166666656));
#27792=CARTESIAN_POINT('Ctrl Pts',(13.5679367061316,15.5000000000001,3.19012499999989));
#27793=CARTESIAN_POINT('Ctrl Pts',(13.5679367061316,14.3845227371939,3.14845833333322));
#27794=CARTESIAN_POINT('Ctrl Pts',(14.5339683530657,13.8267841057908,3.10679166666655));
#27795=CARTESIAN_POINT('Ctrl Pts',(15.4999999999999,13.2690454743877,3.06512499999989));
#27796=CARTESIAN_POINT('Ctrl Pts',(16.466031646934,13.8267841057908,3.02345833333322));
#27797=CARTESIAN_POINT('Ctrl Pts',(17.4320632938681,14.3845227371939,2.98179166666655));
#27798=CARTESIAN_POINT('Ctrl Pts',(17.4320632938681,15.5000000000002,2.94012499999989));
#27799=CARTESIAN_POINT('Ctrl Pts',(17.4320632938681,16.6154772628064,2.89845833333322));
#27800=CARTESIAN_POINT('Ctrl Pts',(16.466031646934,17.1732158942095,2.85679166666655));
#27801=CARTESIAN_POINT('Ctrl Pts',(15.4999999999998,17.7309545256126,2.81512499999988));
#27802=CARTESIAN_POINT('Ctrl Pts',(14.5339683530657,17.1732158942095,2.77345833333322));
#27803=CARTESIAN_POINT('Ctrl Pts',(13.5679367061316,16.6154772628064,2.73179166666655));
#27804=CARTESIAN_POINT('Ctrl Pts',(13.5679367061316,15.5000000000001,2.69012499999988));
#27805=CARTESIAN_POINT('Ctrl Pts',(13.5679367061316,14.3845227371939,2.64845833333321));
#27806=CARTESIAN_POINT('Ctrl Pts',(14.5339683530657,13.8267841057908,2.60679166666655));
#27807=CARTESIAN_POINT('Ctrl Pts',(15.4999999999999,13.2690454743877,2.56512499999988));
#27808=CARTESIAN_POINT('Ctrl Pts',(16.466031646934,13.8267841057908,2.52345833333321));
#27809=CARTESIAN_POINT('Ctrl Pts',(17.4320632938681,14.3845227371939,2.48179166666655));
#27810=CARTESIAN_POINT('Ctrl Pts',(17.4320632938681,15.5000000000002,2.44012499999988));
#27811=CARTESIAN_POINT('Ctrl Pts',(17.4320632938681,16.6154772628064,2.39845833333321));
#27812=CARTESIAN_POINT('Ctrl Pts',(16.466031646934,17.1732158942095,2.35679166666655));
#27813=CARTESIAN_POINT('Ctrl Pts',(15.4999999999998,17.7309545256126,2.31512499999988));
#27814=CARTESIAN_POINT('Ctrl Pts',(14.5339683530657,17.1732158942095,2.27345833333321));
#27815=CARTESIAN_POINT('Ctrl Pts',(13.5679367061316,16.6154772628064,2.23179166666654));
#27816=CARTESIAN_POINT('Ctrl Pts',(13.5679367061316,15.5000000000001,2.19012499999988));
#27817=CARTESIAN_POINT('Ctrl Pts',(13.5679367061316,14.3845227371939,2.14845833333321));
#27818=CARTESIAN_POINT('Ctrl Pts',(14.5339683530657,13.8267841057908,2.10679166666654));
#27819=CARTESIAN_POINT('Ctrl Pts',(15.4999999999999,13.2690454743877,2.06512499999987));
#27820=CARTESIAN_POINT('Ctrl Pts',(16.466031646934,13.8267841057908,2.02345833333321));
#27821=CARTESIAN_POINT('Ctrl Pts',(17.4320632938681,14.3845227371939,1.98179166666654));
#27822=CARTESIAN_POINT('Ctrl Pts',(17.4320632938681,15.5000000000002,1.94012499999987));
#27823=CARTESIAN_POINT('Ctrl Pts',(17.4320632938681,16.6154772628064,1.89845833333321));
#27824=CARTESIAN_POINT('Ctrl Pts',(16.466031646934,17.1732158942095,1.85679166666654));
#27825=CARTESIAN_POINT('Ctrl Pts',(15.4999999999998,17.7309545256126,1.81512499999987));
#27826=CARTESIAN_POINT('Ctrl Pts',(14.5339683530657,17.1732158942095,1.7734583333332));
#27827=CARTESIAN_POINT('Ctrl Pts',(13.5679367061316,16.6154772628064,1.73179166666654));
#27828=CARTESIAN_POINT('Ctrl Pts',(13.5679367061316,15.5000000000001,1.69012499999987));
#27829=CARTESIAN_POINT('Ctrl Pts',(13.5679367061316,14.3845227371939,1.6484583333332));
#27830=CARTESIAN_POINT('Ctrl Pts',(14.5339683530657,13.8267841057908,1.60679166666653));
#27831=CARTESIAN_POINT('Ctrl Pts',(15.4999999999999,13.2690454743877,1.56512499999987));
#27832=CARTESIAN_POINT('Ctrl Pts',(16.466031646934,13.8267841057908,1.5234583333332));
#27833=CARTESIAN_POINT('Ctrl Pts',(17.4320632938681,14.3845227371939,1.48179166666653));
#27834=CARTESIAN_POINT('Ctrl Pts',(17.4320632938681,15.5000000000002,1.44012499999987));
#27835=CARTESIAN_POINT('Ctrl Pts',(17.4320632938681,16.6154772628064,1.3984583333332));
#27836=CARTESIAN_POINT('Ctrl Pts',(16.466031646934,17.1732158942095,1.35679166666653));
#27837=CARTESIAN_POINT('Ctrl Pts',(15.4999999999998,17.7309545256126,1.31512499999987));
#27838=CARTESIAN_POINT('Ctrl Pts',(14.5339683530657,17.1732158942095,1.2734583333332));
#27839=CARTESIAN_POINT('Ctrl Pts',(13.5679367061316,16.6154772628064,1.23179166666653));
#27840=CARTESIAN_POINT('Ctrl Pts',(13.5679367061316,15.5000000000001,1.19012499999986));
#27841=CARTESIAN_POINT('Ctrl Pts',(13.5679367061316,14.3845227371939,1.1484583333332));
#27842=CARTESIAN_POINT('Ctrl Pts',(14.5339683530657,13.8267841057908,1.10679166666653));
#27843=CARTESIAN_POINT('Ctrl Pts',(15.4999999999999,13.2690454743877,1.06512499999986));
#27844=CARTESIAN_POINT('Ctrl Pts',(16.466031646934,13.8267841057908,1.02345833333319));
#27845=CARTESIAN_POINT('Ctrl Pts',(17.4320632938681,14.3845227371939,0.981791666666527));
#27846=CARTESIAN_POINT('Ctrl Pts',(17.4320632938681,15.5000000000002,0.94012499999986));
#27847=CARTESIAN_POINT('Ctrl Pts',(17.4320632938681,16.6154772628064,0.898458333333192));
#27848=CARTESIAN_POINT('Ctrl Pts',(16.466031646934,17.1732158942095,0.856791666666525));
#27849=CARTESIAN_POINT('Ctrl Pts',(15.4999999999998,17.7309545256126,0.815124999999858));
#27850=CARTESIAN_POINT('Ctrl Pts',(14.5339683530657,17.1732158942095,0.77345833333319));
#27851=CARTESIAN_POINT('Ctrl Pts',(13.5679367061316,16.6154772628064,0.731791666666523));
#27852=CARTESIAN_POINT('Ctrl Pts',(13.5679367061316,15.5000000000001,0.690124999999856));
#27853=CARTESIAN_POINT('Ctrl Pts',(13.5679367061316,14.3845227371939,0.648458333333188));
#27854=CARTESIAN_POINT('Ctrl Pts',(14.5339683530657,13.8267841057908,0.606791666666521));
#27855=CARTESIAN_POINT('Ctrl Pts',(15.4999999999999,13.2690454743877,0.565124999999854));
#27856=CARTESIAN_POINT('Ctrl Pts',(16.466031646934,13.8267841057908,0.523458333333187));
#27857=CARTESIAN_POINT('Ctrl Pts',(17.4320632938681,14.3845227371939,0.481791666666519));
#27858=CARTESIAN_POINT('Ctrl Pts',(17.4320632938681,15.5000000000002,0.440124999999852));
#27859=CARTESIAN_POINT('Ctrl Pts',(17.4320632938681,16.6154772628064,0.398458333333185));
#27860=CARTESIAN_POINT('Ctrl Pts',(16.466031646934,17.1732158942095,0.356791666666518));
#27861=CARTESIAN_POINT('Ctrl Pts',(15.4999999999998,17.7309545256126,0.31512499999985));
#27862=CARTESIAN_POINT('Ctrl Pts',(14.5339683530657,17.1732158942095,0.273458333333183));
#27863=CARTESIAN_POINT('Ctrl Pts',(13.5679367061316,16.6154772628064,0.231791666666516));
#27864=CARTESIAN_POINT('Ctrl Pts',(13.5679367061316,15.5000000000001,0.190124999999848));
#27865=CARTESIAN_POINT('Ctrl Pts',(13.5679367061316,14.3845227371939,0.148458333333183));
#27866=CARTESIAN_POINT('Ctrl Pts',(14.5339683530657,13.8267841057908,0.106791666666516));
#27867=CARTESIAN_POINT('Ctrl Pts',(15.4999999999999,13.2690454743877,0.0651249999998483));
#27868=CARTESIAN_POINT('Ctrl Pts',(16.466031646934,13.8267841057908,0.023458333333181));
#27869=CARTESIAN_POINT('Ctrl Pts',(17.4320632938681,14.3845227371939,-0.0182083333334863));
#27870=CARTESIAN_POINT('Ctrl Pts',(17.4320632938681,15.5000000000002,-0.0598750000001536));
#27871=CARTESIAN_POINT('Ctrl Pts',(17.4320632938681,16.6154772628064,-0.101541666666821));
#27872=CARTESIAN_POINT('Ctrl Pts',(16.466031646934,17.1732158942095,-0.143208333333488));
#27873=CARTESIAN_POINT('Ctrl Pts',(15.4999999999998,17.7309545256126,-0.184875000000155));
#27874=CARTESIAN_POINT('Ctrl Pts',(14.5339683530657,17.1732158942095,-0.226541666666823));
#27875=CARTESIAN_POINT('Ctrl Pts',(13.5679367061316,16.6154772628064,-0.26820833333349));
#27876=CARTESIAN_POINT('Ctrl Pts',(13.5679367061316,15.5000000000001,-0.309875000000157));
#27877=CARTESIAN_POINT('Ctrl Pts',(13.5679367061316,14.3845227371939,-0.351541666666825));
#27878=CARTESIAN_POINT('Ctrl Pts',(14.5339683530657,13.8267841057908,-0.393208333333492));
#27879=CARTESIAN_POINT('Ctrl Pts',(15.4999999999999,13.2690454743877,-0.434875000000159));
#27880=CARTESIAN_POINT('Ctrl Pts',(16.466031646934,13.8267841057908,-0.476541666666826));
#27881=CARTESIAN_POINT('Ctrl Pts',(17.4320632938681,14.3845227371939,-0.518208333333494));
#27882=CARTESIAN_POINT('Ctrl Pts',(17.4320632938681,15.5000000000002,-0.559875000000161));
#27883=CARTESIAN_POINT('Ctrl Pts',(17.4320632938681,16.6154772628064,-0.601541666666828));
#27884=CARTESIAN_POINT('Ctrl Pts',(16.466031646934,17.1732158942095,-0.643208333333495));
#27885=CARTESIAN_POINT('Ctrl Pts',(15.4999999999998,17.7309545256126,-0.684875000000163));
#27886=CARTESIAN_POINT('Ctrl Pts',(14.5339683530657,17.1732158942095,-0.72654166666683));
#27887=CARTESIAN_POINT('Ctrl Pts',(13.5679367061316,16.6154772628064,-0.768208333333497));
#27888=CARTESIAN_POINT('Ctrl Pts',(13.5679367061316,15.5000000000001,-0.809875000000165));
#27889=CARTESIAN_POINT('Ctrl Pts',(13.5679367061316,14.3845227371939,-0.851541666666832));
#27890=CARTESIAN_POINT('Ctrl Pts',(14.5339683530657,13.8267841057908,-0.893208333333499));
#27891=CARTESIAN_POINT('Ctrl Pts',(15.4999999999999,13.2690454743877,-0.934875000000167));
#27892=CARTESIAN_POINT('Ctrl Pts',(16.466031646934,13.8267841057908,-0.976541666666834));
#27893=CARTESIAN_POINT('Ctrl Pts',(17.4320632938681,14.3845227371939,-1.0182083333335));
#27894=CARTESIAN_POINT('Ctrl Pts',(17.4320632938681,15.5000000000002,-1.05987500000017));
#27895=CARTESIAN_POINT('Ctrl Pts',(17.4320632938681,16.6154772628064,-1.10154166666683));
#27896=CARTESIAN_POINT('Ctrl Pts',(16.466031646934,17.1732158942095,-1.1432083333335));
#27897=CARTESIAN_POINT('Ctrl Pts',(15.4999999999998,17.7309545256126,-1.18487500000017));
#27898=CARTESIAN_POINT('Ctrl Pts',(14.5339683530657,17.1732158942095,-1.22654166666684));
#27899=CARTESIAN_POINT('Ctrl Pts',(13.5679367061316,16.6154772628064,-1.2682083333335));
#27900=CARTESIAN_POINT('Ctrl Pts',(13.5679367061316,15.5000000000001,-1.30987500000017));
#27901=CARTESIAN_POINT('Ctrl Pts',(13.5679367061316,14.3845227371939,-1.35154166666684));
#27902=CARTESIAN_POINT('Ctrl Pts',(14.5339683530657,13.8267841057908,-1.3932083333335));
#27903=CARTESIAN_POINT('Ctrl Pts',(15.4999999999999,13.2690454743877,-1.43487500000017));
#27904=CARTESIAN_POINT('Ctrl Pts',(16.466031646934,13.8267841057908,-1.47654166666684));
#27905=CARTESIAN_POINT('Ctrl Pts',(17.4320632938681,14.3845227371939,-1.51820833333351));
#27906=CARTESIAN_POINT('Ctrl Pts',(17.4320632938681,15.5000000000002,-1.55987500000017));
#27907=CARTESIAN_POINT('Ctrl Pts',(17.4320632938681,16.6154772628064,-1.60154166666684));
#27908=CARTESIAN_POINT('Ctrl Pts',(16.466031646934,17.1732158942095,-1.64320833333351));
#27909=CARTESIAN_POINT('Ctrl Pts',(15.4999999999998,17.7309545256126,-1.68487500000018));
#27910=CARTESIAN_POINT('Ctrl Pts',(14.5339683530657,17.1732158942095,-1.72654166666684));
#27911=CARTESIAN_POINT('Ctrl Pts',(14.1783081829976,16.9678753992807,-1.74188192368624));
#27912=CARTESIAN_POINT('Ctrl Pts',(13.936918671564,16.6356255246377,-1.75949830599533));
#27913=CARTESIAN_POINT('Ctrl Pts',(17.0802357869869,15.5000000000002,11.2369972941938));
#27914=CARTESIAN_POINT('Ctrl Pts',(17.0802357869869,16.4123495570002,11.1953306275271));
#27915=CARTESIAN_POINT('Ctrl Pts',(16.2901178934933,16.8685243355002,11.1536639608605));
#27916=CARTESIAN_POINT('Ctrl Pts',(15.4999999999998,17.3246991140003,11.1119972941938));
#27917=CARTESIAN_POINT('Ctrl Pts',(14.7098821065064,16.8685243355002,11.0703306275271));
#27918=CARTESIAN_POINT('Ctrl Pts',(13.9197642130128,16.4123495570002,11.0286639608605));
#27919=CARTESIAN_POINT('Ctrl Pts',(13.9197642130128,15.5000000000001,10.9869972941938));
#27920=CARTESIAN_POINT('Ctrl Pts',(13.9197642130128,14.5876504430001,10.9453306275271));
#27921=CARTESIAN_POINT('Ctrl Pts',(14.7098821065064,14.1314756645001,10.9036639608605));
#27922=CARTESIAN_POINT('Ctrl Pts',(15.4999999999999,13.6753008860001,10.8619972941938));
#27923=CARTESIAN_POINT('Ctrl Pts',(16.2901178934933,14.1314756645001,10.8203306275271));
#27924=CARTESIAN_POINT('Ctrl Pts',(17.0802357869869,14.5876504430001,10.7786639608605));
#27925=CARTESIAN_POINT('Ctrl Pts',(17.0802357869869,15.5000000000002,10.7369972941938));
#27926=CARTESIAN_POINT('Ctrl Pts',(17.0802357869869,16.4123495570002,10.6953306275271));
#27927=CARTESIAN_POINT('Ctrl Pts',(16.2901178934933,16.8685243355002,10.6536639608605));
#27928=CARTESIAN_POINT('Ctrl Pts',(15.4999999999998,17.3246991140003,10.6119972941938));
#27929=CARTESIAN_POINT('Ctrl Pts',(14.7098821065064,16.8685243355002,10.5703306275271));
#27930=CARTESIAN_POINT('Ctrl Pts',(13.9197642130128,16.4123495570002,10.5286639608605));
#27931=CARTESIAN_POINT('Ctrl Pts',(13.9197642130128,15.5000000000001,10.4869972941938));
#27932=CARTESIAN_POINT('Ctrl Pts',(13.9197642130128,14.5876504430001,10.4453306275271));
#27933=CARTESIAN_POINT('Ctrl Pts',(14.7098821065064,14.1314756645001,10.4036639608605));
#27934=CARTESIAN_POINT('Ctrl Pts',(15.4999999999999,13.6753008860001,10.3619972941938));
#27935=CARTESIAN_POINT('Ctrl Pts',(16.2901178934933,14.1314756645001,10.3203306275271));
#27936=CARTESIAN_POINT('Ctrl Pts',(17.0802357869869,14.5876504430001,10.2786639608605));
#27937=CARTESIAN_POINT('Ctrl Pts',(17.0802357869869,15.5000000000002,10.2369972941938));
#27938=CARTESIAN_POINT('Ctrl Pts',(17.0802357869869,16.4123495570002,10.1953306275271));
#27939=CARTESIAN_POINT('Ctrl Pts',(16.2901178934933,16.8685243355002,10.1536639608605));
#27940=CARTESIAN_POINT('Ctrl Pts',(15.4999999999998,17.3246991140003,10.1119972941938));
#27941=CARTESIAN_POINT('Ctrl Pts',(14.7098821065064,16.8685243355002,10.0703306275271));
#27942=CARTESIAN_POINT('Ctrl Pts',(13.9197642130128,16.4123495570002,10.0286639608605));
#27943=CARTESIAN_POINT('Ctrl Pts',(13.9197642130128,15.5000000000001,9.98699729419377));
#27944=CARTESIAN_POINT('Ctrl Pts',(13.9197642130128,14.5876504430001,9.94533062752711));
#27945=CARTESIAN_POINT('Ctrl Pts',(14.7098821065064,14.1314756645001,9.90366396086044));
#27946=CARTESIAN_POINT('Ctrl Pts',(15.4999999999999,13.6753008860001,9.86199729419377));
#27947=CARTESIAN_POINT('Ctrl Pts',(16.2901178934933,14.1314756645001,9.82033062752711));
#27948=CARTESIAN_POINT('Ctrl Pts',(17.0802357869869,14.5876504430001,9.77866396086044));
#27949=CARTESIAN_POINT('Ctrl Pts',(17.0802357869869,15.5000000000002,9.73699729419377));
#27950=CARTESIAN_POINT('Ctrl Pts',(17.0802357869869,16.4123495570002,9.6953306275271));
#27951=CARTESIAN_POINT('Ctrl Pts',(16.2901178934933,16.8685243355002,9.65366396086044));
#27952=CARTESIAN_POINT('Ctrl Pts',(15.4999999999998,17.3246991140003,9.61199729419377));
#27953=CARTESIAN_POINT('Ctrl Pts',(14.7098821065064,16.8685243355002,9.5703306275271));
#27954=CARTESIAN_POINT('Ctrl Pts',(13.9197642130128,16.4123495570002,9.52866396086043));
#27955=CARTESIAN_POINT('Ctrl Pts',(13.9197642130128,15.5000000000001,9.48699729419377));
#27956=CARTESIAN_POINT('Ctrl Pts',(13.9197642130128,14.5876504430001,9.4453306275271));
#27957=CARTESIAN_POINT('Ctrl Pts',(14.7098821065064,14.1314756645001,9.40366396086043));
#27958=CARTESIAN_POINT('Ctrl Pts',(15.4999999999999,13.6753008860001,9.36199729419377));
#27959=CARTESIAN_POINT('Ctrl Pts',(16.2901178934933,14.1314756645001,9.3203306275271));
#27960=CARTESIAN_POINT('Ctrl Pts',(17.0802357869869,14.5876504430001,9.27866396086043));
#27961=CARTESIAN_POINT('Ctrl Pts',(17.0802357869869,15.5000000000002,9.23699729419377));
#27962=CARTESIAN_POINT('Ctrl Pts',(17.0802357869869,16.4123495570002,9.1953306275271));
#27963=CARTESIAN_POINT('Ctrl Pts',(16.2901178934933,16.8685243355002,9.15366396086043));
#27964=CARTESIAN_POINT('Ctrl Pts',(15.4999999999998,17.3246991140003,9.11199729419376));
#27965=CARTESIAN_POINT('Ctrl Pts',(14.7098821065064,16.8685243355002,9.07033062752709));
#27966=CARTESIAN_POINT('Ctrl Pts',(13.9197642130128,16.4123495570002,9.02866396086043));
#27967=CARTESIAN_POINT('Ctrl Pts',(13.9197642130128,15.5000000000001,8.98699729419377));
#27968=CARTESIAN_POINT('Ctrl Pts',(13.9197642130128,14.5876504430001,8.94533062752709));
#27969=CARTESIAN_POINT('Ctrl Pts',(14.7098821065064,14.1314756645001,8.90366396086043));
#27970=CARTESIAN_POINT('Ctrl Pts',(15.4999999999999,13.6753008860001,8.86199729419377));
#27971=CARTESIAN_POINT('Ctrl Pts',(16.2901178934933,14.1314756645001,8.82033062752709));
#27972=CARTESIAN_POINT('Ctrl Pts',(17.0802357869869,14.5876504430001,8.77866396086042));
#27973=CARTESIAN_POINT('Ctrl Pts',(17.0802357869869,15.5000000000002,8.73699729419377));
#27974=CARTESIAN_POINT('Ctrl Pts',(17.0802357869869,16.4123495570002,8.69533062752709));
#27975=CARTESIAN_POINT('Ctrl Pts',(16.2901178934933,16.8685243355002,8.65366396086042));
#27976=CARTESIAN_POINT('Ctrl Pts',(15.4999999999998,17.3246991140003,8.61199729419376));
#27977=CARTESIAN_POINT('Ctrl Pts',(14.7098821065064,16.8685243355002,8.57033062752709));
#27978=CARTESIAN_POINT('Ctrl Pts',(13.9197642130128,16.4123495570002,8.52866396086042));
#27979=CARTESIAN_POINT('Ctrl Pts',(13.9197642130128,15.5000000000001,8.48699729419375));
#27980=CARTESIAN_POINT('Ctrl Pts',(13.9197642130128,14.5876504430001,8.44533062752709));
#27981=CARTESIAN_POINT('Ctrl Pts',(14.7098821065064,14.1314756645001,8.40366396086042));
#27982=CARTESIAN_POINT('Ctrl Pts',(15.4999999999999,13.6753008860001,8.36199729419375));
#27983=CARTESIAN_POINT('Ctrl Pts',(16.2901178934933,14.1314756645001,8.32033062752709));
#27984=CARTESIAN_POINT('Ctrl Pts',(17.0802357869869,14.5876504430001,8.27866396086042));
#27985=CARTESIAN_POINT('Ctrl Pts',(17.0802357869869,15.5000000000002,8.23699729419376));
#27986=CARTESIAN_POINT('Ctrl Pts',(17.0802357869869,16.4123495570002,8.19533062752708));
#27987=CARTESIAN_POINT('Ctrl Pts',(16.2901178934933,16.8685243355002,8.15366396086042));
#27988=CARTESIAN_POINT('Ctrl Pts',(15.4999999999998,17.3246991140003,8.11199729419375));
#27989=CARTESIAN_POINT('Ctrl Pts',(14.7098821065064,16.8685243355002,8.07033062752709));
#27990=CARTESIAN_POINT('Ctrl Pts',(13.9197642130128,16.4123495570002,8.02866396086042));
#27991=CARTESIAN_POINT('Ctrl Pts',(13.9197642130128,15.5000000000001,7.98699729419375));
#27992=CARTESIAN_POINT('Ctrl Pts',(13.9197642130128,14.5876504430001,7.94533062752708));
#27993=CARTESIAN_POINT('Ctrl Pts',(14.7098821065064,14.1314756645001,7.90366396086042));
#27994=CARTESIAN_POINT('Ctrl Pts',(15.4999999999999,13.6753008860001,7.86199729419375));
#27995=CARTESIAN_POINT('Ctrl Pts',(16.2901178934933,14.1314756645001,7.82033062752708));
#27996=CARTESIAN_POINT('Ctrl Pts',(17.0802357869869,14.5876504430001,7.77866396086041));
#27997=CARTESIAN_POINT('Ctrl Pts',(17.0802357869869,15.5000000000002,7.73699729419374));
#27998=CARTESIAN_POINT('Ctrl Pts',(17.0802357869869,16.4123495570002,7.69533062752708));
#27999=CARTESIAN_POINT('Ctrl Pts',(16.2901178934933,16.8685243355002,7.65366396086041));
#28000=CARTESIAN_POINT('Ctrl Pts',(15.4999999999998,17.3246991140003,7.61199729419374));
#28001=CARTESIAN_POINT('Ctrl Pts',(14.7098821065064,16.8685243355002,7.57033062752708));
#28002=CARTESIAN_POINT('Ctrl Pts',(13.9197642130128,16.4123495570002,7.52866396086041));
#28003=CARTESIAN_POINT('Ctrl Pts',(13.9197642130128,15.5000000000001,7.48699729419375));
#28004=CARTESIAN_POINT('Ctrl Pts',(13.9197642130128,14.5876504430001,7.44533062752707));
#28005=CARTESIAN_POINT('Ctrl Pts',(14.7098821065064,14.1314756645001,7.4036639608604));
#28006=CARTESIAN_POINT('Ctrl Pts',(15.4999999999999,13.6753008860001,7.36199729419374));
#28007=CARTESIAN_POINT('Ctrl Pts',(16.2901178934933,14.1314756645001,7.32033062752707));
#28008=CARTESIAN_POINT('Ctrl Pts',(17.0802357869869,14.5876504430001,7.27866396086041));
#28009=CARTESIAN_POINT('Ctrl Pts',(17.0802357869869,15.5000000000002,7.23699729419374));
#28010=CARTESIAN_POINT('Ctrl Pts',(17.0802357869869,16.4123495570002,7.19533062752707));
#28011=CARTESIAN_POINT('Ctrl Pts',(16.2901178934933,16.8685243355002,7.1536639608604));
#28012=CARTESIAN_POINT('Ctrl Pts',(15.4999999999998,17.3246991140003,7.11199729419373));
#28013=CARTESIAN_POINT('Ctrl Pts',(14.7098821065064,16.8685243355002,7.07033062752707));
#28014=CARTESIAN_POINT('Ctrl Pts',(13.9197642130128,16.4123495570002,7.0286639608604));
#28015=CARTESIAN_POINT('Ctrl Pts',(13.9197642130128,15.5000000000001,6.98699729419373));
#28016=CARTESIAN_POINT('Ctrl Pts',(13.9197642130128,14.5876504430001,6.94533062752707));
#28017=CARTESIAN_POINT('Ctrl Pts',(14.7098821065064,14.1314756645001,6.90366396086041));
#28018=CARTESIAN_POINT('Ctrl Pts',(15.4999999999999,13.6753008860001,6.86199729419373));
#28019=CARTESIAN_POINT('Ctrl Pts',(16.2901178934933,14.1314756645001,6.82033062752706));
#28020=CARTESIAN_POINT('Ctrl Pts',(17.0802357869869,14.5876504430001,6.7786639608604));
#28021=CARTESIAN_POINT('Ctrl Pts',(17.0802357869869,15.5000000000002,6.73699729419373));
#28022=CARTESIAN_POINT('Ctrl Pts',(17.0802357869869,16.4123495570002,6.69533062752706));
#28023=CARTESIAN_POINT('Ctrl Pts',(16.2901178934933,16.8685243355002,6.6536639608604));
#28024=CARTESIAN_POINT('Ctrl Pts',(15.4999999999998,17.3246991140003,6.61199729419373));
#28025=CARTESIAN_POINT('Ctrl Pts',(14.7098821065064,16.8685243355002,6.57033062752706));
#28026=CARTESIAN_POINT('Ctrl Pts',(13.9197642130128,16.4123495570002,6.52866396086039));
#28027=CARTESIAN_POINT('Ctrl Pts',(13.9197642130128,15.5000000000001,6.48699729419373));
#28028=CARTESIAN_POINT('Ctrl Pts',(13.9197642130128,14.5876504430001,6.44533062752706));
#28029=CARTESIAN_POINT('Ctrl Pts',(14.7098821065064,14.1314756645001,6.40366396086039));
#28030=CARTESIAN_POINT('Ctrl Pts',(15.4999999999999,13.6753008860001,6.36199729419373));
#28031=CARTESIAN_POINT('Ctrl Pts',(16.2901178934933,14.1314756645001,6.32033062752707));
#28032=CARTESIAN_POINT('Ctrl Pts',(17.0802357869869,14.5876504430001,6.27866396086039));
#28033=CARTESIAN_POINT('Ctrl Pts',(17.0802357869869,15.5000000000002,6.23699729419372));
#28034=CARTESIAN_POINT('Ctrl Pts',(17.0802357869869,16.4123495570002,6.19533062752706));
#28035=CARTESIAN_POINT('Ctrl Pts',(16.2901178934933,16.8685243355002,6.1536639608604));
#28036=CARTESIAN_POINT('Ctrl Pts',(15.4999999999998,17.3246991140003,6.11199729419372));
#28037=CARTESIAN_POINT('Ctrl Pts',(14.7098821065064,16.8685243355002,6.07033062752705));
#28038=CARTESIAN_POINT('Ctrl Pts',(13.9197642130128,16.4123495570002,6.02866396086039));
#28039=CARTESIAN_POINT('Ctrl Pts',(13.9197642130128,15.5000000000001,5.98699729419372));
#28040=CARTESIAN_POINT('Ctrl Pts',(13.9197642130128,14.5876504430001,5.94533062752705));
#28041=CARTESIAN_POINT('Ctrl Pts',(14.7098821065064,14.1314756645001,5.90366396086039));
#28042=CARTESIAN_POINT('Ctrl Pts',(15.4999999999999,13.6753008860001,5.86199729419372));
#28043=CARTESIAN_POINT('Ctrl Pts',(16.2901178934933,14.1314756645001,5.82033062752705));
#28044=CARTESIAN_POINT('Ctrl Pts',(17.0802357869869,14.5876504430001,5.77866396086038));
#28045=CARTESIAN_POINT('Ctrl Pts',(17.0802357869869,15.5000000000002,5.73699729419372));
#28046=CARTESIAN_POINT('Ctrl Pts',(17.0802357869869,16.4123495570002,5.69533062752705));
#28047=CARTESIAN_POINT('Ctrl Pts',(16.2901178934933,16.8685243355002,5.65366396086038));
#28048=CARTESIAN_POINT('Ctrl Pts',(15.4999999999998,17.3246991140003,5.61199729419371));
#28049=CARTESIAN_POINT('Ctrl Pts',(14.7098821065064,16.8685243355002,5.57033062752705));
#28050=CARTESIAN_POINT('Ctrl Pts',(13.9197642130128,16.4123495570002,5.52866396086038));
#28051=CARTESIAN_POINT('Ctrl Pts',(13.9197642130128,15.5000000000001,5.48699729419371));
#28052=CARTESIAN_POINT('Ctrl Pts',(13.9197642130128,14.5876504430001,5.44533062752705));
#28053=CARTESIAN_POINT('Ctrl Pts',(14.7098821065064,14.1314756645001,5.40366396086038));
#28054=CARTESIAN_POINT('Ctrl Pts',(15.4999999999999,13.6753008860001,5.36199729419371));
#28055=CARTESIAN_POINT('Ctrl Pts',(16.2901178934933,14.1314756645001,5.32033062752704));
#28056=CARTESIAN_POINT('Ctrl Pts',(17.0802357869869,14.5876504430001,5.27866396086038));
#28057=CARTESIAN_POINT('Ctrl Pts',(17.0802357869869,15.5000000000002,5.23699729419371));
#28058=CARTESIAN_POINT('Ctrl Pts',(17.0802357869869,16.4123495570002,5.19533062752704));
#28059=CARTESIAN_POINT('Ctrl Pts',(16.2901178934933,16.8685243355002,5.15366396086038));
#28060=CARTESIAN_POINT('Ctrl Pts',(15.4999999999998,17.3246991140003,5.11199729419371));
#28061=CARTESIAN_POINT('Ctrl Pts',(14.7098821065064,16.8685243355002,5.07033062752704));
#28062=CARTESIAN_POINT('Ctrl Pts',(13.9197642130128,16.4123495570002,5.02866396086037));
#28063=CARTESIAN_POINT('Ctrl Pts',(13.9197642130128,15.5000000000001,4.98699729419371));
#28064=CARTESIAN_POINT('Ctrl Pts',(13.9197642130128,14.5876504430001,4.94533062752704));
#28065=CARTESIAN_POINT('Ctrl Pts',(14.7098821065064,14.1314756645001,4.90366396086037));
#28066=CARTESIAN_POINT('Ctrl Pts',(15.4999999999999,13.6753008860001,4.8619972941937));
#28067=CARTESIAN_POINT('Ctrl Pts',(16.2901178934933,14.1314756645001,4.82033062752704));
#28068=CARTESIAN_POINT('Ctrl Pts',(17.0802357869869,14.5876504430001,4.77866396086037));
#28069=CARTESIAN_POINT('Ctrl Pts',(17.0802357869869,15.5000000000002,4.7369972941937));
#28070=CARTESIAN_POINT('Ctrl Pts',(17.0802357869869,16.4123495570002,4.69533062752704));
#28071=CARTESIAN_POINT('Ctrl Pts',(16.2901178934933,16.8685243355002,4.65366396086037));
#28072=CARTESIAN_POINT('Ctrl Pts',(15.4999999999998,17.3246991140003,4.6119972941937));
#28073=CARTESIAN_POINT('Ctrl Pts',(14.7098821065064,16.8685243355002,4.57033062752703));
#28074=CARTESIAN_POINT('Ctrl Pts',(13.9197642130128,16.4123495570002,4.52866396086037));
#28075=CARTESIAN_POINT('Ctrl Pts',(13.9197642130128,15.5000000000001,4.4869972941937));
#28076=CARTESIAN_POINT('Ctrl Pts',(13.9197642130128,14.5876504430001,4.44533062752703));
#28077=CARTESIAN_POINT('Ctrl Pts',(14.7098821065064,14.1314756645001,4.40366396086037));
#28078=CARTESIAN_POINT('Ctrl Pts',(15.4999999999999,13.6753008860001,4.3619972941937));
#28079=CARTESIAN_POINT('Ctrl Pts',(16.2901178934933,14.1314756645001,4.32033062752703));
#28080=CARTESIAN_POINT('Ctrl Pts',(17.0802357869869,14.5876504430001,4.27866396086036));
#28081=CARTESIAN_POINT('Ctrl Pts',(17.0802357869869,15.5000000000002,4.2369972941937));
#28082=CARTESIAN_POINT('Ctrl Pts',(17.0802357869869,16.4123495570002,4.19533062752703));
#28083=CARTESIAN_POINT('Ctrl Pts',(16.2901178934933,16.8685243355002,4.15366396086036));
#28084=CARTESIAN_POINT('Ctrl Pts',(15.4999999999998,17.3246991140003,4.11199729419369));
#28085=CARTESIAN_POINT('Ctrl Pts',(14.7098821065064,16.8685243355002,4.07033062752703));
#28086=CARTESIAN_POINT('Ctrl Pts',(13.9197642130128,16.4123495570002,4.02866396086036));
#28087=CARTESIAN_POINT('Ctrl Pts',(13.9197642130128,15.5000000000001,3.98699729419369));
#28088=CARTESIAN_POINT('Ctrl Pts',(13.9197642130128,14.5876504430001,3.94533062752703));
#28089=CARTESIAN_POINT('Ctrl Pts',(14.7098821065064,14.1314756645001,3.90366396086036));
#28090=CARTESIAN_POINT('Ctrl Pts',(15.4999999999999,13.6753008860001,3.86199729419369));
#28091=CARTESIAN_POINT('Ctrl Pts',(16.2901178934933,14.1314756645001,3.82033062752702));
#28092=CARTESIAN_POINT('Ctrl Pts',(17.0802357869869,14.5876504430001,3.77866396086036));
#28093=CARTESIAN_POINT('Ctrl Pts',(17.0802357869869,15.5000000000002,3.73699729419369));
#28094=CARTESIAN_POINT('Ctrl Pts',(17.0802357869869,16.4123495570002,3.69533062752702));
#28095=CARTESIAN_POINT('Ctrl Pts',(16.2901178934933,16.8685243355002,3.65366396086036));
#28096=CARTESIAN_POINT('Ctrl Pts',(15.4999999999998,17.3246991140003,3.61199729419369));
#28097=CARTESIAN_POINT('Ctrl Pts',(14.7098821065064,16.8685243355002,3.57033062752702));
#28098=CARTESIAN_POINT('Ctrl Pts',(13.9197642130128,16.4123495570002,3.52866396086035));
#28099=CARTESIAN_POINT('Ctrl Pts',(13.9197642130128,15.5000000000001,3.48699729419369));
#28100=CARTESIAN_POINT('Ctrl Pts',(13.9197642130128,14.5876504430001,3.44533062752702));
#28101=CARTESIAN_POINT('Ctrl Pts',(14.7098821065064,14.1314756645001,3.40366396086035));
#28102=CARTESIAN_POINT('Ctrl Pts',(15.4999999999999,13.6753008860001,3.36199729419369));
#28103=CARTESIAN_POINT('Ctrl Pts',(16.2901178934933,14.1314756645001,3.32033062752702));
#28104=CARTESIAN_POINT('Ctrl Pts',(17.0802357869869,14.5876504430001,3.27866396086035));
#28105=CARTESIAN_POINT('Ctrl Pts',(17.0802357869869,15.5000000000002,3.23699729419368));
#28106=CARTESIAN_POINT('Ctrl Pts',(17.0802357869869,16.4123495570002,3.19533062752702));
#28107=CARTESIAN_POINT('Ctrl Pts',(16.2901178934933,16.8685243355002,3.15366396086035));
#28108=CARTESIAN_POINT('Ctrl Pts',(15.4999999999998,17.3246991140003,3.11199729419368));
#28109=CARTESIAN_POINT('Ctrl Pts',(14.7098821065064,16.8685243355002,3.07033062752702));
#28110=CARTESIAN_POINT('Ctrl Pts',(13.9197642130128,16.4123495570002,3.02866396086035));
#28111=CARTESIAN_POINT('Ctrl Pts',(13.9197642130128,15.5000000000001,2.98699729419368));
#28112=CARTESIAN_POINT('Ctrl Pts',(13.9197642130128,14.5876504430001,2.94533062752701));
#28113=CARTESIAN_POINT('Ctrl Pts',(14.7098821065064,14.1314756645001,2.90366396086035));
#28114=CARTESIAN_POINT('Ctrl Pts',(15.4999999999999,13.6753008860001,2.86199729419368));
#28115=CARTESIAN_POINT('Ctrl Pts',(16.2901178934933,14.1314756645001,2.82033062752701));
#28116=CARTESIAN_POINT('Ctrl Pts',(17.0802357869869,14.5876504430001,2.77866396086034));
#28117=CARTESIAN_POINT('Ctrl Pts',(17.0802357869869,15.5000000000002,2.73699729419368));
#28118=CARTESIAN_POINT('Ctrl Pts',(17.0802357869869,16.4123495570002,2.69533062752701));
#28119=CARTESIAN_POINT('Ctrl Pts',(16.2901178934933,16.8685243355002,2.65366396086034));
#28120=CARTESIAN_POINT('Ctrl Pts',(15.4999999999998,17.3246991140003,2.61199729419367));
#28121=CARTESIAN_POINT('Ctrl Pts',(14.7098821065064,16.8685243355002,2.57033062752701));
#28122=CARTESIAN_POINT('Ctrl Pts',(13.9197642130128,16.4123495570002,2.52866396086034));
#28123=CARTESIAN_POINT('Ctrl Pts',(13.9197642130128,15.5000000000001,2.48699729419367));
#28124=CARTESIAN_POINT('Ctrl Pts',(13.9197642130128,14.5876504430001,2.44533062752701));
#28125=CARTESIAN_POINT('Ctrl Pts',(14.7098821065064,14.1314756645001,2.40366396086034));
#28126=CARTESIAN_POINT('Ctrl Pts',(15.4999999999999,13.6753008860001,2.36199729419367));
#28127=CARTESIAN_POINT('Ctrl Pts',(16.2901178934933,14.1314756645001,2.32033062752701));
#28128=CARTESIAN_POINT('Ctrl Pts',(17.0802357869869,14.5876504430001,2.27866396086034));
#28129=CARTESIAN_POINT('Ctrl Pts',(17.0802357869869,15.5000000000002,2.23699729419367));
#28130=CARTESIAN_POINT('Ctrl Pts',(17.0802357869869,16.4123495570002,2.195330627527));
#28131=CARTESIAN_POINT('Ctrl Pts',(16.2901178934933,16.8685243355002,2.15366396086034));
#28132=CARTESIAN_POINT('Ctrl Pts',(15.4999999999998,17.3246991140003,2.11199729419367));
#28133=CARTESIAN_POINT('Ctrl Pts',(14.7098821065064,16.8685243355002,2.070330627527));
#28134=CARTESIAN_POINT('Ctrl Pts',(13.9197642130128,16.4123495570002,2.02866396086033));
#28135=CARTESIAN_POINT('Ctrl Pts',(13.9197642130128,15.5000000000001,1.98699729419367));
#28136=CARTESIAN_POINT('Ctrl Pts',(13.9197642130128,14.5876504430001,1.945330627527));
#28137=CARTESIAN_POINT('Ctrl Pts',(14.7098821065064,14.1314756645001,1.90366396086033));
#28138=CARTESIAN_POINT('Ctrl Pts',(15.4999999999999,13.6753008860001,1.86199729419367));
#28139=CARTESIAN_POINT('Ctrl Pts',(16.2901178934933,14.1314756645001,1.820330627527));
#28140=CARTESIAN_POINT('Ctrl Pts',(17.0802357869869,14.5876504430001,1.77866396086033));
#28141=CARTESIAN_POINT('Ctrl Pts',(17.0802357869869,15.5000000000002,1.73699729419366));
#28142=CARTESIAN_POINT('Ctrl Pts',(17.0802357869869,16.4123495570002,1.695330627527));
#28143=CARTESIAN_POINT('Ctrl Pts',(16.2901178934933,16.8685243355002,1.65366396086033));
#28144=CARTESIAN_POINT('Ctrl Pts',(15.4999999999998,17.3246991140003,1.61199729419366));
#28145=CARTESIAN_POINT('Ctrl Pts',(14.7098821065064,16.8685243355002,1.57033062752699));
#28146=CARTESIAN_POINT('Ctrl Pts',(13.9197642130128,16.4123495570002,1.52866396086033));
#28147=CARTESIAN_POINT('Ctrl Pts',(13.9197642130128,15.5000000000001,1.48699729419366));
#28148=CARTESIAN_POINT('Ctrl Pts',(13.9197642130128,14.5876504430001,1.44533062752699));
#28149=CARTESIAN_POINT('Ctrl Pts',(14.7098821065064,14.1314756645001,1.40366396086033));
#28150=CARTESIAN_POINT('Ctrl Pts',(15.4999999999999,13.6753008860001,1.36199729419366));
#28151=CARTESIAN_POINT('Ctrl Pts',(16.2901178934933,14.1314756645001,1.32033062752699));
#28152=CARTESIAN_POINT('Ctrl Pts',(17.0802357869869,14.5876504430001,1.27866396086032));
#28153=CARTESIAN_POINT('Ctrl Pts',(17.0802357869869,15.5000000000002,1.23699729419366));
#28154=CARTESIAN_POINT('Ctrl Pts',(17.0802357869869,16.4123495570002,1.19533062752699));
#28155=CARTESIAN_POINT('Ctrl Pts',(16.2901178934933,16.8685243355002,1.15366396086032));
#28156=CARTESIAN_POINT('Ctrl Pts',(15.4999999999998,17.3246991140003,1.11199729419366));
#28157=CARTESIAN_POINT('Ctrl Pts',(14.7098821065064,16.8685243355002,1.07033062752699));
#28158=CARTESIAN_POINT('Ctrl Pts',(13.9197642130128,16.4123495570002,1.02866396086032));
#28159=CARTESIAN_POINT('Ctrl Pts',(13.9197642130128,15.5000000000001,0.986997294193658));
#28160=CARTESIAN_POINT('Ctrl Pts',(13.9197642130128,14.5876504430001,0.945330627526991));
#28161=CARTESIAN_POINT('Ctrl Pts',(14.7098821065064,14.1314756645001,0.903663960860324));
#28162=CARTESIAN_POINT('Ctrl Pts',(15.4999999999999,13.6753008860001,0.861997294193656));
#28163=CARTESIAN_POINT('Ctrl Pts',(16.2901178934933,14.1314756645001,0.820330627526989));
#28164=CARTESIAN_POINT('Ctrl Pts',(17.0802357869869,14.5876504430001,0.778663960860322));
#28165=CARTESIAN_POINT('Ctrl Pts',(17.0802357869869,15.5000000000002,0.736997294193654));
#28166=CARTESIAN_POINT('Ctrl Pts',(17.0802357869869,16.4123495570002,0.695330627526987));
#28167=CARTESIAN_POINT('Ctrl Pts',(16.2901178934933,16.8685243355002,0.65366396086032));
#28168=CARTESIAN_POINT('Ctrl Pts',(15.4999999999998,17.3246991140003,0.611997294193653));
#28169=CARTESIAN_POINT('Ctrl Pts',(14.7098821065064,16.8685243355002,0.570330627526985));
#28170=CARTESIAN_POINT('Ctrl Pts',(13.9197642130128,16.4123495570002,0.528663960860318));
#28171=CARTESIAN_POINT('Ctrl Pts',(13.9197642130128,15.5000000000001,0.486997294193651));
#28172=CARTESIAN_POINT('Ctrl Pts',(13.9197642130128,14.5876504430001,0.445330627526983));
#28173=CARTESIAN_POINT('Ctrl Pts',(14.7098821065064,14.1314756645001,0.403663960860316));
#28174=CARTESIAN_POINT('Ctrl Pts',(15.4999999999999,13.6753008860001,0.361997294193649));
#28175=CARTESIAN_POINT('Ctrl Pts',(16.2901178934933,14.1314756645001,0.320330627526982));
#28176=CARTESIAN_POINT('Ctrl Pts',(17.0802357869869,14.5876504430001,0.278663960860314));
#28177=CARTESIAN_POINT('Ctrl Pts',(17.0802357869869,15.5000000000002,0.236997294193647));
#28178=CARTESIAN_POINT('Ctrl Pts',(17.0802357869869,16.4123495570002,0.19533062752698));
#28179=CARTESIAN_POINT('Ctrl Pts',(16.2901178934933,16.8685243355002,0.153663960860312));
#28180=CARTESIAN_POINT('Ctrl Pts',(15.4999999999998,17.3246991140003,0.111997294193645));
#28181=CARTESIAN_POINT('Ctrl Pts',(14.7098821065064,16.8685243355002,0.0703306275269777));
#28182=CARTESIAN_POINT('Ctrl Pts',(13.9197642130128,16.4123495570002,0.0286639608603104));
#28183=CARTESIAN_POINT('Ctrl Pts',(13.9197642130128,15.5000000000001,-0.0130027058063568));
#28184=CARTESIAN_POINT('Ctrl Pts',(13.9197642130128,14.5876504430001,-0.0546693724730224));
#28185=CARTESIAN_POINT('Ctrl Pts',(14.7098821065064,14.1314756645001,-0.0963360391396897));
#28186=CARTESIAN_POINT('Ctrl Pts',(15.4999999999999,13.6753008860001,-0.138002705806357));
#28187=CARTESIAN_POINT('Ctrl Pts',(16.2901178934933,14.1314756645001,-0.179669372473024));
#28188=CARTESIAN_POINT('Ctrl Pts',(17.0802357869869,14.5876504430001,-0.221336039139691));
#28189=CARTESIAN_POINT('Ctrl Pts',(17.0802357869869,15.5000000000002,-0.263002705806359));
#28190=CARTESIAN_POINT('Ctrl Pts',(17.0802357869869,16.4123495570002,-0.304669372473026));
#28191=CARTESIAN_POINT('Ctrl Pts',(16.2901178934933,16.8685243355002,-0.346336039139693));
#28192=CARTESIAN_POINT('Ctrl Pts',(15.4999999999998,17.3246991140003,-0.38800270580636));
#28193=CARTESIAN_POINT('Ctrl Pts',(14.7098821065064,16.8685243355002,-0.429669372473028));
#28194=CARTESIAN_POINT('Ctrl Pts',(13.9197642130128,16.4123495570002,-0.471336039139695));
#28195=CARTESIAN_POINT('Ctrl Pts',(13.9197642130128,15.5000000000001,-0.513002705806362));
#28196=CARTESIAN_POINT('Ctrl Pts',(13.9197642130128,14.5876504430001,-0.55466937247303));
#28197=CARTESIAN_POINT('Ctrl Pts',(14.7098821065064,14.1314756645001,-0.596336039139697));
#28198=CARTESIAN_POINT('Ctrl Pts',(15.4999999999999,13.6753008860001,-0.638002705806364));
#28199=CARTESIAN_POINT('Ctrl Pts',(16.2901178934933,14.1314756645001,-0.679669372473032));
#28200=CARTESIAN_POINT('Ctrl Pts',(17.0802357869869,14.5876504430001,-0.721336039139699));
#28201=CARTESIAN_POINT('Ctrl Pts',(17.0802357869869,15.5000000000002,-0.763002705806366));
#28202=CARTESIAN_POINT('Ctrl Pts',(17.0802357869869,16.4123495570002,-0.804669372473033));
#28203=CARTESIAN_POINT('Ctrl Pts',(16.2901178934933,16.8685243355002,-0.846336039139701));
#28204=CARTESIAN_POINT('Ctrl Pts',(15.4999999999998,17.3246991140003,-0.888002705806368));
#28205=CARTESIAN_POINT('Ctrl Pts',(14.7098821065064,16.8685243355002,-0.929669372473035));
#28206=CARTESIAN_POINT('Ctrl Pts',(13.9197642130128,16.4123495570002,-0.971336039139702));
#28207=CARTESIAN_POINT('Ctrl Pts',(13.9197642130128,15.5000000000001,-1.01300270580637));
#28208=CARTESIAN_POINT('Ctrl Pts',(13.9197642130128,14.5876504430001,-1.05466937247304));
#28209=CARTESIAN_POINT('Ctrl Pts',(14.7098821065064,14.1314756645001,-1.09633603913971));
#28210=CARTESIAN_POINT('Ctrl Pts',(15.4999999999999,13.6753008860001,-1.13800270580638));
#28211=CARTESIAN_POINT('Ctrl Pts',(16.2901178934933,14.1314756645001,-1.17966937247304));
#28212=CARTESIAN_POINT('Ctrl Pts',(17.0802357869869,14.5876504430001,-1.22133603913971));
#28213=CARTESIAN_POINT('Ctrl Pts',(17.0802357869869,15.5000000000002,-1.26300270580638));
#28214=CARTESIAN_POINT('Ctrl Pts',(17.0802357869869,16.4123495570002,-1.30466937247304));
#28215=CARTESIAN_POINT('Ctrl Pts',(16.2901178934933,16.8685243355002,-1.34633603913971));
#28216=CARTESIAN_POINT('Ctrl Pts',(15.4999999999998,17.3246991140003,-1.38800270580638));
#28217=CARTESIAN_POINT('Ctrl Pts',(14.7098821065064,16.8685243355002,-1.42966937247304));
#28218=CARTESIAN_POINT('Ctrl Pts',(13.9197642130128,16.4123495570002,-1.47133603913971));
#28219=CARTESIAN_POINT('Ctrl Pts',(13.9197642130128,15.5000000000001,-1.51300270580638));
#28220=CARTESIAN_POINT('Ctrl Pts',(13.9197642130128,14.5876504430001,-1.55466937247305));
#28221=CARTESIAN_POINT('Ctrl Pts',(14.7098821065064,14.1314756645001,-1.59633603913971));
#28222=CARTESIAN_POINT('Ctrl Pts',(15.4999999999999,13.6753008860001,-1.63800270580638));
#28223=CARTESIAN_POINT('Ctrl Pts',(16.2901178934933,14.1314756645001,-1.67966937247305));
#28224=CARTESIAN_POINT('Ctrl Pts',(17.0802357869869,14.5876504430001,-1.72133603913972));
#28225=CARTESIAN_POINT('Ctrl Pts',(17.0802357869869,15.5000000000002,-1.76300270580638));
#28226=CARTESIAN_POINT('Ctrl Pts',(17.0802357869869,16.4123495570002,-1.80466937247305));
#28227=CARTESIAN_POINT('Ctrl Pts',(16.2901178934933,16.8685243355002,-1.84633603913972));
#28228=CARTESIAN_POINT('Ctrl Pts',(15.4999999999998,17.3246991140003,-1.88800270580639));
#28229=CARTESIAN_POINT('Ctrl Pts',(14.7098821065064,16.8685243355002,-1.92966937247305));
#28230=CARTESIAN_POINT('Ctrl Pts',(14.4189874290229,16.7005762151493,-1.94500962949244));
#28231=CARTESIAN_POINT('Ctrl Pts',(14.2215547953295,16.4288288330635,-1.96262601180154));
#28232=CARTESIAN_POINT('',(14.2215509627455,16.4288315898518,-1.9626232418845));
#28233=CARTESIAN_POINT('',(14.2215500160355,16.4288304039467,-1.96262332703658));
#28234=CARTESIAN_POINT('Ctrl Pts',(14.5577749122401,14.231389800475,10.4122404735808));
#28235=CARTESIAN_POINT('Ctrl Pts',(14.6309457974486,14.177044152171,10.407829216981));
#28236=CARTESIAN_POINT('Ctrl Pts',(14.7098797632094,14.1314716057908,10.4036666666667));
#28237=CARTESIAN_POINT('Ctrl Pts',(15.4999999999999,13.6752954743877,10.362));
#28238=CARTESIAN_POINT('Ctrl Pts',(16.2901202367903,14.1314716057908,10.3203333333333));
#28239=CARTESIAN_POINT('Ctrl Pts',(17.0802404735807,14.5876477371939,10.2786666666667));
#28240=CARTESIAN_POINT('Ctrl Pts',(17.0802404735807,15.5000000000002,10.237));
#28241=CARTESIAN_POINT('Ctrl Pts',(17.0802404735807,16.4123522628064,10.1953333333333));
#28242=CARTESIAN_POINT('Ctrl Pts',(16.2901202367902,16.8685283942095,10.1536666666667));
#28243=CARTESIAN_POINT('Ctrl Pts',(15.4999999999998,17.3247045256126,10.112));
#28244=CARTESIAN_POINT('Ctrl Pts',(14.7098797632094,16.8685283942095,10.0703333333333));
#28245=CARTESIAN_POINT('Ctrl Pts',(13.919759526419,16.4123522628064,10.0286666666667));
#28246=CARTESIAN_POINT('Ctrl Pts',(13.919759526419,15.5000000000001,9.98699999999998));
#28247=CARTESIAN_POINT('Ctrl Pts',(13.919759526419,14.5876477371939,9.94533333333331));
#28248=CARTESIAN_POINT('Ctrl Pts',(14.7098797632094,14.1314716057908,9.90366666666665));
#28249=CARTESIAN_POINT('Ctrl Pts',(15.4999999999999,13.6752954743877,9.86199999999998));
#28250=CARTESIAN_POINT('Ctrl Pts',(16.2901202367903,14.1314716057908,9.82033333333331));
#28251=CARTESIAN_POINT('Ctrl Pts',(17.0802404735807,14.5876477371939,9.77866666666665));
#28252=CARTESIAN_POINT('Ctrl Pts',(17.0802404735807,15.5000000000002,9.73699999999998));
#28253=CARTESIAN_POINT('Ctrl Pts',(17.0802404735807,16.4123522628064,9.69533333333331));
#28254=CARTESIAN_POINT('Ctrl Pts',(16.2901202367902,16.8685283942095,9.65366666666664));
#28255=CARTESIAN_POINT('Ctrl Pts',(15.4999999999998,17.3247045256126,9.61199999999998));
#28256=CARTESIAN_POINT('Ctrl Pts',(14.7098797632094,16.8685283942095,9.57033333333331));
#28257=CARTESIAN_POINT('Ctrl Pts',(13.919759526419,16.4123522628064,9.52866666666664));
#28258=CARTESIAN_POINT('Ctrl Pts',(13.919759526419,15.5000000000001,9.48699999999998));
#28259=CARTESIAN_POINT('Ctrl Pts',(13.919759526419,14.5876477371939,9.44533333333331));
#28260=CARTESIAN_POINT('Ctrl Pts',(14.7098797632094,14.1314716057908,9.40366666666664));
#28261=CARTESIAN_POINT('Ctrl Pts',(15.4999999999999,13.6752954743877,9.36199999999998));
#28262=CARTESIAN_POINT('Ctrl Pts',(16.2901202367903,14.1314716057908,9.32033333333331));
#28263=CARTESIAN_POINT('Ctrl Pts',(17.0802404735807,14.5876477371939,9.27866666666664));
#28264=CARTESIAN_POINT('Ctrl Pts',(17.0802404735807,15.5000000000002,9.23699999999997));
#28265=CARTESIAN_POINT('Ctrl Pts',(17.0802404735807,16.4123522628064,9.19533333333331));
#28266=CARTESIAN_POINT('Ctrl Pts',(16.2901202367902,16.8685283942095,9.15366666666664));
#28267=CARTESIAN_POINT('Ctrl Pts',(15.4999999999998,17.3247045256126,9.11199999999997));
#28268=CARTESIAN_POINT('Ctrl Pts',(14.7098797632094,16.8685283942095,9.0703333333333));
#28269=CARTESIAN_POINT('Ctrl Pts',(13.919759526419,16.4123522628064,9.02866666666664));
#28270=CARTESIAN_POINT('Ctrl Pts',(13.919759526419,15.5000000000001,8.98699999999997));
#28271=CARTESIAN_POINT('Ctrl Pts',(13.919759526419,14.5876477371939,8.9453333333333));
#28272=CARTESIAN_POINT('Ctrl Pts',(14.7098797632094,14.1314716057908,8.90366666666664));
#28273=CARTESIAN_POINT('Ctrl Pts',(15.4999999999999,13.6752954743877,8.86199999999997));
#28274=CARTESIAN_POINT('Ctrl Pts',(16.2901202367903,14.1314716057908,8.8203333333333));
#28275=CARTESIAN_POINT('Ctrl Pts',(17.0802404735807,14.5876477371939,8.77866666666663));
#28276=CARTESIAN_POINT('Ctrl Pts',(17.0802404735807,15.5000000000002,8.73699999999997));
#28277=CARTESIAN_POINT('Ctrl Pts',(17.0802404735807,16.4123522628064,8.6953333333333));
#28278=CARTESIAN_POINT('Ctrl Pts',(16.2901202367902,16.8685283942095,8.65366666666663));
#28279=CARTESIAN_POINT('Ctrl Pts',(15.4999999999998,17.3247045256126,8.61199999999996));
#28280=CARTESIAN_POINT('Ctrl Pts',(14.7098797632094,16.8685283942095,8.57033333333329));
#28281=CARTESIAN_POINT('Ctrl Pts',(13.919759526419,16.4123522628064,8.52866666666663));
#28282=CARTESIAN_POINT('Ctrl Pts',(13.919759526419,15.5000000000001,8.48699999999996));
#28283=CARTESIAN_POINT('Ctrl Pts',(13.919759526419,14.5876477371939,8.44533333333329));
#28284=CARTESIAN_POINT('Ctrl Pts',(14.7098797632094,14.1314716057908,8.40366666666663));
#28285=CARTESIAN_POINT('Ctrl Pts',(15.4999999999999,13.6752954743877,8.36199999999996));
#28286=CARTESIAN_POINT('Ctrl Pts',(16.2901202367903,14.1314716057908,8.32033333333329));
#28287=CARTESIAN_POINT('Ctrl Pts',(17.0802404735807,14.5876477371939,8.27866666666663));
#28288=CARTESIAN_POINT('Ctrl Pts',(17.0802404735807,15.5000000000002,8.23699999999996));
#28289=CARTESIAN_POINT('Ctrl Pts',(17.0802404735807,16.4123522628064,8.19533333333329));
#28290=CARTESIAN_POINT('Ctrl Pts',(16.2901202367902,16.8685283942095,8.15366666666663));
#28291=CARTESIAN_POINT('Ctrl Pts',(15.4999999999998,17.3247045256126,8.11199999999996));
#28292=CARTESIAN_POINT('Ctrl Pts',(14.7098797632094,16.8685283942095,8.07033333333329));
#28293=CARTESIAN_POINT('Ctrl Pts',(13.919759526419,16.4123522628064,8.02866666666662));
#28294=CARTESIAN_POINT('Ctrl Pts',(13.919759526419,15.5000000000001,7.98699999999996));
#28295=CARTESIAN_POINT('Ctrl Pts',(13.919759526419,14.5876477371939,7.94533333333329));
#28296=CARTESIAN_POINT('Ctrl Pts',(14.7098797632094,14.1314716057908,7.90366666666662));
#28297=CARTESIAN_POINT('Ctrl Pts',(15.4999999999999,13.6752954743877,7.86199999999995));
#28298=CARTESIAN_POINT('Ctrl Pts',(16.2901202367903,14.1314716057908,7.82033333333329));
#28299=CARTESIAN_POINT('Ctrl Pts',(17.0802404735807,14.5876477371939,7.77866666666662));
#28300=CARTESIAN_POINT('Ctrl Pts',(17.0802404735807,15.5000000000002,7.73699999999995));
#28301=CARTESIAN_POINT('Ctrl Pts',(17.0802404735807,16.4123522628064,7.69533333333329));
#28302=CARTESIAN_POINT('Ctrl Pts',(16.2901202367902,16.8685283942095,7.65366666666662));
#28303=CARTESIAN_POINT('Ctrl Pts',(15.4999999999998,17.3247045256126,7.61199999999995));
#28304=CARTESIAN_POINT('Ctrl Pts',(14.7098797632094,16.8685283942095,7.57033333333328));
#28305=CARTESIAN_POINT('Ctrl Pts',(13.919759526419,16.4123522628064,7.52866666666662));
#28306=CARTESIAN_POINT('Ctrl Pts',(13.919759526419,15.5000000000001,7.48699999999995));
#28307=CARTESIAN_POINT('Ctrl Pts',(13.919759526419,14.5876477371939,7.44533333333328));
#28308=CARTESIAN_POINT('Ctrl Pts',(14.7098797632094,14.1314716057908,7.40366666666661));
#28309=CARTESIAN_POINT('Ctrl Pts',(15.4999999999999,13.6752954743877,7.36199999999995));
#28310=CARTESIAN_POINT('Ctrl Pts',(16.2901202367903,14.1314716057908,7.32033333333328));
#28311=CARTESIAN_POINT('Ctrl Pts',(17.0802404735807,14.5876477371939,7.27866666666661));
#28312=CARTESIAN_POINT('Ctrl Pts',(17.0802404735807,15.5000000000002,7.23699999999995));
#28313=CARTESIAN_POINT('Ctrl Pts',(17.0802404735807,16.4123522628064,7.19533333333328));
#28314=CARTESIAN_POINT('Ctrl Pts',(16.2901202367902,16.8685283942095,7.15366666666661));
#28315=CARTESIAN_POINT('Ctrl Pts',(15.4999999999998,17.3247045256126,7.11199999999994));
#28316=CARTESIAN_POINT('Ctrl Pts',(14.7098797632094,16.8685283942095,7.07033333333328));
#28317=CARTESIAN_POINT('Ctrl Pts',(13.919759526419,16.4123522628064,7.02866666666661));
#28318=CARTESIAN_POINT('Ctrl Pts',(13.919759526419,15.5000000000001,6.98699999999994));
#28319=CARTESIAN_POINT('Ctrl Pts',(13.919759526419,14.5876477371939,6.94533333333327));
#28320=CARTESIAN_POINT('Ctrl Pts',(14.7098797632094,14.1314716057908,6.90366666666661));
#28321=CARTESIAN_POINT('Ctrl Pts',(15.4999999999999,13.6752954743877,6.86199999999994));
#28322=CARTESIAN_POINT('Ctrl Pts',(16.2901202367903,14.1314716057908,6.82033333333327));
#28323=CARTESIAN_POINT('Ctrl Pts',(17.0802404735807,14.5876477371939,6.77866666666661));
#28324=CARTESIAN_POINT('Ctrl Pts',(17.0802404735807,15.5000000000002,6.73699999999994));
#28325=CARTESIAN_POINT('Ctrl Pts',(17.0802404735807,16.4123522628064,6.69533333333327));
#28326=CARTESIAN_POINT('Ctrl Pts',(16.2901202367902,16.8685283942095,6.65366666666661));
#28327=CARTESIAN_POINT('Ctrl Pts',(15.4999999999998,17.3247045256126,6.61199999999994));
#28328=CARTESIAN_POINT('Ctrl Pts',(14.7098797632094,16.8685283942095,6.57033333333327));
#28329=CARTESIAN_POINT('Ctrl Pts',(13.919759526419,16.4123522628064,6.5286666666666));
#28330=CARTESIAN_POINT('Ctrl Pts',(13.919759526419,15.5000000000001,6.48699999999994));
#28331=CARTESIAN_POINT('Ctrl Pts',(13.919759526419,14.5876477371939,6.44533333333327));
#28332=CARTESIAN_POINT('Ctrl Pts',(14.7098797632094,14.1314716057908,6.4036666666666));
#28333=CARTESIAN_POINT('Ctrl Pts',(15.4999999999999,13.6752954743877,6.36199999999993));
#28334=CARTESIAN_POINT('Ctrl Pts',(16.2901202367903,14.1314716057908,6.32033333333327));
#28335=CARTESIAN_POINT('Ctrl Pts',(17.0802404735807,14.5876477371939,6.2786666666666));
#28336=CARTESIAN_POINT('Ctrl Pts',(17.0802404735807,15.5000000000002,6.23699999999993));
#28337=CARTESIAN_POINT('Ctrl Pts',(17.0802404735807,16.4123522628064,6.19533333333326));
#28338=CARTESIAN_POINT('Ctrl Pts',(16.2901202367902,16.8685283942095,6.1536666666666));
#28339=CARTESIAN_POINT('Ctrl Pts',(15.4999999999998,17.3247045256126,6.11199999999993));
#28340=CARTESIAN_POINT('Ctrl Pts',(14.7098797632094,16.8685283942095,6.07033333333326));
#28341=CARTESIAN_POINT('Ctrl Pts',(13.919759526419,16.4123522628064,6.0286666666666));
#28342=CARTESIAN_POINT('Ctrl Pts',(13.919759526419,15.5000000000001,5.98699999999993));
#28343=CARTESIAN_POINT('Ctrl Pts',(13.919759526419,14.5876477371939,5.94533333333326));
#28344=CARTESIAN_POINT('Ctrl Pts',(14.7098797632094,14.1314716057908,5.9036666666666));
#28345=CARTESIAN_POINT('Ctrl Pts',(15.4999999999999,13.6752954743877,5.86199999999993));
#28346=CARTESIAN_POINT('Ctrl Pts',(16.2901202367903,14.1314716057908,5.82033333333326));
#28347=CARTESIAN_POINT('Ctrl Pts',(17.0802404735807,14.5876477371939,5.77866666666659));
#28348=CARTESIAN_POINT('Ctrl Pts',(17.0802404735807,15.5000000000002,5.73699999999993));
#28349=CARTESIAN_POINT('Ctrl Pts',(17.0802404735807,16.4123522628064,5.69533333333326));
#28350=CARTESIAN_POINT('Ctrl Pts',(16.2901202367902,16.8685283942095,5.65366666666659));
#28351=CARTESIAN_POINT('Ctrl Pts',(15.4999999999998,17.3247045256126,5.61199999999992));
#28352=CARTESIAN_POINT('Ctrl Pts',(14.7098797632094,16.8685283942095,5.57033333333326));
#28353=CARTESIAN_POINT('Ctrl Pts',(13.919759526419,16.4123522628064,5.52866666666659));
#28354=CARTESIAN_POINT('Ctrl Pts',(13.919759526419,15.5000000000001,5.48699999999992));
#28355=CARTESIAN_POINT('Ctrl Pts',(13.919759526419,14.5876477371939,5.44533333333326));
#28356=CARTESIAN_POINT('Ctrl Pts',(14.7098797632094,14.1314716057908,5.40366666666659));
#28357=CARTESIAN_POINT('Ctrl Pts',(15.4999999999999,13.6752954743877,5.36199999999992));
#28358=CARTESIAN_POINT('Ctrl Pts',(16.2901202367903,14.1314716057908,5.32033333333325));
#28359=CARTESIAN_POINT('Ctrl Pts',(17.0802404735807,14.5876477371939,5.27866666666659));
#28360=CARTESIAN_POINT('Ctrl Pts',(17.0802404735807,15.5000000000002,5.23699999999992));
#28361=CARTESIAN_POINT('Ctrl Pts',(17.0802404735807,16.4123522628064,5.19533333333325));
#28362=CARTESIAN_POINT('Ctrl Pts',(16.2901202367902,16.8685283942095,5.15366666666658));
#28363=CARTESIAN_POINT('Ctrl Pts',(15.4999999999998,17.3247045256126,5.11199999999992));
#28364=CARTESIAN_POINT('Ctrl Pts',(14.7098797632094,16.8685283942095,5.07033333333325));
#28365=CARTESIAN_POINT('Ctrl Pts',(13.919759526419,16.4123522628064,5.02866666666658));
#28366=CARTESIAN_POINT('Ctrl Pts',(13.919759526419,15.5000000000001,4.98699999999992));
#28367=CARTESIAN_POINT('Ctrl Pts',(13.919759526419,14.5876477371939,4.94533333333325));
#28368=CARTESIAN_POINT('Ctrl Pts',(14.7098797632094,14.1314716057908,4.90366666666658));
#28369=CARTESIAN_POINT('Ctrl Pts',(15.4999999999999,13.6752954743877,4.86199999999991));
#28370=CARTESIAN_POINT('Ctrl Pts',(16.2901202367903,14.1314716057908,4.82033333333325));
#28371=CARTESIAN_POINT('Ctrl Pts',(17.0802404735807,14.5876477371939,4.77866666666658));
#28372=CARTESIAN_POINT('Ctrl Pts',(17.0802404735807,15.5000000000002,4.73699999999991));
#28373=CARTESIAN_POINT('Ctrl Pts',(17.0802404735807,16.4123522628064,4.69533333333325));
#28374=CARTESIAN_POINT('Ctrl Pts',(16.2901202367902,16.8685283942095,4.65366666666658));
#28375=CARTESIAN_POINT('Ctrl Pts',(15.4999999999998,17.3247045256126,4.61199999999991));
#28376=CARTESIAN_POINT('Ctrl Pts',(14.7098797632094,16.8685283942095,4.57033333333324));
#28377=CARTESIAN_POINT('Ctrl Pts',(13.919759526419,16.4123522628064,4.52866666666658));
#28378=CARTESIAN_POINT('Ctrl Pts',(13.919759526419,15.5000000000001,4.48699999999991));
#28379=CARTESIAN_POINT('Ctrl Pts',(13.919759526419,14.5876477371939,4.44533333333324));
#28380=CARTESIAN_POINT('Ctrl Pts',(14.7098797632094,14.1314716057908,4.40366666666658));
#28381=CARTESIAN_POINT('Ctrl Pts',(15.4999999999999,13.6752954743877,4.36199999999991));
#28382=CARTESIAN_POINT('Ctrl Pts',(16.2901202367903,14.1314716057908,4.32033333333324));
#28383=CARTESIAN_POINT('Ctrl Pts',(17.0802404735807,14.5876477371939,4.27866666666657));
#28384=CARTESIAN_POINT('Ctrl Pts',(17.0802404735807,15.5000000000002,4.23699999999991));
#28385=CARTESIAN_POINT('Ctrl Pts',(17.0802404735807,16.4123522628064,4.19533333333324));
#28386=CARTESIAN_POINT('Ctrl Pts',(16.2901202367902,16.8685283942095,4.15366666666657));
#28387=CARTESIAN_POINT('Ctrl Pts',(15.4999999999998,17.3247045256126,4.1119999999999));
#28388=CARTESIAN_POINT('Ctrl Pts',(14.7098797632094,16.8685283942095,4.07033333333324));
#28389=CARTESIAN_POINT('Ctrl Pts',(13.919759526419,16.4123522628064,4.02866666666657));
#28390=CARTESIAN_POINT('Ctrl Pts',(13.919759526419,15.5000000000001,3.9869999999999));
#28391=CARTESIAN_POINT('Ctrl Pts',(13.919759526419,14.5876477371939,3.94533333333323));
#28392=CARTESIAN_POINT('Ctrl Pts',(14.7098797632094,14.1314716057908,3.90366666666657));
#28393=CARTESIAN_POINT('Ctrl Pts',(15.4999999999999,13.6752954743877,3.8619999999999));
#28394=CARTESIAN_POINT('Ctrl Pts',(16.2901202367903,14.1314716057908,3.82033333333323));
#28395=CARTESIAN_POINT('Ctrl Pts',(17.0802404735807,14.5876477371939,3.77866666666657));
#28396=CARTESIAN_POINT('Ctrl Pts',(17.0802404735807,15.5000000000002,3.7369999999999));
#28397=CARTESIAN_POINT('Ctrl Pts',(17.0802404735807,16.4123522628064,3.69533333333323));
#28398=CARTESIAN_POINT('Ctrl Pts',(16.2901202367902,16.8685283942095,3.65366666666656));
#28399=CARTESIAN_POINT('Ctrl Pts',(15.4999999999998,17.3247045256126,3.6119999999999));
#28400=CARTESIAN_POINT('Ctrl Pts',(14.7098797632094,16.8685283942095,3.57033333333323));
#28401=CARTESIAN_POINT('Ctrl Pts',(13.919759526419,16.4123522628064,3.52866666666656));
#28402=CARTESIAN_POINT('Ctrl Pts',(13.919759526419,15.5000000000001,3.4869999999999));
#28403=CARTESIAN_POINT('Ctrl Pts',(13.919759526419,14.5876477371939,3.44533333333323));
#28404=CARTESIAN_POINT('Ctrl Pts',(14.7098797632094,14.1314716057908,3.40366666666656));
#28405=CARTESIAN_POINT('Ctrl Pts',(15.4999999999999,13.6752954743877,3.36199999999989));
#28406=CARTESIAN_POINT('Ctrl Pts',(16.2901202367903,14.1314716057908,3.32033333333323));
#28407=CARTESIAN_POINT('Ctrl Pts',(17.0802404735807,14.5876477371939,3.27866666666656));
#28408=CARTESIAN_POINT('Ctrl Pts',(17.0802404735807,15.5000000000002,3.23699999999989));
#28409=CARTESIAN_POINT('Ctrl Pts',(17.0802404735807,16.4123522628064,3.19533333333323));
#28410=CARTESIAN_POINT('Ctrl Pts',(16.2901202367902,16.8685283942095,3.15366666666656));
#28411=CARTESIAN_POINT('Ctrl Pts',(15.4999999999998,17.3247045256126,3.11199999999989));
#28412=CARTESIAN_POINT('Ctrl Pts',(14.7098797632094,16.8685283942095,3.07033333333322));
#28413=CARTESIAN_POINT('Ctrl Pts',(13.919759526419,16.4123522628064,3.02866666666656));
#28414=CARTESIAN_POINT('Ctrl Pts',(13.919759526419,15.5000000000001,2.98699999999989));
#28415=CARTESIAN_POINT('Ctrl Pts',(13.919759526419,14.5876477371939,2.94533333333322));
#28416=CARTESIAN_POINT('Ctrl Pts',(14.7098797632094,14.1314716057908,2.90366666666656));
#28417=CARTESIAN_POINT('Ctrl Pts',(15.4999999999999,13.6752954743877,2.86199999999989));
#28418=CARTESIAN_POINT('Ctrl Pts',(16.2901202367903,14.1314716057908,2.82033333333322));
#28419=CARTESIAN_POINT('Ctrl Pts',(17.0802404735807,14.5876477371939,2.77866666666655));
#28420=CARTESIAN_POINT('Ctrl Pts',(17.0802404735807,15.5000000000002,2.73699999999989));
#28421=CARTESIAN_POINT('Ctrl Pts',(17.0802404735807,16.4123522628064,2.69533333333322));
#28422=CARTESIAN_POINT('Ctrl Pts',(16.2901202367902,16.8685283942095,2.65366666666655));
#28423=CARTESIAN_POINT('Ctrl Pts',(15.4999999999998,17.3247045256126,2.61199999999988));
#28424=CARTESIAN_POINT('Ctrl Pts',(14.7098797632094,16.8685283942095,2.57033333333322));
#28425=CARTESIAN_POINT('Ctrl Pts',(13.919759526419,16.4123522628064,2.52866666666655));
#28426=CARTESIAN_POINT('Ctrl Pts',(13.919759526419,15.5000000000001,2.48699999999988));
#28427=CARTESIAN_POINT('Ctrl Pts',(13.919759526419,14.5876477371939,2.44533333333321));
#28428=CARTESIAN_POINT('Ctrl Pts',(14.7098797632094,14.1314716057908,2.40366666666655));
#28429=CARTESIAN_POINT('Ctrl Pts',(15.4999999999999,13.6752954743877,2.36199999999988));
#28430=CARTESIAN_POINT('Ctrl Pts',(16.2901202367903,14.1314716057908,2.32033333333321));
#28431=CARTESIAN_POINT('Ctrl Pts',(17.0802404735807,14.5876477371939,2.27866666666655));
#28432=CARTESIAN_POINT('Ctrl Pts',(17.0802404735807,15.5000000000002,2.23699999999988));
#28433=CARTESIAN_POINT('Ctrl Pts',(17.0802404735807,16.4123522628064,2.19533333333321));
#28434=CARTESIAN_POINT('Ctrl Pts',(16.2901202367902,16.8685283942095,2.15366666666655));
#28435=CARTESIAN_POINT('Ctrl Pts',(15.4999999999998,17.3247045256126,2.11199999999988));
#28436=CARTESIAN_POINT('Ctrl Pts',(14.7098797632094,16.8685283942095,2.07033333333321));
#28437=CARTESIAN_POINT('Ctrl Pts',(13.919759526419,16.4123522628064,2.02866666666654));
#28438=CARTESIAN_POINT('Ctrl Pts',(13.919759526419,15.5000000000001,1.98699999999988));
#28439=CARTESIAN_POINT('Ctrl Pts',(13.919759526419,14.5876477371939,1.94533333333321));
#28440=CARTESIAN_POINT('Ctrl Pts',(14.7098797632094,14.1314716057908,1.90366666666654));
#28441=CARTESIAN_POINT('Ctrl Pts',(15.4999999999999,13.6752954743877,1.86199999999987));
#28442=CARTESIAN_POINT('Ctrl Pts',(16.2901202367903,14.1314716057908,1.82033333333321));
#28443=CARTESIAN_POINT('Ctrl Pts',(17.0802404735807,14.5876477371939,1.77866666666654));
#28444=CARTESIAN_POINT('Ctrl Pts',(17.0802404735807,15.5000000000002,1.73699999999987));
#28445=CARTESIAN_POINT('Ctrl Pts',(17.0802404735807,16.4123522628064,1.6953333333332));
#28446=CARTESIAN_POINT('Ctrl Pts',(16.2901202367902,16.8685283942095,1.65366666666654));
#28447=CARTESIAN_POINT('Ctrl Pts',(15.4999999999998,17.3247045256126,1.61199999999987));
#28448=CARTESIAN_POINT('Ctrl Pts',(14.7098797632094,16.8685283942095,1.5703333333332));
#28449=CARTESIAN_POINT('Ctrl Pts',(13.919759526419,16.4123522628064,1.52866666666654));
#28450=CARTESIAN_POINT('Ctrl Pts',(13.919759526419,15.5000000000001,1.48699999999987));
#28451=CARTESIAN_POINT('Ctrl Pts',(13.919759526419,14.5876477371939,1.4453333333332));
#28452=CARTESIAN_POINT('Ctrl Pts',(14.7098797632094,14.1314716057908,1.40366666666653));
#28453=CARTESIAN_POINT('Ctrl Pts',(15.4999999999999,13.6752954743877,1.36199999999987));
#28454=CARTESIAN_POINT('Ctrl Pts',(16.2901202367903,14.1314716057908,1.3203333333332));
#28455=CARTESIAN_POINT('Ctrl Pts',(17.0802404735807,14.5876477371939,1.27866666666653));
#28456=CARTESIAN_POINT('Ctrl Pts',(17.0802404735807,15.5000000000002,1.23699999999987));
#28457=CARTESIAN_POINT('Ctrl Pts',(17.0802404735807,16.4123522628064,1.1953333333332));
#28458=CARTESIAN_POINT('Ctrl Pts',(16.2901202367902,16.8685283942095,1.15366666666653));
#28459=CARTESIAN_POINT('Ctrl Pts',(15.4999999999998,17.3247045256126,1.11199999999986));
#28460=CARTESIAN_POINT('Ctrl Pts',(14.7098797632094,16.8685283942095,1.0703333333332));
#28461=CARTESIAN_POINT('Ctrl Pts',(13.919759526419,16.4123522628064,1.02866666666653));
#28462=CARTESIAN_POINT('Ctrl Pts',(13.919759526419,15.5000000000001,0.986999999999863));
#28463=CARTESIAN_POINT('Ctrl Pts',(13.919759526419,14.5876477371939,0.945333333333196));
#28464=CARTESIAN_POINT('Ctrl Pts',(14.7098797632094,14.1314716057908,0.903666666666529));
#28465=CARTESIAN_POINT('Ctrl Pts',(15.4999999999999,13.6752954743877,0.861999999999861));
#28466=CARTESIAN_POINT('Ctrl Pts',(16.2901202367903,14.1314716057908,0.820333333333194));
#28467=CARTESIAN_POINT('Ctrl Pts',(17.0802404735807,14.5876477371939,0.778666666666527));
#28468=CARTESIAN_POINT('Ctrl Pts',(17.0802404735807,15.5000000000002,0.736999999999859));
#28469=CARTESIAN_POINT('Ctrl Pts',(17.0802404735807,16.4123522628064,0.695333333333192));
#28470=CARTESIAN_POINT('Ctrl Pts',(16.2901202367902,16.8685283942095,0.653666666666525));
#28471=CARTESIAN_POINT('Ctrl Pts',(15.4999999999998,17.3247045256126,0.611999999999858));
#28472=CARTESIAN_POINT('Ctrl Pts',(14.7098797632094,16.8685283942095,0.57033333333319));
#28473=CARTESIAN_POINT('Ctrl Pts',(13.919759526419,16.4123522628064,0.528666666666523));
#28474=CARTESIAN_POINT('Ctrl Pts',(13.919759526419,15.5000000000001,0.486999999999856));
#28475=CARTESIAN_POINT('Ctrl Pts',(13.919759526419,14.5876477371939,0.445333333333188));
#28476=CARTESIAN_POINT('Ctrl Pts',(14.7098797632094,14.1314716057908,0.403666666666521));
#28477=CARTESIAN_POINT('Ctrl Pts',(15.4999999999999,13.6752954743877,0.361999999999854));
#28478=CARTESIAN_POINT('Ctrl Pts',(16.2901202367903,14.1314716057908,0.320333333333186));
#28479=CARTESIAN_POINT('Ctrl Pts',(17.0802404735807,14.5876477371939,0.278666666666519));
#28480=CARTESIAN_POINT('Ctrl Pts',(17.0802404735807,15.5000000000002,0.236999999999852));
#28481=CARTESIAN_POINT('Ctrl Pts',(17.0802404735807,16.4123522628064,0.195333333333185));
#28482=CARTESIAN_POINT('Ctrl Pts',(16.2901202367902,16.8685283942095,0.153666666666517));
#28483=CARTESIAN_POINT('Ctrl Pts',(15.4999999999998,17.3247045256126,0.11199999999985));
#28484=CARTESIAN_POINT('Ctrl Pts',(14.7098797632094,16.8685283942095,0.0703333333331828));
#28485=CARTESIAN_POINT('Ctrl Pts',(13.919759526419,16.4123522628064,0.0286666666665155));
#28486=CARTESIAN_POINT('Ctrl Pts',(13.919759526419,15.5000000000001,-0.0130000000001518));
#28487=CARTESIAN_POINT('Ctrl Pts',(13.919759526419,14.5876477371939,-0.0546666666668173));
#28488=CARTESIAN_POINT('Ctrl Pts',(14.7098797632094,14.1314716057908,-0.0963333333334846));
#28489=CARTESIAN_POINT('Ctrl Pts',(15.4999999999999,13.6752954743877,-0.138000000000152));
#28490=CARTESIAN_POINT('Ctrl Pts',(16.2901202367903,14.1314716057908,-0.179666666666819));
#28491=CARTESIAN_POINT('Ctrl Pts',(17.0802404735807,14.5876477371939,-0.221333333333486));
#28492=CARTESIAN_POINT('Ctrl Pts',(17.0802404735807,15.5000000000002,-0.263000000000154));
#28493=CARTESIAN_POINT('Ctrl Pts',(17.0802404735807,16.4123522628064,-0.304666666666821));
#28494=CARTESIAN_POINT('Ctrl Pts',(16.2901202367902,16.8685283942095,-0.346333333333488));
#28495=CARTESIAN_POINT('Ctrl Pts',(15.4999999999998,17.3247045256126,-0.388000000000156));
#28496=CARTESIAN_POINT('Ctrl Pts',(14.7098797632094,16.8685283942095,-0.429666666666823));
#28497=CARTESIAN_POINT('Ctrl Pts',(13.919759526419,16.4123522628064,-0.47133333333349));
#28498=CARTESIAN_POINT('Ctrl Pts',(13.919759526419,15.5000000000001,-0.513000000000157));
#28499=CARTESIAN_POINT('Ctrl Pts',(13.919759526419,14.5876477371939,-0.554666666666825));
#28500=CARTESIAN_POINT('Ctrl Pts',(14.7098797632094,14.1314716057908,-0.596333333333492));
#28501=CARTESIAN_POINT('Ctrl Pts',(15.4999999999999,13.6752954743877,-0.638000000000159));
#28502=CARTESIAN_POINT('Ctrl Pts',(16.2901202367903,14.1314716057908,-0.679666666666827));
#28503=CARTESIAN_POINT('Ctrl Pts',(17.0802404735807,14.5876477371939,-0.721333333333494));
#28504=CARTESIAN_POINT('Ctrl Pts',(17.0802404735807,15.5000000000002,-0.763000000000161));
#28505=CARTESIAN_POINT('Ctrl Pts',(17.0802404735807,16.4123522628064,-0.804666666666829));
#28506=CARTESIAN_POINT('Ctrl Pts',(16.2901202367902,16.8685283942095,-0.846333333333496));
#28507=CARTESIAN_POINT('Ctrl Pts',(15.4999999999998,17.3247045256126,-0.888000000000163));
#28508=CARTESIAN_POINT('Ctrl Pts',(14.7098797632094,16.8685283942095,-0.92966666666683));
#28509=CARTESIAN_POINT('Ctrl Pts',(13.919759526419,16.4123522628064,-0.971333333333498));
#28510=CARTESIAN_POINT('Ctrl Pts',(13.919759526419,15.5000000000001,-1.01300000000016));
#28511=CARTESIAN_POINT('Ctrl Pts',(13.919759526419,14.5876477371939,-1.05466666666683));
#28512=CARTESIAN_POINT('Ctrl Pts',(14.7098797632094,14.1314716057908,-1.0963333333335));
#28513=CARTESIAN_POINT('Ctrl Pts',(15.4999999999999,13.6752954743877,-1.13800000000017));
#28514=CARTESIAN_POINT('Ctrl Pts',(16.2901202367903,14.1314716057908,-1.17966666666683));
#28515=CARTESIAN_POINT('Ctrl Pts',(17.0802404735807,14.5876477371939,-1.2213333333335));
#28516=CARTESIAN_POINT('Ctrl Pts',(17.0802404735807,15.5000000000002,-1.26300000000017));
#28517=CARTESIAN_POINT('Ctrl Pts',(17.0802404735807,16.4123522628064,-1.30466666666683));
#28518=CARTESIAN_POINT('Ctrl Pts',(16.2901202367902,16.8685283942095,-1.3463333333335));
#28519=CARTESIAN_POINT('Ctrl Pts',(15.4999999999998,17.3247045256126,-1.38800000000017));
#28520=CARTESIAN_POINT('Ctrl Pts',(14.7098797632094,16.8685283942095,-1.42966666666684));
#28521=CARTESIAN_POINT('Ctrl Pts',(13.919759526419,16.4123522628064,-1.4713333333335));
#28522=CARTESIAN_POINT('Ctrl Pts',(13.919759526419,15.5000000000001,-1.51300000000017));
#28523=CARTESIAN_POINT('Ctrl Pts',(13.919759526419,14.5876477371939,-1.55466666666684));
#28524=CARTESIAN_POINT('Ctrl Pts',(14.7098797632094,14.1314716057908,-1.59633333333351));
#28525=CARTESIAN_POINT('Ctrl Pts',(15.4999999999999,13.6752954743877,-1.63800000000017));
#28526=CARTESIAN_POINT('Ctrl Pts',(16.2901202367903,14.1314716057908,-1.67966666666684));
#28527=CARTESIAN_POINT('Ctrl Pts',(17.0802404735807,14.5876477371939,-1.72133333333351));
#28528=CARTESIAN_POINT('Ctrl Pts',(17.0802404735807,15.5000000000002,-1.76300000000017));
#28529=CARTESIAN_POINT('Ctrl Pts',(17.0802404735807,16.4123522628064,-1.80466666666684));
#28530=CARTESIAN_POINT('Ctrl Pts',(16.2901202367902,16.8685283942095,-1.84633333333351));
#28531=CARTESIAN_POINT('Ctrl Pts',(15.4999999999998,17.3247045256126,-1.88800000000018));
#28532=CARTESIAN_POINT('Ctrl Pts',(14.7098797632094,16.8685283942095,-1.92966666666684));
#28533=CARTESIAN_POINT('Ctrl Pts',(14.4189900731897,16.7005831533722,-1.94500661517905));
#28534=CARTESIAN_POINT('Ctrl Pts',(14.221552772606,16.4288340223701,-1.96262314816781));
#28535=CARTESIAN_POINT('Origin',(14.0080754615184,16.5839252605848,-2.17746715486548));
#28536=CARTESIAN_POINT('',(14.2215498957102,16.428830062579,-2.02512301642217));
#28537=CARTESIAN_POINT('Ctrl Pts',(17.0802404735807,15.5000000000002,11.2370201234482));
#28538=CARTESIAN_POINT('Ctrl Pts',(17.0802404735807,16.4123522628064,11.1953534567815));
#28539=CARTESIAN_POINT('Ctrl Pts',(16.2901202367902,16.8685283942095,11.1536867901149));
#28540=CARTESIAN_POINT('Ctrl Pts',(15.4999999999998,17.3247045256126,11.1120201234482));
#28541=CARTESIAN_POINT('Ctrl Pts',(14.7098797632094,16.8685283942095,11.0703534567815));
#28542=CARTESIAN_POINT('Ctrl Pts',(13.919759526419,16.4123522628064,11.0286867901149));
#28543=CARTESIAN_POINT('Ctrl Pts',(13.919759526419,15.5000000000001,10.9870201234482));
#28544=CARTESIAN_POINT('Ctrl Pts',(13.919759526419,14.5876477371939,10.9453534567815));
#28545=CARTESIAN_POINT('Ctrl Pts',(14.7098797632094,14.1314716057908,10.9036867901149));
#28546=CARTESIAN_POINT('Ctrl Pts',(15.4999999999999,13.6752954743877,10.8620201234482));
#28547=CARTESIAN_POINT('Ctrl Pts',(16.2901202367903,14.1314716057908,10.8203534567815));
#28548=CARTESIAN_POINT('Ctrl Pts',(17.0802404735807,14.5876477371939,10.7786867901149));
#28549=CARTESIAN_POINT('Ctrl Pts',(17.0802404735807,15.5000000000002,10.7370201234482));
#28550=CARTESIAN_POINT('Ctrl Pts',(17.0802404735807,16.4123522628064,10.6953534567815));
#28551=CARTESIAN_POINT('Ctrl Pts',(16.2901202367902,16.8685283942095,10.6536867901149));
#28552=CARTESIAN_POINT('Ctrl Pts',(15.4999999999998,17.3247045256126,10.6120201234482));
#28553=CARTESIAN_POINT('Ctrl Pts',(14.7098797632094,16.8685283942095,10.5703534567815));
#28554=CARTESIAN_POINT('Ctrl Pts',(13.919759526419,16.4123522628064,10.5286867901149));
#28555=CARTESIAN_POINT('Ctrl Pts',(13.919759526419,15.5000000000001,10.4870201234482));
#28556=CARTESIAN_POINT('Ctrl Pts',(13.919759526419,14.5876477371939,10.4453534567815));
#28557=CARTESIAN_POINT('Ctrl Pts',(14.7098797632094,14.1314716057908,10.4036867901149));
#28558=CARTESIAN_POINT('Ctrl Pts',(15.4999999999999,13.6752954743877,10.3620201234482));
#28559=CARTESIAN_POINT('Ctrl Pts',(16.2901202367903,14.1314716057908,10.3203534567815));
#28560=CARTESIAN_POINT('Ctrl Pts',(17.0802404735807,14.5876477371939,10.2786867901149));
#28561=CARTESIAN_POINT('Ctrl Pts',(17.0802404735807,15.5000000000002,10.2370201234482));
#28562=CARTESIAN_POINT('Ctrl Pts',(17.0802404735807,16.4123522628064,10.1953534567815));
#28563=CARTESIAN_POINT('Ctrl Pts',(16.2901202367902,16.8685283942095,10.1536867901149));
#28564=CARTESIAN_POINT('Ctrl Pts',(15.4999999999998,17.3247045256126,10.1120201234482));
#28565=CARTESIAN_POINT('Ctrl Pts',(14.7098797632094,16.8685283942095,10.0703534567815));
#28566=CARTESIAN_POINT('Ctrl Pts',(13.919759526419,16.4123522628064,10.0286867901149));
#28567=CARTESIAN_POINT('Ctrl Pts',(13.919759526419,15.5000000000001,9.98702012344819));
#28568=CARTESIAN_POINT('Ctrl Pts',(13.919759526419,14.5876477371939,9.94535345678152));
#28569=CARTESIAN_POINT('Ctrl Pts',(14.7098797632094,14.1314716057908,9.90368679011485));
#28570=CARTESIAN_POINT('Ctrl Pts',(15.4999999999999,13.6752954743877,9.86202012344818));
#28571=CARTESIAN_POINT('Ctrl Pts',(16.2901202367903,14.1314716057908,9.82035345678152));
#28572=CARTESIAN_POINT('Ctrl Pts',(17.0802404735807,14.5876477371939,9.77868679011485));
#28573=CARTESIAN_POINT('Ctrl Pts',(17.0802404735807,15.5000000000002,9.73702012344818));
#28574=CARTESIAN_POINT('Ctrl Pts',(17.0802404735807,16.4123522628064,9.69535345678151));
#28575=CARTESIAN_POINT('Ctrl Pts',(16.2901202367902,16.8685283942095,9.65368679011485));
#28576=CARTESIAN_POINT('Ctrl Pts',(15.4999999999998,17.3247045256126,9.61202012344818));
#28577=CARTESIAN_POINT('Ctrl Pts',(14.7098797632094,16.8685283942095,9.57035345678151));
#28578=CARTESIAN_POINT('Ctrl Pts',(13.919759526419,16.4123522628064,9.52868679011484));
#28579=CARTESIAN_POINT('Ctrl Pts',(13.919759526419,15.5000000000001,9.48702012344818));
#28580=CARTESIAN_POINT('Ctrl Pts',(13.919759526419,14.5876477371939,9.44535345678151));
#28581=CARTESIAN_POINT('Ctrl Pts',(14.7098797632094,14.1314716057908,9.40368679011484));
#28582=CARTESIAN_POINT('Ctrl Pts',(15.4999999999999,13.6752954743877,9.36202012344818));
#28583=CARTESIAN_POINT('Ctrl Pts',(16.2901202367903,14.1314716057908,9.32035345678151));
#28584=CARTESIAN_POINT('Ctrl Pts',(17.0802404735807,14.5876477371939,9.27868679011484));
#28585=CARTESIAN_POINT('Ctrl Pts',(17.0802404735807,15.5000000000002,9.23702012344818));
#28586=CARTESIAN_POINT('Ctrl Pts',(17.0802404735807,16.4123522628064,9.19535345678151));
#28587=CARTESIAN_POINT('Ctrl Pts',(16.2901202367902,16.8685283942095,9.15368679011484));
#28588=CARTESIAN_POINT('Ctrl Pts',(15.4999999999998,17.3247045256126,9.11202012344818));
#28589=CARTESIAN_POINT('Ctrl Pts',(14.7098797632094,16.8685283942095,9.07035345678151));
#28590=CARTESIAN_POINT('Ctrl Pts',(13.919759526419,16.4123522628064,9.02868679011484));
#28591=CARTESIAN_POINT('Ctrl Pts',(13.919759526419,15.5000000000001,8.98702012344817));
#28592=CARTESIAN_POINT('Ctrl Pts',(13.919759526419,14.5876477371939,8.94535345678151));
#28593=CARTESIAN_POINT('Ctrl Pts',(14.7098797632094,14.1314716057908,8.90368679011484));
#28594=CARTESIAN_POINT('Ctrl Pts',(15.4999999999999,13.6752954743877,8.86202012344817));
#28595=CARTESIAN_POINT('Ctrl Pts',(16.2901202367903,14.1314716057908,8.8203534567815));
#28596=CARTESIAN_POINT('Ctrl Pts',(17.0802404735807,14.5876477371939,8.77868679011484));
#28597=CARTESIAN_POINT('Ctrl Pts',(17.0802404735807,15.5000000000002,8.73702012344817));
#28598=CARTESIAN_POINT('Ctrl Pts',(17.0802404735807,16.4123522628064,8.6953534567815));
#28599=CARTESIAN_POINT('Ctrl Pts',(16.2901202367902,16.8685283942095,8.65368679011483));
#28600=CARTESIAN_POINT('Ctrl Pts',(15.4999999999998,17.3247045256126,8.61202012344817));
#28601=CARTESIAN_POINT('Ctrl Pts',(14.7098797632094,16.8685283942095,8.5703534567815));
#28602=CARTESIAN_POINT('Ctrl Pts',(13.919759526419,16.4123522628064,8.52868679011483));
#28603=CARTESIAN_POINT('Ctrl Pts',(13.919759526419,15.5000000000001,8.48702012344816));
#28604=CARTESIAN_POINT('Ctrl Pts',(13.919759526419,14.5876477371939,8.4453534567815));
#28605=CARTESIAN_POINT('Ctrl Pts',(14.7098797632094,14.1314716057908,8.40368679011483));
#28606=CARTESIAN_POINT('Ctrl Pts',(15.4999999999999,13.6752954743877,8.36202012344816));
#28607=CARTESIAN_POINT('Ctrl Pts',(16.2901202367903,14.1314716057908,8.3203534567815));
#28608=CARTESIAN_POINT('Ctrl Pts',(17.0802404735807,14.5876477371939,8.27868679011483));
#28609=CARTESIAN_POINT('Ctrl Pts',(17.0802404735807,15.5000000000002,8.23702012344816));
#28610=CARTESIAN_POINT('Ctrl Pts',(17.0802404735807,16.4123522628064,8.1953534567815));
#28611=CARTESIAN_POINT('Ctrl Pts',(16.2901202367902,16.8685283942095,8.15368679011483));
#28612=CARTESIAN_POINT('Ctrl Pts',(15.4999999999998,17.3247045256126,8.11202012344816));
#28613=CARTESIAN_POINT('Ctrl Pts',(14.7098797632094,16.8685283942095,8.07035345678149));
#28614=CARTESIAN_POINT('Ctrl Pts',(13.919759526419,16.4123522628064,8.02868679011483));
#28615=CARTESIAN_POINT('Ctrl Pts',(13.919759526419,15.5000000000001,7.98702012344816));
#28616=CARTESIAN_POINT('Ctrl Pts',(13.919759526419,14.5876477371939,7.94535345678149));
#28617=CARTESIAN_POINT('Ctrl Pts',(14.7098797632094,14.1314716057908,7.90368679011482));
#28618=CARTESIAN_POINT('Ctrl Pts',(15.4999999999999,13.6752954743877,7.86202012344816));
#28619=CARTESIAN_POINT('Ctrl Pts',(16.2901202367903,14.1314716057908,7.82035345678149));
#28620=CARTESIAN_POINT('Ctrl Pts',(17.0802404735807,14.5876477371939,7.77868679011482));
#28621=CARTESIAN_POINT('Ctrl Pts',(17.0802404735807,15.5000000000002,7.73702012344816));
#28622=CARTESIAN_POINT('Ctrl Pts',(17.0802404735807,16.4123522628064,7.69535345678149));
#28623=CARTESIAN_POINT('Ctrl Pts',(16.2901202367902,16.8685283942095,7.65368679011482));
#28624=CARTESIAN_POINT('Ctrl Pts',(15.4999999999998,17.3247045256126,7.61202012344815));
#28625=CARTESIAN_POINT('Ctrl Pts',(14.7098797632094,16.8685283942095,7.57035345678149));
#28626=CARTESIAN_POINT('Ctrl Pts',(13.919759526419,16.4123522628064,7.52868679011482));
#28627=CARTESIAN_POINT('Ctrl Pts',(13.919759526419,15.5000000000001,7.48702012344815));
#28628=CARTESIAN_POINT('Ctrl Pts',(13.919759526419,14.5876477371939,7.44535345678148));
#28629=CARTESIAN_POINT('Ctrl Pts',(14.7098797632094,14.1314716057908,7.40368679011482));
#28630=CARTESIAN_POINT('Ctrl Pts',(15.4999999999999,13.6752954743877,7.36202012344815));
#28631=CARTESIAN_POINT('Ctrl Pts',(16.2901202367903,14.1314716057908,7.32035345678148));
#28632=CARTESIAN_POINT('Ctrl Pts',(17.0802404735807,14.5876477371939,7.27868679011482));
#28633=CARTESIAN_POINT('Ctrl Pts',(17.0802404735807,15.5000000000002,7.23702012344815));
#28634=CARTESIAN_POINT('Ctrl Pts',(17.0802404735807,16.4123522628064,7.19535345678148));
#28635=CARTESIAN_POINT('Ctrl Pts',(16.2901202367902,16.8685283942095,7.15368679011481));
#28636=CARTESIAN_POINT('Ctrl Pts',(15.4999999999998,17.3247045256126,7.11202012344815));
#28637=CARTESIAN_POINT('Ctrl Pts',(14.7098797632094,16.8685283942095,7.07035345678148));
#28638=CARTESIAN_POINT('Ctrl Pts',(13.919759526419,16.4123522628064,7.02868679011481));
#28639=CARTESIAN_POINT('Ctrl Pts',(13.919759526419,15.5000000000001,6.98702012344815));
#28640=CARTESIAN_POINT('Ctrl Pts',(13.919759526419,14.5876477371939,6.94535345678148));
#28641=CARTESIAN_POINT('Ctrl Pts',(14.7098797632094,14.1314716057908,6.90368679011481));
#28642=CARTESIAN_POINT('Ctrl Pts',(15.4999999999999,13.6752954743877,6.86202012344814));
#28643=CARTESIAN_POINT('Ctrl Pts',(16.2901202367903,14.1314716057908,6.82035345678148));
#28644=CARTESIAN_POINT('Ctrl Pts',(17.0802404735807,14.5876477371939,6.77868679011481));
#28645=CARTESIAN_POINT('Ctrl Pts',(17.0802404735807,15.5000000000002,6.73702012344814));
#28646=CARTESIAN_POINT('Ctrl Pts',(17.0802404735807,16.4123522628064,6.69535345678147));
#28647=CARTESIAN_POINT('Ctrl Pts',(16.2901202367902,16.8685283942095,6.65368679011481));
#28648=CARTESIAN_POINT('Ctrl Pts',(15.4999999999998,17.3247045256126,6.61202012344814));
#28649=CARTESIAN_POINT('Ctrl Pts',(14.7098797632094,16.8685283942095,6.57035345678147));
#28650=CARTESIAN_POINT('Ctrl Pts',(13.919759526419,16.4123522628064,6.52868679011481));
#28651=CARTESIAN_POINT('Ctrl Pts',(13.919759526419,15.5000000000001,6.48702012344814));
#28652=CARTESIAN_POINT('Ctrl Pts',(13.919759526419,14.5876477371939,6.44535345678147));
#28653=CARTESIAN_POINT('Ctrl Pts',(14.7098797632094,14.1314716057908,6.40368679011481));
#28654=CARTESIAN_POINT('Ctrl Pts',(15.4999999999999,13.6752954743877,6.36202012344814));
#28655=CARTESIAN_POINT('Ctrl Pts',(16.2901202367903,14.1314716057908,6.32035345678147));
#28656=CARTESIAN_POINT('Ctrl Pts',(17.0802404735807,14.5876477371939,6.2786867901148));
#28657=CARTESIAN_POINT('Ctrl Pts',(17.0802404735807,15.5000000000002,6.23702012344813));
#28658=CARTESIAN_POINT('Ctrl Pts',(17.0802404735807,16.4123522628064,6.19535345678147));
#28659=CARTESIAN_POINT('Ctrl Pts',(16.2901202367902,16.8685283942095,6.1536867901148));
#28660=CARTESIAN_POINT('Ctrl Pts',(15.4999999999998,17.3247045256126,6.11202012344813));
#28661=CARTESIAN_POINT('Ctrl Pts',(14.7098797632094,16.8685283942095,6.07035345678146));
#28662=CARTESIAN_POINT('Ctrl Pts',(13.919759526419,16.4123522628064,6.0286867901148));
#28663=CARTESIAN_POINT('Ctrl Pts',(13.919759526419,15.5000000000001,5.98702012344813));
#28664=CARTESIAN_POINT('Ctrl Pts',(13.919759526419,14.5876477371939,5.94535345678146));
#28665=CARTESIAN_POINT('Ctrl Pts',(14.7098797632094,14.1314716057908,5.9036867901148));
#28666=CARTESIAN_POINT('Ctrl Pts',(15.4999999999999,13.6752954743877,5.86202012344813));
#28667=CARTESIAN_POINT('Ctrl Pts',(16.2901202367903,14.1314716057908,5.82035345678146));
#28668=CARTESIAN_POINT('Ctrl Pts',(17.0802404735807,14.5876477371939,5.7786867901148));
#28669=CARTESIAN_POINT('Ctrl Pts',(17.0802404735807,15.5000000000002,5.73702012344813));
#28670=CARTESIAN_POINT('Ctrl Pts',(17.0802404735807,16.4123522628064,5.69535345678146));
#28671=CARTESIAN_POINT('Ctrl Pts',(16.2901202367902,16.8685283942095,5.65368679011479));
#28672=CARTESIAN_POINT('Ctrl Pts',(15.4999999999998,17.3247045256126,5.61202012344813));
#28673=CARTESIAN_POINT('Ctrl Pts',(14.7098797632094,16.8685283942095,5.57035345678146));
#28674=CARTESIAN_POINT('Ctrl Pts',(13.919759526419,16.4123522628064,5.52868679011479));
#28675=CARTESIAN_POINT('Ctrl Pts',(13.919759526419,15.5000000000001,5.48702012344813));
#28676=CARTESIAN_POINT('Ctrl Pts',(13.919759526419,14.5876477371939,5.44535345678146));
#28677=CARTESIAN_POINT('Ctrl Pts',(14.7098797632094,14.1314716057908,5.40368679011479));
#28678=CARTESIAN_POINT('Ctrl Pts',(15.4999999999999,13.6752954743877,5.36202012344812));
#28679=CARTESIAN_POINT('Ctrl Pts',(16.2901202367903,14.1314716057908,5.32035345678146));
#28680=CARTESIAN_POINT('Ctrl Pts',(17.0802404735807,14.5876477371939,5.27868679011479));
#28681=CARTESIAN_POINT('Ctrl Pts',(17.0802404735807,15.5000000000002,5.23702012344812));
#28682=CARTESIAN_POINT('Ctrl Pts',(17.0802404735807,16.4123522628064,5.19535345678145));
#28683=CARTESIAN_POINT('Ctrl Pts',(16.2901202367902,16.8685283942095,5.15368679011479));
#28684=CARTESIAN_POINT('Ctrl Pts',(15.4999999999998,17.3247045256126,5.11202012344812));
#28685=CARTESIAN_POINT('Ctrl Pts',(14.7098797632094,16.8685283942095,5.07035345678145));
#28686=CARTESIAN_POINT('Ctrl Pts',(13.919759526419,16.4123522628064,5.02868679011479));
#28687=CARTESIAN_POINT('Ctrl Pts',(13.919759526419,15.5000000000001,4.98702012344812));
#28688=CARTESIAN_POINT('Ctrl Pts',(13.919759526419,14.5876477371939,4.94535345678145));
#28689=CARTESIAN_POINT('Ctrl Pts',(14.7098797632094,14.1314716057908,4.90368679011478));
#28690=CARTESIAN_POINT('Ctrl Pts',(15.4999999999999,13.6752954743877,4.86202012344812));
#28691=CARTESIAN_POINT('Ctrl Pts',(16.2901202367903,14.1314716057908,4.82035345678145));
#28692=CARTESIAN_POINT('Ctrl Pts',(17.0802404735807,14.5876477371939,4.77868679011478));
#28693=CARTESIAN_POINT('Ctrl Pts',(17.0802404735807,15.5000000000002,4.73702012344812));
#28694=CARTESIAN_POINT('Ctrl Pts',(17.0802404735807,16.4123522628064,4.69535345678145));
#28695=CARTESIAN_POINT('Ctrl Pts',(16.2901202367902,16.8685283942095,4.65368679011478));
#28696=CARTESIAN_POINT('Ctrl Pts',(15.4999999999998,17.3247045256126,4.61202012344811));
#28697=CARTESIAN_POINT('Ctrl Pts',(14.7098797632094,16.8685283942095,4.57035345678145));
#28698=CARTESIAN_POINT('Ctrl Pts',(13.919759526419,16.4123522628064,4.52868679011478));
#28699=CARTESIAN_POINT('Ctrl Pts',(13.919759526419,15.5000000000001,4.48702012344811));
#28700=CARTESIAN_POINT('Ctrl Pts',(13.919759526419,14.5876477371939,4.44535345678144));
#28701=CARTESIAN_POINT('Ctrl Pts',(14.7098797632094,14.1314716057908,4.40368679011478));
#28702=CARTESIAN_POINT('Ctrl Pts',(15.4999999999999,13.6752954743877,4.36202012344811));
#28703=CARTESIAN_POINT('Ctrl Pts',(16.2901202367903,14.1314716057908,4.32035345678144));
#28704=CARTESIAN_POINT('Ctrl Pts',(17.0802404735807,14.5876477371939,4.27868679011477));
#28705=CARTESIAN_POINT('Ctrl Pts',(17.0802404735807,15.5000000000002,4.23702012344811));
#28706=CARTESIAN_POINT('Ctrl Pts',(17.0802404735807,16.4123522628064,4.19535345678144));
#28707=CARTESIAN_POINT('Ctrl Pts',(16.2901202367902,16.8685283942095,4.15368679011477));
#28708=CARTESIAN_POINT('Ctrl Pts',(15.4999999999998,17.3247045256126,4.11202012344811));
#28709=CARTESIAN_POINT('Ctrl Pts',(14.7098797632094,16.8685283942095,4.07035345678144));
#28710=CARTESIAN_POINT('Ctrl Pts',(13.919759526419,16.4123522628064,4.02868679011477));
#28711=CARTESIAN_POINT('Ctrl Pts',(13.919759526419,15.5000000000001,3.9870201234481));
#28712=CARTESIAN_POINT('Ctrl Pts',(13.919759526419,14.5876477371939,3.94535345678144));
#28713=CARTESIAN_POINT('Ctrl Pts',(14.7098797632094,14.1314716057908,3.90368679011477));
#28714=CARTESIAN_POINT('Ctrl Pts',(15.4999999999999,13.6752954743877,3.8620201234481));
#28715=CARTESIAN_POINT('Ctrl Pts',(16.2901202367903,14.1314716057908,3.82035345678144));
#28716=CARTESIAN_POINT('Ctrl Pts',(17.0802404735807,14.5876477371939,3.77868679011477));
#28717=CARTESIAN_POINT('Ctrl Pts',(17.0802404735807,15.5000000000002,3.7370201234481));
#28718=CARTESIAN_POINT('Ctrl Pts',(17.0802404735807,16.4123522628064,3.69535345678143));
#28719=CARTESIAN_POINT('Ctrl Pts',(16.2901202367902,16.8685283942095,3.65368679011477));
#28720=CARTESIAN_POINT('Ctrl Pts',(15.4999999999998,17.3247045256126,3.6120201234481));
#28721=CARTESIAN_POINT('Ctrl Pts',(14.7098797632094,16.8685283942095,3.57035345678143));
#28722=CARTESIAN_POINT('Ctrl Pts',(13.919759526419,16.4123522628064,3.52868679011477));
#28723=CARTESIAN_POINT('Ctrl Pts',(13.919759526419,15.5000000000001,3.4870201234481));
#28724=CARTESIAN_POINT('Ctrl Pts',(13.919759526419,14.5876477371939,3.44535345678143));
#28725=CARTESIAN_POINT('Ctrl Pts',(14.7098797632094,14.1314716057908,3.40368679011476));
#28726=CARTESIAN_POINT('Ctrl Pts',(15.4999999999999,13.6752954743877,3.3620201234481));
#28727=CARTESIAN_POINT('Ctrl Pts',(16.2901202367903,14.1314716057908,3.32035345678143));
#28728=CARTESIAN_POINT('Ctrl Pts',(17.0802404735807,14.5876477371939,3.27868679011476));
#28729=CARTESIAN_POINT('Ctrl Pts',(17.0802404735807,15.5000000000002,3.2370201234481));
#28730=CARTESIAN_POINT('Ctrl Pts',(17.0802404735807,16.4123522628064,3.19535345678143));
#28731=CARTESIAN_POINT('Ctrl Pts',(16.2901202367902,16.8685283942095,3.15368679011476));
#28732=CARTESIAN_POINT('Ctrl Pts',(15.4999999999998,17.3247045256126,3.11202012344809));
#28733=CARTESIAN_POINT('Ctrl Pts',(14.7098797632094,16.8685283942095,3.07035345678143));
#28734=CARTESIAN_POINT('Ctrl Pts',(13.919759526419,16.4123522628064,3.02868679011476));
#28735=CARTESIAN_POINT('Ctrl Pts',(13.919759526419,15.5000000000001,2.98702012344809));
#28736=CARTESIAN_POINT('Ctrl Pts',(13.919759526419,14.5876477371939,2.94535345678143));
#28737=CARTESIAN_POINT('Ctrl Pts',(14.7098797632094,14.1314716057908,2.90368679011476));
#28738=CARTESIAN_POINT('Ctrl Pts',(15.4999999999999,13.6752954743877,2.86202012344809));
#28739=CARTESIAN_POINT('Ctrl Pts',(16.2901202367903,14.1314716057908,2.82035345678142));
#28740=CARTESIAN_POINT('Ctrl Pts',(17.0802404735807,14.5876477371939,2.77868679011476));
#28741=CARTESIAN_POINT('Ctrl Pts',(17.0802404735807,15.5000000000002,2.73702012344809));
#28742=CARTESIAN_POINT('Ctrl Pts',(17.0802404735807,16.4123522628064,2.69535345678142));
#28743=CARTESIAN_POINT('Ctrl Pts',(16.2901202367902,16.8685283942095,2.65368679011475));
#28744=CARTESIAN_POINT('Ctrl Pts',(15.4999999999998,17.3247045256126,2.61202012344809));
#28745=CARTESIAN_POINT('Ctrl Pts',(14.7098797632094,16.8685283942095,2.57035345678142));
#28746=CARTESIAN_POINT('Ctrl Pts',(13.919759526419,16.4123522628064,2.52868679011475));
#28747=CARTESIAN_POINT('Ctrl Pts',(13.919759526419,15.5000000000001,2.48702012344808));
#28748=CARTESIAN_POINT('Ctrl Pts',(13.919759526419,14.5876477371939,2.44535345678142));
#28749=CARTESIAN_POINT('Ctrl Pts',(14.7098797632094,14.1314716057908,2.40368679011475));
#28750=CARTESIAN_POINT('Ctrl Pts',(15.4999999999999,13.6752954743877,2.36202012344808));
#28751=CARTESIAN_POINT('Ctrl Pts',(16.2901202367903,14.1314716057908,2.32035345678142));
#28752=CARTESIAN_POINT('Ctrl Pts',(17.0802404735807,14.5876477371939,2.27868679011475));
#28753=CARTESIAN_POINT('Ctrl Pts',(17.0802404735807,15.5000000000002,2.23702012344808));
#28754=CARTESIAN_POINT('Ctrl Pts',(17.0802404735807,16.4123522628064,2.19535345678142));
#28755=CARTESIAN_POINT('Ctrl Pts',(16.2901202367902,16.8685283942095,2.15368679011475));
#28756=CARTESIAN_POINT('Ctrl Pts',(15.4999999999998,17.3247045256126,2.11202012344808));
#28757=CARTESIAN_POINT('Ctrl Pts',(14.7098797632094,16.8685283942095,2.07035345678141));
#28758=CARTESIAN_POINT('Ctrl Pts',(13.919759526419,16.4123522628064,2.02868679011475));
#28759=CARTESIAN_POINT('Ctrl Pts',(13.919759526419,15.5000000000001,1.98702012344808));
#28760=CARTESIAN_POINT('Ctrl Pts',(13.919759526419,14.5876477371939,1.94535345678141));
#28761=CARTESIAN_POINT('Ctrl Pts',(14.7098797632094,14.1314716057908,1.90368679011474));
#28762=CARTESIAN_POINT('Ctrl Pts',(15.4999999999999,13.6752954743877,1.86202012344808));
#28763=CARTESIAN_POINT('Ctrl Pts',(16.2901202367903,14.1314716057908,1.82035345678141));
#28764=CARTESIAN_POINT('Ctrl Pts',(17.0802404735807,14.5876477371939,1.77868679011474));
#28765=CARTESIAN_POINT('Ctrl Pts',(17.0802404735807,15.5000000000002,1.73702012344808));
#28766=CARTESIAN_POINT('Ctrl Pts',(17.0802404735807,16.4123522628064,1.69535345678141));
#28767=CARTESIAN_POINT('Ctrl Pts',(16.2901202367902,16.8685283942095,1.65368679011474));
#28768=CARTESIAN_POINT('Ctrl Pts',(15.4999999999998,17.3247045256126,1.61202012344807));
#28769=CARTESIAN_POINT('Ctrl Pts',(14.7098797632094,16.8685283942095,1.57035345678141));
#28770=CARTESIAN_POINT('Ctrl Pts',(13.919759526419,16.4123522628064,1.52868679011474));
#28771=CARTESIAN_POINT('Ctrl Pts',(13.919759526419,15.5000000000001,1.48702012344807));
#28772=CARTESIAN_POINT('Ctrl Pts',(13.919759526419,14.5876477371939,1.4453534567814));
#28773=CARTESIAN_POINT('Ctrl Pts',(14.7098797632094,14.1314716057908,1.40368679011474));
#28774=CARTESIAN_POINT('Ctrl Pts',(15.4999999999999,13.6752954743877,1.36202012344807));
#28775=CARTESIAN_POINT('Ctrl Pts',(16.2901202367903,14.1314716057908,1.3203534567814));
#28776=CARTESIAN_POINT('Ctrl Pts',(17.0802404735807,14.5876477371939,1.27868679011473));
#28777=CARTESIAN_POINT('Ctrl Pts',(17.0802404735807,15.5000000000002,1.23702012344807));
#28778=CARTESIAN_POINT('Ctrl Pts',(17.0802404735807,16.4123522628064,1.1953534567814));
#28779=CARTESIAN_POINT('Ctrl Pts',(16.2901202367902,16.8685283942095,1.15368679011473));
#28780=CARTESIAN_POINT('Ctrl Pts',(15.4999999999998,17.3247045256126,1.11202012344807));
#28781=CARTESIAN_POINT('Ctrl Pts',(14.7098797632094,16.8685283942095,1.0703534567814));
#28782=CARTESIAN_POINT('Ctrl Pts',(13.919759526419,16.4123522628064,1.02868679011473));
#28783=CARTESIAN_POINT('Ctrl Pts',(13.919759526419,15.5000000000001,0.987020123448066));
#28784=CARTESIAN_POINT('Ctrl Pts',(13.919759526419,14.5876477371939,0.945353456781398));
#28785=CARTESIAN_POINT('Ctrl Pts',(14.7098797632094,14.1314716057908,0.903686790114731));
#28786=CARTESIAN_POINT('Ctrl Pts',(15.4999999999999,13.6752954743877,0.862020123448064));
#28787=CARTESIAN_POINT('Ctrl Pts',(16.2901202367903,14.1314716057908,0.820353456781396));
#28788=CARTESIAN_POINT('Ctrl Pts',(17.0802404735807,14.5876477371939,0.778686790114729));
#28789=CARTESIAN_POINT('Ctrl Pts',(17.0802404735807,15.5000000000002,0.737020123448062));
#28790=CARTESIAN_POINT('Ctrl Pts',(17.0802404735807,16.4123522628064,0.695353456781394));
#28791=CARTESIAN_POINT('Ctrl Pts',(16.2901202367902,16.8685283942095,0.653686790114727));
#28792=CARTESIAN_POINT('Ctrl Pts',(15.4999999999998,17.3247045256126,0.61202012344806));
#28793=CARTESIAN_POINT('Ctrl Pts',(14.7098797632094,16.8685283942095,0.570353456781393));
#28794=CARTESIAN_POINT('Ctrl Pts',(13.919759526419,16.4123522628064,0.528686790114725));
#28795=CARTESIAN_POINT('Ctrl Pts',(13.919759526419,15.5000000000001,0.487020123448058));
#28796=CARTESIAN_POINT('Ctrl Pts',(13.919759526419,14.5876477371939,0.445353456781391));
#28797=CARTESIAN_POINT('Ctrl Pts',(14.7098797632094,14.1314716057908,0.403686790114723));
#28798=CARTESIAN_POINT('Ctrl Pts',(15.4999999999999,13.6752954743877,0.362020123448056));
#28799=CARTESIAN_POINT('Ctrl Pts',(16.2901202367903,14.1314716057908,0.320353456781389));
#28800=CARTESIAN_POINT('Ctrl Pts',(17.0802404735807,14.5876477371939,0.278686790114722));
#28801=CARTESIAN_POINT('Ctrl Pts',(17.0802404735807,15.5000000000002,0.237020123448054));
#28802=CARTESIAN_POINT('Ctrl Pts',(17.0802404735807,16.4123522628064,0.195353456781387));
#28803=CARTESIAN_POINT('Ctrl Pts',(16.2901202367902,16.8685283942095,0.15368679011472));
#28804=CARTESIAN_POINT('Ctrl Pts',(15.4999999999998,17.3247045256126,0.112020123448053));
#28805=CARTESIAN_POINT('Ctrl Pts',(14.7098797632094,16.8685283942095,0.0703534567813852));
#28806=CARTESIAN_POINT('Ctrl Pts',(13.919759526419,16.4123522628064,0.0286867901147179));
#28807=CARTESIAN_POINT('Ctrl Pts',(13.919759526419,15.5000000000001,-0.0129798765519493));
#28808=CARTESIAN_POINT('Ctrl Pts',(13.919759526419,14.5876477371939,-0.0546465432186149));
#28809=CARTESIAN_POINT('Ctrl Pts',(14.7098797632094,14.1314716057908,-0.0963132098852822));
#28810=CARTESIAN_POINT('Ctrl Pts',(15.4999999999999,13.6752954743877,-0.137979876551949));
#28811=CARTESIAN_POINT('Ctrl Pts',(16.2901202367903,14.1314716057908,-0.179646543218617));
#28812=CARTESIAN_POINT('Ctrl Pts',(17.0802404735807,14.5876477371939,-0.221313209885284));
#28813=CARTESIAN_POINT('Ctrl Pts',(17.0802404735807,15.5000000000002,-0.262979876551951));
#28814=CARTESIAN_POINT('Ctrl Pts',(17.0802404735807,16.4123522628064,-0.304646543218619));
#28815=CARTESIAN_POINT('Ctrl Pts',(16.2901202367902,16.8685283942095,-0.346313209885286));
#28816=CARTESIAN_POINT('Ctrl Pts',(15.4999999999998,17.3247045256126,-0.387979876551953));
#28817=CARTESIAN_POINT('Ctrl Pts',(14.7098797632094,16.8685283942095,-0.429646543218621));
#28818=CARTESIAN_POINT('Ctrl Pts',(13.919759526419,16.4123522628064,-0.471313209885288));
#28819=CARTESIAN_POINT('Ctrl Pts',(13.919759526419,15.5000000000001,-0.512979876551955));
#28820=CARTESIAN_POINT('Ctrl Pts',(13.919759526419,14.5876477371939,-0.554646543218622));
#28821=CARTESIAN_POINT('Ctrl Pts',(14.7098797632094,14.1314716057908,-0.59631320988529));
#28822=CARTESIAN_POINT('Ctrl Pts',(15.4999999999999,13.6752954743877,-0.637979876551957));
#28823=CARTESIAN_POINT('Ctrl Pts',(16.2901202367903,14.1314716057908,-0.679646543218624));
#28824=CARTESIAN_POINT('Ctrl Pts',(17.0802404735807,14.5876477371939,-0.721313209885291));
#28825=CARTESIAN_POINT('Ctrl Pts',(17.0802404735807,15.5000000000002,-0.762979876551959));
#28826=CARTESIAN_POINT('Ctrl Pts',(17.0802404735807,16.4123522628064,-0.804646543218626));
#28827=CARTESIAN_POINT('Ctrl Pts',(16.2901202367902,16.8685283942095,-0.846313209885293));
#28828=CARTESIAN_POINT('Ctrl Pts',(15.4999999999998,17.3247045256126,-0.887979876551961));
#28829=CARTESIAN_POINT('Ctrl Pts',(14.7098797632094,16.8685283942095,-0.929646543218628));
#28830=CARTESIAN_POINT('Ctrl Pts',(13.919759526419,16.4123522628064,-0.971313209885295));
#28831=CARTESIAN_POINT('Ctrl Pts',(13.919759526419,15.5000000000001,-1.01297987655196));
#28832=CARTESIAN_POINT('Ctrl Pts',(13.919759526419,14.5876477371939,-1.05464654321863));
#28833=CARTESIAN_POINT('Ctrl Pts',(14.7098797632094,14.1314716057908,-1.0963132098853));
#28834=CARTESIAN_POINT('Ctrl Pts',(15.4999999999999,13.6752954743877,-1.13797987655196));
#28835=CARTESIAN_POINT('Ctrl Pts',(16.2901202367903,14.1314716057908,-1.17964654321863));
#28836=CARTESIAN_POINT('Ctrl Pts',(17.0802404735807,14.5876477371939,-1.2213132098853));
#28837=CARTESIAN_POINT('Ctrl Pts',(17.0802404735807,15.5000000000002,-1.26297987655196));
#28838=CARTESIAN_POINT('Ctrl Pts',(17.0802404735807,16.4123522628064,-1.30464654321863));
#28839=CARTESIAN_POINT('Ctrl Pts',(16.2901202367902,16.8685283942095,-1.3463132098853));
#28840=CARTESIAN_POINT('Ctrl Pts',(15.4999999999998,17.3247045256126,-1.38797987655197));
#28841=CARTESIAN_POINT('Ctrl Pts',(14.7098797632094,16.8685283942095,-1.42964654321863));
#28842=CARTESIAN_POINT('Ctrl Pts',(13.919759526419,16.4123522628064,-1.4713132098853));
#28843=CARTESIAN_POINT('Ctrl Pts',(13.919759526419,15.5000000000001,-1.51297987655197));
#28844=CARTESIAN_POINT('Ctrl Pts',(13.919759526419,14.5876477371939,-1.55464654321864));
#28845=CARTESIAN_POINT('Ctrl Pts',(14.7098797632094,14.1314716057908,-1.5963132098853));
#28846=CARTESIAN_POINT('Ctrl Pts',(15.4999999999999,13.6752954743877,-1.63797987655197));
#28847=CARTESIAN_POINT('Ctrl Pts',(16.2901202367903,14.1314716057908,-1.67964654321864));
#28848=CARTESIAN_POINT('Ctrl Pts',(17.0802404735807,14.5876477371939,-1.7213132098853));
#28849=CARTESIAN_POINT('Ctrl Pts',(17.0802404735807,15.5000000000002,-1.76297987655197));
#28850=CARTESIAN_POINT('Ctrl Pts',(17.0802404735807,16.4123522628064,-1.80464654321864));
#28851=CARTESIAN_POINT('Ctrl Pts',(16.2901202367902,16.8685283942095,-1.84631320988531));
#28852=CARTESIAN_POINT('Ctrl Pts',(15.4999999999998,17.3247045256126,-1.88797987655197));
#28853=CARTESIAN_POINT('Ctrl Pts',(14.7098797632094,16.8685283942095,-1.92964654321864));
#28854=CARTESIAN_POINT('Ctrl Pts',(14.4189900731897,16.7005831533721,-1.94498649173085));
#28855=CARTESIAN_POINT('Ctrl Pts',(14.2215586016754,16.4288420454489,-1.96260250461286));
#28856=CARTESIAN_POINT('Ctrl Pts',(13.4352476007233,15.3465777998747,-2.03276185973389));
#28857=CARTESIAN_POINT('Ctrl Pts',(12.6489365997711,14.2643135543005,-2.10292121485492));
#28858=CARTESIAN_POINT('Ctrl Pts',(17.0802404735807,15.5000000000002,11.1745));
#28859=CARTESIAN_POINT('Ctrl Pts',(17.0802404735807,16.4123522628064,11.1328333333333));
#28860=CARTESIAN_POINT('Ctrl Pts',(16.2901202367902,16.8685283942095,11.0911666666667));
#28861=CARTESIAN_POINT('Ctrl Pts',(15.4999999999998,17.3247045256126,11.0495));
#28862=CARTESIAN_POINT('Ctrl Pts',(14.7098797632094,16.8685283942095,11.0078333333333));
#28863=CARTESIAN_POINT('Ctrl Pts',(13.919759526419,16.4123522628064,10.9661666666667));
#28864=CARTESIAN_POINT('Ctrl Pts',(13.919759526419,15.5000000000001,10.9245));
#28865=CARTESIAN_POINT('Ctrl Pts',(13.919759526419,14.5876477371939,10.8828333333333));
#28866=CARTESIAN_POINT('Ctrl Pts',(14.7098797632094,14.1314716057908,10.8411666666667));
#28867=CARTESIAN_POINT('Ctrl Pts',(15.4999999999999,13.6752954743877,10.7995));
#28868=CARTESIAN_POINT('Ctrl Pts',(16.2901202367903,14.1314716057908,10.7578333333333));
#28869=CARTESIAN_POINT('Ctrl Pts',(17.0802404735807,14.5876477371939,10.7161666666667));
#28870=CARTESIAN_POINT('Ctrl Pts',(17.0802404735807,15.5000000000002,10.6745));
#28871=CARTESIAN_POINT('Ctrl Pts',(17.0802404735807,16.4123522628064,10.6328333333333));
#28872=CARTESIAN_POINT('Ctrl Pts',(16.2901202367902,16.8685283942095,10.5911666666667));
#28873=CARTESIAN_POINT('Ctrl Pts',(15.4999999999998,17.3247045256126,10.5495));
#28874=CARTESIAN_POINT('Ctrl Pts',(14.7098797632094,16.8685283942095,10.5078333333333));
#28875=CARTESIAN_POINT('Ctrl Pts',(13.919759526419,16.4123522628064,10.4661666666667));
#28876=CARTESIAN_POINT('Ctrl Pts',(13.919759526419,15.5000000000001,10.4245));
#28877=CARTESIAN_POINT('Ctrl Pts',(13.919759526419,14.5876477371939,10.3828333333333));
#28878=CARTESIAN_POINT('Ctrl Pts',(14.7098797632094,14.1314716057908,10.3411666666667));
#28879=CARTESIAN_POINT('Ctrl Pts',(15.4999999999999,13.6752954743877,10.2995));
#28880=CARTESIAN_POINT('Ctrl Pts',(16.2901202367903,14.1314716057908,10.2578333333333));
#28881=CARTESIAN_POINT('Ctrl Pts',(17.0802404735807,14.5876477371939,10.2161666666667));
#28882=CARTESIAN_POINT('Ctrl Pts',(17.0802404735807,15.5000000000002,10.1745));
#28883=CARTESIAN_POINT('Ctrl Pts',(17.0802404735807,16.4123522628064,10.1328333333333));
#28884=CARTESIAN_POINT('Ctrl Pts',(16.2901202367902,16.8685283942095,10.0911666666667));
#28885=CARTESIAN_POINT('Ctrl Pts',(15.4999999999998,17.3247045256126,10.0495));
#28886=CARTESIAN_POINT('Ctrl Pts',(14.7098797632094,16.8685283942095,10.0078333333333));
#28887=CARTESIAN_POINT('Ctrl Pts',(13.919759526419,16.4123522628064,9.96616666666665));
#28888=CARTESIAN_POINT('Ctrl Pts',(13.919759526419,15.5000000000001,9.92449999999998));
#28889=CARTESIAN_POINT('Ctrl Pts',(13.919759526419,14.5876477371939,9.88283333333331));
#28890=CARTESIAN_POINT('Ctrl Pts',(14.7098797632094,14.1314716057908,9.84116666666665));
#28891=CARTESIAN_POINT('Ctrl Pts',(15.4999999999999,13.6752954743877,9.79949999999998));
#28892=CARTESIAN_POINT('Ctrl Pts',(16.2901202367903,14.1314716057908,9.75783333333331));
#28893=CARTESIAN_POINT('Ctrl Pts',(17.0802404735807,14.5876477371939,9.71616666666665));
#28894=CARTESIAN_POINT('Ctrl Pts',(17.0802404735807,15.5000000000002,9.67449999999998));
#28895=CARTESIAN_POINT('Ctrl Pts',(17.0802404735807,16.4123522628064,9.63283333333331));
#28896=CARTESIAN_POINT('Ctrl Pts',(16.2901202367902,16.8685283942095,9.59116666666664));
#28897=CARTESIAN_POINT('Ctrl Pts',(15.4999999999998,17.3247045256126,9.54949999999998));
#28898=CARTESIAN_POINT('Ctrl Pts',(14.7098797632094,16.8685283942095,9.50783333333331));
#28899=CARTESIAN_POINT('Ctrl Pts',(13.919759526419,16.4123522628064,9.46616666666664));
#28900=CARTESIAN_POINT('Ctrl Pts',(13.919759526419,15.5000000000001,9.42449999999998));
#28901=CARTESIAN_POINT('Ctrl Pts',(13.919759526419,14.5876477371939,9.38283333333331));
#28902=CARTESIAN_POINT('Ctrl Pts',(14.7098797632094,14.1314716057908,9.34116666666664));
#28903=CARTESIAN_POINT('Ctrl Pts',(15.4999999999999,13.6752954743877,9.29949999999998));
#28904=CARTESIAN_POINT('Ctrl Pts',(16.2901202367903,14.1314716057908,9.25783333333331));
#28905=CARTESIAN_POINT('Ctrl Pts',(17.0802404735807,14.5876477371939,9.21616666666664));
#28906=CARTESIAN_POINT('Ctrl Pts',(17.0802404735807,15.5000000000002,9.17449999999997));
#28907=CARTESIAN_POINT('Ctrl Pts',(17.0802404735807,16.4123522628064,9.13283333333331));
#28908=CARTESIAN_POINT('Ctrl Pts',(16.2901202367902,16.8685283942095,9.09116666666664));
#28909=CARTESIAN_POINT('Ctrl Pts',(15.4999999999998,17.3247045256126,9.04949999999997));
#28910=CARTESIAN_POINT('Ctrl Pts',(14.7098797632094,16.8685283942095,9.0078333333333));
#28911=CARTESIAN_POINT('Ctrl Pts',(13.919759526419,16.4123522628064,8.96616666666664));
#28912=CARTESIAN_POINT('Ctrl Pts',(13.919759526419,15.5000000000001,8.92449999999997));
#28913=CARTESIAN_POINT('Ctrl Pts',(13.919759526419,14.5876477371939,8.8828333333333));
#28914=CARTESIAN_POINT('Ctrl Pts',(14.7098797632094,14.1314716057908,8.84116666666664));
#28915=CARTESIAN_POINT('Ctrl Pts',(15.4999999999999,13.6752954743877,8.79949999999997));
#28916=CARTESIAN_POINT('Ctrl Pts',(16.2901202367903,14.1314716057908,8.7578333333333));
#28917=CARTESIAN_POINT('Ctrl Pts',(17.0802404735807,14.5876477371939,8.71616666666663));
#28918=CARTESIAN_POINT('Ctrl Pts',(17.0802404735807,15.5000000000002,8.67449999999997));
#28919=CARTESIAN_POINT('Ctrl Pts',(17.0802404735807,16.4123522628064,8.6328333333333));
#28920=CARTESIAN_POINT('Ctrl Pts',(16.2901202367902,16.8685283942095,8.59116666666663));
#28921=CARTESIAN_POINT('Ctrl Pts',(15.4999999999998,17.3247045256126,8.54949999999996));
#28922=CARTESIAN_POINT('Ctrl Pts',(14.7098797632094,16.8685283942095,8.50783333333329));
#28923=CARTESIAN_POINT('Ctrl Pts',(13.919759526419,16.4123522628064,8.46616666666663));
#28924=CARTESIAN_POINT('Ctrl Pts',(13.919759526419,15.5000000000001,8.42449999999996));
#28925=CARTESIAN_POINT('Ctrl Pts',(13.919759526419,14.5876477371939,8.3828333333333));
#28926=CARTESIAN_POINT('Ctrl Pts',(14.7098797632094,14.1314716057908,8.34116666666663));
#28927=CARTESIAN_POINT('Ctrl Pts',(15.4999999999999,13.6752954743877,8.29949999999996));
#28928=CARTESIAN_POINT('Ctrl Pts',(16.2901202367903,14.1314716057908,8.25783333333329));
#28929=CARTESIAN_POINT('Ctrl Pts',(17.0802404735807,14.5876477371939,8.21616666666663));
#28930=CARTESIAN_POINT('Ctrl Pts',(17.0802404735807,15.5000000000002,8.17449999999996));
#28931=CARTESIAN_POINT('Ctrl Pts',(17.0802404735807,16.4123522628064,8.13283333333329));
#28932=CARTESIAN_POINT('Ctrl Pts',(16.2901202367902,16.8685283942095,8.09116666666663));
#28933=CARTESIAN_POINT('Ctrl Pts',(15.4999999999998,17.3247045256126,8.04949999999996));
#28934=CARTESIAN_POINT('Ctrl Pts',(14.7098797632094,16.8685283942095,8.00783333333329));
#28935=CARTESIAN_POINT('Ctrl Pts',(13.919759526419,16.4123522628064,7.96616666666662));
#28936=CARTESIAN_POINT('Ctrl Pts',(13.919759526419,15.5000000000001,7.92449999999996));
#28937=CARTESIAN_POINT('Ctrl Pts',(13.919759526419,14.5876477371939,7.88283333333329));
#28938=CARTESIAN_POINT('Ctrl Pts',(14.7098797632094,14.1314716057908,7.84116666666662));
#28939=CARTESIAN_POINT('Ctrl Pts',(15.4999999999999,13.6752954743877,7.79949999999995));
#28940=CARTESIAN_POINT('Ctrl Pts',(16.2901202367903,14.1314716057908,7.75783333333329));
#28941=CARTESIAN_POINT('Ctrl Pts',(17.0802404735807,14.5876477371939,7.71616666666662));
#28942=CARTESIAN_POINT('Ctrl Pts',(17.0802404735807,15.5000000000002,7.67449999999995));
#28943=CARTESIAN_POINT('Ctrl Pts',(17.0802404735807,16.4123522628064,7.63283333333328));
#28944=CARTESIAN_POINT('Ctrl Pts',(16.2901202367902,16.8685283942095,7.59116666666662));
#28945=CARTESIAN_POINT('Ctrl Pts',(15.4999999999998,17.3247045256126,7.54949999999995));
#28946=CARTESIAN_POINT('Ctrl Pts',(14.7098797632094,16.8685283942095,7.50783333333328));
#28947=CARTESIAN_POINT('Ctrl Pts',(13.919759526419,16.4123522628064,7.46616666666662));
#28948=CARTESIAN_POINT('Ctrl Pts',(13.919759526419,15.5000000000001,7.42449999999995));
#28949=CARTESIAN_POINT('Ctrl Pts',(13.919759526419,14.5876477371939,7.38283333333328));
#28950=CARTESIAN_POINT('Ctrl Pts',(14.7098797632094,14.1314716057908,7.34116666666661));
#28951=CARTESIAN_POINT('Ctrl Pts',(15.4999999999999,13.6752954743877,7.29949999999995));
#28952=CARTESIAN_POINT('Ctrl Pts',(16.2901202367903,14.1314716057908,7.25783333333328));
#28953=CARTESIAN_POINT('Ctrl Pts',(17.0802404735807,14.5876477371939,7.21616666666661));
#28954=CARTESIAN_POINT('Ctrl Pts',(17.0802404735807,15.5000000000002,7.17449999999995));
#28955=CARTESIAN_POINT('Ctrl Pts',(17.0802404735807,16.4123522628064,7.13283333333328));
#28956=CARTESIAN_POINT('Ctrl Pts',(16.2901202367902,16.8685283942095,7.09116666666661));
#28957=CARTESIAN_POINT('Ctrl Pts',(15.4999999999998,17.3247045256126,7.04949999999994));
#28958=CARTESIAN_POINT('Ctrl Pts',(14.7098797632094,16.8685283942095,7.00783333333328));
#28959=CARTESIAN_POINT('Ctrl Pts',(13.919759526419,16.4123522628064,6.96616666666661));
#28960=CARTESIAN_POINT('Ctrl Pts',(13.919759526419,15.5000000000001,6.92449999999994));
#28961=CARTESIAN_POINT('Ctrl Pts',(13.919759526419,14.5876477371939,6.88283333333327));
#28962=CARTESIAN_POINT('Ctrl Pts',(14.7098797632094,14.1314716057908,6.84116666666661));
#28963=CARTESIAN_POINT('Ctrl Pts',(15.4999999999999,13.6752954743877,6.79949999999994));
#28964=CARTESIAN_POINT('Ctrl Pts',(16.2901202367903,14.1314716057908,6.75783333333327));
#28965=CARTESIAN_POINT('Ctrl Pts',(17.0802404735807,14.5876477371939,6.71616666666661));
#28966=CARTESIAN_POINT('Ctrl Pts',(17.0802404735807,15.5000000000002,6.67449999999994));
#28967=CARTESIAN_POINT('Ctrl Pts',(17.0802404735807,16.4123522628064,6.63283333333327));
#28968=CARTESIAN_POINT('Ctrl Pts',(16.2901202367902,16.8685283942095,6.59116666666661));
#28969=CARTESIAN_POINT('Ctrl Pts',(15.4999999999998,17.3247045256126,6.54949999999994));
#28970=CARTESIAN_POINT('Ctrl Pts',(14.7098797632094,16.8685283942095,6.50783333333327));
#28971=CARTESIAN_POINT('Ctrl Pts',(13.919759526419,16.4123522628064,6.4661666666666));
#28972=CARTESIAN_POINT('Ctrl Pts',(13.919759526419,15.5000000000001,6.42449999999994));
#28973=CARTESIAN_POINT('Ctrl Pts',(13.919759526419,14.5876477371939,6.38283333333327));
#28974=CARTESIAN_POINT('Ctrl Pts',(14.7098797632094,14.1314716057908,6.3411666666666));
#28975=CARTESIAN_POINT('Ctrl Pts',(15.4999999999999,13.6752954743877,6.29949999999993));
#28976=CARTESIAN_POINT('Ctrl Pts',(16.2901202367903,14.1314716057908,6.25783333333327));
#28977=CARTESIAN_POINT('Ctrl Pts',(17.0802404735807,14.5876477371939,6.2161666666666));
#28978=CARTESIAN_POINT('Ctrl Pts',(17.0802404735807,15.5000000000002,6.17449999999993));
#28979=CARTESIAN_POINT('Ctrl Pts',(17.0802404735807,16.4123522628064,6.13283333333326));
#28980=CARTESIAN_POINT('Ctrl Pts',(16.2901202367902,16.8685283942095,6.0911666666666));
#28981=CARTESIAN_POINT('Ctrl Pts',(15.4999999999998,17.3247045256126,6.04949999999993));
#28982=CARTESIAN_POINT('Ctrl Pts',(14.7098797632094,16.8685283942095,6.00783333333326));
#28983=CARTESIAN_POINT('Ctrl Pts',(13.919759526419,16.4123522628064,5.9661666666666));
#28984=CARTESIAN_POINT('Ctrl Pts',(13.919759526419,15.5000000000001,5.92449999999993));
#28985=CARTESIAN_POINT('Ctrl Pts',(13.919759526419,14.5876477371939,5.88283333333326));
#28986=CARTESIAN_POINT('Ctrl Pts',(14.7098797632094,14.1314716057908,5.8411666666666));
#28987=CARTESIAN_POINT('Ctrl Pts',(15.4999999999999,13.6752954743877,5.79949999999993));
#28988=CARTESIAN_POINT('Ctrl Pts',(16.2901202367903,14.1314716057908,5.75783333333326));
#28989=CARTESIAN_POINT('Ctrl Pts',(17.0802404735807,14.5876477371939,5.71616666666659));
#28990=CARTESIAN_POINT('Ctrl Pts',(17.0802404735807,15.5000000000002,5.67449999999993));
#28991=CARTESIAN_POINT('Ctrl Pts',(17.0802404735807,16.4123522628064,5.63283333333326));
#28992=CARTESIAN_POINT('Ctrl Pts',(16.2901202367902,16.8685283942095,5.59116666666659));
#28993=CARTESIAN_POINT('Ctrl Pts',(15.4999999999998,17.3247045256126,5.54949999999992));
#28994=CARTESIAN_POINT('Ctrl Pts',(14.7098797632094,16.8685283942095,5.50783333333326));
#28995=CARTESIAN_POINT('Ctrl Pts',(13.919759526419,16.4123522628064,5.46616666666659));
#28996=CARTESIAN_POINT('Ctrl Pts',(13.919759526419,15.5000000000001,5.42449999999992));
#28997=CARTESIAN_POINT('Ctrl Pts',(13.919759526419,14.5876477371939,5.38283333333326));
#28998=CARTESIAN_POINT('Ctrl Pts',(14.7098797632094,14.1314716057908,5.34116666666659));
#28999=CARTESIAN_POINT('Ctrl Pts',(15.4999999999999,13.6752954743877,5.29949999999992));
#29000=CARTESIAN_POINT('Ctrl Pts',(16.2901202367903,14.1314716057908,5.25783333333325));
#29001=CARTESIAN_POINT('Ctrl Pts',(17.0802404735807,14.5876477371939,5.21616666666659));
#29002=CARTESIAN_POINT('Ctrl Pts',(17.0802404735807,15.5000000000002,5.17449999999992));
#29003=CARTESIAN_POINT('Ctrl Pts',(17.0802404735807,16.4123522628064,5.13283333333325));
#29004=CARTESIAN_POINT('Ctrl Pts',(16.2901202367902,16.8685283942095,5.09116666666658));
#29005=CARTESIAN_POINT('Ctrl Pts',(15.4999999999998,17.3247045256126,5.04949999999992));
#29006=CARTESIAN_POINT('Ctrl Pts',(14.7098797632094,16.8685283942095,5.00783333333325));
#29007=CARTESIAN_POINT('Ctrl Pts',(13.919759526419,16.4123522628064,4.96616666666658));
#29008=CARTESIAN_POINT('Ctrl Pts',(13.919759526419,15.5000000000001,4.92449999999992));
#29009=CARTESIAN_POINT('Ctrl Pts',(13.919759526419,14.5876477371939,4.88283333333325));
#29010=CARTESIAN_POINT('Ctrl Pts',(14.7098797632094,14.1314716057908,4.84116666666658));
#29011=CARTESIAN_POINT('Ctrl Pts',(15.4999999999999,13.6752954743877,4.79949999999991));
#29012=CARTESIAN_POINT('Ctrl Pts',(16.2901202367903,14.1314716057908,4.75783333333325));
#29013=CARTESIAN_POINT('Ctrl Pts',(17.0802404735807,14.5876477371939,4.71616666666658));
#29014=CARTESIAN_POINT('Ctrl Pts',(17.0802404735807,15.5000000000002,4.67449999999991));
#29015=CARTESIAN_POINT('Ctrl Pts',(17.0802404735807,16.4123522628064,4.63283333333324));
#29016=CARTESIAN_POINT('Ctrl Pts',(16.2901202367902,16.8685283942095,4.59116666666658));
#29017=CARTESIAN_POINT('Ctrl Pts',(15.4999999999998,17.3247045256126,4.54949999999991));
#29018=CARTESIAN_POINT('Ctrl Pts',(14.7098797632094,16.8685283942095,4.50783333333324));
#29019=CARTESIAN_POINT('Ctrl Pts',(13.919759526419,16.4123522628064,4.46616666666658));
#29020=CARTESIAN_POINT('Ctrl Pts',(13.919759526419,15.5000000000001,4.42449999999991));
#29021=CARTESIAN_POINT('Ctrl Pts',(13.919759526419,14.5876477371939,4.38283333333324));
#29022=CARTESIAN_POINT('Ctrl Pts',(14.7098797632094,14.1314716057908,4.34116666666657));
#29023=CARTESIAN_POINT('Ctrl Pts',(15.4999999999999,13.6752954743877,4.29949999999991));
#29024=CARTESIAN_POINT('Ctrl Pts',(16.2901202367903,14.1314716057908,4.25783333333324));
#29025=CARTESIAN_POINT('Ctrl Pts',(17.0802404735807,14.5876477371939,4.21616666666657));
#29026=CARTESIAN_POINT('Ctrl Pts',(17.0802404735807,15.5000000000002,4.17449999999991));
#29027=CARTESIAN_POINT('Ctrl Pts',(17.0802404735807,16.4123522628064,4.13283333333324));
#29028=CARTESIAN_POINT('Ctrl Pts',(16.2901202367902,16.8685283942095,4.09116666666657));
#29029=CARTESIAN_POINT('Ctrl Pts',(15.4999999999998,17.3247045256126,4.0494999999999));
#29030=CARTESIAN_POINT('Ctrl Pts',(14.7098797632094,16.8685283942095,4.00783333333324));
#29031=CARTESIAN_POINT('Ctrl Pts',(13.919759526419,16.4123522628064,3.96616666666657));
#29032=CARTESIAN_POINT('Ctrl Pts',(13.919759526419,15.5000000000001,3.9244999999999));
#29033=CARTESIAN_POINT('Ctrl Pts',(13.919759526419,14.5876477371939,3.88283333333323));
#29034=CARTESIAN_POINT('Ctrl Pts',(14.7098797632094,14.1314716057908,3.84116666666657));
#29035=CARTESIAN_POINT('Ctrl Pts',(15.4999999999999,13.6752954743877,3.7994999999999));
#29036=CARTESIAN_POINT('Ctrl Pts',(16.2901202367903,14.1314716057908,3.75783333333323));
#29037=CARTESIAN_POINT('Ctrl Pts',(17.0802404735807,14.5876477371939,3.71616666666657));
#29038=CARTESIAN_POINT('Ctrl Pts',(17.0802404735807,15.5000000000002,3.6744999999999));
#29039=CARTESIAN_POINT('Ctrl Pts',(17.0802404735807,16.4123522628064,3.63283333333323));
#29040=CARTESIAN_POINT('Ctrl Pts',(16.2901202367902,16.8685283942095,3.59116666666656));
#29041=CARTESIAN_POINT('Ctrl Pts',(15.4999999999998,17.3247045256126,3.5494999999999));
#29042=CARTESIAN_POINT('Ctrl Pts',(14.7098797632094,16.8685283942095,3.50783333333323));
#29043=CARTESIAN_POINT('Ctrl Pts',(13.919759526419,16.4123522628064,3.46616666666656));
#29044=CARTESIAN_POINT('Ctrl Pts',(13.919759526419,15.5000000000001,3.4244999999999));
#29045=CARTESIAN_POINT('Ctrl Pts',(13.919759526419,14.5876477371939,3.38283333333323));
#29046=CARTESIAN_POINT('Ctrl Pts',(14.7098797632094,14.1314716057908,3.34116666666656));
#29047=CARTESIAN_POINT('Ctrl Pts',(15.4999999999999,13.6752954743877,3.29949999999989));
#29048=CARTESIAN_POINT('Ctrl Pts',(16.2901202367903,14.1314716057908,3.25783333333323));
#29049=CARTESIAN_POINT('Ctrl Pts',(17.0802404735807,14.5876477371939,3.21616666666656));
#29050=CARTESIAN_POINT('Ctrl Pts',(17.0802404735807,15.5000000000002,3.17449999999989));
#29051=CARTESIAN_POINT('Ctrl Pts',(17.0802404735807,16.4123522628064,3.13283333333323));
#29052=CARTESIAN_POINT('Ctrl Pts',(16.2901202367902,16.8685283942095,3.09116666666656));
#29053=CARTESIAN_POINT('Ctrl Pts',(15.4999999999998,17.3247045256126,3.04949999999989));
#29054=CARTESIAN_POINT('Ctrl Pts',(14.7098797632094,16.8685283942095,3.00783333333322));
#29055=CARTESIAN_POINT('Ctrl Pts',(13.919759526419,16.4123522628064,2.96616666666656));
#29056=CARTESIAN_POINT('Ctrl Pts',(13.919759526419,15.5000000000001,2.92449999999989));
#29057=CARTESIAN_POINT('Ctrl Pts',(13.919759526419,14.5876477371939,2.88283333333322));
#29058=CARTESIAN_POINT('Ctrl Pts',(14.7098797632094,14.1314716057908,2.84116666666655));
#29059=CARTESIAN_POINT('Ctrl Pts',(15.4999999999999,13.6752954743877,2.79949999999989));
#29060=CARTESIAN_POINT('Ctrl Pts',(16.2901202367903,14.1314716057908,2.75783333333322));
#29061=CARTESIAN_POINT('Ctrl Pts',(17.0802404735807,14.5876477371939,2.71616666666655));
#29062=CARTESIAN_POINT('Ctrl Pts',(17.0802404735807,15.5000000000002,2.67449999999989));
#29063=CARTESIAN_POINT('Ctrl Pts',(17.0802404735807,16.4123522628064,2.63283333333322));
#29064=CARTESIAN_POINT('Ctrl Pts',(16.2901202367902,16.8685283942095,2.59116666666655));
#29065=CARTESIAN_POINT('Ctrl Pts',(15.4999999999998,17.3247045256126,2.54949999999988));
#29066=CARTESIAN_POINT('Ctrl Pts',(14.7098797632094,16.8685283942095,2.50783333333322));
#29067=CARTESIAN_POINT('Ctrl Pts',(13.919759526419,16.4123522628064,2.46616666666655));
#29068=CARTESIAN_POINT('Ctrl Pts',(13.919759526419,15.5000000000001,2.42449999999988));
#29069=CARTESIAN_POINT('Ctrl Pts',(13.919759526419,14.5876477371939,2.38283333333321));
#29070=CARTESIAN_POINT('Ctrl Pts',(14.7098797632094,14.1314716057908,2.34116666666655));
#29071=CARTESIAN_POINT('Ctrl Pts',(15.4999999999999,13.6752954743877,2.29949999999988));
#29072=CARTESIAN_POINT('Ctrl Pts',(16.2901202367903,14.1314716057908,2.25783333333321));
#29073=CARTESIAN_POINT('Ctrl Pts',(17.0802404735807,14.5876477371939,2.21616666666655));
#29074=CARTESIAN_POINT('Ctrl Pts',(17.0802404735807,15.5000000000002,2.17449999999988));
#29075=CARTESIAN_POINT('Ctrl Pts',(17.0802404735807,16.4123522628064,2.13283333333321));
#29076=CARTESIAN_POINT('Ctrl Pts',(16.2901202367902,16.8685283942095,2.09116666666655));
#29077=CARTESIAN_POINT('Ctrl Pts',(15.4999999999998,17.3247045256126,2.04949999999988));
#29078=CARTESIAN_POINT('Ctrl Pts',(14.7098797632094,16.8685283942095,2.00783333333321));
#29079=CARTESIAN_POINT('Ctrl Pts',(13.919759526419,16.4123522628064,1.96616666666654));
#29080=CARTESIAN_POINT('Ctrl Pts',(13.919759526419,15.5000000000001,1.92449999999988));
#29081=CARTESIAN_POINT('Ctrl Pts',(13.919759526419,14.5876477371939,1.88283333333321));
#29082=CARTESIAN_POINT('Ctrl Pts',(14.7098797632094,14.1314716057908,1.84116666666654));
#29083=CARTESIAN_POINT('Ctrl Pts',(15.4999999999999,13.6752954743877,1.79949999999987));
#29084=CARTESIAN_POINT('Ctrl Pts',(16.2901202367903,14.1314716057908,1.75783333333321));
#29085=CARTESIAN_POINT('Ctrl Pts',(17.0802404735807,14.5876477371939,1.71616666666654));
#29086=CARTESIAN_POINT('Ctrl Pts',(17.0802404735807,15.5000000000002,1.67449999999987));
#29087=CARTESIAN_POINT('Ctrl Pts',(17.0802404735807,16.4123522628064,1.63283333333321));
#29088=CARTESIAN_POINT('Ctrl Pts',(16.2901202367902,16.8685283942095,1.59116666666654));
#29089=CARTESIAN_POINT('Ctrl Pts',(15.4999999999998,17.3247045256126,1.54949999999987));
#29090=CARTESIAN_POINT('Ctrl Pts',(14.7098797632094,16.8685283942095,1.5078333333332));
#29091=CARTESIAN_POINT('Ctrl Pts',(13.919759526419,16.4123522628064,1.46616666666654));
#29092=CARTESIAN_POINT('Ctrl Pts',(13.919759526419,15.5000000000001,1.42449999999987));
#29093=CARTESIAN_POINT('Ctrl Pts',(13.919759526419,14.5876477371939,1.3828333333332));
#29094=CARTESIAN_POINT('Ctrl Pts',(14.7098797632094,14.1314716057908,1.34116666666653));
#29095=CARTESIAN_POINT('Ctrl Pts',(15.4999999999999,13.6752954743877,1.29949999999987));
#29096=CARTESIAN_POINT('Ctrl Pts',(16.2901202367903,14.1314716057908,1.2578333333332));
#29097=CARTESIAN_POINT('Ctrl Pts',(17.0802404735807,14.5876477371939,1.21616666666653));
#29098=CARTESIAN_POINT('Ctrl Pts',(17.0802404735807,15.5000000000002,1.17449999999986));
#29099=CARTESIAN_POINT('Ctrl Pts',(17.0802404735807,16.4123522628064,1.1328333333332));
#29100=CARTESIAN_POINT('Ctrl Pts',(16.2901202367902,16.8685283942095,1.09116666666653));
#29101=CARTESIAN_POINT('Ctrl Pts',(15.4999999999998,17.3247045256126,1.04949999999986));
#29102=CARTESIAN_POINT('Ctrl Pts',(14.7098797632094,16.8685283942095,1.0078333333332));
#29103=CARTESIAN_POINT('Ctrl Pts',(13.919759526419,16.4123522628064,0.96616666666653));
#29104=CARTESIAN_POINT('Ctrl Pts',(13.919759526419,15.5000000000001,0.924499999999863));
#29105=CARTESIAN_POINT('Ctrl Pts',(13.919759526419,14.5876477371939,0.882833333333196));
#29106=CARTESIAN_POINT('Ctrl Pts',(14.7098797632094,14.1314716057908,0.841166666666529));
#29107=CARTESIAN_POINT('Ctrl Pts',(15.4999999999999,13.6752954743877,0.799499999999861));
#29108=CARTESIAN_POINT('Ctrl Pts',(16.2901202367903,14.1314716057908,0.757833333333194));
#29109=CARTESIAN_POINT('Ctrl Pts',(17.0802404735807,14.5876477371939,0.716166666666527));
#29110=CARTESIAN_POINT('Ctrl Pts',(17.0802404735807,15.5000000000002,0.674499999999859));
#29111=CARTESIAN_POINT('Ctrl Pts',(17.0802404735807,16.4123522628064,0.632833333333192));
#29112=CARTESIAN_POINT('Ctrl Pts',(16.2901202367902,16.8685283942095,0.591166666666525));
#29113=CARTESIAN_POINT('Ctrl Pts',(15.4999999999998,17.3247045256126,0.549499999999857));
#29114=CARTESIAN_POINT('Ctrl Pts',(14.7098797632094,16.8685283942095,0.50783333333319));
#29115=CARTESIAN_POINT('Ctrl Pts',(13.919759526419,16.4123522628064,0.466166666666523));
#29116=CARTESIAN_POINT('Ctrl Pts',(13.919759526419,15.5000000000001,0.424499999999856));
#29117=CARTESIAN_POINT('Ctrl Pts',(13.919759526419,14.5876477371939,0.382833333333188));
#29118=CARTESIAN_POINT('Ctrl Pts',(14.7098797632094,14.1314716057908,0.341166666666521));
#29119=CARTESIAN_POINT('Ctrl Pts',(15.4999999999999,13.6752954743877,0.299499999999854));
#29120=CARTESIAN_POINT('Ctrl Pts',(16.2901202367903,14.1314716057908,0.257833333333186));
#29121=CARTESIAN_POINT('Ctrl Pts',(17.0802404735807,14.5876477371939,0.216166666666519));
#29122=CARTESIAN_POINT('Ctrl Pts',(17.0802404735807,15.5000000000002,0.174499999999852));
#29123=CARTESIAN_POINT('Ctrl Pts',(17.0802404735807,16.4123522628064,0.132833333333185));
#29124=CARTESIAN_POINT('Ctrl Pts',(16.2901202367902,16.8685283942095,0.0911666666665173));
#29125=CARTESIAN_POINT('Ctrl Pts',(15.4999999999998,17.3247045256126,0.04949999999985));
#29126=CARTESIAN_POINT('Ctrl Pts',(14.7098797632094,16.8685283942095,0.00783333333318273));
#29127=CARTESIAN_POINT('Ctrl Pts',(13.919759526419,16.4123522628064,-0.0338333333334846));
#29128=CARTESIAN_POINT('Ctrl Pts',(13.919759526419,15.5000000000001,-0.0755000000001518));
#29129=CARTESIAN_POINT('Ctrl Pts',(13.919759526419,14.5876477371939,-0.117166666666817));
#29130=CARTESIAN_POINT('Ctrl Pts',(14.7098797632094,14.1314716057908,-0.158833333333485));
#29131=CARTESIAN_POINT('Ctrl Pts',(15.4999999999999,13.6752954743877,-0.200500000000152));
#29132=CARTESIAN_POINT('Ctrl Pts',(16.2901202367903,14.1314716057908,-0.242166666666819));
#29133=CARTESIAN_POINT('Ctrl Pts',(17.0802404735807,14.5876477371939,-0.283833333333486));
#29134=CARTESIAN_POINT('Ctrl Pts',(17.0802404735807,15.5000000000002,-0.325500000000154));
#29135=CARTESIAN_POINT('Ctrl Pts',(17.0802404735807,16.4123522628064,-0.367166666666821));
#29136=CARTESIAN_POINT('Ctrl Pts',(16.2901202367902,16.8685283942095,-0.408833333333488));
#29137=CARTESIAN_POINT('Ctrl Pts',(15.4999999999998,17.3247045256126,-0.450500000000156));
#29138=CARTESIAN_POINT('Ctrl Pts',(14.7098797632094,16.8685283942095,-0.492166666666823));
#29139=CARTESIAN_POINT('Ctrl Pts',(13.919759526419,16.4123522628064,-0.53383333333349));
#29140=CARTESIAN_POINT('Ctrl Pts',(13.919759526419,15.5000000000001,-0.575500000000157));
#29141=CARTESIAN_POINT('Ctrl Pts',(13.919759526419,14.5876477371939,-0.617166666666825));
#29142=CARTESIAN_POINT('Ctrl Pts',(14.7098797632094,14.1314716057908,-0.658833333333492));
#29143=CARTESIAN_POINT('Ctrl Pts',(15.4999999999999,13.6752954743877,-0.700500000000159));
#29144=CARTESIAN_POINT('Ctrl Pts',(16.2901202367903,14.1314716057908,-0.742166666666827));
#29145=CARTESIAN_POINT('Ctrl Pts',(17.0802404735807,14.5876477371939,-0.783833333333494));
#29146=CARTESIAN_POINT('Ctrl Pts',(17.0802404735807,15.5000000000002,-0.825500000000161));
#29147=CARTESIAN_POINT('Ctrl Pts',(17.0802404735807,16.4123522628064,-0.867166666666829));
#29148=CARTESIAN_POINT('Ctrl Pts',(16.2901202367902,16.8685283942095,-0.908833333333496));
#29149=CARTESIAN_POINT('Ctrl Pts',(15.4999999999998,17.3247045256126,-0.950500000000163));
#29150=CARTESIAN_POINT('Ctrl Pts',(14.7098797632094,16.8685283942095,-0.99216666666683));
#29151=CARTESIAN_POINT('Ctrl Pts',(13.919759526419,16.4123522628064,-1.0338333333335));
#29152=CARTESIAN_POINT('Ctrl Pts',(13.919759526419,15.5000000000001,-1.07550000000016));
#29153=CARTESIAN_POINT('Ctrl Pts',(13.919759526419,14.5876477371939,-1.11716666666683));
#29154=CARTESIAN_POINT('Ctrl Pts',(14.7098797632094,14.1314716057908,-1.1588333333335));
#29155=CARTESIAN_POINT('Ctrl Pts',(15.4999999999999,13.6752954743877,-1.20050000000017));
#29156=CARTESIAN_POINT('Ctrl Pts',(16.2901202367903,14.1314716057908,-1.24216666666683));
#29157=CARTESIAN_POINT('Ctrl Pts',(17.0802404735807,14.5876477371939,-1.2838333333335));
#29158=CARTESIAN_POINT('Ctrl Pts',(17.0802404735807,15.5000000000002,-1.32550000000017));
#29159=CARTESIAN_POINT('Ctrl Pts',(17.0802404735807,16.4123522628064,-1.36716666666683));
#29160=CARTESIAN_POINT('Ctrl Pts',(16.2901202367902,16.8685283942095,-1.4088333333335));
#29161=CARTESIAN_POINT('Ctrl Pts',(15.4999999999998,17.3247045256126,-1.45050000000017));
#29162=CARTESIAN_POINT('Ctrl Pts',(14.7098797632094,16.8685283942095,-1.49216666666684));
#29163=CARTESIAN_POINT('Ctrl Pts',(13.919759526419,16.4123522628064,-1.5338333333335));
#29164=CARTESIAN_POINT('Ctrl Pts',(13.919759526419,15.5000000000001,-1.57550000000017));
#29165=CARTESIAN_POINT('Ctrl Pts',(13.919759526419,14.5876477371939,-1.61716666666684));
#29166=CARTESIAN_POINT('Ctrl Pts',(14.7098797632094,14.1314716057908,-1.65883333333351));
#29167=CARTESIAN_POINT('Ctrl Pts',(15.4999999999999,13.6752954743877,-1.70050000000017));
#29168=CARTESIAN_POINT('Ctrl Pts',(16.2901202367903,14.1314716057908,-1.74216666666684));
#29169=CARTESIAN_POINT('Ctrl Pts',(17.0802404735807,14.5876477371939,-1.78383333333351));
#29170=CARTESIAN_POINT('Ctrl Pts',(17.0802404735807,15.5000000000002,-1.82550000000017));
#29171=CARTESIAN_POINT('Ctrl Pts',(17.0802404735807,16.4123522628064,-1.86716666666684));
#29172=CARTESIAN_POINT('Ctrl Pts',(16.2901202367902,16.8685283942095,-1.90883333333351));
#29173=CARTESIAN_POINT('Ctrl Pts',(15.4999999999998,17.3247045256126,-1.95050000000018));
#29174=CARTESIAN_POINT('Ctrl Pts',(14.7098797632094,16.8685283942095,-1.99216666666684));
#29175=CARTESIAN_POINT('Ctrl Pts',(14.4189900731897,16.7005831533721,-2.00750661517905));
#29176=CARTESIAN_POINT('Ctrl Pts',(14.2215586016754,16.4288420454489,-2.02512262806106));
#29177=CARTESIAN_POINT('Ctrl Pts',(13.4352476007233,15.3465777998747,-2.09528198318209));
#29178=CARTESIAN_POINT('Ctrl Pts',(12.6489365997711,14.2643135543005,-2.16544133830312));
#29179=CARTESIAN_POINT('Ctrl Pts',(15.5,-17.0802317716412,11.1745050240672));
#29180=CARTESIAN_POINT('Ctrl Pts',(16.4123472387391,-17.0802317716412,11.1328383574005));
#29181=CARTESIAN_POINT('Ctrl Pts',(16.8685208581086,-16.2901158858206,11.0911716907338));
#29182=CARTESIAN_POINT('Ctrl Pts',(17.3246944774781,-15.5,11.0495050240672));
#29183=CARTESIAN_POINT('Ctrl Pts',(16.8685208581086,-14.7098841141794,11.0078383574005));
#29184=CARTESIAN_POINT('Ctrl Pts',(16.4123472387391,-13.9197682283588,10.9661716907338));
#29185=CARTESIAN_POINT('Ctrl Pts',(15.5,-13.9197682283588,10.9245050240672));
#29186=CARTESIAN_POINT('Ctrl Pts',(14.5876527612609,-13.9197682283588,10.8828383574005));
#29187=CARTESIAN_POINT('Ctrl Pts',(14.1314791418914,-14.7098841141794,10.8411716907338));
#29188=CARTESIAN_POINT('Ctrl Pts',(13.6753055225219,-15.5,10.7995050240672));
#29189=CARTESIAN_POINT('Ctrl Pts',(14.1314791418914,-16.2901158858206,10.7578383574005));
#29190=CARTESIAN_POINT('Ctrl Pts',(14.5876527612609,-17.0802317716412,10.7161716907338));
#29191=CARTESIAN_POINT('Ctrl Pts',(15.5,-17.0802317716412,10.6745050240672));
#29192=CARTESIAN_POINT('Ctrl Pts',(16.4123472387391,-17.0802317716412,10.6328383574005));
#29193=CARTESIAN_POINT('Ctrl Pts',(16.8685208581086,-16.2901158858206,10.5911716907338));
#29194=CARTESIAN_POINT('Ctrl Pts',(17.3246944774781,-15.5,10.5495050240672));
#29195=CARTESIAN_POINT('Ctrl Pts',(16.8685208581086,-14.7098841141794,10.5078383574005));
#29196=CARTESIAN_POINT('Ctrl Pts',(16.4123472387391,-13.9197682283588,10.4661716907338));
#29197=CARTESIAN_POINT('Ctrl Pts',(15.5,-13.9197682283588,10.4245050240672));
#29198=CARTESIAN_POINT('Ctrl Pts',(14.5876527612609,-13.9197682283588,10.3828383574005));
#29199=CARTESIAN_POINT('Ctrl Pts',(14.1314791418914,-14.7098841141794,10.3411716907338));
#29200=CARTESIAN_POINT('Ctrl Pts',(13.6753055225219,-15.5,10.2995050240672));
#29201=CARTESIAN_POINT('Ctrl Pts',(14.1314791418914,-16.2901158858206,10.2578383574005));
#29202=CARTESIAN_POINT('Ctrl Pts',(14.5876527612609,-17.0802317716412,10.2161716907338));
#29203=CARTESIAN_POINT('Ctrl Pts',(15.5,-17.0802317716412,10.1745050240672));
#29204=CARTESIAN_POINT('Ctrl Pts',(16.4123472387391,-17.0802317716412,10.1328383574005));
#29205=CARTESIAN_POINT('Ctrl Pts',(16.8685208581086,-16.2901158858206,10.0911716907338));
#29206=CARTESIAN_POINT('Ctrl Pts',(17.3246944774781,-15.5,10.0495050240672));
#29207=CARTESIAN_POINT('Ctrl Pts',(16.8685208581086,-14.7098841141794,10.0078383574005));
#29208=CARTESIAN_POINT('Ctrl Pts',(16.4123472387391,-13.9197682283588,9.96617169073382));
#29209=CARTESIAN_POINT('Ctrl Pts',(15.5,-13.9197682283588,9.92450502406715));
#29210=CARTESIAN_POINT('Ctrl Pts',(14.5876527612609,-13.9197682283588,9.88283835740048));
#29211=CARTESIAN_POINT('Ctrl Pts',(14.1314791418914,-14.7098841141794,9.84117169073382));
#29212=CARTESIAN_POINT('Ctrl Pts',(13.6753055225219,-15.5,9.79950502406715));
#29213=CARTESIAN_POINT('Ctrl Pts',(14.1314791418914,-16.2901158858206,9.75783835740048));
#29214=CARTESIAN_POINT('Ctrl Pts',(14.5876527612609,-17.0802317716412,9.71617169073381));
#29215=CARTESIAN_POINT('Ctrl Pts',(15.5,-17.0802317716412,9.67450502406715));
#29216=CARTESIAN_POINT('Ctrl Pts',(16.4123472387391,-17.0802317716412,9.63283835740048));
#29217=CARTESIAN_POINT('Ctrl Pts',(16.8685208581086,-16.2901158858206,9.59117169073381));
#29218=CARTESIAN_POINT('Ctrl Pts',(17.3246944774781,-15.5,9.54950502406714));
#29219=CARTESIAN_POINT('Ctrl Pts',(16.8685208581086,-14.7098841141794,9.50783835740048));
#29220=CARTESIAN_POINT('Ctrl Pts',(16.4123472387391,-13.9197682283588,9.46617169073381));
#29221=CARTESIAN_POINT('Ctrl Pts',(15.5,-13.9197682283588,9.42450502406714));
#29222=CARTESIAN_POINT('Ctrl Pts',(14.5876527612609,-13.9197682283588,9.38283835740048));
#29223=CARTESIAN_POINT('Ctrl Pts',(14.1314791418914,-14.7098841141794,9.34117169073381));
#29224=CARTESIAN_POINT('Ctrl Pts',(13.6753055225219,-15.5,9.29950502406714));
#29225=CARTESIAN_POINT('Ctrl Pts',(14.1314791418914,-16.2901158858206,9.25783835740048));
#29226=CARTESIAN_POINT('Ctrl Pts',(14.5876527612609,-17.0802317716412,9.21617169073381));
#29227=CARTESIAN_POINT('Ctrl Pts',(15.5,-17.0802317716412,9.17450502406714));
#29228=CARTESIAN_POINT('Ctrl Pts',(16.4123472387391,-17.0802317716412,9.13283835740047));
#29229=CARTESIAN_POINT('Ctrl Pts',(16.8685208581086,-16.2901158858206,9.09117169073381));
#29230=CARTESIAN_POINT('Ctrl Pts',(17.3246944774781,-15.5,9.04950502406714));
#29231=CARTESIAN_POINT('Ctrl Pts',(16.8685208581086,-14.7098841141794,9.00783835740047));
#29232=CARTESIAN_POINT('Ctrl Pts',(16.4123472387391,-13.9197682283588,8.9661716907338));
#29233=CARTESIAN_POINT('Ctrl Pts',(15.5,-13.9197682283588,8.92450502406714));
#29234=CARTESIAN_POINT('Ctrl Pts',(14.5876527612609,-13.9197682283588,8.88283835740047));
#29235=CARTESIAN_POINT('Ctrl Pts',(14.1314791418914,-14.7098841141794,8.8411716907338));
#29236=CARTESIAN_POINT('Ctrl Pts',(13.6753055225219,-15.5,8.79950502406713));
#29237=CARTESIAN_POINT('Ctrl Pts',(14.1314791418914,-16.2901158858206,8.75783835740047));
#29238=CARTESIAN_POINT('Ctrl Pts',(14.5876527612609,-17.0802317716412,8.7161716907338));
#29239=CARTESIAN_POINT('Ctrl Pts',(15.5,-17.0802317716412,8.67450502406713));
#29240=CARTESIAN_POINT('Ctrl Pts',(16.4123472387391,-17.0802317716412,8.63283835740047));
#29241=CARTESIAN_POINT('Ctrl Pts',(16.8685208581086,-16.2901158858206,8.5911716907338));
#29242=CARTESIAN_POINT('Ctrl Pts',(17.3246944774781,-15.5,8.54950502406713));
#29243=CARTESIAN_POINT('Ctrl Pts',(16.8685208581086,-14.7098841141794,8.50783835740046));
#29244=CARTESIAN_POINT('Ctrl Pts',(16.4123472387391,-13.9197682283588,8.4661716907338));
#29245=CARTESIAN_POINT('Ctrl Pts',(15.5,-13.9197682283588,8.42450502406713));
#29246=CARTESIAN_POINT('Ctrl Pts',(14.5876527612609,-13.9197682283588,8.38283835740046));
#29247=CARTESIAN_POINT('Ctrl Pts',(14.1314791418914,-14.7098841141794,8.3411716907338));
#29248=CARTESIAN_POINT('Ctrl Pts',(13.6753055225219,-15.5,8.29950502406713));
#29249=CARTESIAN_POINT('Ctrl Pts',(14.1314791418914,-16.2901158858206,8.25783835740046));
#29250=CARTESIAN_POINT('Ctrl Pts',(14.5876527612609,-17.0802317716412,8.21617169073379));
#29251=CARTESIAN_POINT('Ctrl Pts',(15.5,-17.0802317716412,8.17450502406713));
#29252=CARTESIAN_POINT('Ctrl Pts',(16.4123472387391,-17.0802317716412,8.13283835740046));
#29253=CARTESIAN_POINT('Ctrl Pts',(16.8685208581086,-16.2901158858206,8.09117169073379));
#29254=CARTESIAN_POINT('Ctrl Pts',(17.3246944774781,-15.5,8.04950502406713));
#29255=CARTESIAN_POINT('Ctrl Pts',(16.8685208581086,-14.7098841141794,8.00783835740046));
#29256=CARTESIAN_POINT('Ctrl Pts',(16.4123472387391,-13.9197682283588,7.96617169073379));
#29257=CARTESIAN_POINT('Ctrl Pts',(15.5,-13.9197682283588,7.92450502406712));
#29258=CARTESIAN_POINT('Ctrl Pts',(14.5876527612609,-13.9197682283588,7.88283835740046));
#29259=CARTESIAN_POINT('Ctrl Pts',(14.1314791418914,-14.7098841141794,7.84117169073379));
#29260=CARTESIAN_POINT('Ctrl Pts',(13.6753055225219,-15.5,7.79950502406712));
#29261=CARTESIAN_POINT('Ctrl Pts',(14.1314791418914,-16.2901158858206,7.75783835740046));
#29262=CARTESIAN_POINT('Ctrl Pts',(14.5876527612609,-17.0802317716412,7.71617169073378));
#29263=CARTESIAN_POINT('Ctrl Pts',(15.5,-17.0802317716412,7.67450502406712));
#29264=CARTESIAN_POINT('Ctrl Pts',(16.4123472387391,-17.0802317716412,7.63283835740045));
#29265=CARTESIAN_POINT('Ctrl Pts',(16.8685208581086,-16.2901158858206,7.59117169073379));
#29266=CARTESIAN_POINT('Ctrl Pts',(17.3246944774781,-15.5,7.54950502406712));
#29267=CARTESIAN_POINT('Ctrl Pts',(16.8685208581086,-14.7098841141794,7.50783835740045));
#29268=CARTESIAN_POINT('Ctrl Pts',(16.4123472387391,-13.9197682283588,7.46617169073379));
#29269=CARTESIAN_POINT('Ctrl Pts',(15.5,-13.9197682283588,7.42450502406712));
#29270=CARTESIAN_POINT('Ctrl Pts',(14.5876527612609,-13.9197682283588,7.38283835740045));
#29271=CARTESIAN_POINT('Ctrl Pts',(14.1314791418914,-14.7098841141794,7.34117169073378));
#29272=CARTESIAN_POINT('Ctrl Pts',(13.6753055225219,-15.5,7.29950502406711));
#29273=CARTESIAN_POINT('Ctrl Pts',(14.1314791418914,-16.2901158858206,7.25783835740045));
#29274=CARTESIAN_POINT('Ctrl Pts',(14.5876527612609,-17.0802317716412,7.21617169073378));
#29275=CARTESIAN_POINT('Ctrl Pts',(15.5,-17.0802317716412,7.17450502406711));
#29276=CARTESIAN_POINT('Ctrl Pts',(16.4123472387391,-17.0802317716412,7.13283835740044));
#29277=CARTESIAN_POINT('Ctrl Pts',(16.8685208581086,-16.2901158858206,7.09117169073378));
#29278=CARTESIAN_POINT('Ctrl Pts',(17.3246944774781,-15.5,7.04950502406711));
#29279=CARTESIAN_POINT('Ctrl Pts',(16.8685208581086,-14.7098841141794,7.00783835740045));
#29280=CARTESIAN_POINT('Ctrl Pts',(16.4123472387391,-13.9197682283588,6.96617169073378));
#29281=CARTESIAN_POINT('Ctrl Pts',(15.5,-13.9197682283588,6.92450502406711));
#29282=CARTESIAN_POINT('Ctrl Pts',(14.5876527612609,-13.9197682283588,6.88283835740044));
#29283=CARTESIAN_POINT('Ctrl Pts',(14.1314791418914,-14.7098841141794,6.84117169073378));
#29284=CARTESIAN_POINT('Ctrl Pts',(13.6753055225219,-15.5,6.79950502406711));
#29285=CARTESIAN_POINT('Ctrl Pts',(14.1314791418914,-16.2901158858206,6.75783835740044));
#29286=CARTESIAN_POINT('Ctrl Pts',(14.5876527612609,-17.0802317716412,6.71617169073377));
#29287=CARTESIAN_POINT('Ctrl Pts',(15.5,-17.0802317716412,6.67450502406711));
#29288=CARTESIAN_POINT('Ctrl Pts',(16.4123472387391,-17.0802317716412,6.63283835740044));
#29289=CARTESIAN_POINT('Ctrl Pts',(16.8685208581086,-16.2901158858206,6.59117169073377));
#29290=CARTESIAN_POINT('Ctrl Pts',(17.3246944774781,-15.5,6.54950502406711));
#29291=CARTESIAN_POINT('Ctrl Pts',(16.8685208581086,-14.7098841141794,6.50783835740044));
#29292=CARTESIAN_POINT('Ctrl Pts',(16.4123472387391,-13.9197682283588,6.46617169073377));
#29293=CARTESIAN_POINT('Ctrl Pts',(15.5,-13.9197682283588,6.4245050240671));
#29294=CARTESIAN_POINT('Ctrl Pts',(14.5876527612609,-13.9197682283588,6.38283835740044));
#29295=CARTESIAN_POINT('Ctrl Pts',(14.1314791418914,-14.7098841141794,6.34117169073377));
#29296=CARTESIAN_POINT('Ctrl Pts',(13.6753055225219,-15.5,6.2995050240671));
#29297=CARTESIAN_POINT('Ctrl Pts',(14.1314791418914,-16.2901158858206,6.25783835740044));
#29298=CARTESIAN_POINT('Ctrl Pts',(14.5876527612609,-17.0802317716412,6.21617169073377));
#29299=CARTESIAN_POINT('Ctrl Pts',(15.5,-17.0802317716412,6.1745050240671));
#29300=CARTESIAN_POINT('Ctrl Pts',(16.4123472387391,-17.0802317716412,6.13283835740043));
#29301=CARTESIAN_POINT('Ctrl Pts',(16.8685208581086,-16.2901158858206,6.09117169073377));
#29302=CARTESIAN_POINT('Ctrl Pts',(17.3246944774781,-15.5,6.0495050240671));
#29303=CARTESIAN_POINT('Ctrl Pts',(16.8685208581086,-14.7098841141794,6.00783835740043));
#29304=CARTESIAN_POINT('Ctrl Pts',(16.4123472387391,-13.9197682283588,5.96617169073376));
#29305=CARTESIAN_POINT('Ctrl Pts',(15.5,-13.9197682283588,5.9245050240671));
#29306=CARTESIAN_POINT('Ctrl Pts',(14.5876527612609,-13.9197682283588,5.88283835740043));
#29307=CARTESIAN_POINT('Ctrl Pts',(14.1314791418914,-14.7098841141794,5.84117169073376));
#29308=CARTESIAN_POINT('Ctrl Pts',(13.6753055225219,-15.5,5.79950502406709));
#29309=CARTESIAN_POINT('Ctrl Pts',(14.1314791418914,-16.2901158858206,5.75783835740043));
#29310=CARTESIAN_POINT('Ctrl Pts',(14.5876527612609,-17.0802317716412,5.71617169073376));
#29311=CARTESIAN_POINT('Ctrl Pts',(15.5,-17.0802317716412,5.67450502406709));
#29312=CARTESIAN_POINT('Ctrl Pts',(16.4123472387391,-17.0802317716412,5.63283835740043));
#29313=CARTESIAN_POINT('Ctrl Pts',(16.8685208581086,-16.2901158858206,5.59117169073376));
#29314=CARTESIAN_POINT('Ctrl Pts',(17.3246944774781,-15.5,5.54950502406709));
#29315=CARTESIAN_POINT('Ctrl Pts',(16.8685208581086,-14.7098841141794,5.50783835740043));
#29316=CARTESIAN_POINT('Ctrl Pts',(16.4123472387391,-13.9197682283588,5.46617169073376));
#29317=CARTESIAN_POINT('Ctrl Pts',(15.5,-13.9197682283588,5.42450502406709));
#29318=CARTESIAN_POINT('Ctrl Pts',(14.5876527612609,-13.9197682283588,5.38283835740042));
#29319=CARTESIAN_POINT('Ctrl Pts',(14.1314791418914,-14.7098841141794,5.34117169073376));
#29320=CARTESIAN_POINT('Ctrl Pts',(13.6753055225219,-15.5,5.29950502406709));
#29321=CARTESIAN_POINT('Ctrl Pts',(14.1314791418914,-16.2901158858206,5.25783835740042));
#29322=CARTESIAN_POINT('Ctrl Pts',(14.5876527612609,-17.0802317716412,5.21617169073375));
#29323=CARTESIAN_POINT('Ctrl Pts',(15.5,-17.0802317716412,5.17450502406709));
#29324=CARTESIAN_POINT('Ctrl Pts',(16.4123472387391,-17.0802317716412,5.13283835740042));
#29325=CARTESIAN_POINT('Ctrl Pts',(16.8685208581086,-16.2901158858206,5.09117169073375));
#29326=CARTESIAN_POINT('Ctrl Pts',(17.3246944774781,-15.5,5.04950502406708));
#29327=CARTESIAN_POINT('Ctrl Pts',(16.8685208581086,-14.7098841141794,5.00783835740042));
#29328=CARTESIAN_POINT('Ctrl Pts',(16.4123472387391,-13.9197682283588,4.96617169073375));
#29329=CARTESIAN_POINT('Ctrl Pts',(15.5,-13.9197682283588,4.92450502406708));
#29330=CARTESIAN_POINT('Ctrl Pts',(14.5876527612609,-13.9197682283588,4.88283835740042));
#29331=CARTESIAN_POINT('Ctrl Pts',(14.1314791418914,-14.7098841141794,4.84117169073375));
#29332=CARTESIAN_POINT('Ctrl Pts',(13.6753055225219,-15.5,4.79950502406708));
#29333=CARTESIAN_POINT('Ctrl Pts',(14.1314791418914,-16.2901158858206,4.75783835740041));
#29334=CARTESIAN_POINT('Ctrl Pts',(14.5876527612609,-17.0802317716412,4.71617169073375));
#29335=CARTESIAN_POINT('Ctrl Pts',(15.5,-17.0802317716412,4.67450502406708));
#29336=CARTESIAN_POINT('Ctrl Pts',(16.4123472387391,-17.0802317716412,4.63283835740041));
#29337=CARTESIAN_POINT('Ctrl Pts',(16.8685208581086,-16.2901158858206,4.59117169073375));
#29338=CARTESIAN_POINT('Ctrl Pts',(17.3246944774781,-15.5,4.54950502406708));
#29339=CARTESIAN_POINT('Ctrl Pts',(16.8685208581086,-14.7098841141794,4.50783835740041));
#29340=CARTESIAN_POINT('Ctrl Pts',(16.4123472387391,-13.9197682283588,4.46617169073374));
#29341=CARTESIAN_POINT('Ctrl Pts',(15.5,-13.9197682283588,4.42450502406708));
#29342=CARTESIAN_POINT('Ctrl Pts',(14.5876527612609,-13.9197682283588,4.38283835740041));
#29343=CARTESIAN_POINT('Ctrl Pts',(14.1314791418914,-14.7098841141794,4.34117169073374));
#29344=CARTESIAN_POINT('Ctrl Pts',(13.6753055225219,-15.5,4.29950502406708));
#29345=CARTESIAN_POINT('Ctrl Pts',(14.1314791418914,-16.2901158858206,4.25783835740041));
#29346=CARTESIAN_POINT('Ctrl Pts',(14.5876527612609,-17.0802317716412,4.21617169073374));
#29347=CARTESIAN_POINT('Ctrl Pts',(15.5,-17.0802317716412,4.17450502406707));
#29348=CARTESIAN_POINT('Ctrl Pts',(16.4123472387391,-17.0802317716412,4.13283835740041));
#29349=CARTESIAN_POINT('Ctrl Pts',(16.8685208581086,-16.2901158858206,4.09117169073374));
#29350=CARTESIAN_POINT('Ctrl Pts',(17.3246944774781,-15.5,4.04950502406707));
#29351=CARTESIAN_POINT('Ctrl Pts',(16.8685208581086,-14.7098841141794,4.0078383574004));
#29352=CARTESIAN_POINT('Ctrl Pts',(16.4123472387391,-13.9197682283588,3.96617169073374));
#29353=CARTESIAN_POINT('Ctrl Pts',(15.5,-13.9197682283588,3.92450502406707));
#29354=CARTESIAN_POINT('Ctrl Pts',(14.5876527612609,-13.9197682283588,3.8828383574004));
#29355=CARTESIAN_POINT('Ctrl Pts',(14.1314791418914,-14.7098841141794,3.84117169073374));
#29356=CARTESIAN_POINT('Ctrl Pts',(13.6753055225219,-15.5,3.79950502406707));
#29357=CARTESIAN_POINT('Ctrl Pts',(14.1314791418914,-16.2901158858206,3.7578383574004));
#29358=CARTESIAN_POINT('Ctrl Pts',(14.5876527612609,-17.0802317716412,3.71617169073373));
#29359=CARTESIAN_POINT('Ctrl Pts',(15.5,-17.0802317716412,3.67450502406707));
#29360=CARTESIAN_POINT('Ctrl Pts',(16.4123472387391,-17.0802317716412,3.6328383574004));
#29361=CARTESIAN_POINT('Ctrl Pts',(16.8685208581086,-16.2901158858206,3.59117169073373));
#29362=CARTESIAN_POINT('Ctrl Pts',(17.3246944774781,-15.5,3.54950502406707));
#29363=CARTESIAN_POINT('Ctrl Pts',(16.8685208581086,-14.7098841141794,3.5078383574004));
#29364=CARTESIAN_POINT('Ctrl Pts',(16.4123472387391,-13.9197682283588,3.46617169073373));
#29365=CARTESIAN_POINT('Ctrl Pts',(15.5,-13.9197682283588,3.42450502406706));
#29366=CARTESIAN_POINT('Ctrl Pts',(14.5876527612609,-13.9197682283588,3.3828383574004));
#29367=CARTESIAN_POINT('Ctrl Pts',(14.1314791418914,-14.7098841141794,3.34117169073373));
#29368=CARTESIAN_POINT('Ctrl Pts',(13.6753055225219,-15.5,3.29950502406706));
#29369=CARTESIAN_POINT('Ctrl Pts',(14.1314791418914,-16.2901158858206,3.2578383574004));
#29370=CARTESIAN_POINT('Ctrl Pts',(14.5876527612609,-17.0802317716412,3.21617169073373));
#29371=CARTESIAN_POINT('Ctrl Pts',(15.5,-17.0802317716412,3.17450502406706));
#29372=CARTESIAN_POINT('Ctrl Pts',(16.4123472387391,-17.0802317716412,3.13283835740039));
#29373=CARTESIAN_POINT('Ctrl Pts',(16.8685208581086,-16.2901158858206,3.09117169073373));
#29374=CARTESIAN_POINT('Ctrl Pts',(17.3246944774781,-15.5,3.04950502406706));
#29375=CARTESIAN_POINT('Ctrl Pts',(16.8685208581086,-14.7098841141794,3.00783835740039));
#29376=CARTESIAN_POINT('Ctrl Pts',(16.4123472387391,-13.9197682283588,2.96617169073372));
#29377=CARTESIAN_POINT('Ctrl Pts',(15.5,-13.9197682283588,2.92450502406706));
#29378=CARTESIAN_POINT('Ctrl Pts',(14.5876527612609,-13.9197682283588,2.88283835740039));
#29379=CARTESIAN_POINT('Ctrl Pts',(14.1314791418914,-14.7098841141794,2.84117169073372));
#29380=CARTESIAN_POINT('Ctrl Pts',(13.6753055225219,-15.5,2.79950502406705));
#29381=CARTESIAN_POINT('Ctrl Pts',(14.1314791418914,-16.2901158858206,2.75783835740039));
#29382=CARTESIAN_POINT('Ctrl Pts',(14.5876527612609,-17.0802317716412,2.71617169073372));
#29383=CARTESIAN_POINT('Ctrl Pts',(15.5,-17.0802317716412,2.67450502406705));
#29384=CARTESIAN_POINT('Ctrl Pts',(16.4123472387391,-17.0802317716412,2.63283835740039));
#29385=CARTESIAN_POINT('Ctrl Pts',(16.8685208581086,-16.2901158858206,2.59117169073372));
#29386=CARTESIAN_POINT('Ctrl Pts',(17.3246944774781,-15.5,2.54950502406705));
#29387=CARTESIAN_POINT('Ctrl Pts',(16.8685208581086,-14.7098841141794,2.50783835740038));
#29388=CARTESIAN_POINT('Ctrl Pts',(16.4123472387391,-13.9197682283588,2.46617169073372));
#29389=CARTESIAN_POINT('Ctrl Pts',(15.5,-13.9197682283588,2.42450502406705));
#29390=CARTESIAN_POINT('Ctrl Pts',(14.5876527612609,-13.9197682283588,2.38283835740038));
#29391=CARTESIAN_POINT('Ctrl Pts',(14.1314791418914,-14.7098841141794,2.34117169073371));
#29392=CARTESIAN_POINT('Ctrl Pts',(13.6753055225219,-15.5,2.29950502406705));
#29393=CARTESIAN_POINT('Ctrl Pts',(14.1314791418914,-16.2901158858206,2.25783835740038));
#29394=CARTESIAN_POINT('Ctrl Pts',(14.5876527612609,-17.0802317716412,2.21617169073371));
#29395=CARTESIAN_POINT('Ctrl Pts',(15.5,-17.0802317716412,2.17450502406705));
#29396=CARTESIAN_POINT('Ctrl Pts',(16.4123472387391,-17.0802317716412,2.13283835740038));
#29397=CARTESIAN_POINT('Ctrl Pts',(16.8685208581086,-16.2901158858206,2.09117169073371));
#29398=CARTESIAN_POINT('Ctrl Pts',(17.3246944774781,-15.5,2.04950502406705));
#29399=CARTESIAN_POINT('Ctrl Pts',(16.8685208581086,-14.7098841141794,2.00783835740038));
#29400=CARTESIAN_POINT('Ctrl Pts',(16.4123472387391,-13.9197682283588,1.96617169073371));
#29401=CARTESIAN_POINT('Ctrl Pts',(15.5,-13.9197682283588,1.92450502406704));
#29402=CARTESIAN_POINT('Ctrl Pts',(14.5876527612609,-13.9197682283588,1.88283835740038));
#29403=CARTESIAN_POINT('Ctrl Pts',(14.1314791418914,-14.7098841141794,1.84117169073371));
#29404=CARTESIAN_POINT('Ctrl Pts',(13.6753055225219,-15.5,1.79950502406704));
#29405=CARTESIAN_POINT('Ctrl Pts',(14.1314791418914,-16.2901158858206,1.75783835740037));
#29406=CARTESIAN_POINT('Ctrl Pts',(14.5876527612609,-17.0802317716412,1.71617169073371));
#29407=CARTESIAN_POINT('Ctrl Pts',(15.5,-17.0802317716412,1.67450502406704));
#29408=CARTESIAN_POINT('Ctrl Pts',(16.4123472387391,-17.0802317716412,1.63283835740037));
#29409=CARTESIAN_POINT('Ctrl Pts',(16.8685208581086,-16.2901158858206,1.59117169073371));
#29410=CARTESIAN_POINT('Ctrl Pts',(17.3246944774781,-15.5,1.54950502406704));
#29411=CARTESIAN_POINT('Ctrl Pts',(16.8685208581086,-14.7098841141794,1.50783835740037));
#29412=CARTESIAN_POINT('Ctrl Pts',(16.4123472387391,-13.9197682283588,1.4661716907337));
#29413=CARTESIAN_POINT('Ctrl Pts',(15.5,-13.9197682283588,1.42450502406704));
#29414=CARTESIAN_POINT('Ctrl Pts',(14.5876527612609,-13.9197682283588,1.38283835740037));
#29415=CARTESIAN_POINT('Ctrl Pts',(14.1314791418914,-14.7098841141794,1.3411716907337));
#29416=CARTESIAN_POINT('Ctrl Pts',(13.6753055225219,-15.5,1.29950502406703));
#29417=CARTESIAN_POINT('Ctrl Pts',(14.1314791418914,-16.2901158858206,1.25783835740037));
#29418=CARTESIAN_POINT('Ctrl Pts',(14.5876527612609,-17.0802317716412,1.2161716907337));
#29419=CARTESIAN_POINT('Ctrl Pts',(15.5,-17.0802317716412,1.17450502406703));
#29420=CARTESIAN_POINT('Ctrl Pts',(16.4123472387391,-17.0802317716412,1.13283835740037));
#29421=CARTESIAN_POINT('Ctrl Pts',(16.8685208581086,-16.2901158858206,1.0911716907337));
#29422=CARTESIAN_POINT('Ctrl Pts',(17.3246944774781,-15.5,1.04950502406703));
#29423=CARTESIAN_POINT('Ctrl Pts',(16.8685208581086,-14.7098841141794,1.00783835740037));
#29424=CARTESIAN_POINT('Ctrl Pts',(16.4123472387391,-13.9197682283588,0.966171690733698));
#29425=CARTESIAN_POINT('Ctrl Pts',(15.5,-13.9197682283588,0.924505024067031));
#29426=CARTESIAN_POINT('Ctrl Pts',(14.5876527612609,-13.9197682283588,0.882838357400363));
#29427=CARTESIAN_POINT('Ctrl Pts',(14.1314791418914,-14.7098841141794,0.841171690733696));
#29428=CARTESIAN_POINT('Ctrl Pts',(13.6753055225219,-15.5,0.799505024067029));
#29429=CARTESIAN_POINT('Ctrl Pts',(14.1314791418914,-16.2901158858206,0.757838357400362));
#29430=CARTESIAN_POINT('Ctrl Pts',(14.5876527612609,-17.0802317716412,0.716171690733694));
#29431=CARTESIAN_POINT('Ctrl Pts',(15.5,-17.0802317716412,0.674505024067027));
#29432=CARTESIAN_POINT('Ctrl Pts',(16.4123472387391,-17.0802317716412,0.632838357400359));
#29433=CARTESIAN_POINT('Ctrl Pts',(16.8685208581086,-16.2901158858206,0.591171690733692));
#29434=CARTESIAN_POINT('Ctrl Pts',(17.3246944774781,-15.5,0.549505024067025));
#29435=CARTESIAN_POINT('Ctrl Pts',(16.8685208581086,-14.7098841141794,0.507838357400358));
#29436=CARTESIAN_POINT('Ctrl Pts',(16.4123472387391,-13.9197682283588,0.46617169073369));
#29437=CARTESIAN_POINT('Ctrl Pts',(15.5,-13.9197682283588,0.424505024067023));
#29438=CARTESIAN_POINT('Ctrl Pts',(14.5876527612609,-13.9197682283588,0.382838357400356));
#29439=CARTESIAN_POINT('Ctrl Pts',(14.1314791418914,-14.7098841141794,0.341171690733689));
#29440=CARTESIAN_POINT('Ctrl Pts',(13.6753055225219,-15.5,0.299505024067021));
#29441=CARTESIAN_POINT('Ctrl Pts',(14.1314791418914,-16.2901158858206,0.257838357400354));
#29442=CARTESIAN_POINT('Ctrl Pts',(14.5876527612609,-17.0802317716412,0.216171690733687));
#29443=CARTESIAN_POINT('Ctrl Pts',(15.5,-17.0802317716412,0.174505024067019));
#29444=CARTESIAN_POINT('Ctrl Pts',(16.4123472387391,-17.0802317716412,0.132838357400352));
#29445=CARTESIAN_POINT('Ctrl Pts',(16.8685208581086,-16.2901158858206,0.0911716907336849));
#29446=CARTESIAN_POINT('Ctrl Pts',(17.3246944774781,-15.5,0.0495050240670176));
#29447=CARTESIAN_POINT('Ctrl Pts',(16.8685208581086,-14.7098841141794,0.00783835740035031));
#29448=CARTESIAN_POINT('Ctrl Pts',(16.4123472387391,-13.9197682283588,-0.033828309266317));
#29449=CARTESIAN_POINT('Ctrl Pts',(15.5,-13.9197682283588,-0.0754949759329843));
#29450=CARTESIAN_POINT('Ctrl Pts',(14.5876527612609,-13.9197682283588,-0.11716164259965));
#29451=CARTESIAN_POINT('Ctrl Pts',(14.1314791418914,-14.7098841141794,-0.158828309266317));
#29452=CARTESIAN_POINT('Ctrl Pts',(13.6753055225219,-15.5,-0.200494975932984));
#29453=CARTESIAN_POINT('Ctrl Pts',(14.1314791418914,-16.2901158858206,-0.242161642599652));
#29454=CARTESIAN_POINT('Ctrl Pts',(14.5876527612609,-17.0802317716412,-0.283828309266319));
#29455=CARTESIAN_POINT('Ctrl Pts',(15.5,-17.0802317716412,-0.325494975932986));
#29456=CARTESIAN_POINT('Ctrl Pts',(16.4123472387391,-17.0802317716412,-0.367161642599654));
#29457=CARTESIAN_POINT('Ctrl Pts',(16.8685208581086,-16.2901158858206,-0.408828309266321));
#29458=CARTESIAN_POINT('Ctrl Pts',(17.3246944774781,-15.5,-0.450494975932988));
#29459=CARTESIAN_POINT('Ctrl Pts',(16.8685208581086,-14.7098841141794,-0.492161642599655));
#29460=CARTESIAN_POINT('Ctrl Pts',(16.4123472387391,-13.9197682283588,-0.533828309266323));
#29461=CARTESIAN_POINT('Ctrl Pts',(15.5,-13.9197682283588,-0.57549497593299));
#29462=CARTESIAN_POINT('Ctrl Pts',(14.5876527612609,-13.9197682283588,-0.617161642599657));
#29463=CARTESIAN_POINT('Ctrl Pts',(14.1314791418914,-14.7098841141794,-0.658828309266325));
#29464=CARTESIAN_POINT('Ctrl Pts',(13.6753055225219,-15.5,-0.700494975932992));
#29465=CARTESIAN_POINT('Ctrl Pts',(14.1314791418914,-16.2901158858206,-0.742161642599659));
#29466=CARTESIAN_POINT('Ctrl Pts',(14.5876527612609,-17.0802317716412,-0.783828309266326));
#29467=CARTESIAN_POINT('Ctrl Pts',(15.5,-17.0802317716412,-0.825494975932993));
#29468=CARTESIAN_POINT('Ctrl Pts',(16.4123472387391,-17.0802317716412,-0.867161642599661));
#29469=CARTESIAN_POINT('Ctrl Pts',(16.8685208581086,-16.2901158858206,-0.908828309266328));
#29470=CARTESIAN_POINT('Ctrl Pts',(17.3246944774781,-15.5,-0.950494975932995));
#29471=CARTESIAN_POINT('Ctrl Pts',(16.8685208581086,-14.7098841141794,-0.992161642599663));
#29472=CARTESIAN_POINT('Ctrl Pts',(16.4123472387391,-13.9197682283588,-1.03382830926633));
#29473=CARTESIAN_POINT('Ctrl Pts',(15.5,-13.9197682283588,-1.075494975933));
#29474=CARTESIAN_POINT('Ctrl Pts',(14.5876527612609,-13.9197682283588,-1.11716164259966));
#29475=CARTESIAN_POINT('Ctrl Pts',(14.1314791418914,-14.7098841141794,-1.15882830926633));
#29476=CARTESIAN_POINT('Ctrl Pts',(13.6753055225219,-15.5,-1.200494975933));
#29477=CARTESIAN_POINT('Ctrl Pts',(14.1314791418914,-16.2901158858206,-1.24216164259967));
#29478=CARTESIAN_POINT('Ctrl Pts',(14.5876527612609,-17.0802317716412,-1.28382830926633));
#29479=CARTESIAN_POINT('Ctrl Pts',(15.5,-17.0802317716412,-1.325494975933));
#29480=CARTESIAN_POINT('Ctrl Pts',(16.4123472387391,-17.0802317716412,-1.36716164259967));
#29481=CARTESIAN_POINT('Ctrl Pts',(16.8685208581086,-16.2901158858206,-1.40882830926633));
#29482=CARTESIAN_POINT('Ctrl Pts',(17.3246944774781,-15.5,-1.450494975933));
#29483=CARTESIAN_POINT('Ctrl Pts',(16.8685208581086,-14.7098841141794,-1.49216164259967));
#29484=CARTESIAN_POINT('Ctrl Pts',(16.4123472387391,-13.9197682283588,-1.53382830926634));
#29485=CARTESIAN_POINT('Ctrl Pts',(15.5,-13.9197682283588,-1.575494975933));
#29486=CARTESIAN_POINT('Ctrl Pts',(14.5876527612609,-13.9197682283588,-1.61716164259967));
#29487=CARTESIAN_POINT('Ctrl Pts',(14.1314791418914,-14.7098841141794,-1.65882830926634));
#29488=CARTESIAN_POINT('Ctrl Pts',(13.6753055225219,-15.5,-1.70049497593301));
#29489=CARTESIAN_POINT('Ctrl Pts',(14.1314791418914,-16.2901158858206,-1.74216164259967));
#29490=CARTESIAN_POINT('Ctrl Pts',(14.5876527612609,-17.0802317716412,-1.78382830926634));
#29491=CARTESIAN_POINT('Ctrl Pts',(15.5,-17.0802317716412,-1.82549497593301));
#29492=CARTESIAN_POINT('Ctrl Pts',(16.4123472387391,-17.0802317716412,-1.86716164259967));
#29493=CARTESIAN_POINT('Ctrl Pts',(16.8685208581086,-16.2901158858206,-1.90882830926634));
#29494=CARTESIAN_POINT('Ctrl Pts',(17.3246944774781,-15.5,-1.95049497593301));
#29495=CARTESIAN_POINT('Ctrl Pts',(16.8685208581086,-14.7098841141794,-1.99216164259968));
#29496=CARTESIAN_POINT('Ctrl Pts',(16.7005726719216,-14.4189893226644,-2.00750194461187));
#29497=CARTESIAN_POINT('Ctrl Pts',(16.4288249477777,-14.2215569357652,-2.02511838079831));
#29498=CARTESIAN_POINT('Ctrl Pts',(15.5,-17.4320632938683,10.971375));
#29499=CARTESIAN_POINT('Ctrl Pts',(16.6154772628062,-17.4320632938683,10.9297083333333));
#29500=CARTESIAN_POINT('Ctrl Pts',(17.1732158942094,-16.4660316469341,10.8880416666667));
#29501=CARTESIAN_POINT('Ctrl Pts',(17.7309545256125,-15.5,10.846375));
#29502=CARTESIAN_POINT('Ctrl Pts',(17.1732158942094,-14.5339683530659,10.8047083333333));
#29503=CARTESIAN_POINT('Ctrl Pts',(16.6154772628062,-13.5679367061317,10.7630416666667));
#29504=CARTESIAN_POINT('Ctrl Pts',(15.5,-13.5679367061317,10.721375));
#29505=CARTESIAN_POINT('Ctrl Pts',(14.3845227371938,-13.5679367061317,10.6797083333333));
#29506=CARTESIAN_POINT('Ctrl Pts',(13.8267841057906,-14.5339683530659,10.6380416666667));
#29507=CARTESIAN_POINT('Ctrl Pts',(13.2690454743875,-15.5,10.596375));
#29508=CARTESIAN_POINT('Ctrl Pts',(13.8267841057906,-16.4660316469341,10.5547083333333));
#29509=CARTESIAN_POINT('Ctrl Pts',(14.3845227371938,-17.4320632938683,10.5130416666667));
#29510=CARTESIAN_POINT('Ctrl Pts',(15.5,-17.4320632938683,10.471375));
#29511=CARTESIAN_POINT('Ctrl Pts',(16.6154772628062,-17.4320632938683,10.4297083333333));
#29512=CARTESIAN_POINT('Ctrl Pts',(17.1732158942094,-16.4660316469341,10.3880416666667));
#29513=CARTESIAN_POINT('Ctrl Pts',(17.7309545256125,-15.5,10.346375));
#29514=CARTESIAN_POINT('Ctrl Pts',(17.1732158942094,-14.5339683530659,10.3047083333333));
#29515=CARTESIAN_POINT('Ctrl Pts',(16.6154772628062,-13.5679367061317,10.2630416666667));
#29516=CARTESIAN_POINT('Ctrl Pts',(15.5,-13.5679367061317,10.221375));
#29517=CARTESIAN_POINT('Ctrl Pts',(14.3845227371938,-13.5679367061317,10.1797083333333));
#29518=CARTESIAN_POINT('Ctrl Pts',(13.8267841057906,-14.5339683530659,10.1380416666667));
#29519=CARTESIAN_POINT('Ctrl Pts',(13.2690454743875,-15.5,10.096375));
#29520=CARTESIAN_POINT('Ctrl Pts',(13.8267841057906,-16.4660316469341,10.0547083333333));
#29521=CARTESIAN_POINT('Ctrl Pts',(14.3845227371938,-17.4320632938683,10.0130416666666));
#29522=CARTESIAN_POINT('Ctrl Pts',(15.5,-17.4320632938683,9.97137499999998));
#29523=CARTESIAN_POINT('Ctrl Pts',(16.6154772628062,-17.4320632938683,9.92970833333332));
#29524=CARTESIAN_POINT('Ctrl Pts',(17.1732158942094,-16.4660316469341,9.88804166666665));
#29525=CARTESIAN_POINT('Ctrl Pts',(17.7309545256125,-15.5,9.84637499999998));
#29526=CARTESIAN_POINT('Ctrl Pts',(17.1732158942094,-14.5339683530659,9.80470833333331));
#29527=CARTESIAN_POINT('Ctrl Pts',(16.6154772628062,-13.5679367061317,9.76304166666665));
#29528=CARTESIAN_POINT('Ctrl Pts',(15.5,-13.5679367061317,9.72137499999998));
#29529=CARTESIAN_POINT('Ctrl Pts',(14.3845227371938,-13.5679367061317,9.67970833333331));
#29530=CARTESIAN_POINT('Ctrl Pts',(13.8267841057906,-14.5339683530659,9.63804166666664));
#29531=CARTESIAN_POINT('Ctrl Pts',(13.2690454743875,-15.5,9.59637499999998));
#29532=CARTESIAN_POINT('Ctrl Pts',(13.8267841057906,-16.4660316469341,9.55470833333331));
#29533=CARTESIAN_POINT('Ctrl Pts',(14.3845227371938,-17.4320632938683,9.51304166666664));
#29534=CARTESIAN_POINT('Ctrl Pts',(15.5,-17.4320632938683,9.47137499999998));
#29535=CARTESIAN_POINT('Ctrl Pts',(16.6154772628062,-17.4320632938683,9.42970833333331));
#29536=CARTESIAN_POINT('Ctrl Pts',(17.1732158942094,-16.4660316469341,9.38804166666664));
#29537=CARTESIAN_POINT('Ctrl Pts',(17.7309545256125,-15.5,9.34637499999997));
#29538=CARTESIAN_POINT('Ctrl Pts',(17.1732158942094,-14.5339683530659,9.30470833333331));
#29539=CARTESIAN_POINT('Ctrl Pts',(16.6154772628062,-13.5679367061317,9.26304166666664));
#29540=CARTESIAN_POINT('Ctrl Pts',(15.5,-13.5679367061317,9.22137499999997));
#29541=CARTESIAN_POINT('Ctrl Pts',(14.3845227371938,-13.5679367061317,9.1797083333333));
#29542=CARTESIAN_POINT('Ctrl Pts',(13.8267841057906,-14.5339683530659,9.13804166666664));
#29543=CARTESIAN_POINT('Ctrl Pts',(13.2690454743875,-15.5,9.09637499999997));
#29544=CARTESIAN_POINT('Ctrl Pts',(13.8267841057906,-16.4660316469341,9.0547083333333));
#29545=CARTESIAN_POINT('Ctrl Pts',(14.3845227371938,-17.4320632938683,9.01304166666664));
#29546=CARTESIAN_POINT('Ctrl Pts',(15.5,-17.4320632938683,8.97137499999997));
#29547=CARTESIAN_POINT('Ctrl Pts',(16.6154772628062,-17.4320632938683,8.9297083333333));
#29548=CARTESIAN_POINT('Ctrl Pts',(17.1732158942094,-16.4660316469341,8.88804166666663));
#29549=CARTESIAN_POINT('Ctrl Pts',(17.7309545256125,-15.5,8.84637499999997));
#29550=CARTESIAN_POINT('Ctrl Pts',(17.1732158942094,-14.5339683530659,8.8047083333333));
#29551=CARTESIAN_POINT('Ctrl Pts',(16.6154772628062,-13.5679367061317,8.76304166666663));
#29552=CARTESIAN_POINT('Ctrl Pts',(15.5,-13.5679367061317,8.72137499999997));
#29553=CARTESIAN_POINT('Ctrl Pts',(14.3845227371938,-13.5679367061317,8.6797083333333));
#29554=CARTESIAN_POINT('Ctrl Pts',(13.8267841057906,-14.5339683530659,8.63804166666663));
#29555=CARTESIAN_POINT('Ctrl Pts',(13.2690454743875,-15.5,8.59637499999996));
#29556=CARTESIAN_POINT('Ctrl Pts',(13.8267841057906,-16.4660316469341,8.5547083333333));
#29557=CARTESIAN_POINT('Ctrl Pts',(14.3845227371938,-17.4320632938683,8.51304166666663));
#29558=CARTESIAN_POINT('Ctrl Pts',(15.5,-17.4320632938683,8.47137499999996));
#29559=CARTESIAN_POINT('Ctrl Pts',(16.6154772628062,-17.4320632938683,8.42970833333329));
#29560=CARTESIAN_POINT('Ctrl Pts',(17.1732158942094,-16.4660316469341,8.38804166666663));
#29561=CARTESIAN_POINT('Ctrl Pts',(17.7309545256125,-15.5,8.34637499999996));
#29562=CARTESIAN_POINT('Ctrl Pts',(17.1732158942094,-14.5339683530659,8.30470833333329));
#29563=CARTESIAN_POINT('Ctrl Pts',(16.6154772628062,-13.5679367061317,8.26304166666663));
#29564=CARTESIAN_POINT('Ctrl Pts',(15.5,-13.5679367061317,8.22137499999996));
#29565=CARTESIAN_POINT('Ctrl Pts',(14.3845227371938,-13.5679367061317,8.17970833333329));
#29566=CARTESIAN_POINT('Ctrl Pts',(13.8267841057906,-14.5339683530659,8.13804166666662));
#29567=CARTESIAN_POINT('Ctrl Pts',(13.2690454743875,-15.5,8.09637499999996));
#29568=CARTESIAN_POINT('Ctrl Pts',(13.8267841057906,-16.4660316469341,8.05470833333329));
#29569=CARTESIAN_POINT('Ctrl Pts',(14.3845227371938,-17.4320632938683,8.01304166666662));
#29570=CARTESIAN_POINT('Ctrl Pts',(15.5,-17.4320632938683,7.97137499999995));
#29571=CARTESIAN_POINT('Ctrl Pts',(16.6154772628062,-17.4320632938683,7.92970833333329));
#29572=CARTESIAN_POINT('Ctrl Pts',(17.1732158942094,-16.4660316469341,7.88804166666662));
#29573=CARTESIAN_POINT('Ctrl Pts',(17.7309545256125,-15.5,7.84637499999995));
#29574=CARTESIAN_POINT('Ctrl Pts',(17.1732158942094,-14.5339683530659,7.80470833333329));
#29575=CARTESIAN_POINT('Ctrl Pts',(16.6154772628062,-13.5679367061317,7.76304166666662));
#29576=CARTESIAN_POINT('Ctrl Pts',(15.5,-13.5679367061317,7.72137499999995));
#29577=CARTESIAN_POINT('Ctrl Pts',(14.3845227371938,-13.5679367061317,7.67970833333329));
#29578=CARTESIAN_POINT('Ctrl Pts',(13.8267841057906,-14.5339683530659,7.63804166666662));
#29579=CARTESIAN_POINT('Ctrl Pts',(13.2690454743875,-15.5,7.59637499999995));
#29580=CARTESIAN_POINT('Ctrl Pts',(13.8267841057906,-16.4660316469341,7.55470833333328));
#29581=CARTESIAN_POINT('Ctrl Pts',(14.3845227371938,-17.4320632938683,7.51304166666662));
#29582=CARTESIAN_POINT('Ctrl Pts',(15.5,-17.4320632938683,7.47137499999995));
#29583=CARTESIAN_POINT('Ctrl Pts',(16.6154772628062,-17.4320632938683,7.42970833333328));
#29584=CARTESIAN_POINT('Ctrl Pts',(17.1732158942094,-16.4660316469341,7.38804166666661));
#29585=CARTESIAN_POINT('Ctrl Pts',(17.7309545256125,-15.5,7.34637499999995));
#29586=CARTESIAN_POINT('Ctrl Pts',(17.1732158942094,-14.5339683530659,7.30470833333328));
#29587=CARTESIAN_POINT('Ctrl Pts',(16.6154772628062,-13.5679367061317,7.26304166666661));
#29588=CARTESIAN_POINT('Ctrl Pts',(15.5,-13.5679367061317,7.22137499999994));
#29589=CARTESIAN_POINT('Ctrl Pts',(14.3845227371938,-13.5679367061317,7.17970833333328));
#29590=CARTESIAN_POINT('Ctrl Pts',(13.8267841057906,-14.5339683530659,7.13804166666661));
#29591=CARTESIAN_POINT('Ctrl Pts',(13.2690454743875,-15.5,7.09637499999995));
#29592=CARTESIAN_POINT('Ctrl Pts',(13.8267841057906,-16.4660316469341,7.05470833333328));
#29593=CARTESIAN_POINT('Ctrl Pts',(14.3845227371938,-17.4320632938683,7.01304166666661));
#29594=CARTESIAN_POINT('Ctrl Pts',(15.5,-17.4320632938683,6.97137499999994));
#29595=CARTESIAN_POINT('Ctrl Pts',(16.6154772628062,-17.4320632938683,6.92970833333328));
#29596=CARTESIAN_POINT('Ctrl Pts',(17.1732158942094,-16.4660316469341,6.88804166666661));
#29597=CARTESIAN_POINT('Ctrl Pts',(17.7309545256125,-15.5,6.84637499999994));
#29598=CARTESIAN_POINT('Ctrl Pts',(17.1732158942094,-14.5339683530659,6.80470833333327));
#29599=CARTESIAN_POINT('Ctrl Pts',(16.6154772628062,-13.5679367061317,6.76304166666661));
#29600=CARTESIAN_POINT('Ctrl Pts',(15.5,-13.5679367061317,6.72137499999994));
#29601=CARTESIAN_POINT('Ctrl Pts',(14.3845227371938,-13.5679367061317,6.67970833333327));
#29602=CARTESIAN_POINT('Ctrl Pts',(13.8267841057906,-14.5339683530659,6.6380416666666));
#29603=CARTESIAN_POINT('Ctrl Pts',(13.2690454743875,-15.5,6.59637499999994));
#29604=CARTESIAN_POINT('Ctrl Pts',(13.8267841057906,-16.4660316469341,6.55470833333327));
#29605=CARTESIAN_POINT('Ctrl Pts',(14.3845227371938,-17.4320632938683,6.5130416666666));
#29606=CARTESIAN_POINT('Ctrl Pts',(15.5,-17.4320632938683,6.47137499999994));
#29607=CARTESIAN_POINT('Ctrl Pts',(16.6154772628062,-17.4320632938683,6.42970833333327));
#29608=CARTESIAN_POINT('Ctrl Pts',(17.1732158942094,-16.4660316469341,6.3880416666666));
#29609=CARTESIAN_POINT('Ctrl Pts',(17.7309545256125,-15.5,6.34637499999993));
#29610=CARTESIAN_POINT('Ctrl Pts',(17.1732158942094,-14.5339683530659,6.30470833333327));
#29611=CARTESIAN_POINT('Ctrl Pts',(16.6154772628062,-13.5679367061317,6.2630416666666));
#29612=CARTESIAN_POINT('Ctrl Pts',(15.5,-13.5679367061317,6.22137499999993));
#29613=CARTESIAN_POINT('Ctrl Pts',(14.3845227371938,-13.5679367061317,6.17970833333327));
#29614=CARTESIAN_POINT('Ctrl Pts',(13.8267841057906,-14.5339683530659,6.1380416666666));
#29615=CARTESIAN_POINT('Ctrl Pts',(13.2690454743875,-15.5,6.09637499999993));
#29616=CARTESIAN_POINT('Ctrl Pts',(13.8267841057906,-16.4660316469341,6.05470833333326));
#29617=CARTESIAN_POINT('Ctrl Pts',(14.3845227371938,-17.4320632938683,6.0130416666666));
#29618=CARTESIAN_POINT('Ctrl Pts',(15.5,-17.4320632938683,5.97137499999993));
#29619=CARTESIAN_POINT('Ctrl Pts',(16.6154772628062,-17.4320632938683,5.92970833333326));
#29620=CARTESIAN_POINT('Ctrl Pts',(17.1732158942094,-16.4660316469341,5.8880416666666));
#29621=CARTESIAN_POINT('Ctrl Pts',(17.7309545256125,-15.5,5.84637499999993));
#29622=CARTESIAN_POINT('Ctrl Pts',(17.1732158942094,-14.5339683530659,5.80470833333326));
#29623=CARTESIAN_POINT('Ctrl Pts',(16.6154772628062,-13.5679367061317,5.76304166666659));
#29624=CARTESIAN_POINT('Ctrl Pts',(15.5,-13.5679367061317,5.72137499999993));
#29625=CARTESIAN_POINT('Ctrl Pts',(14.3845227371938,-13.5679367061317,5.67970833333326));
#29626=CARTESIAN_POINT('Ctrl Pts',(13.8267841057906,-14.5339683530659,5.63804166666659));
#29627=CARTESIAN_POINT('Ctrl Pts',(13.2690454743875,-15.5,5.59637499999992));
#29628=CARTESIAN_POINT('Ctrl Pts',(13.8267841057906,-16.4660316469341,5.55470833333326));
#29629=CARTESIAN_POINT('Ctrl Pts',(14.3845227371938,-17.4320632938683,5.51304166666659));
#29630=CARTESIAN_POINT('Ctrl Pts',(15.5,-17.4320632938683,5.47137499999992));
#29631=CARTESIAN_POINT('Ctrl Pts',(16.6154772628062,-17.4320632938683,5.42970833333325));
#29632=CARTESIAN_POINT('Ctrl Pts',(17.1732158942094,-16.4660316469341,5.38804166666659));
#29633=CARTESIAN_POINT('Ctrl Pts',(17.7309545256125,-15.5,5.34637499999992));
#29634=CARTESIAN_POINT('Ctrl Pts',(17.1732158942094,-14.5339683530659,5.30470833333325));
#29635=CARTESIAN_POINT('Ctrl Pts',(16.6154772628062,-13.5679367061317,5.26304166666659));
#29636=CARTESIAN_POINT('Ctrl Pts',(15.5,-13.5679367061317,5.22137499999992));
#29637=CARTESIAN_POINT('Ctrl Pts',(14.3845227371938,-13.5679367061317,5.17970833333325));
#29638=CARTESIAN_POINT('Ctrl Pts',(13.8267841057906,-14.5339683530659,5.13804166666659));
#29639=CARTESIAN_POINT('Ctrl Pts',(13.2690454743875,-15.5,5.09637499999992));
#29640=CARTESIAN_POINT('Ctrl Pts',(13.8267841057906,-16.4660316469341,5.05470833333325));
#29641=CARTESIAN_POINT('Ctrl Pts',(14.3845227371938,-17.4320632938683,5.01304166666658));
#29642=CARTESIAN_POINT('Ctrl Pts',(15.5,-17.4320632938683,4.97137499999991));
#29643=CARTESIAN_POINT('Ctrl Pts',(16.6154772628062,-17.4320632938683,4.92970833333325));
#29644=CARTESIAN_POINT('Ctrl Pts',(17.1732158942094,-16.4660316469341,4.88804166666658));
#29645=CARTESIAN_POINT('Ctrl Pts',(17.7309545256125,-15.5,4.84637499999991));
#29646=CARTESIAN_POINT('Ctrl Pts',(17.1732158942094,-14.5339683530659,4.80470833333325));
#29647=CARTESIAN_POINT('Ctrl Pts',(16.6154772628062,-13.5679367061317,4.76304166666658));
#29648=CARTESIAN_POINT('Ctrl Pts',(15.5,-13.5679367061317,4.72137499999991));
#29649=CARTESIAN_POINT('Ctrl Pts',(14.3845227371938,-13.5679367061317,4.67970833333325));
#29650=CARTESIAN_POINT('Ctrl Pts',(13.8267841057906,-14.5339683530659,4.63804166666658));
#29651=CARTESIAN_POINT('Ctrl Pts',(13.2690454743875,-15.5,4.59637499999991));
#29652=CARTESIAN_POINT('Ctrl Pts',(13.8267841057906,-16.4660316469341,4.55470833333324));
#29653=CARTESIAN_POINT('Ctrl Pts',(14.3845227371938,-17.4320632938683,4.51304166666658));
#29654=CARTESIAN_POINT('Ctrl Pts',(15.5,-17.4320632938683,4.47137499999991));
#29655=CARTESIAN_POINT('Ctrl Pts',(16.6154772628062,-17.4320632938683,4.42970833333324));
#29656=CARTESIAN_POINT('Ctrl Pts',(17.1732158942094,-16.4660316469341,4.38804166666657));
#29657=CARTESIAN_POINT('Ctrl Pts',(17.7309545256125,-15.5,4.34637499999991));
#29658=CARTESIAN_POINT('Ctrl Pts',(17.1732158942094,-14.5339683530659,4.30470833333324));
#29659=CARTESIAN_POINT('Ctrl Pts',(16.6154772628062,-13.5679367061317,4.26304166666657));
#29660=CARTESIAN_POINT('Ctrl Pts',(15.5,-13.5679367061317,4.22137499999991));
#29661=CARTESIAN_POINT('Ctrl Pts',(14.3845227371938,-13.5679367061317,4.17970833333324));
#29662=CARTESIAN_POINT('Ctrl Pts',(13.8267841057906,-14.5339683530659,4.13804166666657));
#29663=CARTESIAN_POINT('Ctrl Pts',(13.2690454743875,-15.5,4.0963749999999));
#29664=CARTESIAN_POINT('Ctrl Pts',(13.8267841057906,-16.4660316469341,4.05470833333324));
#29665=CARTESIAN_POINT('Ctrl Pts',(14.3845227371938,-17.4320632938683,4.01304166666657));
#29666=CARTESIAN_POINT('Ctrl Pts',(15.5,-17.4320632938683,3.9713749999999));
#29667=CARTESIAN_POINT('Ctrl Pts',(16.6154772628062,-17.4320632938683,3.92970833333323));
#29668=CARTESIAN_POINT('Ctrl Pts',(17.1732158942094,-16.4660316469341,3.88804166666657));
#29669=CARTESIAN_POINT('Ctrl Pts',(17.7309545256125,-15.5,3.8463749999999));
#29670=CARTESIAN_POINT('Ctrl Pts',(17.1732158942094,-14.5339683530659,3.80470833333323));
#29671=CARTESIAN_POINT('Ctrl Pts',(16.6154772628062,-13.5679367061317,3.76304166666656));
#29672=CARTESIAN_POINT('Ctrl Pts',(15.5,-13.5679367061317,3.7213749999999));
#29673=CARTESIAN_POINT('Ctrl Pts',(14.3845227371938,-13.5679367061317,3.67970833333323));
#29674=CARTESIAN_POINT('Ctrl Pts',(13.8267841057906,-14.5339683530659,3.63804166666656));
#29675=CARTESIAN_POINT('Ctrl Pts',(13.2690454743875,-15.5,3.5963749999999));
#29676=CARTESIAN_POINT('Ctrl Pts',(13.8267841057906,-16.4660316469341,3.55470833333323));
#29677=CARTESIAN_POINT('Ctrl Pts',(14.3845227371938,-17.4320632938683,3.51304166666656));
#29678=CARTESIAN_POINT('Ctrl Pts',(15.5,-17.4320632938683,3.4713749999999));
#29679=CARTESIAN_POINT('Ctrl Pts',(16.6154772628062,-17.4320632938683,3.42970833333323));
#29680=CARTESIAN_POINT('Ctrl Pts',(17.1732158942094,-16.4660316469341,3.38804166666656));
#29681=CARTESIAN_POINT('Ctrl Pts',(17.7309545256125,-15.5,3.34637499999989));
#29682=CARTESIAN_POINT('Ctrl Pts',(17.1732158942094,-14.5339683530659,3.30470833333323));
#29683=CARTESIAN_POINT('Ctrl Pts',(16.6154772628062,-13.5679367061317,3.26304166666656));
#29684=CARTESIAN_POINT('Ctrl Pts',(15.5,-13.5679367061317,3.22137499999989));
#29685=CARTESIAN_POINT('Ctrl Pts',(14.3845227371938,-13.5679367061317,3.17970833333322));
#29686=CARTESIAN_POINT('Ctrl Pts',(13.8267841057906,-14.5339683530659,3.13804166666656));
#29687=CARTESIAN_POINT('Ctrl Pts',(13.2690454743875,-15.5,3.09637499999989));
#29688=CARTESIAN_POINT('Ctrl Pts',(13.8267841057906,-16.4660316469341,3.05470833333322));
#29689=CARTESIAN_POINT('Ctrl Pts',(14.3845227371938,-17.4320632938683,3.01304166666656));
#29690=CARTESIAN_POINT('Ctrl Pts',(15.5,-17.4320632938683,2.97137499999989));
#29691=CARTESIAN_POINT('Ctrl Pts',(16.6154772628062,-17.4320632938683,2.92970833333322));
#29692=CARTESIAN_POINT('Ctrl Pts',(17.1732158942094,-16.4660316469341,2.88804166666655));
#29693=CARTESIAN_POINT('Ctrl Pts',(17.7309545256125,-15.5,2.84637499999989));
#29694=CARTESIAN_POINT('Ctrl Pts',(17.1732158942094,-14.5339683530659,2.80470833333322));
#29695=CARTESIAN_POINT('Ctrl Pts',(16.6154772628062,-13.5679367061317,2.76304166666655));
#29696=CARTESIAN_POINT('Ctrl Pts',(15.5,-13.5679367061317,2.72137499999989));
#29697=CARTESIAN_POINT('Ctrl Pts',(14.3845227371938,-13.5679367061317,2.67970833333322));
#29698=CARTESIAN_POINT('Ctrl Pts',(13.8267841057906,-14.5339683530659,2.63804166666655));
#29699=CARTESIAN_POINT('Ctrl Pts',(13.2690454743875,-15.5,2.59637499999988));
#29700=CARTESIAN_POINT('Ctrl Pts',(13.8267841057906,-16.4660316469341,2.55470833333322));
#29701=CARTESIAN_POINT('Ctrl Pts',(14.3845227371938,-17.4320632938683,2.51304166666655));
#29702=CARTESIAN_POINT('Ctrl Pts',(15.5,-17.4320632938683,2.47137499999988));
#29703=CARTESIAN_POINT('Ctrl Pts',(16.6154772628062,-17.4320632938683,2.42970833333321));
#29704=CARTESIAN_POINT('Ctrl Pts',(17.1732158942094,-16.4660316469341,2.38804166666655));
#29705=CARTESIAN_POINT('Ctrl Pts',(17.7309545256125,-15.5,2.34637499999988));
#29706=CARTESIAN_POINT('Ctrl Pts',(17.1732158942094,-14.5339683530659,2.30470833333321));
#29707=CARTESIAN_POINT('Ctrl Pts',(16.6154772628062,-13.5679367061317,2.26304166666655));
#29708=CARTESIAN_POINT('Ctrl Pts',(15.5,-13.5679367061317,2.22137499999988));
#29709=CARTESIAN_POINT('Ctrl Pts',(14.3845227371938,-13.5679367061317,2.17970833333321));
#29710=CARTESIAN_POINT('Ctrl Pts',(13.8267841057906,-14.5339683530659,2.13804166666654));
#29711=CARTESIAN_POINT('Ctrl Pts',(13.2690454743875,-15.5,2.09637499999988));
#29712=CARTESIAN_POINT('Ctrl Pts',(13.8267841057906,-16.4660316469341,2.05470833333321));
#29713=CARTESIAN_POINT('Ctrl Pts',(14.3845227371938,-17.4320632938683,2.01304166666654));
#29714=CARTESIAN_POINT('Ctrl Pts',(15.5,-17.4320632938683,1.97137499999988));
#29715=CARTESIAN_POINT('Ctrl Pts',(16.6154772628062,-17.4320632938683,1.92970833333321));
#29716=CARTESIAN_POINT('Ctrl Pts',(17.1732158942094,-16.4660316469341,1.88804166666654));
#29717=CARTESIAN_POINT('Ctrl Pts',(17.7309545256125,-15.5,1.84637499999987));
#29718=CARTESIAN_POINT('Ctrl Pts',(17.1732158942094,-14.5339683530659,1.80470833333321));
#29719=CARTESIAN_POINT('Ctrl Pts',(16.6154772628062,-13.5679367061317,1.76304166666654));
#29720=CARTESIAN_POINT('Ctrl Pts',(15.5,-13.5679367061317,1.72137499999987));
#29721=CARTESIAN_POINT('Ctrl Pts',(14.3845227371938,-13.5679367061317,1.67970833333321));
#29722=CARTESIAN_POINT('Ctrl Pts',(13.8267841057906,-14.5339683530659,1.63804166666654));
#29723=CARTESIAN_POINT('Ctrl Pts',(13.2690454743875,-15.5,1.59637499999987));
#29724=CARTESIAN_POINT('Ctrl Pts',(13.8267841057906,-16.4660316469341,1.5547083333332));
#29725=CARTESIAN_POINT('Ctrl Pts',(14.3845227371938,-17.4320632938683,1.51304166666654));
#29726=CARTESIAN_POINT('Ctrl Pts',(15.5,-17.4320632938683,1.47137499999987));
#29727=CARTESIAN_POINT('Ctrl Pts',(16.6154772628062,-17.4320632938683,1.4297083333332));
#29728=CARTESIAN_POINT('Ctrl Pts',(17.1732158942094,-16.4660316469341,1.38804166666653));
#29729=CARTESIAN_POINT('Ctrl Pts',(17.7309545256125,-15.5,1.34637499999987));
#29730=CARTESIAN_POINT('Ctrl Pts',(17.1732158942094,-14.5339683530659,1.3047083333332));
#29731=CARTESIAN_POINT('Ctrl Pts',(16.6154772628062,-13.5679367061317,1.26304166666653));
#29732=CARTESIAN_POINT('Ctrl Pts',(15.5,-13.5679367061317,1.22137499999987));
#29733=CARTESIAN_POINT('Ctrl Pts',(14.3845227371938,-13.5679367061317,1.1797083333332));
#29734=CARTESIAN_POINT('Ctrl Pts',(13.8267841057906,-14.5339683530659,1.13804166666653));
#29735=CARTESIAN_POINT('Ctrl Pts',(13.2690454743875,-15.5,1.09637499999986));
#29736=CARTESIAN_POINT('Ctrl Pts',(13.8267841057906,-16.4660316469341,1.0547083333332));
#29737=CARTESIAN_POINT('Ctrl Pts',(14.3845227371938,-17.4320632938683,1.01304166666653));
#29738=CARTESIAN_POINT('Ctrl Pts',(15.5,-17.4320632938683,0.971374999999861));
#29739=CARTESIAN_POINT('Ctrl Pts',(16.6154772628062,-17.4320632938683,0.929708333333194));
#29740=CARTESIAN_POINT('Ctrl Pts',(17.1732158942094,-16.4660316469341,0.888041666666528));
#29741=CARTESIAN_POINT('Ctrl Pts',(17.7309545256125,-15.5,0.846374999999861));
#29742=CARTESIAN_POINT('Ctrl Pts',(17.1732158942094,-14.5339683530659,0.804708333333194));
#29743=CARTESIAN_POINT('Ctrl Pts',(16.6154772628062,-13.5679367061317,0.763041666666526));
#29744=CARTESIAN_POINT('Ctrl Pts',(15.5,-13.5679367061317,0.721374999999859));
#29745=CARTESIAN_POINT('Ctrl Pts',(14.3845227371938,-13.5679367061317,0.679708333333192));
#29746=CARTESIAN_POINT('Ctrl Pts',(13.8267841057906,-14.5339683530659,0.638041666666525));
#29747=CARTESIAN_POINT('Ctrl Pts',(13.2690454743875,-15.5,0.596374999999858));
#29748=CARTESIAN_POINT('Ctrl Pts',(13.8267841057906,-16.4660316469341,0.55470833333319));
#29749=CARTESIAN_POINT('Ctrl Pts',(14.3845227371938,-17.4320632938683,0.513041666666523));
#29750=CARTESIAN_POINT('Ctrl Pts',(15.5,-17.4320632938683,0.471374999999856));
#29751=CARTESIAN_POINT('Ctrl Pts',(16.6154772628062,-17.4320632938683,0.429708333333188));
#29752=CARTESIAN_POINT('Ctrl Pts',(17.1732158942094,-16.4660316469341,0.388041666666521));
#29753=CARTESIAN_POINT('Ctrl Pts',(17.7309545256125,-15.5,0.346374999999854));
#29754=CARTESIAN_POINT('Ctrl Pts',(17.1732158942094,-14.5339683530659,0.304708333333186));
#29755=CARTESIAN_POINT('Ctrl Pts',(16.6154772628062,-13.5679367061317,0.263041666666519));
#29756=CARTESIAN_POINT('Ctrl Pts',(15.5,-13.5679367061317,0.221374999999852));
#29757=CARTESIAN_POINT('Ctrl Pts',(14.3845227371938,-13.5679367061317,0.179708333333185));
#29758=CARTESIAN_POINT('Ctrl Pts',(13.8267841057906,-14.5339683530659,0.138041666666517));
#29759=CARTESIAN_POINT('Ctrl Pts',(13.2690454743875,-15.5,0.0963749999998501));
#29760=CARTESIAN_POINT('Ctrl Pts',(13.8267841057906,-16.4660316469341,0.0547083333331828));
#29761=CARTESIAN_POINT('Ctrl Pts',(14.3845227371938,-17.4320632938683,0.0130416666665155));
#29762=CARTESIAN_POINT('Ctrl Pts',(15.5,-17.4320632938683,-0.0286250000001518));
#29763=CARTESIAN_POINT('Ctrl Pts',(16.6154772628062,-17.4320632938683,-0.0702916666668191));
#29764=CARTESIAN_POINT('Ctrl Pts',(17.1732158942094,-16.4660316469341,-0.111958333333486));
#29765=CARTESIAN_POINT('Ctrl Pts',(17.7309545256125,-15.5,-0.153625000000154));
#29766=CARTESIAN_POINT('Ctrl Pts',(17.1732158942094,-14.5339683530659,-0.195291666666821));
#29767=CARTESIAN_POINT('Ctrl Pts',(16.6154772628062,-13.5679367061317,-0.236958333333488));
#29768=CARTESIAN_POINT('Ctrl Pts',(15.5,-13.5679367061317,-0.278625000000155));
#29769=CARTESIAN_POINT('Ctrl Pts',(14.3845227371938,-13.5679367061317,-0.320291666666821));
#29770=CARTESIAN_POINT('Ctrl Pts',(13.8267841057906,-14.5339683530659,-0.361958333333488));
#29771=CARTESIAN_POINT('Ctrl Pts',(13.2690454743875,-15.5,-0.403625000000156));
#29772=CARTESIAN_POINT('Ctrl Pts',(13.8267841057906,-16.4660316469341,-0.445291666666823));
#29773=CARTESIAN_POINT('Ctrl Pts',(14.3845227371938,-17.4320632938683,-0.48695833333349));
#29774=CARTESIAN_POINT('Ctrl Pts',(15.5,-17.4320632938683,-0.528625000000157));
#29775=CARTESIAN_POINT('Ctrl Pts',(16.6154772628062,-17.4320632938683,-0.570291666666825));
#29776=CARTESIAN_POINT('Ctrl Pts',(17.1732158942094,-16.4660316469341,-0.611958333333492));
#29777=CARTESIAN_POINT('Ctrl Pts',(17.7309545256125,-15.5,-0.653625000000159));
#29778=CARTESIAN_POINT('Ctrl Pts',(17.1732158942094,-14.5339683530659,-0.695291666666827));
#29779=CARTESIAN_POINT('Ctrl Pts',(16.6154772628062,-13.5679367061317,-0.736958333333494));
#29780=CARTESIAN_POINT('Ctrl Pts',(15.5,-13.5679367061317,-0.778625000000161));
#29781=CARTESIAN_POINT('Ctrl Pts',(14.3845227371938,-13.5679367061317,-0.820291666666829));
#29782=CARTESIAN_POINT('Ctrl Pts',(13.8267841057906,-14.5339683530659,-0.861958333333496));
#29783=CARTESIAN_POINT('Ctrl Pts',(13.2690454743875,-15.5,-0.903625000000163));
#29784=CARTESIAN_POINT('Ctrl Pts',(13.8267841057906,-16.4660316469341,-0.94529166666683));
#29785=CARTESIAN_POINT('Ctrl Pts',(14.3845227371938,-17.4320632938683,-0.986958333333498));
#29786=CARTESIAN_POINT('Ctrl Pts',(15.5,-17.4320632938683,-1.02862500000016));
#29787=CARTESIAN_POINT('Ctrl Pts',(16.6154772628062,-17.4320632938683,-1.07029166666683));
#29788=CARTESIAN_POINT('Ctrl Pts',(17.1732158942094,-16.4660316469341,-1.1119583333335));
#29789=CARTESIAN_POINT('Ctrl Pts',(17.7309545256125,-15.5,-1.15362500000017));
#29790=CARTESIAN_POINT('Ctrl Pts',(17.1732158942094,-14.5339683530659,-1.19529166666683));
#29791=CARTESIAN_POINT('Ctrl Pts',(16.6154772628062,-13.5679367061317,-1.2369583333335));
#29792=CARTESIAN_POINT('Ctrl Pts',(15.5,-13.5679367061317,-1.27862500000017));
#29793=CARTESIAN_POINT('Ctrl Pts',(14.3845227371938,-13.5679367061317,-1.32029166666684));
#29794=CARTESIAN_POINT('Ctrl Pts',(13.8267841057906,-14.5339683530659,-1.3619583333335));
#29795=CARTESIAN_POINT('Ctrl Pts',(13.2690454743875,-15.5,-1.40362500000017));
#29796=CARTESIAN_POINT('Ctrl Pts',(13.8267841057906,-16.4660316469341,-1.44529166666684));
#29797=CARTESIAN_POINT('Ctrl Pts',(14.3845227371938,-17.4320632938683,-1.4869583333335));
#29798=CARTESIAN_POINT('Ctrl Pts',(15.5,-17.4320632938683,-1.52862500000017));
#29799=CARTESIAN_POINT('Ctrl Pts',(16.6154772628062,-17.4320632938683,-1.57029166666684));
#29800=CARTESIAN_POINT('Ctrl Pts',(17.1732158942094,-16.4660316469341,-1.61195833333351));
#29801=CARTESIAN_POINT('Ctrl Pts',(17.7309545256125,-15.5,-1.65362500000017));
#29802=CARTESIAN_POINT('Ctrl Pts',(17.1732158942094,-14.5339683530659,-1.69529166666684));
#29803=CARTESIAN_POINT('Ctrl Pts',(16.6154772628062,-13.5679367061317,-1.73695833333351));
#29804=CARTESIAN_POINT('Ctrl Pts',(15.5,-13.5679367061317,-1.77862500000017));
#29805=CARTESIAN_POINT('Ctrl Pts',(14.3845227371938,-13.5679367061317,-1.82029166666684));
#29806=CARTESIAN_POINT('Ctrl Pts',(13.8267841057906,-14.5339683530659,-1.86195833333351));
#29807=CARTESIAN_POINT('Ctrl Pts',(13.2690454743875,-15.5,-1.90362500000018));
#29808=CARTESIAN_POINT('Ctrl Pts',(13.8267841057906,-16.4660316469341,-1.94529166666684));
#29809=CARTESIAN_POINT('Ctrl Pts',(14.3845227371938,-17.4320632938683,-1.98695833333351));
#29810=CARTESIAN_POINT('Ctrl Pts',(15.5,-17.4320632938683,-2.02862500000018));
#29811=CARTESIAN_POINT('Ctrl Pts',(16.6154772628062,-17.4320632938683,-2.07029166666685));
#29812=CARTESIAN_POINT('Ctrl Pts',(17.1732158942094,-16.4660316469341,-2.11195833333351));
#29813=CARTESIAN_POINT('Ctrl Pts',(17.7309545256125,-15.5,-2.15362500000018));
#29814=CARTESIAN_POINT('Ctrl Pts',(17.1732158942094,-14.5339683530659,-2.19529166666685));
#29815=CARTESIAN_POINT('Ctrl Pts',(16.9678747970191,-14.1783071398504,-2.21063196867905));
#29816=CARTESIAN_POINT('Ctrl Pts',(16.6356236599184,-13.9369173167914,-2.22824840486548));
#29817=CARTESIAN_POINT('',(16.4288320706156,-14.2215513317122,-2.02512305032214));
#29818=CARTESIAN_POINT('Ctrl Pts',(15.2436450846258,-13.9406917842497,10.4122404735808));
#29819=CARTESIAN_POINT('Ctrl Pts',(14.5054990725557,-14.0620451873462,10.3753299573543));
#29820=CARTESIAN_POINT('Ctrl Pts',(14.1314716057906,-14.7098797632096,10.3411666666667));
#29821=CARTESIAN_POINT('Ctrl Pts',(13.6752954743875,-15.5,10.2995));
#29822=CARTESIAN_POINT('Ctrl Pts',(14.1314716057906,-16.2901202367904,10.2578333333333));
#29823=CARTESIAN_POINT('Ctrl Pts',(14.5876477371938,-17.0802404735808,10.2161666666667));
#29824=CARTESIAN_POINT('Ctrl Pts',(15.5,-17.0802404735808,10.1745));
#29825=CARTESIAN_POINT('Ctrl Pts',(16.4123522628062,-17.0802404735808,10.1328333333333));
#29826=CARTESIAN_POINT('Ctrl Pts',(16.8685283942094,-16.2901202367904,10.0911666666667));
#29827=CARTESIAN_POINT('Ctrl Pts',(17.3247045256125,-15.5,10.0495));
#29828=CARTESIAN_POINT('Ctrl Pts',(16.8685283942094,-14.7098797632096,10.0078333333333));
#29829=CARTESIAN_POINT('Ctrl Pts',(16.4123522628062,-13.9197595264192,9.96616666666665));
#29830=CARTESIAN_POINT('Ctrl Pts',(15.5,-13.9197595264192,9.92449999999998));
#29831=CARTESIAN_POINT('Ctrl Pts',(14.5876477371938,-13.9197595264192,9.88283333333331));
#29832=CARTESIAN_POINT('Ctrl Pts',(14.1314716057906,-14.7098797632096,9.84116666666665));
#29833=CARTESIAN_POINT('Ctrl Pts',(13.6752954743875,-15.5,9.79949999999998));
#29834=CARTESIAN_POINT('Ctrl Pts',(14.1314716057906,-16.2901202367904,9.75783333333331));
#29835=CARTESIAN_POINT('Ctrl Pts',(14.5876477371938,-17.0802404735808,9.71616666666665));
#29836=CARTESIAN_POINT('Ctrl Pts',(15.5,-17.0802404735808,9.67449999999998));
#29837=CARTESIAN_POINT('Ctrl Pts',(16.4123522628062,-17.0802404735808,9.63283333333331));
#29838=CARTESIAN_POINT('Ctrl Pts',(16.8685283942094,-16.2901202367904,9.59116666666664));
#29839=CARTESIAN_POINT('Ctrl Pts',(17.3247045256125,-15.5,9.54949999999998));
#29840=CARTESIAN_POINT('Ctrl Pts',(16.8685283942094,-14.7098797632096,9.50783333333331));
#29841=CARTESIAN_POINT('Ctrl Pts',(16.4123522628062,-13.9197595264192,9.46616666666664));
#29842=CARTESIAN_POINT('Ctrl Pts',(15.5,-13.9197595264192,9.42449999999998));
#29843=CARTESIAN_POINT('Ctrl Pts',(14.5876477371938,-13.9197595264192,9.38283333333331));
#29844=CARTESIAN_POINT('Ctrl Pts',(14.1314716057906,-14.7098797632096,9.34116666666664));
#29845=CARTESIAN_POINT('Ctrl Pts',(13.6752954743875,-15.5,9.29949999999997));
#29846=CARTESIAN_POINT('Ctrl Pts',(14.1314716057906,-16.2901202367904,9.25783333333331));
#29847=CARTESIAN_POINT('Ctrl Pts',(14.5876477371938,-17.0802404735808,9.21616666666664));
#29848=CARTESIAN_POINT('Ctrl Pts',(15.5,-17.0802404735808,9.17449999999997));
#29849=CARTESIAN_POINT('Ctrl Pts',(16.4123522628062,-17.0802404735808,9.13283333333331));
#29850=CARTESIAN_POINT('Ctrl Pts',(16.8685283942094,-16.2901202367904,9.09116666666664));
#29851=CARTESIAN_POINT('Ctrl Pts',(17.3247045256125,-15.5,9.04949999999997));
#29852=CARTESIAN_POINT('Ctrl Pts',(16.8685283942094,-14.7098797632096,9.0078333333333));
#29853=CARTESIAN_POINT('Ctrl Pts',(16.4123522628062,-13.9197595264192,8.96616666666664));
#29854=CARTESIAN_POINT('Ctrl Pts',(15.5,-13.9197595264192,8.92449999999997));
#29855=CARTESIAN_POINT('Ctrl Pts',(14.5876477371938,-13.9197595264192,8.8828333333333));
#29856=CARTESIAN_POINT('Ctrl Pts',(14.1314716057906,-14.7098797632096,8.84116666666664));
#29857=CARTESIAN_POINT('Ctrl Pts',(13.6752954743875,-15.5,8.79949999999997));
#29858=CARTESIAN_POINT('Ctrl Pts',(14.1314716057906,-16.2901202367904,8.7578333333333));
#29859=CARTESIAN_POINT('Ctrl Pts',(14.5876477371938,-17.0802404735808,8.71616666666663));
#29860=CARTESIAN_POINT('Ctrl Pts',(15.5,-17.0802404735808,8.67449999999997));
#29861=CARTESIAN_POINT('Ctrl Pts',(16.4123522628062,-17.0802404735808,8.6328333333333));
#29862=CARTESIAN_POINT('Ctrl Pts',(16.8685283942094,-16.2901202367904,8.59116666666663));
#29863=CARTESIAN_POINT('Ctrl Pts',(17.3247045256125,-15.5,8.54949999999996));
#29864=CARTESIAN_POINT('Ctrl Pts',(16.8685283942094,-14.7098797632096,8.50783333333329));
#29865=CARTESIAN_POINT('Ctrl Pts',(16.4123522628062,-13.9197595264192,8.46616666666663));
#29866=CARTESIAN_POINT('Ctrl Pts',(15.5,-13.9197595264192,8.42449999999996));
#29867=CARTESIAN_POINT('Ctrl Pts',(14.5876477371938,-13.9197595264192,8.38283333333329));
#29868=CARTESIAN_POINT('Ctrl Pts',(14.1314716057906,-14.7098797632096,8.34116666666663));
#29869=CARTESIAN_POINT('Ctrl Pts',(13.6752954743875,-15.5,8.29949999999996));
#29870=CARTESIAN_POINT('Ctrl Pts',(14.1314716057906,-16.2901202367904,8.25783333333329));
#29871=CARTESIAN_POINT('Ctrl Pts',(14.5876477371938,-17.0802404735808,8.21616666666663));
#29872=CARTESIAN_POINT('Ctrl Pts',(15.5,-17.0802404735808,8.17449999999996));
#29873=CARTESIAN_POINT('Ctrl Pts',(16.4123522628062,-17.0802404735808,8.13283333333329));
#29874=CARTESIAN_POINT('Ctrl Pts',(16.8685283942094,-16.2901202367904,8.09116666666663));
#29875=CARTESIAN_POINT('Ctrl Pts',(17.3247045256125,-15.5,8.04949999999996));
#29876=CARTESIAN_POINT('Ctrl Pts',(16.8685283942094,-14.7098797632096,8.00783333333329));
#29877=CARTESIAN_POINT('Ctrl Pts',(16.4123522628062,-13.9197595264192,7.96616666666662));
#29878=CARTESIAN_POINT('Ctrl Pts',(15.5,-13.9197595264192,7.92449999999996));
#29879=CARTESIAN_POINT('Ctrl Pts',(14.5876477371938,-13.9197595264192,7.88283333333329));
#29880=CARTESIAN_POINT('Ctrl Pts',(14.1314716057906,-14.7098797632096,7.84116666666662));
#29881=CARTESIAN_POINT('Ctrl Pts',(13.6752954743875,-15.5,7.79949999999995));
#29882=CARTESIAN_POINT('Ctrl Pts',(14.1314716057906,-16.2901202367904,7.75783333333329));
#29883=CARTESIAN_POINT('Ctrl Pts',(14.5876477371938,-17.0802404735808,7.71616666666662));
#29884=CARTESIAN_POINT('Ctrl Pts',(15.5,-17.0802404735808,7.67449999999995));
#29885=CARTESIAN_POINT('Ctrl Pts',(16.4123522628062,-17.0802404735808,7.63283333333328));
#29886=CARTESIAN_POINT('Ctrl Pts',(16.8685283942094,-16.2901202367904,7.59116666666662));
#29887=CARTESIAN_POINT('Ctrl Pts',(17.3247045256125,-15.5,7.54949999999995));
#29888=CARTESIAN_POINT('Ctrl Pts',(16.8685283942094,-14.7098797632096,7.50783333333328));
#29889=CARTESIAN_POINT('Ctrl Pts',(16.4123522628062,-13.9197595264192,7.46616666666662));
#29890=CARTESIAN_POINT('Ctrl Pts',(15.5,-13.9197595264192,7.42449999999995));
#29891=CARTESIAN_POINT('Ctrl Pts',(14.5876477371938,-13.9197595264192,7.38283333333328));
#29892=CARTESIAN_POINT('Ctrl Pts',(14.1314716057906,-14.7098797632096,7.34116666666661));
#29893=CARTESIAN_POINT('Ctrl Pts',(13.6752954743875,-15.5,7.29949999999995));
#29894=CARTESIAN_POINT('Ctrl Pts',(14.1314716057906,-16.2901202367904,7.25783333333328));
#29895=CARTESIAN_POINT('Ctrl Pts',(14.5876477371938,-17.0802404735808,7.21616666666661));
#29896=CARTESIAN_POINT('Ctrl Pts',(15.5,-17.0802404735808,7.17449999999995));
#29897=CARTESIAN_POINT('Ctrl Pts',(16.4123522628062,-17.0802404735808,7.13283333333328));
#29898=CARTESIAN_POINT('Ctrl Pts',(16.8685283942094,-16.2901202367904,7.09116666666661));
#29899=CARTESIAN_POINT('Ctrl Pts',(17.3247045256125,-15.5,7.04949999999994));
#29900=CARTESIAN_POINT('Ctrl Pts',(16.8685283942094,-14.7098797632096,7.00783333333328));
#29901=CARTESIAN_POINT('Ctrl Pts',(16.4123522628062,-13.9197595264192,6.96616666666661));
#29902=CARTESIAN_POINT('Ctrl Pts',(15.5,-13.9197595264192,6.92449999999994));
#29903=CARTESIAN_POINT('Ctrl Pts',(14.5876477371938,-13.9197595264192,6.88283333333327));
#29904=CARTESIAN_POINT('Ctrl Pts',(14.1314716057906,-14.7098797632096,6.84116666666661));
#29905=CARTESIAN_POINT('Ctrl Pts',(13.6752954743875,-15.5,6.79949999999994));
#29906=CARTESIAN_POINT('Ctrl Pts',(14.1314716057906,-16.2901202367904,6.75783333333327));
#29907=CARTESIAN_POINT('Ctrl Pts',(14.5876477371938,-17.0802404735808,6.71616666666661));
#29908=CARTESIAN_POINT('Ctrl Pts',(15.5,-17.0802404735808,6.67449999999994));
#29909=CARTESIAN_POINT('Ctrl Pts',(16.4123522628062,-17.0802404735808,6.63283333333327));
#29910=CARTESIAN_POINT('Ctrl Pts',(16.8685283942094,-16.2901202367904,6.59116666666661));
#29911=CARTESIAN_POINT('Ctrl Pts',(17.3247045256125,-15.5,6.54949999999994));
#29912=CARTESIAN_POINT('Ctrl Pts',(16.8685283942094,-14.7098797632096,6.50783333333327));
#29913=CARTESIAN_POINT('Ctrl Pts',(16.4123522628062,-13.9197595264192,6.4661666666666));
#29914=CARTESIAN_POINT('Ctrl Pts',(15.5,-13.9197595264192,6.42449999999994));
#29915=CARTESIAN_POINT('Ctrl Pts',(14.5876477371938,-13.9197595264192,6.38283333333327));
#29916=CARTESIAN_POINT('Ctrl Pts',(14.1314716057906,-14.7098797632096,6.3411666666666));
#29917=CARTESIAN_POINT('Ctrl Pts',(13.6752954743875,-15.5,6.29949999999993));
#29918=CARTESIAN_POINT('Ctrl Pts',(14.1314716057906,-16.2901202367904,6.25783333333327));
#29919=CARTESIAN_POINT('Ctrl Pts',(14.5876477371938,-17.0802404735808,6.2161666666666));
#29920=CARTESIAN_POINT('Ctrl Pts',(15.5,-17.0802404735808,6.17449999999993));
#29921=CARTESIAN_POINT('Ctrl Pts',(16.4123522628062,-17.0802404735808,6.13283333333326));
#29922=CARTESIAN_POINT('Ctrl Pts',(16.8685283942094,-16.2901202367904,6.0911666666666));
#29923=CARTESIAN_POINT('Ctrl Pts',(17.3247045256125,-15.5,6.04949999999993));
#29924=CARTESIAN_POINT('Ctrl Pts',(16.8685283942094,-14.7098797632096,6.00783333333326));
#29925=CARTESIAN_POINT('Ctrl Pts',(16.4123522628062,-13.9197595264192,5.9661666666666));
#29926=CARTESIAN_POINT('Ctrl Pts',(15.5,-13.9197595264192,5.92449999999993));
#29927=CARTESIAN_POINT('Ctrl Pts',(14.5876477371938,-13.9197595264192,5.88283333333326));
#29928=CARTESIAN_POINT('Ctrl Pts',(14.1314716057906,-14.7098797632096,5.8411666666666));
#29929=CARTESIAN_POINT('Ctrl Pts',(13.6752954743875,-15.5,5.79949999999993));
#29930=CARTESIAN_POINT('Ctrl Pts',(14.1314716057906,-16.2901202367904,5.75783333333326));
#29931=CARTESIAN_POINT('Ctrl Pts',(14.5876477371938,-17.0802404735808,5.71616666666659));
#29932=CARTESIAN_POINT('Ctrl Pts',(15.5,-17.0802404735808,5.67449999999993));
#29933=CARTESIAN_POINT('Ctrl Pts',(16.4123522628062,-17.0802404735808,5.63283333333326));
#29934=CARTESIAN_POINT('Ctrl Pts',(16.8685283942094,-16.2901202367904,5.59116666666659));
#29935=CARTESIAN_POINT('Ctrl Pts',(17.3247045256125,-15.5,5.54949999999992));
#29936=CARTESIAN_POINT('Ctrl Pts',(16.8685283942094,-14.7098797632096,5.50783333333326));
#29937=CARTESIAN_POINT('Ctrl Pts',(16.4123522628062,-13.9197595264192,5.46616666666659));
#29938=CARTESIAN_POINT('Ctrl Pts',(15.5,-13.9197595264192,5.42449999999992));
#29939=CARTESIAN_POINT('Ctrl Pts',(14.5876477371938,-13.9197595264192,5.38283333333326));
#29940=CARTESIAN_POINT('Ctrl Pts',(14.1314716057906,-14.7098797632096,5.34116666666659));
#29941=CARTESIAN_POINT('Ctrl Pts',(13.6752954743875,-15.5,5.29949999999992));
#29942=CARTESIAN_POINT('Ctrl Pts',(14.1314716057906,-16.2901202367904,5.25783333333325));
#29943=CARTESIAN_POINT('Ctrl Pts',(14.5876477371938,-17.0802404735808,5.21616666666659));
#29944=CARTESIAN_POINT('Ctrl Pts',(15.5,-17.0802404735808,5.17449999999992));
#29945=CARTESIAN_POINT('Ctrl Pts',(16.4123522628062,-17.0802404735808,5.13283333333325));
#29946=CARTESIAN_POINT('Ctrl Pts',(16.8685283942094,-16.2901202367904,5.09116666666658));
#29947=CARTESIAN_POINT('Ctrl Pts',(17.3247045256125,-15.5,5.04949999999992));
#29948=CARTESIAN_POINT('Ctrl Pts',(16.8685283942094,-14.7098797632096,5.00783333333325));
#29949=CARTESIAN_POINT('Ctrl Pts',(16.4123522628062,-13.9197595264192,4.96616666666658));
#29950=CARTESIAN_POINT('Ctrl Pts',(15.5,-13.9197595264192,4.92449999999992));
#29951=CARTESIAN_POINT('Ctrl Pts',(14.5876477371938,-13.9197595264192,4.88283333333325));
#29952=CARTESIAN_POINT('Ctrl Pts',(14.1314716057906,-14.7098797632096,4.84116666666658));
#29953=CARTESIAN_POINT('Ctrl Pts',(13.6752954743875,-15.5,4.79949999999991));
#29954=CARTESIAN_POINT('Ctrl Pts',(14.1314716057906,-16.2901202367904,4.75783333333325));
#29955=CARTESIAN_POINT('Ctrl Pts',(14.5876477371938,-17.0802404735808,4.71616666666658));
#29956=CARTESIAN_POINT('Ctrl Pts',(15.5,-17.0802404735808,4.67449999999991));
#29957=CARTESIAN_POINT('Ctrl Pts',(16.4123522628062,-17.0802404735808,4.63283333333325));
#29958=CARTESIAN_POINT('Ctrl Pts',(16.8685283942094,-16.2901202367904,4.59116666666658));
#29959=CARTESIAN_POINT('Ctrl Pts',(17.3247045256125,-15.5,4.54949999999991));
#29960=CARTESIAN_POINT('Ctrl Pts',(16.8685283942094,-14.7098797632096,4.50783333333324));
#29961=CARTESIAN_POINT('Ctrl Pts',(16.4123522628062,-13.9197595264192,4.46616666666658));
#29962=CARTESIAN_POINT('Ctrl Pts',(15.5,-13.9197595264192,4.42449999999991));
#29963=CARTESIAN_POINT('Ctrl Pts',(14.5876477371938,-13.9197595264192,4.38283333333324));
#29964=CARTESIAN_POINT('Ctrl Pts',(14.1314716057906,-14.7098797632096,4.34116666666657));
#29965=CARTESIAN_POINT('Ctrl Pts',(13.6752954743875,-15.5,4.29949999999991));
#29966=CARTESIAN_POINT('Ctrl Pts',(14.1314716057906,-16.2901202367904,4.25783333333324));
#29967=CARTESIAN_POINT('Ctrl Pts',(14.5876477371938,-17.0802404735808,4.21616666666657));
#29968=CARTESIAN_POINT('Ctrl Pts',(15.5,-17.0802404735808,4.17449999999991));
#29969=CARTESIAN_POINT('Ctrl Pts',(16.4123522628062,-17.0802404735808,4.13283333333324));
#29970=CARTESIAN_POINT('Ctrl Pts',(16.8685283942094,-16.2901202367904,4.09116666666657));
#29971=CARTESIAN_POINT('Ctrl Pts',(17.3247045256125,-15.5,4.0494999999999));
#29972=CARTESIAN_POINT('Ctrl Pts',(16.8685283942094,-14.7098797632096,4.00783333333324));
#29973=CARTESIAN_POINT('Ctrl Pts',(16.4123522628062,-13.9197595264192,3.96616666666657));
#29974=CARTESIAN_POINT('Ctrl Pts',(15.5,-13.9197595264192,3.9244999999999));
#29975=CARTESIAN_POINT('Ctrl Pts',(14.5876477371938,-13.9197595264192,3.88283333333323));
#29976=CARTESIAN_POINT('Ctrl Pts',(14.1314716057906,-14.7098797632096,3.84116666666657));
#29977=CARTESIAN_POINT('Ctrl Pts',(13.6752954743875,-15.5,3.7994999999999));
#29978=CARTESIAN_POINT('Ctrl Pts',(14.1314716057906,-16.2901202367904,3.75783333333323));
#29979=CARTESIAN_POINT('Ctrl Pts',(14.5876477371938,-17.0802404735808,3.71616666666657));
#29980=CARTESIAN_POINT('Ctrl Pts',(15.5,-17.0802404735808,3.6744999999999));
#29981=CARTESIAN_POINT('Ctrl Pts',(16.4123522628062,-17.0802404735808,3.63283333333323));
#29982=CARTESIAN_POINT('Ctrl Pts',(16.8685283942094,-16.2901202367904,3.59116666666656));
#29983=CARTESIAN_POINT('Ctrl Pts',(17.3247045256125,-15.5,3.5494999999999));
#29984=CARTESIAN_POINT('Ctrl Pts',(16.8685283942094,-14.7098797632096,3.50783333333323));
#29985=CARTESIAN_POINT('Ctrl Pts',(16.4123522628062,-13.9197595264192,3.46616666666656));
#29986=CARTESIAN_POINT('Ctrl Pts',(15.5,-13.9197595264192,3.4244999999999));
#29987=CARTESIAN_POINT('Ctrl Pts',(14.5876477371938,-13.9197595264192,3.38283333333323));
#29988=CARTESIAN_POINT('Ctrl Pts',(14.1314716057906,-14.7098797632096,3.34116666666656));
#29989=CARTESIAN_POINT('Ctrl Pts',(13.6752954743875,-15.5,3.29949999999989));
#29990=CARTESIAN_POINT('Ctrl Pts',(14.1314716057906,-16.2901202367904,3.25783333333323));
#29991=CARTESIAN_POINT('Ctrl Pts',(14.5876477371938,-17.0802404735808,3.21616666666656));
#29992=CARTESIAN_POINT('Ctrl Pts',(15.5,-17.0802404735808,3.17449999999989));
#29993=CARTESIAN_POINT('Ctrl Pts',(16.4123522628062,-17.0802404735808,3.13283333333323));
#29994=CARTESIAN_POINT('Ctrl Pts',(16.8685283942094,-16.2901202367904,3.09116666666656));
#29995=CARTESIAN_POINT('Ctrl Pts',(17.3247045256125,-15.5,3.04949999999989));
#29996=CARTESIAN_POINT('Ctrl Pts',(16.8685283942094,-14.7098797632096,3.00783333333322));
#29997=CARTESIAN_POINT('Ctrl Pts',(16.4123522628062,-13.9197595264192,2.96616666666656));
#29998=CARTESIAN_POINT('Ctrl Pts',(15.5,-13.9197595264192,2.92449999999989));
#29999=CARTESIAN_POINT('Ctrl Pts',(14.5876477371938,-13.9197595264192,2.88283333333322));
#30000=CARTESIAN_POINT('Ctrl Pts',(14.1314716057906,-14.7098797632096,2.84116666666655));
#30001=CARTESIAN_POINT('Ctrl Pts',(13.6752954743875,-15.5,2.79949999999989));
#30002=CARTESIAN_POINT('Ctrl Pts',(14.1314716057906,-16.2901202367904,2.75783333333322));
#30003=CARTESIAN_POINT('Ctrl Pts',(14.5876477371938,-17.0802404735808,2.71616666666655));
#30004=CARTESIAN_POINT('Ctrl Pts',(15.5,-17.0802404735808,2.67449999999989));
#30005=CARTESIAN_POINT('Ctrl Pts',(16.4123522628062,-17.0802404735808,2.63283333333322));
#30006=CARTESIAN_POINT('Ctrl Pts',(16.8685283942094,-16.2901202367904,2.59116666666655));
#30007=CARTESIAN_POINT('Ctrl Pts',(17.3247045256125,-15.5,2.54949999999988));
#30008=CARTESIAN_POINT('Ctrl Pts',(16.8685283942094,-14.7098797632096,2.50783333333322));
#30009=CARTESIAN_POINT('Ctrl Pts',(16.4123522628062,-13.9197595264192,2.46616666666655));
#30010=CARTESIAN_POINT('Ctrl Pts',(15.5,-13.9197595264192,2.42449999999988));
#30011=CARTESIAN_POINT('Ctrl Pts',(14.5876477371938,-13.9197595264192,2.38283333333321));
#30012=CARTESIAN_POINT('Ctrl Pts',(14.1314716057906,-14.7098797632096,2.34116666666655));
#30013=CARTESIAN_POINT('Ctrl Pts',(13.6752954743875,-15.5,2.29949999999988));
#30014=CARTESIAN_POINT('Ctrl Pts',(14.1314716057906,-16.2901202367904,2.25783333333321));
#30015=CARTESIAN_POINT('Ctrl Pts',(14.5876477371938,-17.0802404735808,2.21616666666655));
#30016=CARTESIAN_POINT('Ctrl Pts',(15.5,-17.0802404735808,2.17449999999988));
#30017=CARTESIAN_POINT('Ctrl Pts',(16.4123522628062,-17.0802404735808,2.13283333333321));
#30018=CARTESIAN_POINT('Ctrl Pts',(16.8685283942094,-16.2901202367904,2.09116666666655));
#30019=CARTESIAN_POINT('Ctrl Pts',(17.3247045256125,-15.5,2.04949999999988));
#30020=CARTESIAN_POINT('Ctrl Pts',(16.8685283942094,-14.7098797632096,2.00783333333321));
#30021=CARTESIAN_POINT('Ctrl Pts',(16.4123522628062,-13.9197595264192,1.96616666666654));
#30022=CARTESIAN_POINT('Ctrl Pts',(15.5,-13.9197595264192,1.92449999999988));
#30023=CARTESIAN_POINT('Ctrl Pts',(14.5876477371938,-13.9197595264192,1.88283333333321));
#30024=CARTESIAN_POINT('Ctrl Pts',(14.1314716057906,-14.7098797632096,1.84116666666654));
#30025=CARTESIAN_POINT('Ctrl Pts',(13.6752954743875,-15.5,1.79949999999987));
#30026=CARTESIAN_POINT('Ctrl Pts',(14.1314716057906,-16.2901202367904,1.75783333333321));
#30027=CARTESIAN_POINT('Ctrl Pts',(14.5876477371938,-17.0802404735808,1.71616666666654));
#30028=CARTESIAN_POINT('Ctrl Pts',(15.5,-17.0802404735808,1.67449999999987));
#30029=CARTESIAN_POINT('Ctrl Pts',(16.4123522628062,-17.0802404735808,1.63283333333321));
#30030=CARTESIAN_POINT('Ctrl Pts',(16.8685283942094,-16.2901202367904,1.59116666666654));
#30031=CARTESIAN_POINT('Ctrl Pts',(17.3247045256125,-15.5,1.54949999999987));
#30032=CARTESIAN_POINT('Ctrl Pts',(16.8685283942094,-14.7098797632096,1.5078333333332));
#30033=CARTESIAN_POINT('Ctrl Pts',(16.4123522628062,-13.9197595264192,1.46616666666654));
#30034=CARTESIAN_POINT('Ctrl Pts',(15.5,-13.9197595264192,1.42449999999987));
#30035=CARTESIAN_POINT('Ctrl Pts',(14.5876477371938,-13.9197595264192,1.3828333333332));
#30036=CARTESIAN_POINT('Ctrl Pts',(14.1314716057906,-14.7098797632096,1.34116666666653));
#30037=CARTESIAN_POINT('Ctrl Pts',(13.6752954743875,-15.5,1.29949999999987));
#30038=CARTESIAN_POINT('Ctrl Pts',(14.1314716057906,-16.2901202367904,1.2578333333332));
#30039=CARTESIAN_POINT('Ctrl Pts',(14.5876477371938,-17.0802404735808,1.21616666666653));
#30040=CARTESIAN_POINT('Ctrl Pts',(15.5,-17.0802404735808,1.17449999999986));
#30041=CARTESIAN_POINT('Ctrl Pts',(16.4123522628062,-17.0802404735808,1.1328333333332));
#30042=CARTESIAN_POINT('Ctrl Pts',(16.8685283942094,-16.2901202367904,1.09116666666653));
#30043=CARTESIAN_POINT('Ctrl Pts',(17.3247045256125,-15.5,1.04949999999987));
#30044=CARTESIAN_POINT('Ctrl Pts',(16.8685283942094,-14.7098797632096,1.0078333333332));
#30045=CARTESIAN_POINT('Ctrl Pts',(16.4123522628062,-13.9197595264192,0.96616666666653));
#30046=CARTESIAN_POINT('Ctrl Pts',(15.5,-13.9197595264192,0.924499999999863));
#30047=CARTESIAN_POINT('Ctrl Pts',(14.5876477371938,-13.9197595264192,0.882833333333196));
#30048=CARTESIAN_POINT('Ctrl Pts',(14.1314716057906,-14.7098797632096,0.841166666666529));
#30049=CARTESIAN_POINT('Ctrl Pts',(13.6752954743875,-15.5,0.799499999999861));
#30050=CARTESIAN_POINT('Ctrl Pts',(14.1314716057906,-16.2901202367904,0.757833333333194));
#30051=CARTESIAN_POINT('Ctrl Pts',(14.5876477371938,-17.0802404735808,0.716166666666527));
#30052=CARTESIAN_POINT('Ctrl Pts',(15.5,-17.0802404735808,0.674499999999859));
#30053=CARTESIAN_POINT('Ctrl Pts',(16.4123522628062,-17.0802404735808,0.632833333333192));
#30054=CARTESIAN_POINT('Ctrl Pts',(16.8685283942094,-16.2901202367904,0.591166666666525));
#30055=CARTESIAN_POINT('Ctrl Pts',(17.3247045256125,-15.5,0.549499999999857));
#30056=CARTESIAN_POINT('Ctrl Pts',(16.8685283942094,-14.7098797632096,0.50783333333319));
#30057=CARTESIAN_POINT('Ctrl Pts',(16.4123522628062,-13.9197595264192,0.466166666666523));
#30058=CARTESIAN_POINT('Ctrl Pts',(15.5,-13.9197595264192,0.424499999999856));
#30059=CARTESIAN_POINT('Ctrl Pts',(14.5876477371938,-13.9197595264192,0.382833333333188));
#30060=CARTESIAN_POINT('Ctrl Pts',(14.1314716057906,-14.7098797632096,0.341166666666521));
#30061=CARTESIAN_POINT('Ctrl Pts',(13.6752954743875,-15.5,0.299499999999854));
#30062=CARTESIAN_POINT('Ctrl Pts',(14.1314716057906,-16.2901202367904,0.257833333333186));
#30063=CARTESIAN_POINT('Ctrl Pts',(14.5876477371938,-17.0802404735808,0.216166666666519));
#30064=CARTESIAN_POINT('Ctrl Pts',(15.5,-17.0802404735808,0.174499999999852));
#30065=CARTESIAN_POINT('Ctrl Pts',(16.4123522628062,-17.0802404735808,0.132833333333185));
#30066=CARTESIAN_POINT('Ctrl Pts',(16.8685283942094,-16.2901202367904,0.0911666666665173));
#30067=CARTESIAN_POINT('Ctrl Pts',(17.3247045256125,-15.5,0.04949999999985));
#30068=CARTESIAN_POINT('Ctrl Pts',(16.8685283942094,-14.7098797632096,0.00783333333318273));
#30069=CARTESIAN_POINT('Ctrl Pts',(16.4123522628062,-13.9197595264192,-0.0338333333334846));
#30070=CARTESIAN_POINT('Ctrl Pts',(15.5,-13.9197595264192,-0.0755000000001518));
#30071=CARTESIAN_POINT('Ctrl Pts',(14.5876477371938,-13.9197595264192,-0.117166666666817));
#30072=CARTESIAN_POINT('Ctrl Pts',(14.1314716057906,-14.7098797632096,-0.158833333333485));
#30073=CARTESIAN_POINT('Ctrl Pts',(13.6752954743875,-15.5,-0.200500000000152));
#30074=CARTESIAN_POINT('Ctrl Pts',(14.1314716057906,-16.2901202367904,-0.242166666666819));
#30075=CARTESIAN_POINT('Ctrl Pts',(14.5876477371938,-17.0802404735808,-0.283833333333487));
#30076=CARTESIAN_POINT('Ctrl Pts',(15.5,-17.0802404735808,-0.325500000000154));
#30077=CARTESIAN_POINT('Ctrl Pts',(16.4123522628062,-17.0802404735808,-0.367166666666821));
#30078=CARTESIAN_POINT('Ctrl Pts',(16.8685283942094,-16.2901202367904,-0.408833333333488));
#30079=CARTESIAN_POINT('Ctrl Pts',(17.3247045256125,-15.5,-0.450500000000156));
#30080=CARTESIAN_POINT('Ctrl Pts',(16.8685283942094,-14.7098797632096,-0.492166666666823));
#30081=CARTESIAN_POINT('Ctrl Pts',(16.4123522628062,-13.9197595264192,-0.53383333333349));
#30082=CARTESIAN_POINT('Ctrl Pts',(15.5,-13.9197595264192,-0.575500000000157));
#30083=CARTESIAN_POINT('Ctrl Pts',(14.5876477371938,-13.9197595264192,-0.617166666666825));
#30084=CARTESIAN_POINT('Ctrl Pts',(14.1314716057906,-14.7098797632096,-0.658833333333492));
#30085=CARTESIAN_POINT('Ctrl Pts',(13.6752954743875,-15.5,-0.700500000000159));
#30086=CARTESIAN_POINT('Ctrl Pts',(14.1314716057906,-16.2901202367904,-0.742166666666827));
#30087=CARTESIAN_POINT('Ctrl Pts',(14.5876477371938,-17.0802404735808,-0.783833333333494));
#30088=CARTESIAN_POINT('Ctrl Pts',(15.5,-17.0802404735808,-0.825500000000161));
#30089=CARTESIAN_POINT('Ctrl Pts',(16.4123522628062,-17.0802404735808,-0.867166666666829));
#30090=CARTESIAN_POINT('Ctrl Pts',(16.8685283942094,-16.2901202367904,-0.908833333333496));
#30091=CARTESIAN_POINT('Ctrl Pts',(17.3247045256125,-15.5,-0.950500000000163));
#30092=CARTESIAN_POINT('Ctrl Pts',(16.8685283942094,-14.7098797632096,-0.99216666666683));
#30093=CARTESIAN_POINT('Ctrl Pts',(16.4123522628062,-13.9197595264192,-1.0338333333335));
#30094=CARTESIAN_POINT('Ctrl Pts',(15.5,-13.9197595264192,-1.07550000000016));
#30095=CARTESIAN_POINT('Ctrl Pts',(14.5876477371938,-13.9197595264192,-1.11716666666683));
#30096=CARTESIAN_POINT('Ctrl Pts',(14.1314716057906,-14.7098797632096,-1.1588333333335));
#30097=CARTESIAN_POINT('Ctrl Pts',(13.6752954743875,-15.5,-1.20050000000017));
#30098=CARTESIAN_POINT('Ctrl Pts',(14.1314716057906,-16.2901202367904,-1.24216666666683));
#30099=CARTESIAN_POINT('Ctrl Pts',(14.5876477371938,-17.0802404735808,-1.2838333333335));
#30100=CARTESIAN_POINT('Ctrl Pts',(15.5,-17.0802404735808,-1.32550000000017));
#30101=CARTESIAN_POINT('Ctrl Pts',(16.4123522628062,-17.0802404735808,-1.36716666666683));
#30102=CARTESIAN_POINT('Ctrl Pts',(16.8685283942094,-16.2901202367904,-1.4088333333335));
#30103=CARTESIAN_POINT('Ctrl Pts',(17.3247045256125,-15.5,-1.45050000000017));
#30104=CARTESIAN_POINT('Ctrl Pts',(16.8685283942094,-14.7098797632096,-1.49216666666684));
#30105=CARTESIAN_POINT('Ctrl Pts',(16.4123522628062,-13.9197595264192,-1.5338333333335));
#30106=CARTESIAN_POINT('Ctrl Pts',(15.5,-13.9197595264192,-1.57550000000017));
#30107=CARTESIAN_POINT('Ctrl Pts',(14.5876477371938,-13.9197595264192,-1.61716666666684));
#30108=CARTESIAN_POINT('Ctrl Pts',(14.1314716057906,-14.7098797632096,-1.65883333333351));
#30109=CARTESIAN_POINT('Ctrl Pts',(13.6752954743875,-15.5,-1.70050000000017));
#30110=CARTESIAN_POINT('Ctrl Pts',(14.1314716057906,-16.2901202367904,-1.74216666666684));
#30111=CARTESIAN_POINT('Ctrl Pts',(14.5876477371938,-17.0802404735808,-1.78383333333351));
#30112=CARTESIAN_POINT('Ctrl Pts',(15.5,-17.0802404735808,-1.82550000000017));
#30113=CARTESIAN_POINT('Ctrl Pts',(16.4123522628062,-17.0802404735808,-1.86716666666684));
#30114=CARTESIAN_POINT('Ctrl Pts',(16.8685283942094,-16.2901202367904,-1.90883333333351));
#30115=CARTESIAN_POINT('Ctrl Pts',(17.3247045256125,-15.5,-1.95050000000018));
#30116=CARTESIAN_POINT('Ctrl Pts',(16.8685283942094,-14.7098797632096,-1.99216666666684));
#30117=CARTESIAN_POINT('Ctrl Pts',(16.7005831533691,-14.4189900731849,-2.00750661517932));
#30118=CARTESIAN_POINT('Ctrl Pts',(16.4288360540161,-14.2215542486879,-2.02512301646327));
#30119=CARTESIAN_POINT('',(16.6356236599184,-13.9369173167914,-2.22824840486548));
#30120=CARTESIAN_POINT('Ctrl Pts',(15.5,-17.4320632938683,11.440125));
#30121=CARTESIAN_POINT('Ctrl Pts',(16.6154772628062,-17.4320632938683,11.3984583333333));
#30122=CARTESIAN_POINT('Ctrl Pts',(17.1732158942094,-16.4660316469341,11.3567916666667));
#30123=CARTESIAN_POINT('Ctrl Pts',(17.7309545256125,-15.5,11.315125));
#30124=CARTESIAN_POINT('Ctrl Pts',(17.1732158942094,-14.5339683530659,11.2734583333333));
#30125=CARTESIAN_POINT('Ctrl Pts',(16.6154772628062,-13.5679367061317,11.2317916666667));
#30126=CARTESIAN_POINT('Ctrl Pts',(15.5,-13.5679367061317,11.190125));
#30127=CARTESIAN_POINT('Ctrl Pts',(14.3845227371938,-13.5679367061317,11.1484583333333));
#30128=CARTESIAN_POINT('Ctrl Pts',(13.8267841057906,-14.5339683530659,11.1067916666667));
#30129=CARTESIAN_POINT('Ctrl Pts',(13.2690454743875,-15.5,11.065125));
#30130=CARTESIAN_POINT('Ctrl Pts',(13.8267841057906,-16.4660316469341,11.0234583333333));
#30131=CARTESIAN_POINT('Ctrl Pts',(14.3845227371938,-17.4320632938683,10.9817916666667));
#30132=CARTESIAN_POINT('Ctrl Pts',(15.5,-17.4320632938683,10.940125));
#30133=CARTESIAN_POINT('Ctrl Pts',(16.6154772628062,-17.4320632938683,10.8984583333333));
#30134=CARTESIAN_POINT('Ctrl Pts',(17.1732158942094,-16.4660316469341,10.8567916666667));
#30135=CARTESIAN_POINT('Ctrl Pts',(17.7309545256125,-15.5,10.815125));
#30136=CARTESIAN_POINT('Ctrl Pts',(17.1732158942094,-14.5339683530659,10.7734583333333));
#30137=CARTESIAN_POINT('Ctrl Pts',(16.6154772628062,-13.5679367061317,10.7317916666667));
#30138=CARTESIAN_POINT('Ctrl Pts',(15.5,-13.5679367061317,10.690125));
#30139=CARTESIAN_POINT('Ctrl Pts',(14.3845227371938,-13.5679367061317,10.6484583333333));
#30140=CARTESIAN_POINT('Ctrl Pts',(13.8267841057906,-14.5339683530659,10.6067916666667));
#30141=CARTESIAN_POINT('Ctrl Pts',(13.2690454743875,-15.5,10.565125));
#30142=CARTESIAN_POINT('Ctrl Pts',(13.8267841057906,-16.4660316469341,10.5234583333333));
#30143=CARTESIAN_POINT('Ctrl Pts',(14.3845227371938,-17.4320632938683,10.4817916666667));
#30144=CARTESIAN_POINT('Ctrl Pts',(15.5,-17.4320632938683,10.440125));
#30145=CARTESIAN_POINT('Ctrl Pts',(16.6154772628062,-17.4320632938683,10.3984583333333));
#30146=CARTESIAN_POINT('Ctrl Pts',(17.1732158942094,-16.4660316469341,10.3567916666667));
#30147=CARTESIAN_POINT('Ctrl Pts',(17.7309545256125,-15.5,10.315125));
#30148=CARTESIAN_POINT('Ctrl Pts',(17.1732158942094,-14.5339683530659,10.2734583333333));
#30149=CARTESIAN_POINT('Ctrl Pts',(16.6154772628062,-13.5679367061317,10.2317916666667));
#30150=CARTESIAN_POINT('Ctrl Pts',(15.5,-13.5679367061317,10.190125));
#30151=CARTESIAN_POINT('Ctrl Pts',(14.3845227371938,-13.5679367061317,10.1484583333333));
#30152=CARTESIAN_POINT('Ctrl Pts',(13.8267841057906,-14.5339683530659,10.1067916666666));
#30153=CARTESIAN_POINT('Ctrl Pts',(13.2690454743875,-15.5,10.065125));
#30154=CARTESIAN_POINT('Ctrl Pts',(13.8267841057906,-16.4660316469341,10.0234583333333));
#30155=CARTESIAN_POINT('Ctrl Pts',(14.3845227371938,-17.4320632938683,9.98179166666664));
#30156=CARTESIAN_POINT('Ctrl Pts',(15.5,-17.4320632938683,9.94012499999998));
#30157=CARTESIAN_POINT('Ctrl Pts',(16.6154772628062,-17.4320632938683,9.89845833333331));
#30158=CARTESIAN_POINT('Ctrl Pts',(17.1732158942094,-16.4660316469341,9.85679166666664));
#30159=CARTESIAN_POINT('Ctrl Pts',(17.7309545256125,-15.5,9.81512499999998));
#30160=CARTESIAN_POINT('Ctrl Pts',(17.1732158942094,-14.5339683530659,9.77345833333331));
#30161=CARTESIAN_POINT('Ctrl Pts',(16.6154772628062,-13.5679367061317,9.73179166666664));
#30162=CARTESIAN_POINT('Ctrl Pts',(15.5,-13.5679367061317,9.69012499999998));
#30163=CARTESIAN_POINT('Ctrl Pts',(14.3845227371938,-13.5679367061317,9.64845833333331));
#30164=CARTESIAN_POINT('Ctrl Pts',(13.8267841057906,-14.5339683530659,9.60679166666664));
#30165=CARTESIAN_POINT('Ctrl Pts',(13.2690454743875,-15.5,9.56512499999998));
#30166=CARTESIAN_POINT('Ctrl Pts',(13.8267841057906,-16.4660316469341,9.52345833333331));
#30167=CARTESIAN_POINT('Ctrl Pts',(14.3845227371938,-17.4320632938683,9.48179166666664));
#30168=CARTESIAN_POINT('Ctrl Pts',(15.5,-17.4320632938683,9.44012499999997));
#30169=CARTESIAN_POINT('Ctrl Pts',(16.6154772628062,-17.4320632938683,9.39845833333331));
#30170=CARTESIAN_POINT('Ctrl Pts',(17.1732158942094,-16.4660316469341,9.35679166666664));
#30171=CARTESIAN_POINT('Ctrl Pts',(17.7309545256125,-15.5,9.31512499999997));
#30172=CARTESIAN_POINT('Ctrl Pts',(17.1732158942094,-14.5339683530659,9.2734583333333));
#30173=CARTESIAN_POINT('Ctrl Pts',(16.6154772628062,-13.5679367061317,9.23179166666664));
#30174=CARTESIAN_POINT('Ctrl Pts',(15.5,-13.5679367061317,9.19012499999997));
#30175=CARTESIAN_POINT('Ctrl Pts',(14.3845227371938,-13.5679367061317,9.1484583333333));
#30176=CARTESIAN_POINT('Ctrl Pts',(13.8267841057906,-14.5339683530659,9.10679166666664));
#30177=CARTESIAN_POINT('Ctrl Pts',(13.2690454743875,-15.5,9.06512499999997));
#30178=CARTESIAN_POINT('Ctrl Pts',(13.8267841057906,-16.4660316469341,9.0234583333333));
#30179=CARTESIAN_POINT('Ctrl Pts',(14.3845227371938,-17.4320632938683,8.98179166666663));
#30180=CARTESIAN_POINT('Ctrl Pts',(15.5,-17.4320632938683,8.94012499999997));
#30181=CARTESIAN_POINT('Ctrl Pts',(16.6154772628062,-17.4320632938683,8.8984583333333));
#30182=CARTESIAN_POINT('Ctrl Pts',(17.1732158942094,-16.4660316469341,8.85679166666663));
#30183=CARTESIAN_POINT('Ctrl Pts',(17.7309545256125,-15.5,8.81512499999996));
#30184=CARTESIAN_POINT('Ctrl Pts',(17.1732158942094,-14.5339683530659,8.7734583333333));
#30185=CARTESIAN_POINT('Ctrl Pts',(16.6154772628062,-13.5679367061317,8.73179166666663));
#30186=CARTESIAN_POINT('Ctrl Pts',(15.5,-13.5679367061317,8.69012499999996));
#30187=CARTESIAN_POINT('Ctrl Pts',(14.3845227371938,-13.5679367061317,8.64845833333329));
#30188=CARTESIAN_POINT('Ctrl Pts',(13.8267841057906,-14.5339683530659,8.60679166666663));
#30189=CARTESIAN_POINT('Ctrl Pts',(13.2690454743875,-15.5,8.56512499999996));
#30190=CARTESIAN_POINT('Ctrl Pts',(13.8267841057906,-16.4660316469341,8.52345833333329));
#30191=CARTESIAN_POINT('Ctrl Pts',(14.3845227371938,-17.4320632938683,8.48179166666663));
#30192=CARTESIAN_POINT('Ctrl Pts',(15.5,-17.4320632938683,8.44012499999996));
#30193=CARTESIAN_POINT('Ctrl Pts',(16.6154772628062,-17.4320632938683,8.39845833333329));
#30194=CARTESIAN_POINT('Ctrl Pts',(17.1732158942094,-16.4660316469341,8.35679166666662));
#30195=CARTESIAN_POINT('Ctrl Pts',(17.7309545256125,-15.5,8.31512499999996));
#30196=CARTESIAN_POINT('Ctrl Pts',(17.1732158942094,-14.5339683530659,8.27345833333329));
#30197=CARTESIAN_POINT('Ctrl Pts',(16.6154772628062,-13.5679367061317,8.23179166666662));
#30198=CARTESIAN_POINT('Ctrl Pts',(15.5,-13.5679367061317,8.19012499999996));
#30199=CARTESIAN_POINT('Ctrl Pts',(14.3845227371938,-13.5679367061317,8.14845833333329));
#30200=CARTESIAN_POINT('Ctrl Pts',(13.8267841057906,-14.5339683530659,8.10679166666662));
#30201=CARTESIAN_POINT('Ctrl Pts',(13.2690454743875,-15.5,8.06512499999995));
#30202=CARTESIAN_POINT('Ctrl Pts',(13.8267841057906,-16.4660316469341,8.02345833333329));
#30203=CARTESIAN_POINT('Ctrl Pts',(14.3845227371938,-17.4320632938683,7.98179166666662));
#30204=CARTESIAN_POINT('Ctrl Pts',(15.5,-17.4320632938683,7.94012499999995));
#30205=CARTESIAN_POINT('Ctrl Pts',(16.6154772628062,-17.4320632938683,7.89845833333329));
#30206=CARTESIAN_POINT('Ctrl Pts',(17.1732158942094,-16.4660316469341,7.85679166666662));
#30207=CARTESIAN_POINT('Ctrl Pts',(17.7309545256125,-15.5,7.81512499999995));
#30208=CARTESIAN_POINT('Ctrl Pts',(17.1732158942094,-14.5339683530659,7.77345833333328));
#30209=CARTESIAN_POINT('Ctrl Pts',(16.6154772628062,-13.5679367061317,7.73179166666662));
#30210=CARTESIAN_POINT('Ctrl Pts',(15.5,-13.5679367061317,7.69012499999995));
#30211=CARTESIAN_POINT('Ctrl Pts',(14.3845227371938,-13.5679367061317,7.64845833333328));
#30212=CARTESIAN_POINT('Ctrl Pts',(13.8267841057906,-14.5339683530659,7.60679166666661));
#30213=CARTESIAN_POINT('Ctrl Pts',(13.2690454743875,-15.5,7.56512499999995));
#30214=CARTESIAN_POINT('Ctrl Pts',(13.8267841057906,-16.4660316469341,7.52345833333328));
#30215=CARTESIAN_POINT('Ctrl Pts',(14.3845227371938,-17.4320632938683,7.48179166666661));
#30216=CARTESIAN_POINT('Ctrl Pts',(15.5,-17.4320632938683,7.44012499999995));
#30217=CARTESIAN_POINT('Ctrl Pts',(16.6154772628062,-17.4320632938683,7.39845833333328));
#30218=CARTESIAN_POINT('Ctrl Pts',(17.1732158942094,-16.4660316469341,7.35679166666661));
#30219=CARTESIAN_POINT('Ctrl Pts',(17.7309545256125,-15.5,7.31512499999995));
#30220=CARTESIAN_POINT('Ctrl Pts',(17.1732158942094,-14.5339683530659,7.27345833333328));
#30221=CARTESIAN_POINT('Ctrl Pts',(16.6154772628062,-13.5679367061317,7.23179166666661));
#30222=CARTESIAN_POINT('Ctrl Pts',(15.5,-13.5679367061317,7.19012499999994));
#30223=CARTESIAN_POINT('Ctrl Pts',(14.3845227371938,-13.5679367061317,7.14845833333328));
#30224=CARTESIAN_POINT('Ctrl Pts',(13.8267841057906,-14.5339683530659,7.10679166666661));
#30225=CARTESIAN_POINT('Ctrl Pts',(13.2690454743875,-15.5,7.06512499999994));
#30226=CARTESIAN_POINT('Ctrl Pts',(13.8267841057906,-16.4660316469341,7.02345833333327));
#30227=CARTESIAN_POINT('Ctrl Pts',(14.3845227371938,-17.4320632938683,6.98179166666661));
#30228=CARTESIAN_POINT('Ctrl Pts',(15.5,-17.4320632938683,6.94012499999994));
#30229=CARTESIAN_POINT('Ctrl Pts',(16.6154772628062,-17.4320632938683,6.89845833333327));
#30230=CARTESIAN_POINT('Ctrl Pts',(17.1732158942094,-16.4660316469341,6.8567916666666));
#30231=CARTESIAN_POINT('Ctrl Pts',(17.7309545256125,-15.5,6.81512499999994));
#30232=CARTESIAN_POINT('Ctrl Pts',(17.1732158942094,-14.5339683530659,6.77345833333327));
#30233=CARTESIAN_POINT('Ctrl Pts',(16.6154772628062,-13.5679367061317,6.7317916666666));
#30234=CARTESIAN_POINT('Ctrl Pts',(15.5,-13.5679367061317,6.69012499999994));
#30235=CARTESIAN_POINT('Ctrl Pts',(14.3845227371938,-13.5679367061317,6.64845833333327));
#30236=CARTESIAN_POINT('Ctrl Pts',(13.8267841057906,-14.5339683530659,6.6067916666666));
#30237=CARTESIAN_POINT('Ctrl Pts',(13.2690454743875,-15.5,6.56512499999993));
#30238=CARTESIAN_POINT('Ctrl Pts',(13.8267841057906,-16.4660316469341,6.52345833333327));
#30239=CARTESIAN_POINT('Ctrl Pts',(14.3845227371938,-17.4320632938683,6.4817916666666));
#30240=CARTESIAN_POINT('Ctrl Pts',(15.5,-17.4320632938683,6.44012499999993));
#30241=CARTESIAN_POINT('Ctrl Pts',(16.6154772628062,-17.4320632938683,6.39845833333327));
#30242=CARTESIAN_POINT('Ctrl Pts',(17.1732158942094,-16.4660316469341,6.3567916666666));
#30243=CARTESIAN_POINT('Ctrl Pts',(17.7309545256125,-15.5,6.31512499999993));
#30244=CARTESIAN_POINT('Ctrl Pts',(17.1732158942094,-14.5339683530659,6.27345833333326));
#30245=CARTESIAN_POINT('Ctrl Pts',(16.6154772628062,-13.5679367061317,6.2317916666666));
#30246=CARTESIAN_POINT('Ctrl Pts',(15.5,-13.5679367061317,6.19012499999993));
#30247=CARTESIAN_POINT('Ctrl Pts',(14.3845227371938,-13.5679367061317,6.14845833333326));
#30248=CARTESIAN_POINT('Ctrl Pts',(13.8267841057906,-14.5339683530659,6.10679166666659));
#30249=CARTESIAN_POINT('Ctrl Pts',(13.2690454743875,-15.5,6.06512499999993));
#30250=CARTESIAN_POINT('Ctrl Pts',(13.8267841057906,-16.4660316469341,6.02345833333326));
#30251=CARTESIAN_POINT('Ctrl Pts',(14.3845227371938,-17.4320632938683,5.98179166666659));
#30252=CARTESIAN_POINT('Ctrl Pts',(15.5,-17.4320632938683,5.94012499999993));
#30253=CARTESIAN_POINT('Ctrl Pts',(16.6154772628062,-17.4320632938683,5.89845833333326));
#30254=CARTESIAN_POINT('Ctrl Pts',(17.1732158942094,-16.4660316469341,5.85679166666659));
#30255=CARTESIAN_POINT('Ctrl Pts',(17.7309545256125,-15.5,5.81512499999992));
#30256=CARTESIAN_POINT('Ctrl Pts',(17.1732158942094,-14.5339683530659,5.77345833333326));
#30257=CARTESIAN_POINT('Ctrl Pts',(16.6154772628062,-13.5679367061317,5.73179166666659));
#30258=CARTESIAN_POINT('Ctrl Pts',(15.5,-13.5679367061317,5.69012499999992));
#30259=CARTESIAN_POINT('Ctrl Pts',(14.3845227371938,-13.5679367061317,5.64845833333326));
#30260=CARTESIAN_POINT('Ctrl Pts',(13.8267841057906,-14.5339683530659,5.60679166666659));
#30261=CARTESIAN_POINT('Ctrl Pts',(13.2690454743875,-15.5,5.56512499999992));
#30262=CARTESIAN_POINT('Ctrl Pts',(13.8267841057906,-16.4660316469341,5.52345833333325));
#30263=CARTESIAN_POINT('Ctrl Pts',(14.3845227371938,-17.4320632938683,5.48179166666659));
#30264=CARTESIAN_POINT('Ctrl Pts',(15.5,-17.4320632938683,5.44012499999992));
#30265=CARTESIAN_POINT('Ctrl Pts',(16.6154772628062,-17.4320632938683,5.39845833333325));
#30266=CARTESIAN_POINT('Ctrl Pts',(17.1732158942094,-16.4660316469341,5.35679166666658));
#30267=CARTESIAN_POINT('Ctrl Pts',(17.7309545256125,-15.5,5.31512499999992));
#30268=CARTESIAN_POINT('Ctrl Pts',(17.1732158942094,-14.5339683530659,5.27345833333325));
#30269=CARTESIAN_POINT('Ctrl Pts',(16.6154772628062,-13.5679367061317,5.23179166666658));
#30270=CARTESIAN_POINT('Ctrl Pts',(15.5,-13.5679367061317,5.19012499999992));
#30271=CARTESIAN_POINT('Ctrl Pts',(14.3845227371938,-13.5679367061317,5.14845833333325));
#30272=CARTESIAN_POINT('Ctrl Pts',(13.8267841057906,-14.5339683530659,5.10679166666658));
#30273=CARTESIAN_POINT('Ctrl Pts',(13.2690454743875,-15.5,5.06512499999991));
#30274=CARTESIAN_POINT('Ctrl Pts',(13.8267841057906,-16.4660316469341,5.02345833333325));
#30275=CARTESIAN_POINT('Ctrl Pts',(14.3845227371938,-17.4320632938683,4.98179166666658));
#30276=CARTESIAN_POINT('Ctrl Pts',(15.5,-17.4320632938683,4.94012499999991));
#30277=CARTESIAN_POINT('Ctrl Pts',(16.6154772628062,-17.4320632938683,4.89845833333325));
#30278=CARTESIAN_POINT('Ctrl Pts',(17.1732158942094,-16.4660316469341,4.85679166666658));
#30279=CARTESIAN_POINT('Ctrl Pts',(17.7309545256125,-15.5,4.81512499999991));
#30280=CARTESIAN_POINT('Ctrl Pts',(17.1732158942094,-14.5339683530659,4.77345833333324));
#30281=CARTESIAN_POINT('Ctrl Pts',(16.6154772628062,-13.5679367061317,4.73179166666658));
#30282=CARTESIAN_POINT('Ctrl Pts',(15.5,-13.5679367061317,4.69012499999991));
#30283=CARTESIAN_POINT('Ctrl Pts',(14.3845227371938,-13.5679367061317,4.64845833333324));
#30284=CARTESIAN_POINT('Ctrl Pts',(13.8267841057906,-14.5339683530659,4.60679166666657));
#30285=CARTESIAN_POINT('Ctrl Pts',(13.2690454743875,-15.5,4.56512499999991));
#30286=CARTESIAN_POINT('Ctrl Pts',(13.8267841057906,-16.4660316469341,4.52345833333324));
#30287=CARTESIAN_POINT('Ctrl Pts',(14.3845227371938,-17.4320632938683,4.48179166666657));
#30288=CARTESIAN_POINT('Ctrl Pts',(15.5,-17.4320632938683,4.44012499999991));
#30289=CARTESIAN_POINT('Ctrl Pts',(16.6154772628062,-17.4320632938683,4.39845833333324));
#30290=CARTESIAN_POINT('Ctrl Pts',(17.1732158942094,-16.4660316469341,4.35679166666657));
#30291=CARTESIAN_POINT('Ctrl Pts',(17.7309545256125,-15.5,4.31512499999991));
#30292=CARTESIAN_POINT('Ctrl Pts',(17.1732158942094,-14.5339683530659,4.27345833333324));
#30293=CARTESIAN_POINT('Ctrl Pts',(16.6154772628062,-13.5679367061317,4.23179166666657));
#30294=CARTESIAN_POINT('Ctrl Pts',(15.5,-13.5679367061317,4.1901249999999));
#30295=CARTESIAN_POINT('Ctrl Pts',(14.3845227371938,-13.5679367061317,4.14845833333324));
#30296=CARTESIAN_POINT('Ctrl Pts',(13.8267841057906,-14.5339683530659,4.10679166666657));
#30297=CARTESIAN_POINT('Ctrl Pts',(13.2690454743875,-15.5,4.0651249999999));
#30298=CARTESIAN_POINT('Ctrl Pts',(13.8267841057906,-16.4660316469341,4.02345833333323));
#30299=CARTESIAN_POINT('Ctrl Pts',(14.3845227371938,-17.4320632938683,3.98179166666657));
#30300=CARTESIAN_POINT('Ctrl Pts',(15.5,-17.4320632938683,3.9401249999999));
#30301=CARTESIAN_POINT('Ctrl Pts',(16.6154772628062,-17.4320632938683,3.89845833333323));
#30302=CARTESIAN_POINT('Ctrl Pts',(17.1732158942094,-16.4660316469341,3.85679166666657));
#30303=CARTESIAN_POINT('Ctrl Pts',(17.7309545256125,-15.5,3.8151249999999));
#30304=CARTESIAN_POINT('Ctrl Pts',(17.1732158942094,-14.5339683530659,3.77345833333323));
#30305=CARTESIAN_POINT('Ctrl Pts',(16.6154772628062,-13.5679367061317,3.73179166666656));
#30306=CARTESIAN_POINT('Ctrl Pts',(15.5,-13.5679367061317,3.6901249999999));
#30307=CARTESIAN_POINT('Ctrl Pts',(14.3845227371938,-13.5679367061317,3.64845833333323));
#30308=CARTESIAN_POINT('Ctrl Pts',(13.8267841057906,-14.5339683530659,3.60679166666656));
#30309=CARTESIAN_POINT('Ctrl Pts',(13.2690454743875,-15.5,3.5651249999999));
#30310=CARTESIAN_POINT('Ctrl Pts',(13.8267841057906,-16.4660316469341,3.52345833333323));
#30311=CARTESIAN_POINT('Ctrl Pts',(14.3845227371938,-17.4320632938683,3.48179166666656));
#30312=CARTESIAN_POINT('Ctrl Pts',(15.5,-17.4320632938683,3.44012499999989));
#30313=CARTESIAN_POINT('Ctrl Pts',(16.6154772628062,-17.4320632938683,3.39845833333323));
#30314=CARTESIAN_POINT('Ctrl Pts',(17.1732158942094,-16.4660316469341,3.35679166666656));
#30315=CARTESIAN_POINT('Ctrl Pts',(17.7309545256125,-15.5,3.31512499999989));
#30316=CARTESIAN_POINT('Ctrl Pts',(17.1732158942094,-14.5339683530659,3.27345833333322));
#30317=CARTESIAN_POINT('Ctrl Pts',(16.6154772628062,-13.5679367061317,3.23179166666656));
#30318=CARTESIAN_POINT('Ctrl Pts',(15.5,-13.5679367061317,3.19012499999989));
#30319=CARTESIAN_POINT('Ctrl Pts',(14.3845227371938,-13.5679367061317,3.14845833333322));
#30320=CARTESIAN_POINT('Ctrl Pts',(13.8267841057906,-14.5339683530659,3.10679166666655));
#30321=CARTESIAN_POINT('Ctrl Pts',(13.2690454743875,-15.5,3.06512499999989));
#30322=CARTESIAN_POINT('Ctrl Pts',(13.8267841057906,-16.4660316469341,3.02345833333322));
#30323=CARTESIAN_POINT('Ctrl Pts',(14.3845227371938,-17.4320632938683,2.98179166666655));
#30324=CARTESIAN_POINT('Ctrl Pts',(15.5,-17.4320632938683,2.94012499999989));
#30325=CARTESIAN_POINT('Ctrl Pts',(16.6154772628062,-17.4320632938683,2.89845833333322));
#30326=CARTESIAN_POINT('Ctrl Pts',(17.1732158942094,-16.4660316469341,2.85679166666655));
#30327=CARTESIAN_POINT('Ctrl Pts',(17.7309545256125,-15.5,2.81512499999988));
#30328=CARTESIAN_POINT('Ctrl Pts',(17.1732158942094,-14.5339683530659,2.77345833333322));
#30329=CARTESIAN_POINT('Ctrl Pts',(16.6154772628062,-13.5679367061317,2.73179166666655));
#30330=CARTESIAN_POINT('Ctrl Pts',(15.5,-13.5679367061317,2.69012499999988));
#30331=CARTESIAN_POINT('Ctrl Pts',(14.3845227371938,-13.5679367061317,2.64845833333321));
#30332=CARTESIAN_POINT('Ctrl Pts',(13.8267841057906,-14.5339683530659,2.60679166666655));
#30333=CARTESIAN_POINT('Ctrl Pts',(13.2690454743875,-15.5,2.56512499999988));
#30334=CARTESIAN_POINT('Ctrl Pts',(13.8267841057906,-16.4660316469341,2.52345833333321));
#30335=CARTESIAN_POINT('Ctrl Pts',(14.3845227371938,-17.4320632938683,2.48179166666655));
#30336=CARTESIAN_POINT('Ctrl Pts',(15.5,-17.4320632938683,2.44012499999988));
#30337=CARTESIAN_POINT('Ctrl Pts',(16.6154772628062,-17.4320632938683,2.39845833333321));
#30338=CARTESIAN_POINT('Ctrl Pts',(17.1732158942094,-16.4660316469341,2.35679166666655));
#30339=CARTESIAN_POINT('Ctrl Pts',(17.7309545256125,-15.5,2.31512499999988));
#30340=CARTESIAN_POINT('Ctrl Pts',(17.1732158942094,-14.5339683530659,2.27345833333321));
#30341=CARTESIAN_POINT('Ctrl Pts',(16.6154772628062,-13.5679367061317,2.23179166666654));
#30342=CARTESIAN_POINT('Ctrl Pts',(15.5,-13.5679367061317,2.19012499999988));
#30343=CARTESIAN_POINT('Ctrl Pts',(14.3845227371938,-13.5679367061317,2.14845833333321));
#30344=CARTESIAN_POINT('Ctrl Pts',(13.8267841057906,-14.5339683530659,2.10679166666654));
#30345=CARTESIAN_POINT('Ctrl Pts',(13.2690454743875,-15.5,2.06512499999987));
#30346=CARTESIAN_POINT('Ctrl Pts',(13.8267841057906,-16.4660316469341,2.02345833333321));
#30347=CARTESIAN_POINT('Ctrl Pts',(14.3845227371938,-17.4320632938683,1.98179166666654));
#30348=CARTESIAN_POINT('Ctrl Pts',(15.5,-17.4320632938683,1.94012499999987));
#30349=CARTESIAN_POINT('Ctrl Pts',(16.6154772628062,-17.4320632938683,1.89845833333321));
#30350=CARTESIAN_POINT('Ctrl Pts',(17.1732158942094,-16.4660316469341,1.85679166666654));
#30351=CARTESIAN_POINT('Ctrl Pts',(17.7309545256125,-15.5,1.81512499999987));
#30352=CARTESIAN_POINT('Ctrl Pts',(17.1732158942094,-14.5339683530659,1.7734583333332));
#30353=CARTESIAN_POINT('Ctrl Pts',(16.6154772628062,-13.5679367061317,1.73179166666654));
#30354=CARTESIAN_POINT('Ctrl Pts',(15.5,-13.5679367061317,1.69012499999987));
#30355=CARTESIAN_POINT('Ctrl Pts',(14.3845227371938,-13.5679367061317,1.6484583333332));
#30356=CARTESIAN_POINT('Ctrl Pts',(13.8267841057906,-14.5339683530659,1.60679166666653));
#30357=CARTESIAN_POINT('Ctrl Pts',(13.2690454743875,-15.5,1.56512499999987));
#30358=CARTESIAN_POINT('Ctrl Pts',(13.8267841057906,-16.4660316469341,1.5234583333332));
#30359=CARTESIAN_POINT('Ctrl Pts',(14.3845227371938,-17.4320632938683,1.48179166666653));
#30360=CARTESIAN_POINT('Ctrl Pts',(15.5,-17.4320632938683,1.44012499999987));
#30361=CARTESIAN_POINT('Ctrl Pts',(16.6154772628062,-17.4320632938683,1.3984583333332));
#30362=CARTESIAN_POINT('Ctrl Pts',(17.1732158942094,-16.4660316469341,1.35679166666653));
#30363=CARTESIAN_POINT('Ctrl Pts',(17.7309545256125,-15.5,1.31512499999987));
#30364=CARTESIAN_POINT('Ctrl Pts',(17.1732158942094,-14.5339683530659,1.2734583333332));
#30365=CARTESIAN_POINT('Ctrl Pts',(16.6154772628062,-13.5679367061317,1.23179166666653));
#30366=CARTESIAN_POINT('Ctrl Pts',(15.5,-13.5679367061317,1.19012499999986));
#30367=CARTESIAN_POINT('Ctrl Pts',(14.3845227371938,-13.5679367061317,1.1484583333332));
#30368=CARTESIAN_POINT('Ctrl Pts',(13.8267841057906,-14.5339683530659,1.10679166666653));
#30369=CARTESIAN_POINT('Ctrl Pts',(13.2690454743875,-15.5,1.06512499999986));
#30370=CARTESIAN_POINT('Ctrl Pts',(13.8267841057906,-16.4660316469341,1.02345833333319));
#30371=CARTESIAN_POINT('Ctrl Pts',(14.3845227371938,-17.4320632938683,0.981791666666527));
#30372=CARTESIAN_POINT('Ctrl Pts',(15.5,-17.4320632938683,0.94012499999986));
#30373=CARTESIAN_POINT('Ctrl Pts',(16.6154772628062,-17.4320632938683,0.898458333333192));
#30374=CARTESIAN_POINT('Ctrl Pts',(17.1732158942094,-16.4660316469341,0.856791666666525));
#30375=CARTESIAN_POINT('Ctrl Pts',(17.7309545256125,-15.5,0.815124999999858));
#30376=CARTESIAN_POINT('Ctrl Pts',(17.1732158942094,-14.5339683530659,0.77345833333319));
#30377=CARTESIAN_POINT('Ctrl Pts',(16.6154772628062,-13.5679367061317,0.731791666666523));
#30378=CARTESIAN_POINT('Ctrl Pts',(15.5,-13.5679367061317,0.690124999999856));
#30379=CARTESIAN_POINT('Ctrl Pts',(14.3845227371938,-13.5679367061317,0.648458333333188));
#30380=CARTESIAN_POINT('Ctrl Pts',(13.8267841057906,-14.5339683530659,0.606791666666521));
#30381=CARTESIAN_POINT('Ctrl Pts',(13.2690454743875,-15.5,0.565124999999854));
#30382=CARTESIAN_POINT('Ctrl Pts',(13.8267841057906,-16.4660316469341,0.523458333333187));
#30383=CARTESIAN_POINT('Ctrl Pts',(14.3845227371938,-17.4320632938683,0.481791666666519));
#30384=CARTESIAN_POINT('Ctrl Pts',(15.5,-17.4320632938683,0.440124999999852));
#30385=CARTESIAN_POINT('Ctrl Pts',(16.6154772628062,-17.4320632938683,0.398458333333185));
#30386=CARTESIAN_POINT('Ctrl Pts',(17.1732158942094,-16.4660316469341,0.356791666666518));
#30387=CARTESIAN_POINT('Ctrl Pts',(17.7309545256125,-15.5,0.31512499999985));
#30388=CARTESIAN_POINT('Ctrl Pts',(17.1732158942094,-14.5339683530659,0.273458333333183));
#30389=CARTESIAN_POINT('Ctrl Pts',(16.6154772628062,-13.5679367061317,0.231791666666516));
#30390=CARTESIAN_POINT('Ctrl Pts',(15.5,-13.5679367061317,0.190124999999848));
#30391=CARTESIAN_POINT('Ctrl Pts',(14.3845227371938,-13.5679367061317,0.148458333333183));
#30392=CARTESIAN_POINT('Ctrl Pts',(13.8267841057906,-14.5339683530659,0.106791666666516));
#30393=CARTESIAN_POINT('Ctrl Pts',(13.2690454743875,-15.5,0.0651249999998483));
#30394=CARTESIAN_POINT('Ctrl Pts',(13.8267841057906,-16.4660316469341,0.023458333333181));
#30395=CARTESIAN_POINT('Ctrl Pts',(14.3845227371938,-17.4320632938683,-0.0182083333334863));
#30396=CARTESIAN_POINT('Ctrl Pts',(15.5,-17.4320632938683,-0.0598750000001536));
#30397=CARTESIAN_POINT('Ctrl Pts',(16.6154772628062,-17.4320632938683,-0.101541666666821));
#30398=CARTESIAN_POINT('Ctrl Pts',(17.1732158942094,-16.4660316469341,-0.143208333333488));
#30399=CARTESIAN_POINT('Ctrl Pts',(17.7309545256125,-15.5,-0.184875000000155));
#30400=CARTESIAN_POINT('Ctrl Pts',(17.1732158942094,-14.5339683530659,-0.226541666666823));
#30401=CARTESIAN_POINT('Ctrl Pts',(16.6154772628062,-13.5679367061317,-0.26820833333349));
#30402=CARTESIAN_POINT('Ctrl Pts',(15.5,-13.5679367061317,-0.309875000000157));
#30403=CARTESIAN_POINT('Ctrl Pts',(14.3845227371938,-13.5679367061317,-0.351541666666825));
#30404=CARTESIAN_POINT('Ctrl Pts',(13.8267841057906,-14.5339683530659,-0.393208333333492));
#30405=CARTESIAN_POINT('Ctrl Pts',(13.2690454743875,-15.5,-0.434875000000159));
#30406=CARTESIAN_POINT('Ctrl Pts',(13.8267841057906,-16.4660316469341,-0.476541666666826));
#30407=CARTESIAN_POINT('Ctrl Pts',(14.3845227371938,-17.4320632938683,-0.518208333333494));
#30408=CARTESIAN_POINT('Ctrl Pts',(15.5,-17.4320632938683,-0.559875000000161));
#30409=CARTESIAN_POINT('Ctrl Pts',(16.6154772628062,-17.4320632938683,-0.601541666666828));
#30410=CARTESIAN_POINT('Ctrl Pts',(17.1732158942094,-16.4660316469341,-0.643208333333495));
#30411=CARTESIAN_POINT('Ctrl Pts',(17.7309545256125,-15.5,-0.684875000000163));
#30412=CARTESIAN_POINT('Ctrl Pts',(17.1732158942094,-14.5339683530659,-0.72654166666683));
#30413=CARTESIAN_POINT('Ctrl Pts',(16.6154772628062,-13.5679367061317,-0.768208333333497));
#30414=CARTESIAN_POINT('Ctrl Pts',(15.5,-13.5679367061317,-0.809875000000165));
#30415=CARTESIAN_POINT('Ctrl Pts',(14.3845227371938,-13.5679367061317,-0.851541666666832));
#30416=CARTESIAN_POINT('Ctrl Pts',(13.8267841057906,-14.5339683530659,-0.893208333333499));
#30417=CARTESIAN_POINT('Ctrl Pts',(13.2690454743875,-15.5,-0.934875000000167));
#30418=CARTESIAN_POINT('Ctrl Pts',(13.8267841057906,-16.4660316469341,-0.976541666666834));
#30419=CARTESIAN_POINT('Ctrl Pts',(14.3845227371938,-17.4320632938683,-1.0182083333335));
#30420=CARTESIAN_POINT('Ctrl Pts',(15.5,-17.4320632938683,-1.05987500000017));
#30421=CARTESIAN_POINT('Ctrl Pts',(16.6154772628062,-17.4320632938683,-1.10154166666683));
#30422=CARTESIAN_POINT('Ctrl Pts',(17.1732158942094,-16.4660316469341,-1.1432083333335));
#30423=CARTESIAN_POINT('Ctrl Pts',(17.7309545256125,-15.5,-1.18487500000017));
#30424=CARTESIAN_POINT('Ctrl Pts',(17.1732158942094,-14.5339683530659,-1.22654166666684));
#30425=CARTESIAN_POINT('Ctrl Pts',(16.6154772628062,-13.5679367061317,-1.2682083333335));
#30426=CARTESIAN_POINT('Ctrl Pts',(15.5,-13.5679367061317,-1.30987500000017));
#30427=CARTESIAN_POINT('Ctrl Pts',(14.3845227371938,-13.5679367061317,-1.35154166666684));
#30428=CARTESIAN_POINT('Ctrl Pts',(13.8267841057906,-14.5339683530659,-1.3932083333335));
#30429=CARTESIAN_POINT('Ctrl Pts',(13.2690454743875,-15.5,-1.43487500000017));
#30430=CARTESIAN_POINT('Ctrl Pts',(13.8267841057906,-16.4660316469341,-1.47654166666684));
#30431=CARTESIAN_POINT('Ctrl Pts',(14.3845227371938,-17.4320632938683,-1.51820833333351));
#30432=CARTESIAN_POINT('Ctrl Pts',(15.5,-17.4320632938683,-1.55987500000017));
#30433=CARTESIAN_POINT('Ctrl Pts',(16.6154772628062,-17.4320632938683,-1.60154166666684));
#30434=CARTESIAN_POINT('Ctrl Pts',(17.1732158942094,-16.4660316469341,-1.64320833333351));
#30435=CARTESIAN_POINT('Ctrl Pts',(17.7309545256125,-15.5,-1.68487500000018));
#30436=CARTESIAN_POINT('Ctrl Pts',(17.1732158942094,-14.5339683530659,-1.72654166666684));
#30437=CARTESIAN_POINT('Ctrl Pts',(16.9678753992805,-14.1783081829978,-1.74188192368624));
#30438=CARTESIAN_POINT('Ctrl Pts',(16.6356255246375,-13.9369186715641,-1.75949830599533));
#30439=CARTESIAN_POINT('Ctrl Pts',(15.5,-17.080235786987,11.2369972941938));
#30440=CARTESIAN_POINT('Ctrl Pts',(16.412349557,-17.080235786987,11.1953306275271));
#30441=CARTESIAN_POINT('Ctrl Pts',(16.8685243355001,-16.2901178934935,11.1536639608605));
#30442=CARTESIAN_POINT('Ctrl Pts',(17.3246991140001,-15.5,11.1119972941938));
#30443=CARTESIAN_POINT('Ctrl Pts',(16.8685243355001,-14.7098821065065,11.0703306275271));
#30444=CARTESIAN_POINT('Ctrl Pts',(16.412349557,-13.919764213013,11.0286639608605));
#30445=CARTESIAN_POINT('Ctrl Pts',(15.5,-13.919764213013,10.9869972941938));
#30446=CARTESIAN_POINT('Ctrl Pts',(14.587650443,-13.919764213013,10.9453306275271));
#30447=CARTESIAN_POINT('Ctrl Pts',(14.1314756644999,-14.7098821065065,10.9036639608605));
#30448=CARTESIAN_POINT('Ctrl Pts',(13.6753008859999,-15.5,10.8619972941938));
#30449=CARTESIAN_POINT('Ctrl Pts',(14.1314756644999,-16.2901178934935,10.8203306275271));
#30450=CARTESIAN_POINT('Ctrl Pts',(14.587650443,-17.080235786987,10.7786639608605));
#30451=CARTESIAN_POINT('Ctrl Pts',(15.5,-17.080235786987,10.7369972941938));
#30452=CARTESIAN_POINT('Ctrl Pts',(16.412349557,-17.080235786987,10.6953306275271));
#30453=CARTESIAN_POINT('Ctrl Pts',(16.8685243355001,-16.2901178934935,10.6536639608605));
#30454=CARTESIAN_POINT('Ctrl Pts',(17.3246991140001,-15.5,10.6119972941938));
#30455=CARTESIAN_POINT('Ctrl Pts',(16.8685243355001,-14.7098821065065,10.5703306275271));
#30456=CARTESIAN_POINT('Ctrl Pts',(16.412349557,-13.919764213013,10.5286639608605));
#30457=CARTESIAN_POINT('Ctrl Pts',(15.5,-13.919764213013,10.4869972941938));
#30458=CARTESIAN_POINT('Ctrl Pts',(14.587650443,-13.919764213013,10.4453306275271));
#30459=CARTESIAN_POINT('Ctrl Pts',(14.1314756644999,-14.7098821065065,10.4036639608605));
#30460=CARTESIAN_POINT('Ctrl Pts',(13.6753008859999,-15.5,10.3619972941938));
#30461=CARTESIAN_POINT('Ctrl Pts',(14.1314756644999,-16.2901178934935,10.3203306275271));
#30462=CARTESIAN_POINT('Ctrl Pts',(14.587650443,-17.080235786987,10.2786639608605));
#30463=CARTESIAN_POINT('Ctrl Pts',(15.5,-17.080235786987,10.2369972941938));
#30464=CARTESIAN_POINT('Ctrl Pts',(16.412349557,-17.080235786987,10.1953306275271));
#30465=CARTESIAN_POINT('Ctrl Pts',(16.8685243355001,-16.2901178934935,10.1536639608605));
#30466=CARTESIAN_POINT('Ctrl Pts',(17.3246991140001,-15.5,10.1119972941938));
#30467=CARTESIAN_POINT('Ctrl Pts',(16.8685243355001,-14.7098821065065,10.0703306275271));
#30468=CARTESIAN_POINT('Ctrl Pts',(16.412349557,-13.919764213013,10.0286639608605));
#30469=CARTESIAN_POINT('Ctrl Pts',(15.5,-13.919764213013,9.98699729419378));
#30470=CARTESIAN_POINT('Ctrl Pts',(14.587650443,-13.919764213013,9.94533062752712));
#30471=CARTESIAN_POINT('Ctrl Pts',(14.1314756644999,-14.7098821065065,9.90366396086045));
#30472=CARTESIAN_POINT('Ctrl Pts',(13.6753008859999,-15.5,9.86199729419378));
#30473=CARTESIAN_POINT('Ctrl Pts',(14.1314756644999,-16.2901178934935,9.82033062752711));
#30474=CARTESIAN_POINT('Ctrl Pts',(14.587650443,-17.080235786987,9.77866396086045));
#30475=CARTESIAN_POINT('Ctrl Pts',(15.5,-17.080235786987,9.73699729419378));
#30476=CARTESIAN_POINT('Ctrl Pts',(16.412349557,-17.080235786987,9.69533062752711));
#30477=CARTESIAN_POINT('Ctrl Pts',(16.8685243355001,-16.2901178934935,9.65366396086044));
#30478=CARTESIAN_POINT('Ctrl Pts',(17.3246991140001,-15.5,9.61199729419378));
#30479=CARTESIAN_POINT('Ctrl Pts',(16.8685243355001,-14.7098821065065,9.57033062752711));
#30480=CARTESIAN_POINT('Ctrl Pts',(16.412349557,-13.919764213013,9.52866396086044));
#30481=CARTESIAN_POINT('Ctrl Pts',(15.5,-13.919764213013,9.48699729419378));
#30482=CARTESIAN_POINT('Ctrl Pts',(14.587650443,-13.919764213013,9.44533062752711));
#30483=CARTESIAN_POINT('Ctrl Pts',(14.1314756644999,-14.7098821065065,9.40366396086044));
#30484=CARTESIAN_POINT('Ctrl Pts',(13.6753008859999,-15.5,9.36199729419377));
#30485=CARTESIAN_POINT('Ctrl Pts',(14.1314756644999,-16.2901178934935,9.32033062752711));
#30486=CARTESIAN_POINT('Ctrl Pts',(14.587650443,-17.080235786987,9.27866396086044));
#30487=CARTESIAN_POINT('Ctrl Pts',(15.5,-17.080235786987,9.23699729419377));
#30488=CARTESIAN_POINT('Ctrl Pts',(16.412349557,-17.080235786987,9.19533062752711));
#30489=CARTESIAN_POINT('Ctrl Pts',(16.8685243355001,-16.2901178934935,9.15366396086044));
#30490=CARTESIAN_POINT('Ctrl Pts',(17.3246991140001,-15.5,9.11199729419377));
#30491=CARTESIAN_POINT('Ctrl Pts',(16.8685243355001,-14.7098821065065,9.0703306275271));
#30492=CARTESIAN_POINT('Ctrl Pts',(16.412349557,-13.919764213013,9.02866396086044));
#30493=CARTESIAN_POINT('Ctrl Pts',(15.5,-13.919764213013,8.98699729419377));
#30494=CARTESIAN_POINT('Ctrl Pts',(14.587650443,-13.919764213013,8.9453306275271));
#30495=CARTESIAN_POINT('Ctrl Pts',(14.1314756644999,-14.7098821065065,8.90366396086044));
#30496=CARTESIAN_POINT('Ctrl Pts',(13.6753008859999,-15.5,8.86199729419377));
#30497=CARTESIAN_POINT('Ctrl Pts',(14.1314756644999,-16.2901178934935,8.8203306275271));
#30498=CARTESIAN_POINT('Ctrl Pts',(14.587650443,-17.080235786987,8.77866396086043));
#30499=CARTESIAN_POINT('Ctrl Pts',(15.5,-17.080235786987,8.73699729419377));
#30500=CARTESIAN_POINT('Ctrl Pts',(16.412349557,-17.080235786987,8.6953306275271));
#30501=CARTESIAN_POINT('Ctrl Pts',(16.8685243355001,-16.2901178934935,8.65366396086043));
#30502=CARTESIAN_POINT('Ctrl Pts',(17.3246991140001,-15.5,8.61199729419376));
#30503=CARTESIAN_POINT('Ctrl Pts',(16.8685243355001,-14.7098821065065,8.57033062752709));
#30504=CARTESIAN_POINT('Ctrl Pts',(16.412349557,-13.919764213013,8.52866396086043));
#30505=CARTESIAN_POINT('Ctrl Pts',(15.5,-13.919764213013,8.48699729419376));
#30506=CARTESIAN_POINT('Ctrl Pts',(14.587650443,-13.919764213013,8.44533062752709));
#30507=CARTESIAN_POINT('Ctrl Pts',(14.1314756644999,-14.7098821065065,8.40366396086043));
#30508=CARTESIAN_POINT('Ctrl Pts',(13.6753008859999,-15.5,8.36199729419376));
#30509=CARTESIAN_POINT('Ctrl Pts',(14.1314756644999,-16.2901178934935,8.32033062752709));
#30510=CARTESIAN_POINT('Ctrl Pts',(14.587650443,-17.080235786987,8.27866396086043));
#30511=CARTESIAN_POINT('Ctrl Pts',(15.5,-17.080235786987,8.23699729419376));
#30512=CARTESIAN_POINT('Ctrl Pts',(16.412349557,-17.080235786987,8.19533062752709));
#30513=CARTESIAN_POINT('Ctrl Pts',(16.8685243355001,-16.2901178934935,8.15366396086043));
#30514=CARTESIAN_POINT('Ctrl Pts',(17.3246991140001,-15.5,8.11199729419376));
#30515=CARTESIAN_POINT('Ctrl Pts',(16.8685243355001,-14.7098821065065,8.07033062752709));
#30516=CARTESIAN_POINT('Ctrl Pts',(16.412349557,-13.919764213013,8.02866396086042));
#30517=CARTESIAN_POINT('Ctrl Pts',(15.5,-13.919764213013,7.98699729419376));
#30518=CARTESIAN_POINT('Ctrl Pts',(14.587650443,-13.919764213013,7.94533062752709));
#30519=CARTESIAN_POINT('Ctrl Pts',(14.1314756644999,-14.7098821065065,7.90366396086042));
#30520=CARTESIAN_POINT('Ctrl Pts',(13.6753008859999,-15.5,7.86199729419375));
#30521=CARTESIAN_POINT('Ctrl Pts',(14.1314756644999,-16.2901178934935,7.82033062752709));
#30522=CARTESIAN_POINT('Ctrl Pts',(14.587650443,-17.080235786987,7.77866396086042));
#30523=CARTESIAN_POINT('Ctrl Pts',(15.5,-17.080235786987,7.73699729419375));
#30524=CARTESIAN_POINT('Ctrl Pts',(16.412349557,-17.080235786987,7.69533062752709));
#30525=CARTESIAN_POINT('Ctrl Pts',(16.8685243355001,-16.2901178934935,7.65366396086042));
#30526=CARTESIAN_POINT('Ctrl Pts',(17.3246991140001,-15.5,7.61199729419375));
#30527=CARTESIAN_POINT('Ctrl Pts',(16.8685243355001,-14.7098821065065,7.57033062752708));
#30528=CARTESIAN_POINT('Ctrl Pts',(16.412349557,-13.919764213013,7.52866396086041));
#30529=CARTESIAN_POINT('Ctrl Pts',(15.5,-13.919764213013,7.48699729419375));
#30530=CARTESIAN_POINT('Ctrl Pts',(14.587650443,-13.919764213013,7.44533062752708));
#30531=CARTESIAN_POINT('Ctrl Pts',(14.1314756644999,-14.7098821065065,7.40366396086041));
#30532=CARTESIAN_POINT('Ctrl Pts',(13.6753008859999,-15.5,7.36199729419375));
#30533=CARTESIAN_POINT('Ctrl Pts',(14.1314756644999,-16.2901178934935,7.32033062752708));
#30534=CARTESIAN_POINT('Ctrl Pts',(14.587650443,-17.080235786987,7.27866396086041));
#30535=CARTESIAN_POINT('Ctrl Pts',(15.5,-17.080235786987,7.23699729419375));
#30536=CARTESIAN_POINT('Ctrl Pts',(16.412349557,-17.080235786987,7.19533062752708));
#30537=CARTESIAN_POINT('Ctrl Pts',(16.8685243355001,-16.2901178934935,7.15366396086041));
#30538=CARTESIAN_POINT('Ctrl Pts',(17.3246991140001,-15.5,7.11199729419374));
#30539=CARTESIAN_POINT('Ctrl Pts',(16.8685243355001,-14.7098821065065,7.07033062752708));
#30540=CARTESIAN_POINT('Ctrl Pts',(16.412349557,-13.919764213013,7.02866396086041));
#30541=CARTESIAN_POINT('Ctrl Pts',(15.5,-13.919764213013,6.98699729419374));
#30542=CARTESIAN_POINT('Ctrl Pts',(14.587650443,-13.919764213013,6.94533062752707));
#30543=CARTESIAN_POINT('Ctrl Pts',(14.1314756644999,-14.7098821065065,6.90366396086041));
#30544=CARTESIAN_POINT('Ctrl Pts',(13.6753008859999,-15.5,6.86199729419374));
#30545=CARTESIAN_POINT('Ctrl Pts',(14.1314756644999,-16.2901178934935,6.82033062752707));
#30546=CARTESIAN_POINT('Ctrl Pts',(14.587650443,-17.080235786987,6.77866396086041));
#30547=CARTESIAN_POINT('Ctrl Pts',(15.5,-17.080235786987,6.73699729419374));
#30548=CARTESIAN_POINT('Ctrl Pts',(16.412349557,-17.080235786987,6.69533062752707));
#30549=CARTESIAN_POINT('Ctrl Pts',(16.8685243355001,-16.2901178934935,6.65366396086041));
#30550=CARTESIAN_POINT('Ctrl Pts',(17.3246991140001,-15.5,6.61199729419374));
#30551=CARTESIAN_POINT('Ctrl Pts',(16.8685243355001,-14.7098821065065,6.57033062752707));
#30552=CARTESIAN_POINT('Ctrl Pts',(16.412349557,-13.919764213013,6.5286639608604));
#30553=CARTESIAN_POINT('Ctrl Pts',(15.5,-13.919764213013,6.48699729419374));
#30554=CARTESIAN_POINT('Ctrl Pts',(14.587650443,-13.919764213013,6.44533062752707));
#30555=CARTESIAN_POINT('Ctrl Pts',(14.1314756644999,-14.7098821065065,6.4036639608604));
#30556=CARTESIAN_POINT('Ctrl Pts',(13.6753008859999,-15.5,6.36199729419373));
#30557=CARTESIAN_POINT('Ctrl Pts',(14.1314756644999,-16.2901178934935,6.32033062752707));
#30558=CARTESIAN_POINT('Ctrl Pts',(14.587650443,-17.080235786987,6.2786639608604));
#30559=CARTESIAN_POINT('Ctrl Pts',(15.5,-17.080235786987,6.23699729419373));
#30560=CARTESIAN_POINT('Ctrl Pts',(16.412349557,-17.080235786987,6.19533062752706));
#30561=CARTESIAN_POINT('Ctrl Pts',(16.8685243355001,-16.2901178934935,6.1536639608604));
#30562=CARTESIAN_POINT('Ctrl Pts',(17.3246991140001,-15.5,6.11199729419373));
#30563=CARTESIAN_POINT('Ctrl Pts',(16.8685243355001,-14.7098821065065,6.07033062752706));
#30564=CARTESIAN_POINT('Ctrl Pts',(16.412349557,-13.919764213013,6.0286639608604));
#30565=CARTESIAN_POINT('Ctrl Pts',(15.5,-13.919764213013,5.98699729419373));
#30566=CARTESIAN_POINT('Ctrl Pts',(14.587650443,-13.919764213013,5.94533062752706));
#30567=CARTESIAN_POINT('Ctrl Pts',(14.1314756644999,-14.7098821065065,5.9036639608604));
#30568=CARTESIAN_POINT('Ctrl Pts',(13.6753008859999,-15.5,5.86199729419373));
#30569=CARTESIAN_POINT('Ctrl Pts',(14.1314756644999,-16.2901178934935,5.82033062752706));
#30570=CARTESIAN_POINT('Ctrl Pts',(14.587650443,-17.080235786987,5.77866396086039));
#30571=CARTESIAN_POINT('Ctrl Pts',(15.5,-17.080235786987,5.73699729419373));
#30572=CARTESIAN_POINT('Ctrl Pts',(16.412349557,-17.080235786987,5.69533062752706));
#30573=CARTESIAN_POINT('Ctrl Pts',(16.8685243355001,-16.2901178934935,5.65366396086039));
#30574=CARTESIAN_POINT('Ctrl Pts',(17.3246991140001,-15.5,5.61199729419372));
#30575=CARTESIAN_POINT('Ctrl Pts',(16.8685243355001,-14.7098821065065,5.57033062752706));
#30576=CARTESIAN_POINT('Ctrl Pts',(16.412349557,-13.919764213013,5.52866396086039));
#30577=CARTESIAN_POINT('Ctrl Pts',(15.5,-13.919764213013,5.48699729419372));
#30578=CARTESIAN_POINT('Ctrl Pts',(14.587650443,-13.919764213013,5.44533062752706));
#30579=CARTESIAN_POINT('Ctrl Pts',(14.1314756644999,-14.7098821065065,5.40366396086039));
#30580=CARTESIAN_POINT('Ctrl Pts',(13.6753008859999,-15.5,5.36199729419372));
#30581=CARTESIAN_POINT('Ctrl Pts',(14.1314756644999,-16.2901178934935,5.32033062752705));
#30582=CARTESIAN_POINT('Ctrl Pts',(14.587650443,-17.080235786987,5.27866396086039));
#30583=CARTESIAN_POINT('Ctrl Pts',(15.5,-17.080235786987,5.23699729419372));
#30584=CARTESIAN_POINT('Ctrl Pts',(16.412349557,-17.080235786987,5.19533062752705));
#30585=CARTESIAN_POINT('Ctrl Pts',(16.8685243355001,-16.2901178934935,5.15366396086038));
#30586=CARTESIAN_POINT('Ctrl Pts',(17.3246991140001,-15.5,5.11199729419372));
#30587=CARTESIAN_POINT('Ctrl Pts',(16.8685243355001,-14.7098821065065,5.07033062752705));
#30588=CARTESIAN_POINT('Ctrl Pts',(16.412349557,-13.919764213013,5.02866396086038));
#30589=CARTESIAN_POINT('Ctrl Pts',(15.5,-13.919764213013,4.98699729419372));
#30590=CARTESIAN_POINT('Ctrl Pts',(14.587650443,-13.919764213013,4.94533062752705));
#30591=CARTESIAN_POINT('Ctrl Pts',(14.1314756644999,-14.7098821065065,4.90366396086038));
#30592=CARTESIAN_POINT('Ctrl Pts',(13.6753008859999,-15.5,4.86199729419371));
#30593=CARTESIAN_POINT('Ctrl Pts',(14.1314756644999,-16.2901178934935,4.82033062752705));
#30594=CARTESIAN_POINT('Ctrl Pts',(14.587650443,-17.080235786987,4.77866396086038));
#30595=CARTESIAN_POINT('Ctrl Pts',(15.5,-17.080235786987,4.73699729419371));
#30596=CARTESIAN_POINT('Ctrl Pts',(16.412349557,-17.080235786987,4.69533062752705));
#30597=CARTESIAN_POINT('Ctrl Pts',(16.8685243355001,-16.2901178934935,4.65366396086038));
#30598=CARTESIAN_POINT('Ctrl Pts',(17.3246991140001,-15.5,4.61199729419371));
#30599=CARTESIAN_POINT('Ctrl Pts',(16.8685243355001,-14.7098821065065,4.57033062752704));
#30600=CARTESIAN_POINT('Ctrl Pts',(16.412349557,-13.919764213013,4.52866396086038));
#30601=CARTESIAN_POINT('Ctrl Pts',(15.5,-13.919764213013,4.48699729419371));
#30602=CARTESIAN_POINT('Ctrl Pts',(14.587650443,-13.919764213013,4.44533062752704));
#30603=CARTESIAN_POINT('Ctrl Pts',(14.1314756644999,-14.7098821065065,4.40366396086038));
#30604=CARTESIAN_POINT('Ctrl Pts',(13.6753008859999,-15.5,4.36199729419371));
#30605=CARTESIAN_POINT('Ctrl Pts',(14.1314756644999,-16.2901178934935,4.32033062752704));
#30606=CARTESIAN_POINT('Ctrl Pts',(14.587650443,-17.080235786987,4.27866396086037));
#30607=CARTESIAN_POINT('Ctrl Pts',(15.5,-17.080235786987,4.23699729419371));
#30608=CARTESIAN_POINT('Ctrl Pts',(16.412349557,-17.080235786987,4.19533062752704));
#30609=CARTESIAN_POINT('Ctrl Pts',(16.8685243355001,-16.2901178934935,4.15366396086037));
#30610=CARTESIAN_POINT('Ctrl Pts',(17.3246991140001,-15.5,4.1119972941937));
#30611=CARTESIAN_POINT('Ctrl Pts',(16.8685243355001,-14.7098821065065,4.07033062752704));
#30612=CARTESIAN_POINT('Ctrl Pts',(16.412349557,-13.919764213013,4.02866396086037));
#30613=CARTESIAN_POINT('Ctrl Pts',(15.5,-13.919764213013,3.9869972941937));
#30614=CARTESIAN_POINT('Ctrl Pts',(14.587650443,-13.919764213013,3.94533062752703));
#30615=CARTESIAN_POINT('Ctrl Pts',(14.1314756644999,-14.7098821065065,3.90366396086037));
#30616=CARTESIAN_POINT('Ctrl Pts',(13.6753008859999,-15.5,3.8619972941937));
#30617=CARTESIAN_POINT('Ctrl Pts',(14.1314756644999,-16.2901178934935,3.82033062752703));
#30618=CARTESIAN_POINT('Ctrl Pts',(14.587650443,-17.080235786987,3.77866396086037));
#30619=CARTESIAN_POINT('Ctrl Pts',(15.5,-17.080235786987,3.7369972941937));
#30620=CARTESIAN_POINT('Ctrl Pts',(16.412349557,-17.080235786987,3.69533062752703));
#30621=CARTESIAN_POINT('Ctrl Pts',(16.8685243355001,-16.2901178934935,3.65366396086036));
#30622=CARTESIAN_POINT('Ctrl Pts',(17.3246991140001,-15.5,3.6119972941937));
#30623=CARTESIAN_POINT('Ctrl Pts',(16.8685243355001,-14.7098821065065,3.57033062752703));
#30624=CARTESIAN_POINT('Ctrl Pts',(16.412349557,-13.919764213013,3.52866396086036));
#30625=CARTESIAN_POINT('Ctrl Pts',(15.5,-13.919764213013,3.4869972941937));
#30626=CARTESIAN_POINT('Ctrl Pts',(14.587650443,-13.919764213013,3.44533062752703));
#30627=CARTESIAN_POINT('Ctrl Pts',(14.1314756644999,-14.7098821065065,3.40366396086036));
#30628=CARTESIAN_POINT('Ctrl Pts',(13.6753008859999,-15.5,3.36199729419369));
#30629=CARTESIAN_POINT('Ctrl Pts',(14.1314756644999,-16.2901178934935,3.32033062752703));
#30630=CARTESIAN_POINT('Ctrl Pts',(14.587650443,-17.080235786987,3.27866396086036));
#30631=CARTESIAN_POINT('Ctrl Pts',(15.5,-17.080235786987,3.23699729419369));
#30632=CARTESIAN_POINT('Ctrl Pts',(16.412349557,-17.080235786987,3.19533062752703));
#30633=CARTESIAN_POINT('Ctrl Pts',(16.8685243355001,-16.2901178934935,3.15366396086036));
#30634=CARTESIAN_POINT('Ctrl Pts',(17.3246991140001,-15.5,3.11199729419369));
#30635=CARTESIAN_POINT('Ctrl Pts',(16.8685243355001,-14.7098821065065,3.07033062752702));
#30636=CARTESIAN_POINT('Ctrl Pts',(16.412349557,-13.919764213013,3.02866396086036));
#30637=CARTESIAN_POINT('Ctrl Pts',(15.5,-13.919764213013,2.98699729419369));
#30638=CARTESIAN_POINT('Ctrl Pts',(14.587650443,-13.919764213013,2.94533062752702));
#30639=CARTESIAN_POINT('Ctrl Pts',(14.1314756644999,-14.7098821065065,2.90366396086036));
#30640=CARTESIAN_POINT('Ctrl Pts',(13.6753008859999,-15.5,2.86199729419369));
#30641=CARTESIAN_POINT('Ctrl Pts',(14.1314756644999,-16.2901178934935,2.82033062752702));
#30642=CARTESIAN_POINT('Ctrl Pts',(14.587650443,-17.080235786987,2.77866396086035));
#30643=CARTESIAN_POINT('Ctrl Pts',(15.5,-17.080235786987,2.73699729419369));
#30644=CARTESIAN_POINT('Ctrl Pts',(16.412349557,-17.080235786987,2.69533062752702));
#30645=CARTESIAN_POINT('Ctrl Pts',(16.8685243355001,-16.2901178934935,2.65366396086035));
#30646=CARTESIAN_POINT('Ctrl Pts',(17.3246991140001,-15.5,2.61199729419368));
#30647=CARTESIAN_POINT('Ctrl Pts',(16.8685243355001,-14.7098821065065,2.57033062752702));
#30648=CARTESIAN_POINT('Ctrl Pts',(16.412349557,-13.919764213013,2.52866396086035));
#30649=CARTESIAN_POINT('Ctrl Pts',(15.5,-13.919764213013,2.48699729419368));
#30650=CARTESIAN_POINT('Ctrl Pts',(14.587650443,-13.919764213013,2.44533062752701));
#30651=CARTESIAN_POINT('Ctrl Pts',(14.1314756644999,-14.7098821065065,2.40366396086035));
#30652=CARTESIAN_POINT('Ctrl Pts',(13.6753008859999,-15.5,2.36199729419368));
#30653=CARTESIAN_POINT('Ctrl Pts',(14.1314756644999,-16.2901178934935,2.32033062752701));
#30654=CARTESIAN_POINT('Ctrl Pts',(14.587650443,-17.080235786987,2.27866396086035));
#30655=CARTESIAN_POINT('Ctrl Pts',(15.5,-17.080235786987,2.23699729419368));
#30656=CARTESIAN_POINT('Ctrl Pts',(16.412349557,-17.080235786987,2.19533062752701));
#30657=CARTESIAN_POINT('Ctrl Pts',(16.8685243355001,-16.2901178934935,2.15366396086035));
#30658=CARTESIAN_POINT('Ctrl Pts',(17.3246991140001,-15.5,2.11199729419368));
#30659=CARTESIAN_POINT('Ctrl Pts',(16.8685243355001,-14.7098821065065,2.07033062752701));
#30660=CARTESIAN_POINT('Ctrl Pts',(16.412349557,-13.919764213013,2.02866396086034));
#30661=CARTESIAN_POINT('Ctrl Pts',(15.5,-13.919764213013,1.98699729419368));
#30662=CARTESIAN_POINT('Ctrl Pts',(14.587650443,-13.919764213013,1.94533062752701));
#30663=CARTESIAN_POINT('Ctrl Pts',(14.1314756644999,-14.7098821065065,1.90366396086034));
#30664=CARTESIAN_POINT('Ctrl Pts',(13.6753008859999,-15.5,1.86199729419367));
#30665=CARTESIAN_POINT('Ctrl Pts',(14.1314756644999,-16.2901178934935,1.82033062752701));
#30666=CARTESIAN_POINT('Ctrl Pts',(14.587650443,-17.080235786987,1.77866396086034));
#30667=CARTESIAN_POINT('Ctrl Pts',(15.5,-17.080235786987,1.73699729419367));
#30668=CARTESIAN_POINT('Ctrl Pts',(16.412349557,-17.080235786987,1.695330627527));
#30669=CARTESIAN_POINT('Ctrl Pts',(16.8685243355001,-16.2901178934935,1.65366396086034));
#30670=CARTESIAN_POINT('Ctrl Pts',(17.3246991140001,-15.5,1.61199729419367));
#30671=CARTESIAN_POINT('Ctrl Pts',(16.8685243355001,-14.7098821065065,1.570330627527));
#30672=CARTESIAN_POINT('Ctrl Pts',(16.412349557,-13.919764213013,1.52866396086034));
#30673=CARTESIAN_POINT('Ctrl Pts',(15.5,-13.919764213013,1.48699729419367));
#30674=CARTESIAN_POINT('Ctrl Pts',(14.587650443,-13.919764213013,1.445330627527));
#30675=CARTESIAN_POINT('Ctrl Pts',(14.1314756644999,-14.7098821065065,1.40366396086033));
#30676=CARTESIAN_POINT('Ctrl Pts',(13.6753008859999,-15.5,1.36199729419367));
#30677=CARTESIAN_POINT('Ctrl Pts',(14.1314756644999,-16.2901178934935,1.320330627527));
#30678=CARTESIAN_POINT('Ctrl Pts',(14.587650443,-17.080235786987,1.27866396086033));
#30679=CARTESIAN_POINT('Ctrl Pts',(15.5,-17.080235786987,1.23699729419367));
#30680=CARTESIAN_POINT('Ctrl Pts',(16.412349557,-17.080235786987,1.195330627527));
#30681=CARTESIAN_POINT('Ctrl Pts',(16.8685243355001,-16.2901178934935,1.15366396086033));
#30682=CARTESIAN_POINT('Ctrl Pts',(17.3246991140001,-15.5,1.11199729419366));
#30683=CARTESIAN_POINT('Ctrl Pts',(16.8685243355001,-14.7098821065065,1.070330627527));
#30684=CARTESIAN_POINT('Ctrl Pts',(16.412349557,-13.919764213013,1.02866396086033));
#30685=CARTESIAN_POINT('Ctrl Pts',(15.5,-13.919764213013,0.986997294193663));
#30686=CARTESIAN_POINT('Ctrl Pts',(14.587650443,-13.919764213013,0.945330627526996));
#30687=CARTESIAN_POINT('Ctrl Pts',(14.1314756644999,-14.7098821065065,0.903663960860329));
#30688=CARTESIAN_POINT('Ctrl Pts',(13.6753008859999,-15.5,0.861997294193661));
#30689=CARTESIAN_POINT('Ctrl Pts',(14.1314756644999,-16.2901178934935,0.820330627526994));
#30690=CARTESIAN_POINT('Ctrl Pts',(14.587650443,-17.080235786987,0.778663960860328));
#30691=CARTESIAN_POINT('Ctrl Pts',(15.5,-17.080235786987,0.736997294193659));
#30692=CARTESIAN_POINT('Ctrl Pts',(16.412349557,-17.080235786987,0.695330627526992));
#30693=CARTESIAN_POINT('Ctrl Pts',(16.8685243355001,-16.2901178934935,0.653663960860325));
#30694=CARTESIAN_POINT('Ctrl Pts',(17.3246991140001,-15.5,0.611997294193657));
#30695=CARTESIAN_POINT('Ctrl Pts',(16.8685243355001,-14.7098821065065,0.57033062752699));
#30696=CARTESIAN_POINT('Ctrl Pts',(16.412349557,-13.919764213013,0.528663960860323));
#30697=CARTESIAN_POINT('Ctrl Pts',(15.5,-13.919764213013,0.486997294193656));
#30698=CARTESIAN_POINT('Ctrl Pts',(14.587650443,-13.919764213013,0.445330627526988));
#30699=CARTESIAN_POINT('Ctrl Pts',(14.1314756644999,-14.7098821065065,0.403663960860321));
#30700=CARTESIAN_POINT('Ctrl Pts',(13.6753008859999,-15.5,0.361997294193654));
#30701=CARTESIAN_POINT('Ctrl Pts',(14.1314756644999,-16.2901178934935,0.320330627526986));
#30702=CARTESIAN_POINT('Ctrl Pts',(14.587650443,-17.080235786987,0.278663960860319));
#30703=CARTESIAN_POINT('Ctrl Pts',(15.5,-17.080235786987,0.236997294193652));
#30704=CARTESIAN_POINT('Ctrl Pts',(16.412349557,-17.080235786987,0.195330627526985));
#30705=CARTESIAN_POINT('Ctrl Pts',(16.8685243355001,-16.2901178934935,0.153663960860317));
#30706=CARTESIAN_POINT('Ctrl Pts',(17.3246991140001,-15.5,0.11199729419365));
#30707=CARTESIAN_POINT('Ctrl Pts',(16.8685243355001,-14.7098821065065,0.0703306275269832));
#30708=CARTESIAN_POINT('Ctrl Pts',(16.412349557,-13.919764213013,0.0286639608603159));
#30709=CARTESIAN_POINT('Ctrl Pts',(15.5,-13.919764213013,-0.0130027058063514));
#30710=CARTESIAN_POINT('Ctrl Pts',(14.587650443,-13.919764213013,-0.0546693724730169));
#30711=CARTESIAN_POINT('Ctrl Pts',(14.1314756644999,-14.7098821065065,-0.0963360391396842));
#30712=CARTESIAN_POINT('Ctrl Pts',(13.6753008859999,-15.5,-0.138002705806352));
#30713=CARTESIAN_POINT('Ctrl Pts',(14.1314756644999,-16.2901178934935,-0.179669372473019));
#30714=CARTESIAN_POINT('Ctrl Pts',(14.587650443,-17.080235786987,-0.221336039139686));
#30715=CARTESIAN_POINT('Ctrl Pts',(15.5,-17.080235786987,-0.263002705806354));
#30716=CARTESIAN_POINT('Ctrl Pts',(16.412349557,-17.080235786987,-0.304669372473021));
#30717=CARTESIAN_POINT('Ctrl Pts',(16.8685243355001,-16.2901178934935,-0.346336039139688));
#30718=CARTESIAN_POINT('Ctrl Pts',(17.3246991140001,-15.5,-0.388002705806356));
#30719=CARTESIAN_POINT('Ctrl Pts',(16.8685243355001,-14.7098821065065,-0.429669372473023));
#30720=CARTESIAN_POINT('Ctrl Pts',(16.412349557,-13.919764213013,-0.47133603913969));
#30721=CARTESIAN_POINT('Ctrl Pts',(15.5,-13.919764213013,-0.513002705806357));
#30722=CARTESIAN_POINT('Ctrl Pts',(14.587650443,-13.919764213013,-0.554669372473025));
#30723=CARTESIAN_POINT('Ctrl Pts',(14.1314756644999,-14.7098821065065,-0.596336039139692));
#30724=CARTESIAN_POINT('Ctrl Pts',(13.6753008859999,-15.5,-0.638002705806359));
#30725=CARTESIAN_POINT('Ctrl Pts',(14.1314756644999,-16.2901178934935,-0.679669372473027));
#30726=CARTESIAN_POINT('Ctrl Pts',(14.587650443,-17.080235786987,-0.721336039139694));
#30727=CARTESIAN_POINT('Ctrl Pts',(15.5,-17.080235786987,-0.763002705806361));
#30728=CARTESIAN_POINT('Ctrl Pts',(16.412349557,-17.080235786987,-0.804669372473029));
#30729=CARTESIAN_POINT('Ctrl Pts',(16.8685243355001,-16.2901178934935,-0.846336039139696));
#30730=CARTESIAN_POINT('Ctrl Pts',(17.3246991140001,-15.5,-0.888002705806363));
#30731=CARTESIAN_POINT('Ctrl Pts',(16.8685243355001,-14.7098821065065,-0.92966937247303));
#30732=CARTESIAN_POINT('Ctrl Pts',(16.412349557,-13.919764213013,-0.971336039139697));
#30733=CARTESIAN_POINT('Ctrl Pts',(15.5,-13.919764213013,-1.01300270580636));
#30734=CARTESIAN_POINT('Ctrl Pts',(14.587650443,-13.919764213013,-1.05466937247303));
#30735=CARTESIAN_POINT('Ctrl Pts',(14.1314756644999,-14.7098821065065,-1.0963360391397));
#30736=CARTESIAN_POINT('Ctrl Pts',(13.6753008859999,-15.5,-1.13800270580637));
#30737=CARTESIAN_POINT('Ctrl Pts',(14.1314756644999,-16.2901178934935,-1.17966937247303));
#30738=CARTESIAN_POINT('Ctrl Pts',(14.587650443,-17.080235786987,-1.2213360391397));
#30739=CARTESIAN_POINT('Ctrl Pts',(15.5,-17.080235786987,-1.26300270580637));
#30740=CARTESIAN_POINT('Ctrl Pts',(16.412349557,-17.080235786987,-1.30466937247303));
#30741=CARTESIAN_POINT('Ctrl Pts',(16.8685243355001,-16.2901178934935,-1.3463360391397));
#30742=CARTESIAN_POINT('Ctrl Pts',(17.3246991140001,-15.5,-1.38800270580637));
#30743=CARTESIAN_POINT('Ctrl Pts',(16.8685243355001,-14.7098821065065,-1.42966937247304));
#30744=CARTESIAN_POINT('Ctrl Pts',(16.412349557,-13.919764213013,-1.4713360391397));
#30745=CARTESIAN_POINT('Ctrl Pts',(15.5,-13.919764213013,-1.51300270580637));
#30746=CARTESIAN_POINT('Ctrl Pts',(14.587650443,-13.919764213013,-1.55466937247304));
#30747=CARTESIAN_POINT('Ctrl Pts',(14.1314756644999,-14.7098821065065,-1.59633603913971));
#30748=CARTESIAN_POINT('Ctrl Pts',(13.6753008859999,-15.5,-1.63800270580637));
#30749=CARTESIAN_POINT('Ctrl Pts',(14.1314756644999,-16.2901178934935,-1.67966937247304));
#30750=CARTESIAN_POINT('Ctrl Pts',(14.587650443,-17.080235786987,-1.72133603913971));
#30751=CARTESIAN_POINT('Ctrl Pts',(15.5,-17.080235786987,-1.76300270580637));
#30752=CARTESIAN_POINT('Ctrl Pts',(16.412349557,-17.080235786987,-1.80466937247304));
#30753=CARTESIAN_POINT('Ctrl Pts',(16.8685243355001,-16.2901178934935,-1.84633603913971));
#30754=CARTESIAN_POINT('Ctrl Pts',(17.3246991140001,-15.5,-1.88800270580638));
#30755=CARTESIAN_POINT('Ctrl Pts',(16.8685243355001,-14.7098821065065,-1.92966937247304));
#30756=CARTESIAN_POINT('Ctrl Pts',(16.7005762151491,-14.4189874290231,-1.94500962949244));
#30757=CARTESIAN_POINT('Ctrl Pts',(16.4288288330633,-14.2215547953296,-1.96262601180153));
#30758=CARTESIAN_POINT('',(16.4288315898516,-14.2215509627457,-1.96262324188451));
#30759=CARTESIAN_POINT('',(16.4288304039466,-14.2215500160357,-1.96262332703658));
#30760=CARTESIAN_POINT('Ctrl Pts',(14.2313898004749,-14.5577749122403,10.4122404735808));
#30761=CARTESIAN_POINT('Ctrl Pts',(14.1770441521709,-14.6309457974488,10.407829216981));
#30762=CARTESIAN_POINT('Ctrl Pts',(14.1314716057906,-14.7098797632096,10.4036666666667));
#30763=CARTESIAN_POINT('Ctrl Pts',(13.6752954743875,-15.5,10.362));
#30764=CARTESIAN_POINT('Ctrl Pts',(14.1314716057906,-16.2901202367904,10.3203333333333));
#30765=CARTESIAN_POINT('Ctrl Pts',(14.5876477371938,-17.0802404735808,10.2786666666667));
#30766=CARTESIAN_POINT('Ctrl Pts',(15.5,-17.0802404735808,10.237));
#30767=CARTESIAN_POINT('Ctrl Pts',(16.4123522628062,-17.0802404735808,10.1953333333333));
#30768=CARTESIAN_POINT('Ctrl Pts',(16.8685283942094,-16.2901202367904,10.1536666666667));
#30769=CARTESIAN_POINT('Ctrl Pts',(17.3247045256125,-15.5,10.112));
#30770=CARTESIAN_POINT('Ctrl Pts',(16.8685283942094,-14.7098797632096,10.0703333333333));
#30771=CARTESIAN_POINT('Ctrl Pts',(16.4123522628062,-13.9197595264192,10.0286666666667));
#30772=CARTESIAN_POINT('Ctrl Pts',(15.5,-13.9197595264192,9.98699999999998));
#30773=CARTESIAN_POINT('Ctrl Pts',(14.5876477371938,-13.9197595264192,9.94533333333331));
#30774=CARTESIAN_POINT('Ctrl Pts',(14.1314716057906,-14.7098797632096,9.90366666666665));
#30775=CARTESIAN_POINT('Ctrl Pts',(13.6752954743875,-15.5,9.86199999999998));
#30776=CARTESIAN_POINT('Ctrl Pts',(14.1314716057906,-16.2901202367904,9.82033333333331));
#30777=CARTESIAN_POINT('Ctrl Pts',(14.5876477371938,-17.0802404735808,9.77866666666665));
#30778=CARTESIAN_POINT('Ctrl Pts',(15.5,-17.0802404735808,9.73699999999998));
#30779=CARTESIAN_POINT('Ctrl Pts',(16.4123522628062,-17.0802404735808,9.69533333333331));
#30780=CARTESIAN_POINT('Ctrl Pts',(16.8685283942094,-16.2901202367904,9.65366666666664));
#30781=CARTESIAN_POINT('Ctrl Pts',(17.3247045256125,-15.5,9.61199999999998));
#30782=CARTESIAN_POINT('Ctrl Pts',(16.8685283942094,-14.7098797632096,9.57033333333331));
#30783=CARTESIAN_POINT('Ctrl Pts',(16.4123522628062,-13.9197595264192,9.52866666666664));
#30784=CARTESIAN_POINT('Ctrl Pts',(15.5,-13.9197595264192,9.48699999999998));
#30785=CARTESIAN_POINT('Ctrl Pts',(14.5876477371938,-13.9197595264192,9.44533333333331));
#30786=CARTESIAN_POINT('Ctrl Pts',(14.1314716057906,-14.7098797632096,9.40366666666664));
#30787=CARTESIAN_POINT('Ctrl Pts',(13.6752954743875,-15.5,9.36199999999998));
#30788=CARTESIAN_POINT('Ctrl Pts',(14.1314716057906,-16.2901202367904,9.32033333333331));
#30789=CARTESIAN_POINT('Ctrl Pts',(14.5876477371938,-17.0802404735808,9.27866666666664));
#30790=CARTESIAN_POINT('Ctrl Pts',(15.5,-17.0802404735808,9.23699999999997));
#30791=CARTESIAN_POINT('Ctrl Pts',(16.4123522628062,-17.0802404735808,9.19533333333331));
#30792=CARTESIAN_POINT('Ctrl Pts',(16.8685283942094,-16.2901202367904,9.15366666666664));
#30793=CARTESIAN_POINT('Ctrl Pts',(17.3247045256125,-15.5,9.11199999999997));
#30794=CARTESIAN_POINT('Ctrl Pts',(16.8685283942094,-14.7098797632096,9.0703333333333));
#30795=CARTESIAN_POINT('Ctrl Pts',(16.4123522628062,-13.9197595264192,9.02866666666664));
#30796=CARTESIAN_POINT('Ctrl Pts',(15.5,-13.9197595264192,8.98699999999997));
#30797=CARTESIAN_POINT('Ctrl Pts',(14.5876477371938,-13.9197595264192,8.9453333333333));
#30798=CARTESIAN_POINT('Ctrl Pts',(14.1314716057906,-14.7098797632096,8.90366666666664));
#30799=CARTESIAN_POINT('Ctrl Pts',(13.6752954743875,-15.5,8.86199999999997));
#30800=CARTESIAN_POINT('Ctrl Pts',(14.1314716057906,-16.2901202367904,8.8203333333333));
#30801=CARTESIAN_POINT('Ctrl Pts',(14.5876477371938,-17.0802404735808,8.77866666666663));
#30802=CARTESIAN_POINT('Ctrl Pts',(15.5,-17.0802404735808,8.73699999999997));
#30803=CARTESIAN_POINT('Ctrl Pts',(16.4123522628062,-17.0802404735808,8.6953333333333));
#30804=CARTESIAN_POINT('Ctrl Pts',(16.8685283942094,-16.2901202367904,8.65366666666663));
#30805=CARTESIAN_POINT('Ctrl Pts',(17.3247045256125,-15.5,8.61199999999996));
#30806=CARTESIAN_POINT('Ctrl Pts',(16.8685283942094,-14.7098797632096,8.57033333333329));
#30807=CARTESIAN_POINT('Ctrl Pts',(16.4123522628062,-13.9197595264192,8.52866666666663));
#30808=CARTESIAN_POINT('Ctrl Pts',(15.5,-13.9197595264192,8.48699999999996));
#30809=CARTESIAN_POINT('Ctrl Pts',(14.5876477371938,-13.9197595264192,8.44533333333329));
#30810=CARTESIAN_POINT('Ctrl Pts',(14.1314716057906,-14.7098797632096,8.40366666666663));
#30811=CARTESIAN_POINT('Ctrl Pts',(13.6752954743875,-15.5,8.36199999999996));
#30812=CARTESIAN_POINT('Ctrl Pts',(14.1314716057906,-16.2901202367904,8.32033333333329));
#30813=CARTESIAN_POINT('Ctrl Pts',(14.5876477371938,-17.0802404735808,8.27866666666663));
#30814=CARTESIAN_POINT('Ctrl Pts',(15.5,-17.0802404735808,8.23699999999996));
#30815=CARTESIAN_POINT('Ctrl Pts',(16.4123522628062,-17.0802404735808,8.19533333333329));
#30816=CARTESIAN_POINT('Ctrl Pts',(16.8685283942094,-16.2901202367904,8.15366666666663));
#30817=CARTESIAN_POINT('Ctrl Pts',(17.3247045256125,-15.5,8.11199999999996));
#30818=CARTESIAN_POINT('Ctrl Pts',(16.8685283942094,-14.7098797632096,8.07033333333329));
#30819=CARTESIAN_POINT('Ctrl Pts',(16.4123522628062,-13.9197595264192,8.02866666666662));
#30820=CARTESIAN_POINT('Ctrl Pts',(15.5,-13.9197595264192,7.98699999999996));
#30821=CARTESIAN_POINT('Ctrl Pts',(14.5876477371938,-13.9197595264192,7.94533333333329));
#30822=CARTESIAN_POINT('Ctrl Pts',(14.1314716057906,-14.7098797632096,7.90366666666662));
#30823=CARTESIAN_POINT('Ctrl Pts',(13.6752954743875,-15.5,7.86199999999995));
#30824=CARTESIAN_POINT('Ctrl Pts',(14.1314716057906,-16.2901202367904,7.82033333333329));
#30825=CARTESIAN_POINT('Ctrl Pts',(14.5876477371938,-17.0802404735808,7.77866666666662));
#30826=CARTESIAN_POINT('Ctrl Pts',(15.5,-17.0802404735808,7.73699999999995));
#30827=CARTESIAN_POINT('Ctrl Pts',(16.4123522628062,-17.0802404735808,7.69533333333329));
#30828=CARTESIAN_POINT('Ctrl Pts',(16.8685283942094,-16.2901202367904,7.65366666666662));
#30829=CARTESIAN_POINT('Ctrl Pts',(17.3247045256125,-15.5,7.61199999999995));
#30830=CARTESIAN_POINT('Ctrl Pts',(16.8685283942094,-14.7098797632096,7.57033333333328));
#30831=CARTESIAN_POINT('Ctrl Pts',(16.4123522628062,-13.9197595264192,7.52866666666662));
#30832=CARTESIAN_POINT('Ctrl Pts',(15.5,-13.9197595264192,7.48699999999995));
#30833=CARTESIAN_POINT('Ctrl Pts',(14.5876477371938,-13.9197595264192,7.44533333333328));
#30834=CARTESIAN_POINT('Ctrl Pts',(14.1314716057906,-14.7098797632096,7.40366666666661));
#30835=CARTESIAN_POINT('Ctrl Pts',(13.6752954743875,-15.5,7.36199999999995));
#30836=CARTESIAN_POINT('Ctrl Pts',(14.1314716057906,-16.2901202367904,7.32033333333328));
#30837=CARTESIAN_POINT('Ctrl Pts',(14.5876477371938,-17.0802404735808,7.27866666666661));
#30838=CARTESIAN_POINT('Ctrl Pts',(15.5,-17.0802404735808,7.23699999999995));
#30839=CARTESIAN_POINT('Ctrl Pts',(16.4123522628062,-17.0802404735808,7.19533333333328));
#30840=CARTESIAN_POINT('Ctrl Pts',(16.8685283942094,-16.2901202367904,7.15366666666661));
#30841=CARTESIAN_POINT('Ctrl Pts',(17.3247045256125,-15.5,7.11199999999994));
#30842=CARTESIAN_POINT('Ctrl Pts',(16.8685283942094,-14.7098797632096,7.07033333333328));
#30843=CARTESIAN_POINT('Ctrl Pts',(16.4123522628062,-13.9197595264192,7.02866666666661));
#30844=CARTESIAN_POINT('Ctrl Pts',(15.5,-13.9197595264192,6.98699999999994));
#30845=CARTESIAN_POINT('Ctrl Pts',(14.5876477371938,-13.9197595264192,6.94533333333327));
#30846=CARTESIAN_POINT('Ctrl Pts',(14.1314716057906,-14.7098797632096,6.90366666666661));
#30847=CARTESIAN_POINT('Ctrl Pts',(13.6752954743875,-15.5,6.86199999999994));
#30848=CARTESIAN_POINT('Ctrl Pts',(14.1314716057906,-16.2901202367904,6.82033333333327));
#30849=CARTESIAN_POINT('Ctrl Pts',(14.5876477371938,-17.0802404735808,6.77866666666661));
#30850=CARTESIAN_POINT('Ctrl Pts',(15.5,-17.0802404735808,6.73699999999994));
#30851=CARTESIAN_POINT('Ctrl Pts',(16.4123522628062,-17.0802404735808,6.69533333333327));
#30852=CARTESIAN_POINT('Ctrl Pts',(16.8685283942094,-16.2901202367904,6.65366666666661));
#30853=CARTESIAN_POINT('Ctrl Pts',(17.3247045256125,-15.5,6.61199999999994));
#30854=CARTESIAN_POINT('Ctrl Pts',(16.8685283942094,-14.7098797632096,6.57033333333327));
#30855=CARTESIAN_POINT('Ctrl Pts',(16.4123522628062,-13.9197595264192,6.5286666666666));
#30856=CARTESIAN_POINT('Ctrl Pts',(15.5,-13.9197595264192,6.48699999999994));
#30857=CARTESIAN_POINT('Ctrl Pts',(14.5876477371938,-13.9197595264192,6.44533333333327));
#30858=CARTESIAN_POINT('Ctrl Pts',(14.1314716057906,-14.7098797632096,6.4036666666666));
#30859=CARTESIAN_POINT('Ctrl Pts',(13.6752954743875,-15.5,6.36199999999993));
#30860=CARTESIAN_POINT('Ctrl Pts',(14.1314716057906,-16.2901202367904,6.32033333333327));
#30861=CARTESIAN_POINT('Ctrl Pts',(14.5876477371938,-17.0802404735808,6.2786666666666));
#30862=CARTESIAN_POINT('Ctrl Pts',(15.5,-17.0802404735808,6.23699999999993));
#30863=CARTESIAN_POINT('Ctrl Pts',(16.4123522628062,-17.0802404735808,6.19533333333326));
#30864=CARTESIAN_POINT('Ctrl Pts',(16.8685283942094,-16.2901202367904,6.1536666666666));
#30865=CARTESIAN_POINT('Ctrl Pts',(17.3247045256125,-15.5,6.11199999999993));
#30866=CARTESIAN_POINT('Ctrl Pts',(16.8685283942094,-14.7098797632096,6.07033333333326));
#30867=CARTESIAN_POINT('Ctrl Pts',(16.4123522628062,-13.9197595264192,6.0286666666666));
#30868=CARTESIAN_POINT('Ctrl Pts',(15.5,-13.9197595264192,5.98699999999993));
#30869=CARTESIAN_POINT('Ctrl Pts',(14.5876477371938,-13.9197595264192,5.94533333333326));
#30870=CARTESIAN_POINT('Ctrl Pts',(14.1314716057906,-14.7098797632096,5.9036666666666));
#30871=CARTESIAN_POINT('Ctrl Pts',(13.6752954743875,-15.5,5.86199999999993));
#30872=CARTESIAN_POINT('Ctrl Pts',(14.1314716057906,-16.2901202367904,5.82033333333326));
#30873=CARTESIAN_POINT('Ctrl Pts',(14.5876477371938,-17.0802404735808,5.77866666666659));
#30874=CARTESIAN_POINT('Ctrl Pts',(15.5,-17.0802404735808,5.73699999999993));
#30875=CARTESIAN_POINT('Ctrl Pts',(16.4123522628062,-17.0802404735808,5.69533333333326));
#30876=CARTESIAN_POINT('Ctrl Pts',(16.8685283942094,-16.2901202367904,5.65366666666659));
#30877=CARTESIAN_POINT('Ctrl Pts',(17.3247045256125,-15.5,5.61199999999992));
#30878=CARTESIAN_POINT('Ctrl Pts',(16.8685283942094,-14.7098797632096,5.57033333333326));
#30879=CARTESIAN_POINT('Ctrl Pts',(16.4123522628062,-13.9197595264192,5.52866666666659));
#30880=CARTESIAN_POINT('Ctrl Pts',(15.5,-13.9197595264192,5.48699999999992));
#30881=CARTESIAN_POINT('Ctrl Pts',(14.5876477371938,-13.9197595264192,5.44533333333326));
#30882=CARTESIAN_POINT('Ctrl Pts',(14.1314716057906,-14.7098797632096,5.40366666666659));
#30883=CARTESIAN_POINT('Ctrl Pts',(13.6752954743875,-15.5,5.36199999999992));
#30884=CARTESIAN_POINT('Ctrl Pts',(14.1314716057906,-16.2901202367904,5.32033333333325));
#30885=CARTESIAN_POINT('Ctrl Pts',(14.5876477371938,-17.0802404735808,5.27866666666659));
#30886=CARTESIAN_POINT('Ctrl Pts',(15.5,-17.0802404735808,5.23699999999992));
#30887=CARTESIAN_POINT('Ctrl Pts',(16.4123522628062,-17.0802404735808,5.19533333333325));
#30888=CARTESIAN_POINT('Ctrl Pts',(16.8685283942094,-16.2901202367904,5.15366666666658));
#30889=CARTESIAN_POINT('Ctrl Pts',(17.3247045256125,-15.5,5.11199999999992));
#30890=CARTESIAN_POINT('Ctrl Pts',(16.8685283942094,-14.7098797632096,5.07033333333325));
#30891=CARTESIAN_POINT('Ctrl Pts',(16.4123522628062,-13.9197595264192,5.02866666666658));
#30892=CARTESIAN_POINT('Ctrl Pts',(15.5,-13.9197595264192,4.98699999999992));
#30893=CARTESIAN_POINT('Ctrl Pts',(14.5876477371938,-13.9197595264192,4.94533333333325));
#30894=CARTESIAN_POINT('Ctrl Pts',(14.1314716057906,-14.7098797632096,4.90366666666658));
#30895=CARTESIAN_POINT('Ctrl Pts',(13.6752954743875,-15.5,4.86199999999991));
#30896=CARTESIAN_POINT('Ctrl Pts',(14.1314716057906,-16.2901202367904,4.82033333333325));
#30897=CARTESIAN_POINT('Ctrl Pts',(14.5876477371938,-17.0802404735808,4.77866666666658));
#30898=CARTESIAN_POINT('Ctrl Pts',(15.5,-17.0802404735808,4.73699999999991));
#30899=CARTESIAN_POINT('Ctrl Pts',(16.4123522628062,-17.0802404735808,4.69533333333325));
#30900=CARTESIAN_POINT('Ctrl Pts',(16.8685283942094,-16.2901202367904,4.65366666666658));
#30901=CARTESIAN_POINT('Ctrl Pts',(17.3247045256125,-15.5,4.61199999999991));
#30902=CARTESIAN_POINT('Ctrl Pts',(16.8685283942094,-14.7098797632096,4.57033333333324));
#30903=CARTESIAN_POINT('Ctrl Pts',(16.4123522628062,-13.9197595264192,4.52866666666658));
#30904=CARTESIAN_POINT('Ctrl Pts',(15.5,-13.9197595264192,4.48699999999991));
#30905=CARTESIAN_POINT('Ctrl Pts',(14.5876477371938,-13.9197595264192,4.44533333333324));
#30906=CARTESIAN_POINT('Ctrl Pts',(14.1314716057906,-14.7098797632096,4.40366666666658));
#30907=CARTESIAN_POINT('Ctrl Pts',(13.6752954743875,-15.5,4.36199999999991));
#30908=CARTESIAN_POINT('Ctrl Pts',(14.1314716057906,-16.2901202367904,4.32033333333324));
#30909=CARTESIAN_POINT('Ctrl Pts',(14.5876477371938,-17.0802404735808,4.27866666666657));
#30910=CARTESIAN_POINT('Ctrl Pts',(15.5,-17.0802404735808,4.23699999999991));
#30911=CARTESIAN_POINT('Ctrl Pts',(16.4123522628062,-17.0802404735808,4.19533333333324));
#30912=CARTESIAN_POINT('Ctrl Pts',(16.8685283942094,-16.2901202367904,4.15366666666657));
#30913=CARTESIAN_POINT('Ctrl Pts',(17.3247045256125,-15.5,4.1119999999999));
#30914=CARTESIAN_POINT('Ctrl Pts',(16.8685283942094,-14.7098797632096,4.07033333333324));
#30915=CARTESIAN_POINT('Ctrl Pts',(16.4123522628062,-13.9197595264192,4.02866666666657));
#30916=CARTESIAN_POINT('Ctrl Pts',(15.5,-13.9197595264192,3.9869999999999));
#30917=CARTESIAN_POINT('Ctrl Pts',(14.5876477371938,-13.9197595264192,3.94533333333323));
#30918=CARTESIAN_POINT('Ctrl Pts',(14.1314716057906,-14.7098797632096,3.90366666666657));
#30919=CARTESIAN_POINT('Ctrl Pts',(13.6752954743875,-15.5,3.8619999999999));
#30920=CARTESIAN_POINT('Ctrl Pts',(14.1314716057906,-16.2901202367904,3.82033333333323));
#30921=CARTESIAN_POINT('Ctrl Pts',(14.5876477371938,-17.0802404735808,3.77866666666657));
#30922=CARTESIAN_POINT('Ctrl Pts',(15.5,-17.0802404735808,3.7369999999999));
#30923=CARTESIAN_POINT('Ctrl Pts',(16.4123522628062,-17.0802404735808,3.69533333333323));
#30924=CARTESIAN_POINT('Ctrl Pts',(16.8685283942094,-16.2901202367904,3.65366666666656));
#30925=CARTESIAN_POINT('Ctrl Pts',(17.3247045256125,-15.5,3.6119999999999));
#30926=CARTESIAN_POINT('Ctrl Pts',(16.8685283942094,-14.7098797632096,3.57033333333323));
#30927=CARTESIAN_POINT('Ctrl Pts',(16.4123522628062,-13.9197595264192,3.52866666666656));
#30928=CARTESIAN_POINT('Ctrl Pts',(15.5,-13.9197595264192,3.4869999999999));
#30929=CARTESIAN_POINT('Ctrl Pts',(14.5876477371938,-13.9197595264192,3.44533333333323));
#30930=CARTESIAN_POINT('Ctrl Pts',(14.1314716057906,-14.7098797632096,3.40366666666656));
#30931=CARTESIAN_POINT('Ctrl Pts',(13.6752954743875,-15.5,3.36199999999989));
#30932=CARTESIAN_POINT('Ctrl Pts',(14.1314716057906,-16.2901202367904,3.32033333333323));
#30933=CARTESIAN_POINT('Ctrl Pts',(14.5876477371938,-17.0802404735808,3.27866666666656));
#30934=CARTESIAN_POINT('Ctrl Pts',(15.5,-17.0802404735808,3.23699999999989));
#30935=CARTESIAN_POINT('Ctrl Pts',(16.4123522628062,-17.0802404735808,3.19533333333323));
#30936=CARTESIAN_POINT('Ctrl Pts',(16.8685283942094,-16.2901202367904,3.15366666666656));
#30937=CARTESIAN_POINT('Ctrl Pts',(17.3247045256125,-15.5,3.11199999999989));
#30938=CARTESIAN_POINT('Ctrl Pts',(16.8685283942094,-14.7098797632096,3.07033333333322));
#30939=CARTESIAN_POINT('Ctrl Pts',(16.4123522628062,-13.9197595264192,3.02866666666656));
#30940=CARTESIAN_POINT('Ctrl Pts',(15.5,-13.9197595264192,2.98699999999989));
#30941=CARTESIAN_POINT('Ctrl Pts',(14.5876477371938,-13.9197595264192,2.94533333333322));
#30942=CARTESIAN_POINT('Ctrl Pts',(14.1314716057906,-14.7098797632096,2.90366666666656));
#30943=CARTESIAN_POINT('Ctrl Pts',(13.6752954743875,-15.5,2.86199999999989));
#30944=CARTESIAN_POINT('Ctrl Pts',(14.1314716057906,-16.2901202367904,2.82033333333322));
#30945=CARTESIAN_POINT('Ctrl Pts',(14.5876477371938,-17.0802404735808,2.77866666666655));
#30946=CARTESIAN_POINT('Ctrl Pts',(15.5,-17.0802404735808,2.73699999999989));
#30947=CARTESIAN_POINT('Ctrl Pts',(16.4123522628062,-17.0802404735808,2.69533333333322));
#30948=CARTESIAN_POINT('Ctrl Pts',(16.8685283942094,-16.2901202367904,2.65366666666655));
#30949=CARTESIAN_POINT('Ctrl Pts',(17.3247045256125,-15.5,2.61199999999988));
#30950=CARTESIAN_POINT('Ctrl Pts',(16.8685283942094,-14.7098797632096,2.57033333333322));
#30951=CARTESIAN_POINT('Ctrl Pts',(16.4123522628062,-13.9197595264192,2.52866666666655));
#30952=CARTESIAN_POINT('Ctrl Pts',(15.5,-13.9197595264192,2.48699999999988));
#30953=CARTESIAN_POINT('Ctrl Pts',(14.5876477371938,-13.9197595264192,2.44533333333321));
#30954=CARTESIAN_POINT('Ctrl Pts',(14.1314716057906,-14.7098797632096,2.40366666666655));
#30955=CARTESIAN_POINT('Ctrl Pts',(13.6752954743875,-15.5,2.36199999999988));
#30956=CARTESIAN_POINT('Ctrl Pts',(14.1314716057906,-16.2901202367904,2.32033333333321));
#30957=CARTESIAN_POINT('Ctrl Pts',(14.5876477371938,-17.0802404735808,2.27866666666655));
#30958=CARTESIAN_POINT('Ctrl Pts',(15.5,-17.0802404735808,2.23699999999988));
#30959=CARTESIAN_POINT('Ctrl Pts',(16.4123522628062,-17.0802404735808,2.19533333333321));
#30960=CARTESIAN_POINT('Ctrl Pts',(16.8685283942094,-16.2901202367904,2.15366666666655));
#30961=CARTESIAN_POINT('Ctrl Pts',(17.3247045256125,-15.5,2.11199999999988));
#30962=CARTESIAN_POINT('Ctrl Pts',(16.8685283942094,-14.7098797632096,2.07033333333321));
#30963=CARTESIAN_POINT('Ctrl Pts',(16.4123522628062,-13.9197595264192,2.02866666666654));
#30964=CARTESIAN_POINT('Ctrl Pts',(15.5,-13.9197595264192,1.98699999999988));
#30965=CARTESIAN_POINT('Ctrl Pts',(14.5876477371938,-13.9197595264192,1.94533333333321));
#30966=CARTESIAN_POINT('Ctrl Pts',(14.1314716057906,-14.7098797632096,1.90366666666654));
#30967=CARTESIAN_POINT('Ctrl Pts',(13.6752954743875,-15.5,1.86199999999987));
#30968=CARTESIAN_POINT('Ctrl Pts',(14.1314716057906,-16.2901202367904,1.82033333333321));
#30969=CARTESIAN_POINT('Ctrl Pts',(14.5876477371938,-17.0802404735808,1.77866666666654));
#30970=CARTESIAN_POINT('Ctrl Pts',(15.5,-17.0802404735808,1.73699999999987));
#30971=CARTESIAN_POINT('Ctrl Pts',(16.4123522628062,-17.0802404735808,1.6953333333332));
#30972=CARTESIAN_POINT('Ctrl Pts',(16.8685283942094,-16.2901202367904,1.65366666666654));
#30973=CARTESIAN_POINT('Ctrl Pts',(17.3247045256125,-15.5,1.61199999999987));
#30974=CARTESIAN_POINT('Ctrl Pts',(16.8685283942094,-14.7098797632096,1.5703333333332));
#30975=CARTESIAN_POINT('Ctrl Pts',(16.4123522628062,-13.9197595264192,1.52866666666654));
#30976=CARTESIAN_POINT('Ctrl Pts',(15.5,-13.9197595264192,1.48699999999987));
#30977=CARTESIAN_POINT('Ctrl Pts',(14.5876477371938,-13.9197595264192,1.4453333333332));
#30978=CARTESIAN_POINT('Ctrl Pts',(14.1314716057906,-14.7098797632096,1.40366666666653));
#30979=CARTESIAN_POINT('Ctrl Pts',(13.6752954743875,-15.5,1.36199999999987));
#30980=CARTESIAN_POINT('Ctrl Pts',(14.1314716057906,-16.2901202367904,1.3203333333332));
#30981=CARTESIAN_POINT('Ctrl Pts',(14.5876477371938,-17.0802404735808,1.27866666666653));
#30982=CARTESIAN_POINT('Ctrl Pts',(15.5,-17.0802404735808,1.23699999999987));
#30983=CARTESIAN_POINT('Ctrl Pts',(16.4123522628062,-17.0802404735808,1.1953333333332));
#30984=CARTESIAN_POINT('Ctrl Pts',(16.8685283942094,-16.2901202367904,1.15366666666653));
#30985=CARTESIAN_POINT('Ctrl Pts',(17.3247045256125,-15.5,1.11199999999986));
#30986=CARTESIAN_POINT('Ctrl Pts',(16.8685283942094,-14.7098797632096,1.0703333333332));
#30987=CARTESIAN_POINT('Ctrl Pts',(16.4123522628062,-13.9197595264192,1.02866666666653));
#30988=CARTESIAN_POINT('Ctrl Pts',(15.5,-13.9197595264192,0.986999999999863));
#30989=CARTESIAN_POINT('Ctrl Pts',(14.5876477371938,-13.9197595264192,0.945333333333196));
#30990=CARTESIAN_POINT('Ctrl Pts',(14.1314716057906,-14.7098797632096,0.903666666666529));
#30991=CARTESIAN_POINT('Ctrl Pts',(13.6752954743875,-15.5,0.861999999999861));
#30992=CARTESIAN_POINT('Ctrl Pts',(14.1314716057906,-16.2901202367904,0.820333333333194));
#30993=CARTESIAN_POINT('Ctrl Pts',(14.5876477371938,-17.0802404735808,0.778666666666527));
#30994=CARTESIAN_POINT('Ctrl Pts',(15.5,-17.0802404735808,0.736999999999859));
#30995=CARTESIAN_POINT('Ctrl Pts',(16.4123522628062,-17.0802404735808,0.695333333333192));
#30996=CARTESIAN_POINT('Ctrl Pts',(16.8685283942094,-16.2901202367904,0.653666666666525));
#30997=CARTESIAN_POINT('Ctrl Pts',(17.3247045256125,-15.5,0.611999999999858));
#30998=CARTESIAN_POINT('Ctrl Pts',(16.8685283942094,-14.7098797632096,0.57033333333319));
#30999=CARTESIAN_POINT('Ctrl Pts',(16.4123522628062,-13.9197595264192,0.528666666666523));
#31000=CARTESIAN_POINT('Ctrl Pts',(15.5,-13.9197595264192,0.486999999999856));
#31001=CARTESIAN_POINT('Ctrl Pts',(14.5876477371938,-13.9197595264192,0.445333333333188));
#31002=CARTESIAN_POINT('Ctrl Pts',(14.1314716057906,-14.7098797632096,0.403666666666521));
#31003=CARTESIAN_POINT('Ctrl Pts',(13.6752954743875,-15.5,0.361999999999854));
#31004=CARTESIAN_POINT('Ctrl Pts',(14.1314716057906,-16.2901202367904,0.320333333333186));
#31005=CARTESIAN_POINT('Ctrl Pts',(14.5876477371938,-17.0802404735808,0.278666666666519));
#31006=CARTESIAN_POINT('Ctrl Pts',(15.5,-17.0802404735808,0.236999999999852));
#31007=CARTESIAN_POINT('Ctrl Pts',(16.4123522628062,-17.0802404735808,0.195333333333185));
#31008=CARTESIAN_POINT('Ctrl Pts',(16.8685283942094,-16.2901202367904,0.153666666666517));
#31009=CARTESIAN_POINT('Ctrl Pts',(17.3247045256125,-15.5,0.11199999999985));
#31010=CARTESIAN_POINT('Ctrl Pts',(16.8685283942094,-14.7098797632096,0.0703333333331828));
#31011=CARTESIAN_POINT('Ctrl Pts',(16.4123522628062,-13.9197595264192,0.0286666666665155));
#31012=CARTESIAN_POINT('Ctrl Pts',(15.5,-13.9197595264192,-0.0130000000001518));
#31013=CARTESIAN_POINT('Ctrl Pts',(14.5876477371938,-13.9197595264192,-0.0546666666668173));
#31014=CARTESIAN_POINT('Ctrl Pts',(14.1314716057906,-14.7098797632096,-0.0963333333334846));
#31015=CARTESIAN_POINT('Ctrl Pts',(13.6752954743875,-15.5,-0.138000000000152));
#31016=CARTESIAN_POINT('Ctrl Pts',(14.1314716057906,-16.2901202367904,-0.179666666666819));
#31017=CARTESIAN_POINT('Ctrl Pts',(14.5876477371938,-17.0802404735808,-0.221333333333486));
#31018=CARTESIAN_POINT('Ctrl Pts',(15.5,-17.0802404735808,-0.263000000000154));
#31019=CARTESIAN_POINT('Ctrl Pts',(16.4123522628062,-17.0802404735808,-0.304666666666821));
#31020=CARTESIAN_POINT('Ctrl Pts',(16.8685283942094,-16.2901202367904,-0.346333333333488));
#31021=CARTESIAN_POINT('Ctrl Pts',(17.3247045256125,-15.5,-0.388000000000156));
#31022=CARTESIAN_POINT('Ctrl Pts',(16.8685283942094,-14.7098797632096,-0.429666666666823));
#31023=CARTESIAN_POINT('Ctrl Pts',(16.4123522628062,-13.9197595264192,-0.47133333333349));
#31024=CARTESIAN_POINT('Ctrl Pts',(15.5,-13.9197595264192,-0.513000000000157));
#31025=CARTESIAN_POINT('Ctrl Pts',(14.5876477371938,-13.9197595264192,-0.554666666666825));
#31026=CARTESIAN_POINT('Ctrl Pts',(14.1314716057906,-14.7098797632096,-0.596333333333492));
#31027=CARTESIAN_POINT('Ctrl Pts',(13.6752954743875,-15.5,-0.638000000000159));
#31028=CARTESIAN_POINT('Ctrl Pts',(14.1314716057906,-16.2901202367904,-0.679666666666827));
#31029=CARTESIAN_POINT('Ctrl Pts',(14.5876477371938,-17.0802404735808,-0.721333333333494));
#31030=CARTESIAN_POINT('Ctrl Pts',(15.5,-17.0802404735808,-0.763000000000161));
#31031=CARTESIAN_POINT('Ctrl Pts',(16.4123522628062,-17.0802404735808,-0.804666666666829));
#31032=CARTESIAN_POINT('Ctrl Pts',(16.8685283942094,-16.2901202367904,-0.846333333333496));
#31033=CARTESIAN_POINT('Ctrl Pts',(17.3247045256125,-15.5,-0.888000000000163));
#31034=CARTESIAN_POINT('Ctrl Pts',(16.8685283942094,-14.7098797632096,-0.92966666666683));
#31035=CARTESIAN_POINT('Ctrl Pts',(16.4123522628062,-13.9197595264192,-0.971333333333498));
#31036=CARTESIAN_POINT('Ctrl Pts',(15.5,-13.9197595264192,-1.01300000000016));
#31037=CARTESIAN_POINT('Ctrl Pts',(14.5876477371938,-13.9197595264192,-1.05466666666683));
#31038=CARTESIAN_POINT('Ctrl Pts',(14.1314716057906,-14.7098797632096,-1.0963333333335));
#31039=CARTESIAN_POINT('Ctrl Pts',(13.6752954743875,-15.5,-1.13800000000017));
#31040=CARTESIAN_POINT('Ctrl Pts',(14.1314716057906,-16.2901202367904,-1.17966666666683));
#31041=CARTESIAN_POINT('Ctrl Pts',(14.5876477371938,-17.0802404735808,-1.2213333333335));
#31042=CARTESIAN_POINT('Ctrl Pts',(15.5,-17.0802404735808,-1.26300000000017));
#31043=CARTESIAN_POINT('Ctrl Pts',(16.4123522628062,-17.0802404735808,-1.30466666666683));
#31044=CARTESIAN_POINT('Ctrl Pts',(16.8685283942094,-16.2901202367904,-1.3463333333335));
#31045=CARTESIAN_POINT('Ctrl Pts',(17.3247045256125,-15.5,-1.38800000000017));
#31046=CARTESIAN_POINT('Ctrl Pts',(16.8685283942094,-14.7098797632096,-1.42966666666684));
#31047=CARTESIAN_POINT('Ctrl Pts',(16.4123522628062,-13.9197595264192,-1.4713333333335));
#31048=CARTESIAN_POINT('Ctrl Pts',(15.5,-13.9197595264192,-1.51300000000017));
#31049=CARTESIAN_POINT('Ctrl Pts',(14.5876477371938,-13.9197595264192,-1.55466666666684));
#31050=CARTESIAN_POINT('Ctrl Pts',(14.1314716057906,-14.7098797632096,-1.59633333333351));
#31051=CARTESIAN_POINT('Ctrl Pts',(13.6752954743875,-15.5,-1.63800000000017));
#31052=CARTESIAN_POINT('Ctrl Pts',(14.1314716057906,-16.2901202367904,-1.67966666666684));
#31053=CARTESIAN_POINT('Ctrl Pts',(14.5876477371938,-17.0802404735808,-1.72133333333351));
#31054=CARTESIAN_POINT('Ctrl Pts',(15.5,-17.0802404735808,-1.76300000000017));
#31055=CARTESIAN_POINT('Ctrl Pts',(16.4123522628062,-17.0802404735808,-1.80466666666684));
#31056=CARTESIAN_POINT('Ctrl Pts',(16.8685283942094,-16.2901202367904,-1.84633333333351));
#31057=CARTESIAN_POINT('Ctrl Pts',(17.3247045256125,-15.5,-1.88800000000018));
#31058=CARTESIAN_POINT('Ctrl Pts',(16.8685283942094,-14.7098797632096,-1.92966666666684));
#31059=CARTESIAN_POINT('Ctrl Pts',(16.700583153372,-14.4189900731899,-1.94500661517905));
#31060=CARTESIAN_POINT('Ctrl Pts',(16.4288340223699,-14.2215527726061,-1.96262314816781));
#31061=CARTESIAN_POINT('Origin',(16.5839252605846,-14.0080754615186,-2.17746715486548));
#31062=CARTESIAN_POINT('',(16.4288300625788,-14.2215498957104,-2.02512301642216));
#31063=CARTESIAN_POINT('Ctrl Pts',(15.5,-17.0802404735808,11.2370201234482));
#31064=CARTESIAN_POINT('Ctrl Pts',(16.4123522628062,-17.0802404735808,11.1953534567815));
#31065=CARTESIAN_POINT('Ctrl Pts',(16.8685283942094,-16.2901202367904,11.1536867901149));
#31066=CARTESIAN_POINT('Ctrl Pts',(17.3247045256125,-15.5,11.1120201234482));
#31067=CARTESIAN_POINT('Ctrl Pts',(16.8685283942094,-14.7098797632096,11.0703534567815));
#31068=CARTESIAN_POINT('Ctrl Pts',(16.4123522628062,-13.9197595264192,11.0286867901149));
#31069=CARTESIAN_POINT('Ctrl Pts',(15.5,-13.9197595264192,10.9870201234482));
#31070=CARTESIAN_POINT('Ctrl Pts',(14.5876477371938,-13.9197595264192,10.9453534567815));
#31071=CARTESIAN_POINT('Ctrl Pts',(14.1314716057906,-14.7098797632096,10.9036867901149));
#31072=CARTESIAN_POINT('Ctrl Pts',(13.6752954743875,-15.5,10.8620201234482));
#31073=CARTESIAN_POINT('Ctrl Pts',(14.1314716057906,-16.2901202367904,10.8203534567815));
#31074=CARTESIAN_POINT('Ctrl Pts',(14.5876477371938,-17.0802404735808,10.7786867901149));
#31075=CARTESIAN_POINT('Ctrl Pts',(15.5,-17.0802404735808,10.7370201234482));
#31076=CARTESIAN_POINT('Ctrl Pts',(16.4123522628062,-17.0802404735808,10.6953534567815));
#31077=CARTESIAN_POINT('Ctrl Pts',(16.8685283942094,-16.2901202367904,10.6536867901149));
#31078=CARTESIAN_POINT('Ctrl Pts',(17.3247045256125,-15.5,10.6120201234482));
#31079=CARTESIAN_POINT('Ctrl Pts',(16.8685283942094,-14.7098797632096,10.5703534567815));
#31080=CARTESIAN_POINT('Ctrl Pts',(16.4123522628062,-13.9197595264192,10.5286867901149));
#31081=CARTESIAN_POINT('Ctrl Pts',(15.5,-13.9197595264192,10.4870201234482));
#31082=CARTESIAN_POINT('Ctrl Pts',(14.5876477371938,-13.9197595264192,10.4453534567815));
#31083=CARTESIAN_POINT('Ctrl Pts',(14.1314716057906,-14.7098797632096,10.4036867901149));
#31084=CARTESIAN_POINT('Ctrl Pts',(13.6752954743875,-15.5,10.3620201234482));
#31085=CARTESIAN_POINT('Ctrl Pts',(14.1314716057906,-16.2901202367904,10.3203534567815));
#31086=CARTESIAN_POINT('Ctrl Pts',(14.5876477371938,-17.0802404735808,10.2786867901149));
#31087=CARTESIAN_POINT('Ctrl Pts',(15.5,-17.0802404735808,10.2370201234482));
#31088=CARTESIAN_POINT('Ctrl Pts',(16.4123522628062,-17.0802404735808,10.1953534567815));
#31089=CARTESIAN_POINT('Ctrl Pts',(16.8685283942094,-16.2901202367904,10.1536867901149));
#31090=CARTESIAN_POINT('Ctrl Pts',(17.3247045256125,-15.5,10.1120201234482));
#31091=CARTESIAN_POINT('Ctrl Pts',(16.8685283942094,-14.7098797632096,10.0703534567815));
#31092=CARTESIAN_POINT('Ctrl Pts',(16.4123522628062,-13.9197595264192,10.0286867901149));
#31093=CARTESIAN_POINT('Ctrl Pts',(15.5,-13.9197595264192,9.98702012344819));
#31094=CARTESIAN_POINT('Ctrl Pts',(14.5876477371938,-13.9197595264192,9.94535345678152));
#31095=CARTESIAN_POINT('Ctrl Pts',(14.1314716057906,-14.7098797632096,9.90368679011485));
#31096=CARTESIAN_POINT('Ctrl Pts',(13.6752954743875,-15.5,9.86202012344818));
#31097=CARTESIAN_POINT('Ctrl Pts',(14.1314716057906,-16.2901202367904,9.82035345678151));
#31098=CARTESIAN_POINT('Ctrl Pts',(14.5876477371938,-17.0802404735808,9.77868679011485));
#31099=CARTESIAN_POINT('Ctrl Pts',(15.5,-17.0802404735808,9.73702012344818));
#31100=CARTESIAN_POINT('Ctrl Pts',(16.4123522628062,-17.0802404735808,9.69535345678151));
#31101=CARTESIAN_POINT('Ctrl Pts',(16.8685283942094,-16.2901202367904,9.65368679011485));
#31102=CARTESIAN_POINT('Ctrl Pts',(17.3247045256125,-15.5,9.61202012344818));
#31103=CARTESIAN_POINT('Ctrl Pts',(16.8685283942094,-14.7098797632096,9.57035345678151));
#31104=CARTESIAN_POINT('Ctrl Pts',(16.4123522628062,-13.9197595264192,9.52868679011484));
#31105=CARTESIAN_POINT('Ctrl Pts',(15.5,-13.9197595264192,9.48702012344818));
#31106=CARTESIAN_POINT('Ctrl Pts',(14.5876477371938,-13.9197595264192,9.44535345678151));
#31107=CARTESIAN_POINT('Ctrl Pts',(14.1314716057906,-14.7098797632096,9.40368679011484));
#31108=CARTESIAN_POINT('Ctrl Pts',(13.6752954743875,-15.5,9.36202012344818));
#31109=CARTESIAN_POINT('Ctrl Pts',(14.1314716057906,-16.2901202367904,9.32035345678151));
#31110=CARTESIAN_POINT('Ctrl Pts',(14.5876477371938,-17.0802404735808,9.27868679011484));
#31111=CARTESIAN_POINT('Ctrl Pts',(15.5,-17.0802404735808,9.23702012344818));
#31112=CARTESIAN_POINT('Ctrl Pts',(16.4123522628062,-17.0802404735808,9.19535345678151));
#31113=CARTESIAN_POINT('Ctrl Pts',(16.8685283942094,-16.2901202367904,9.15368679011484));
#31114=CARTESIAN_POINT('Ctrl Pts',(17.3247045256125,-15.5,9.11202012344818));
#31115=CARTESIAN_POINT('Ctrl Pts',(16.8685283942094,-14.7098797632096,9.07035345678151));
#31116=CARTESIAN_POINT('Ctrl Pts',(16.4123522628062,-13.9197595264192,9.02868679011484));
#31117=CARTESIAN_POINT('Ctrl Pts',(15.5,-13.9197595264192,8.98702012344817));
#31118=CARTESIAN_POINT('Ctrl Pts',(14.5876477371938,-13.9197595264192,8.9453534567815));
#31119=CARTESIAN_POINT('Ctrl Pts',(14.1314716057906,-14.7098797632096,8.90368679011484));
#31120=CARTESIAN_POINT('Ctrl Pts',(13.6752954743875,-15.5,8.86202012344817));
#31121=CARTESIAN_POINT('Ctrl Pts',(14.1314716057906,-16.2901202367904,8.8203534567815));
#31122=CARTESIAN_POINT('Ctrl Pts',(14.5876477371938,-17.0802404735808,8.77868679011483));
#31123=CARTESIAN_POINT('Ctrl Pts',(15.5,-17.0802404735808,8.73702012344817));
#31124=CARTESIAN_POINT('Ctrl Pts',(16.4123522628062,-17.0802404735808,8.6953534567815));
#31125=CARTESIAN_POINT('Ctrl Pts',(16.8685283942094,-16.2901202367904,8.65368679011483));
#31126=CARTESIAN_POINT('Ctrl Pts',(17.3247045256125,-15.5,8.61202012344817));
#31127=CARTESIAN_POINT('Ctrl Pts',(16.8685283942094,-14.7098797632096,8.5703534567815));
#31128=CARTESIAN_POINT('Ctrl Pts',(16.4123522628062,-13.9197595264192,8.52868679011483));
#31129=CARTESIAN_POINT('Ctrl Pts',(15.5,-13.9197595264192,8.48702012344816));
#31130=CARTESIAN_POINT('Ctrl Pts',(14.5876477371938,-13.9197595264192,8.4453534567815));
#31131=CARTESIAN_POINT('Ctrl Pts',(14.1314716057906,-14.7098797632096,8.40368679011483));
#31132=CARTESIAN_POINT('Ctrl Pts',(13.6752954743875,-15.5,8.36202012344816));
#31133=CARTESIAN_POINT('Ctrl Pts',(14.1314716057906,-16.2901202367904,8.3203534567815));
#31134=CARTESIAN_POINT('Ctrl Pts',(14.5876477371938,-17.0802404735808,8.27868679011483));
#31135=CARTESIAN_POINT('Ctrl Pts',(15.5,-17.0802404735808,8.23702012344816));
#31136=CARTESIAN_POINT('Ctrl Pts',(16.4123522628062,-17.0802404735808,8.19535345678149));
#31137=CARTESIAN_POINT('Ctrl Pts',(16.8685283942094,-16.2901202367904,8.15368679011483));
#31138=CARTESIAN_POINT('Ctrl Pts',(17.3247045256125,-15.5,8.11202012344816));
#31139=CARTESIAN_POINT('Ctrl Pts',(16.8685283942094,-14.7098797632096,8.0703534567815));
#31140=CARTESIAN_POINT('Ctrl Pts',(16.4123522628062,-13.9197595264192,8.02868679011483));
#31141=CARTESIAN_POINT('Ctrl Pts',(15.5,-13.9197595264192,7.98702012344816));
#31142=CARTESIAN_POINT('Ctrl Pts',(14.5876477371938,-13.9197595264192,7.94535345678149));
#31143=CARTESIAN_POINT('Ctrl Pts',(14.1314716057906,-14.7098797632096,7.90368679011482));
#31144=CARTESIAN_POINT('Ctrl Pts',(13.6752954743875,-15.5,7.86202012344816));
#31145=CARTESIAN_POINT('Ctrl Pts',(14.1314716057906,-16.2901202367904,7.82035345678149));
#31146=CARTESIAN_POINT('Ctrl Pts',(14.5876477371938,-17.0802404735808,7.77868679011482));
#31147=CARTESIAN_POINT('Ctrl Pts',(15.5,-17.0802404735808,7.73702012344816));
#31148=CARTESIAN_POINT('Ctrl Pts',(16.4123522628062,-17.0802404735808,7.69535345678149));
#31149=CARTESIAN_POINT('Ctrl Pts',(16.8685283942094,-16.2901202367904,7.65368679011482));
#31150=CARTESIAN_POINT('Ctrl Pts',(17.3247045256125,-15.5,7.61202012344815));
#31151=CARTESIAN_POINT('Ctrl Pts',(16.8685283942094,-14.7098797632096,7.57035345678149));
#31152=CARTESIAN_POINT('Ctrl Pts',(16.4123522628062,-13.9197595264192,7.52868679011482));
#31153=CARTESIAN_POINT('Ctrl Pts',(15.5,-13.9197595264192,7.48702012344815));
#31154=CARTESIAN_POINT('Ctrl Pts',(14.5876477371938,-13.9197595264192,7.44535345678148));
#31155=CARTESIAN_POINT('Ctrl Pts',(14.1314716057906,-14.7098797632096,7.40368679011482));
#31156=CARTESIAN_POINT('Ctrl Pts',(13.6752954743875,-15.5,7.36202012344815));
#31157=CARTESIAN_POINT('Ctrl Pts',(14.1314716057906,-16.2901202367904,7.32035345678148));
#31158=CARTESIAN_POINT('Ctrl Pts',(14.5876477371938,-17.0802404735808,7.27868679011482));
#31159=CARTESIAN_POINT('Ctrl Pts',(15.5,-17.0802404735808,7.23702012344815));
#31160=CARTESIAN_POINT('Ctrl Pts',(16.4123522628062,-17.0802404735808,7.19535345678148));
#31161=CARTESIAN_POINT('Ctrl Pts',(16.8685283942094,-16.2901202367904,7.15368679011481));
#31162=CARTESIAN_POINT('Ctrl Pts',(17.3247045256125,-15.5,7.11202012344815));
#31163=CARTESIAN_POINT('Ctrl Pts',(16.8685283942094,-14.7098797632096,7.07035345678148));
#31164=CARTESIAN_POINT('Ctrl Pts',(16.4123522628062,-13.9197595264192,7.02868679011481));
#31165=CARTESIAN_POINT('Ctrl Pts',(15.5,-13.9197595264192,6.98702012344815));
#31166=CARTESIAN_POINT('Ctrl Pts',(14.5876477371938,-13.9197595264192,6.94535345678148));
#31167=CARTESIAN_POINT('Ctrl Pts',(14.1314716057906,-14.7098797632096,6.90368679011481));
#31168=CARTESIAN_POINT('Ctrl Pts',(13.6752954743875,-15.5,6.86202012344814));
#31169=CARTESIAN_POINT('Ctrl Pts',(14.1314716057906,-16.2901202367904,6.82035345678148));
#31170=CARTESIAN_POINT('Ctrl Pts',(14.5876477371938,-17.0802404735808,6.77868679011481));
#31171=CARTESIAN_POINT('Ctrl Pts',(15.5,-17.0802404735808,6.73702012344814));
#31172=CARTESIAN_POINT('Ctrl Pts',(16.4123522628062,-17.0802404735808,6.69535345678147));
#31173=CARTESIAN_POINT('Ctrl Pts',(16.8685283942094,-16.2901202367904,6.65368679011481));
#31174=CARTESIAN_POINT('Ctrl Pts',(17.3247045256125,-15.5,6.61202012344814));
#31175=CARTESIAN_POINT('Ctrl Pts',(16.8685283942094,-14.7098797632096,6.57035345678147));
#31176=CARTESIAN_POINT('Ctrl Pts',(16.4123522628062,-13.9197595264192,6.52868679011481));
#31177=CARTESIAN_POINT('Ctrl Pts',(15.5,-13.9197595264192,6.48702012344814));
#31178=CARTESIAN_POINT('Ctrl Pts',(14.5876477371938,-13.9197595264192,6.44535345678147));
#31179=CARTESIAN_POINT('Ctrl Pts',(14.1314716057906,-14.7098797632096,6.40368679011481));
#31180=CARTESIAN_POINT('Ctrl Pts',(13.6752954743875,-15.5,6.36202012344814));
#31181=CARTESIAN_POINT('Ctrl Pts',(14.1314716057906,-16.2901202367904,6.32035345678147));
#31182=CARTESIAN_POINT('Ctrl Pts',(14.5876477371938,-17.0802404735808,6.2786867901148));
#31183=CARTESIAN_POINT('Ctrl Pts',(15.5,-17.0802404735808,6.23702012344813));
#31184=CARTESIAN_POINT('Ctrl Pts',(16.4123522628062,-17.0802404735808,6.19535345678147));
#31185=CARTESIAN_POINT('Ctrl Pts',(16.8685283942094,-16.2901202367904,6.1536867901148));
#31186=CARTESIAN_POINT('Ctrl Pts',(17.3247045256125,-15.5,6.11202012344813));
#31187=CARTESIAN_POINT('Ctrl Pts',(16.8685283942094,-14.7098797632096,6.07035345678147));
#31188=CARTESIAN_POINT('Ctrl Pts',(16.4123522628062,-13.9197595264192,6.0286867901148));
#31189=CARTESIAN_POINT('Ctrl Pts',(15.5,-13.9197595264192,5.98702012344813));
#31190=CARTESIAN_POINT('Ctrl Pts',(14.5876477371938,-13.9197595264192,5.94535345678146));
#31191=CARTESIAN_POINT('Ctrl Pts',(14.1314716057906,-14.7098797632096,5.9036867901148));
#31192=CARTESIAN_POINT('Ctrl Pts',(13.6752954743875,-15.5,5.86202012344813));
#31193=CARTESIAN_POINT('Ctrl Pts',(14.1314716057906,-16.2901202367904,5.82035345678146));
#31194=CARTESIAN_POINT('Ctrl Pts',(14.5876477371938,-17.0802404735808,5.7786867901148));
#31195=CARTESIAN_POINT('Ctrl Pts',(15.5,-17.0802404735808,5.73702012344813));
#31196=CARTESIAN_POINT('Ctrl Pts',(16.4123522628062,-17.0802404735808,5.69535345678146));
#31197=CARTESIAN_POINT('Ctrl Pts',(16.8685283942094,-16.2901202367904,5.65368679011479));
#31198=CARTESIAN_POINT('Ctrl Pts',(17.3247045256125,-15.5,5.61202012344813));
#31199=CARTESIAN_POINT('Ctrl Pts',(16.8685283942094,-14.7098797632096,5.57035345678146));
#31200=CARTESIAN_POINT('Ctrl Pts',(16.4123522628062,-13.9197595264192,5.52868679011479));
#31201=CARTESIAN_POINT('Ctrl Pts',(15.5,-13.9197595264192,5.48702012344813));
#31202=CARTESIAN_POINT('Ctrl Pts',(14.5876477371938,-13.9197595264192,5.44535345678146));
#31203=CARTESIAN_POINT('Ctrl Pts',(14.1314716057906,-14.7098797632096,5.40368679011479));
#31204=CARTESIAN_POINT('Ctrl Pts',(13.6752954743875,-15.5,5.36202012344812));
#31205=CARTESIAN_POINT('Ctrl Pts',(14.1314716057906,-16.2901202367904,5.32035345678146));
#31206=CARTESIAN_POINT('Ctrl Pts',(14.5876477371938,-17.0802404735808,5.27868679011479));
#31207=CARTESIAN_POINT('Ctrl Pts',(15.5,-17.0802404735808,5.23702012344812));
#31208=CARTESIAN_POINT('Ctrl Pts',(16.4123522628062,-17.0802404735808,5.19535345678145));
#31209=CARTESIAN_POINT('Ctrl Pts',(16.8685283942094,-16.2901202367904,5.15368679011479));
#31210=CARTESIAN_POINT('Ctrl Pts',(17.3247045256125,-15.5,5.11202012344812));
#31211=CARTESIAN_POINT('Ctrl Pts',(16.8685283942094,-14.7098797632096,5.07035345678145));
#31212=CARTESIAN_POINT('Ctrl Pts',(16.4123522628062,-13.9197595264192,5.02868679011478));
#31213=CARTESIAN_POINT('Ctrl Pts',(15.5,-13.9197595264192,4.98702012344812));
#31214=CARTESIAN_POINT('Ctrl Pts',(14.5876477371938,-13.9197595264192,4.94535345678145));
#31215=CARTESIAN_POINT('Ctrl Pts',(14.1314716057906,-14.7098797632096,4.90368679011478));
#31216=CARTESIAN_POINT('Ctrl Pts',(13.6752954743875,-15.5,4.86202012344812));
#31217=CARTESIAN_POINT('Ctrl Pts',(14.1314716057906,-16.2901202367904,4.82035345678145));
#31218=CARTESIAN_POINT('Ctrl Pts',(14.5876477371938,-17.0802404735808,4.77868679011478));
#31219=CARTESIAN_POINT('Ctrl Pts',(15.5,-17.0802404735808,4.73702012344812));
#31220=CARTESIAN_POINT('Ctrl Pts',(16.4123522628062,-17.0802404735808,4.69535345678145));
#31221=CARTESIAN_POINT('Ctrl Pts',(16.8685283942094,-16.2901202367904,4.65368679011478));
#31222=CARTESIAN_POINT('Ctrl Pts',(17.3247045256125,-15.5,4.61202012344811));
#31223=CARTESIAN_POINT('Ctrl Pts',(16.8685283942094,-14.7098797632096,4.57035345678145));
#31224=CARTESIAN_POINT('Ctrl Pts',(16.4123522628062,-13.9197595264192,4.52868679011478));
#31225=CARTESIAN_POINT('Ctrl Pts',(15.5,-13.9197595264192,4.48702012344811));
#31226=CARTESIAN_POINT('Ctrl Pts',(14.5876477371938,-13.9197595264192,4.44535345678144));
#31227=CARTESIAN_POINT('Ctrl Pts',(14.1314716057906,-14.7098797632096,4.40368679011478));
#31228=CARTESIAN_POINT('Ctrl Pts',(13.6752954743875,-15.5,4.36202012344811));
#31229=CARTESIAN_POINT('Ctrl Pts',(14.1314716057906,-16.2901202367904,4.32035345678144));
#31230=CARTESIAN_POINT('Ctrl Pts',(14.5876477371938,-17.0802404735808,4.27868679011477));
#31231=CARTESIAN_POINT('Ctrl Pts',(15.5,-17.0802404735808,4.23702012344811));
#31232=CARTESIAN_POINT('Ctrl Pts',(16.4123522628062,-17.0802404735808,4.19535345678144));
#31233=CARTESIAN_POINT('Ctrl Pts',(16.8685283942094,-16.2901202367904,4.15368679011477));
#31234=CARTESIAN_POINT('Ctrl Pts',(17.3247045256125,-15.5,4.11202012344811));
#31235=CARTESIAN_POINT('Ctrl Pts',(16.8685283942094,-14.7098797632096,4.07035345678144));
#31236=CARTESIAN_POINT('Ctrl Pts',(16.4123522628062,-13.9197595264192,4.02868679011477));
#31237=CARTESIAN_POINT('Ctrl Pts',(15.5,-13.9197595264192,3.9870201234481));
#31238=CARTESIAN_POINT('Ctrl Pts',(14.5876477371938,-13.9197595264192,3.94535345678144));
#31239=CARTESIAN_POINT('Ctrl Pts',(14.1314716057906,-14.7098797632096,3.90368679011477));
#31240=CARTESIAN_POINT('Ctrl Pts',(13.6752954743875,-15.5,3.8620201234481));
#31241=CARTESIAN_POINT('Ctrl Pts',(14.1314716057906,-16.2901202367904,3.82035345678144));
#31242=CARTESIAN_POINT('Ctrl Pts',(14.5876477371938,-17.0802404735808,3.77868679011477));
#31243=CARTESIAN_POINT('Ctrl Pts',(15.5,-17.0802404735808,3.7370201234481));
#31244=CARTESIAN_POINT('Ctrl Pts',(16.4123522628062,-17.0802404735808,3.69535345678143));
#31245=CARTESIAN_POINT('Ctrl Pts',(16.8685283942094,-16.2901202367904,3.65368679011477));
#31246=CARTESIAN_POINT('Ctrl Pts',(17.3247045256125,-15.5,3.6120201234481));
#31247=CARTESIAN_POINT('Ctrl Pts',(16.8685283942094,-14.7098797632096,3.57035345678143));
#31248=CARTESIAN_POINT('Ctrl Pts',(16.4123522628062,-13.9197595264192,3.52868679011477));
#31249=CARTESIAN_POINT('Ctrl Pts',(15.5,-13.9197595264192,3.4870201234481));
#31250=CARTESIAN_POINT('Ctrl Pts',(14.5876477371938,-13.9197595264192,3.44535345678143));
#31251=CARTESIAN_POINT('Ctrl Pts',(14.1314716057906,-14.7098797632096,3.40368679011477));
#31252=CARTESIAN_POINT('Ctrl Pts',(13.6752954743875,-15.5,3.3620201234481));
#31253=CARTESIAN_POINT('Ctrl Pts',(14.1314716057906,-16.2901202367904,3.32035345678143));
#31254=CARTESIAN_POINT('Ctrl Pts',(14.5876477371938,-17.0802404735808,3.27868679011476));
#31255=CARTESIAN_POINT('Ctrl Pts',(15.5,-17.0802404735808,3.2370201234481));
#31256=CARTESIAN_POINT('Ctrl Pts',(16.4123522628062,-17.0802404735808,3.19535345678143));
#31257=CARTESIAN_POINT('Ctrl Pts',(16.8685283942094,-16.2901202367904,3.15368679011476));
#31258=CARTESIAN_POINT('Ctrl Pts',(17.3247045256125,-15.5,3.11202012344809));
#31259=CARTESIAN_POINT('Ctrl Pts',(16.8685283942094,-14.7098797632096,3.07035345678143));
#31260=CARTESIAN_POINT('Ctrl Pts',(16.4123522628062,-13.9197595264192,3.02868679011476));
#31261=CARTESIAN_POINT('Ctrl Pts',(15.5,-13.9197595264192,2.98702012344809));
#31262=CARTESIAN_POINT('Ctrl Pts',(14.5876477371938,-13.9197595264192,2.94535345678143));
#31263=CARTESIAN_POINT('Ctrl Pts',(14.1314716057906,-14.7098797632096,2.90368679011476));
#31264=CARTESIAN_POINT('Ctrl Pts',(13.6752954743875,-15.5,2.86202012344809));
#31265=CARTESIAN_POINT('Ctrl Pts',(14.1314716057906,-16.2901202367904,2.82035345678142));
#31266=CARTESIAN_POINT('Ctrl Pts',(14.5876477371938,-17.0802404735808,2.77868679011475));
#31267=CARTESIAN_POINT('Ctrl Pts',(15.5,-17.0802404735808,2.73702012344809));
#31268=CARTESIAN_POINT('Ctrl Pts',(16.4123522628062,-17.0802404735808,2.69535345678142));
#31269=CARTESIAN_POINT('Ctrl Pts',(16.8685283942094,-16.2901202367904,2.65368679011475));
#31270=CARTESIAN_POINT('Ctrl Pts',(17.3247045256125,-15.5,2.61202012344809));
#31271=CARTESIAN_POINT('Ctrl Pts',(16.8685283942094,-14.7098797632096,2.57035345678142));
#31272=CARTESIAN_POINT('Ctrl Pts',(16.4123522628062,-13.9197595264192,2.52868679011475));
#31273=CARTESIAN_POINT('Ctrl Pts',(15.5,-13.9197595264192,2.48702012344808));
#31274=CARTESIAN_POINT('Ctrl Pts',(14.5876477371938,-13.9197595264192,2.44535345678142));
#31275=CARTESIAN_POINT('Ctrl Pts',(14.1314716057906,-14.7098797632096,2.40368679011475));
#31276=CARTESIAN_POINT('Ctrl Pts',(13.6752954743875,-15.5,2.36202012344808));
#31277=CARTESIAN_POINT('Ctrl Pts',(14.1314716057906,-16.2901202367904,2.32035345678142));
#31278=CARTESIAN_POINT('Ctrl Pts',(14.5876477371938,-17.0802404735808,2.27868679011475));
#31279=CARTESIAN_POINT('Ctrl Pts',(15.5,-17.0802404735808,2.23702012344808));
#31280=CARTESIAN_POINT('Ctrl Pts',(16.4123522628062,-17.0802404735808,2.19535345678142));
#31281=CARTESIAN_POINT('Ctrl Pts',(16.8685283942094,-16.2901202367904,2.15368679011475));
#31282=CARTESIAN_POINT('Ctrl Pts',(17.3247045256125,-15.5,2.11202012344808));
#31283=CARTESIAN_POINT('Ctrl Pts',(16.8685283942094,-14.7098797632096,2.07035345678141));
#31284=CARTESIAN_POINT('Ctrl Pts',(16.4123522628062,-13.9197595264192,2.02868679011475));
#31285=CARTESIAN_POINT('Ctrl Pts',(15.5,-13.9197595264192,1.98702012344808));
#31286=CARTESIAN_POINT('Ctrl Pts',(14.5876477371938,-13.9197595264192,1.94535345678141));
#31287=CARTESIAN_POINT('Ctrl Pts',(14.1314716057906,-14.7098797632096,1.90368679011474));
#31288=CARTESIAN_POINT('Ctrl Pts',(13.6752954743875,-15.5,1.86202012344808));
#31289=CARTESIAN_POINT('Ctrl Pts',(14.1314716057906,-16.2901202367904,1.82035345678141));
#31290=CARTESIAN_POINT('Ctrl Pts',(14.5876477371938,-17.0802404735808,1.77868679011474));
#31291=CARTESIAN_POINT('Ctrl Pts',(15.5,-17.0802404735808,1.73702012344808));
#31292=CARTESIAN_POINT('Ctrl Pts',(16.4123522628062,-17.0802404735808,1.69535345678141));
#31293=CARTESIAN_POINT('Ctrl Pts',(16.8685283942094,-16.2901202367904,1.65368679011474));
#31294=CARTESIAN_POINT('Ctrl Pts',(17.3247045256125,-15.5,1.61202012344807));
#31295=CARTESIAN_POINT('Ctrl Pts',(16.8685283942094,-14.7098797632096,1.57035345678141));
#31296=CARTESIAN_POINT('Ctrl Pts',(16.4123522628062,-13.9197595264192,1.52868679011474));
#31297=CARTESIAN_POINT('Ctrl Pts',(15.5,-13.9197595264192,1.48702012344807));
#31298=CARTESIAN_POINT('Ctrl Pts',(14.5876477371938,-13.9197595264192,1.4453534567814));
#31299=CARTESIAN_POINT('Ctrl Pts',(14.1314716057906,-14.7098797632096,1.40368679011474));
#31300=CARTESIAN_POINT('Ctrl Pts',(13.6752954743875,-15.5,1.36202012344807));
#31301=CARTESIAN_POINT('Ctrl Pts',(14.1314716057906,-16.2901202367904,1.3203534567814));
#31302=CARTESIAN_POINT('Ctrl Pts',(14.5876477371938,-17.0802404735808,1.27868679011473));
#31303=CARTESIAN_POINT('Ctrl Pts',(15.5,-17.0802404735808,1.23702012344807));
#31304=CARTESIAN_POINT('Ctrl Pts',(16.4123522628062,-17.0802404735808,1.1953534567814));
#31305=CARTESIAN_POINT('Ctrl Pts',(16.8685283942094,-16.2901202367904,1.15368679011473));
#31306=CARTESIAN_POINT('Ctrl Pts',(17.3247045256125,-15.5,1.11202012344807));
#31307=CARTESIAN_POINT('Ctrl Pts',(16.8685283942094,-14.7098797632096,1.0703534567814));
#31308=CARTESIAN_POINT('Ctrl Pts',(16.4123522628062,-13.9197595264192,1.02868679011473));
#31309=CARTESIAN_POINT('Ctrl Pts',(15.5,-13.9197595264192,0.987020123448066));
#31310=CARTESIAN_POINT('Ctrl Pts',(14.5876477371938,-13.9197595264192,0.945353456781398));
#31311=CARTESIAN_POINT('Ctrl Pts',(14.1314716057906,-14.7098797632096,0.903686790114731));
#31312=CARTESIAN_POINT('Ctrl Pts',(13.6752954743875,-15.5,0.862020123448063));
#31313=CARTESIAN_POINT('Ctrl Pts',(14.1314716057906,-16.2901202367904,0.820353456781396));
#31314=CARTESIAN_POINT('Ctrl Pts',(14.5876477371938,-17.0802404735808,0.778686790114729));
#31315=CARTESIAN_POINT('Ctrl Pts',(15.5,-17.0802404735808,0.737020123448062));
#31316=CARTESIAN_POINT('Ctrl Pts',(16.4123522628062,-17.0802404735808,0.695353456781395));
#31317=CARTESIAN_POINT('Ctrl Pts',(16.8685283942094,-16.2901202367904,0.653686790114727));
#31318=CARTESIAN_POINT('Ctrl Pts',(17.3247045256125,-15.5,0.61202012344806));
#31319=CARTESIAN_POINT('Ctrl Pts',(16.8685283942094,-14.7098797632096,0.570353456781393));
#31320=CARTESIAN_POINT('Ctrl Pts',(16.4123522628062,-13.9197595264192,0.528686790114725));
#31321=CARTESIAN_POINT('Ctrl Pts',(15.5,-13.9197595264192,0.487020123448058));
#31322=CARTESIAN_POINT('Ctrl Pts',(14.5876477371938,-13.9197595264192,0.445353456781391));
#31323=CARTESIAN_POINT('Ctrl Pts',(14.1314716057906,-14.7098797632096,0.403686790114724));
#31324=CARTESIAN_POINT('Ctrl Pts',(13.6752954743875,-15.5,0.362020123448056));
#31325=CARTESIAN_POINT('Ctrl Pts',(14.1314716057906,-16.2901202367904,0.320353456781389));
#31326=CARTESIAN_POINT('Ctrl Pts',(14.5876477371938,-17.0802404735808,0.278686790114722));
#31327=CARTESIAN_POINT('Ctrl Pts',(15.5,-17.0802404735808,0.237020123448055));
#31328=CARTESIAN_POINT('Ctrl Pts',(16.4123522628062,-17.0802404735808,0.195353456781387));
#31329=CARTESIAN_POINT('Ctrl Pts',(16.8685283942094,-16.2901202367904,0.15368679011472));
#31330=CARTESIAN_POINT('Ctrl Pts',(17.3247045256125,-15.5,0.112020123448053));
#31331=CARTESIAN_POINT('Ctrl Pts',(16.8685283942094,-14.7098797632096,0.0703534567813853));
#31332=CARTESIAN_POINT('Ctrl Pts',(16.4123522628062,-13.9197595264192,0.028686790114718));
#31333=CARTESIAN_POINT('Ctrl Pts',(15.5,-13.9197595264192,-0.0129798765519492));
#31334=CARTESIAN_POINT('Ctrl Pts',(14.5876477371938,-13.9197595264192,-0.0546465432186148));
#31335=CARTESIAN_POINT('Ctrl Pts',(14.1314716057906,-14.7098797632096,-0.0963132098852821));
#31336=CARTESIAN_POINT('Ctrl Pts',(13.6752954743875,-15.5,-0.137979876551949));
#31337=CARTESIAN_POINT('Ctrl Pts',(14.1314716057906,-16.2901202367904,-0.179646543218617));
#31338=CARTESIAN_POINT('Ctrl Pts',(14.5876477371938,-17.0802404735808,-0.221313209885284));
#31339=CARTESIAN_POINT('Ctrl Pts',(15.5,-17.0802404735808,-0.262979876551951));
#31340=CARTESIAN_POINT('Ctrl Pts',(16.4123522628062,-17.0802404735808,-0.304646543218618));
#31341=CARTESIAN_POINT('Ctrl Pts',(16.8685283942094,-16.2901202367904,-0.346313209885286));
#31342=CARTESIAN_POINT('Ctrl Pts',(17.3247045256125,-15.5,-0.387979876551953));
#31343=CARTESIAN_POINT('Ctrl Pts',(16.8685283942094,-14.7098797632096,-0.42964654321862));
#31344=CARTESIAN_POINT('Ctrl Pts',(16.4123522628062,-13.9197595264192,-0.471313209885288));
#31345=CARTESIAN_POINT('Ctrl Pts',(15.5,-13.9197595264192,-0.512979876551955));
#31346=CARTESIAN_POINT('Ctrl Pts',(14.5876477371938,-13.9197595264192,-0.554646543218622));
#31347=CARTESIAN_POINT('Ctrl Pts',(14.1314716057906,-14.7098797632096,-0.596313209885289));
#31348=CARTESIAN_POINT('Ctrl Pts',(13.6752954743875,-15.5,-0.637979876551957));
#31349=CARTESIAN_POINT('Ctrl Pts',(14.1314716057906,-16.2901202367904,-0.679646543218624));
#31350=CARTESIAN_POINT('Ctrl Pts',(14.5876477371938,-17.0802404735808,-0.721313209885291));
#31351=CARTESIAN_POINT('Ctrl Pts',(15.5,-17.0802404735808,-0.762979876551959));
#31352=CARTESIAN_POINT('Ctrl Pts',(16.4123522628062,-17.0802404735808,-0.804646543218626));
#31353=CARTESIAN_POINT('Ctrl Pts',(16.8685283942094,-16.2901202367904,-0.846313209885293));
#31354=CARTESIAN_POINT('Ctrl Pts',(17.3247045256125,-15.5,-0.88797987655196));
#31355=CARTESIAN_POINT('Ctrl Pts',(16.8685283942094,-14.7098797632096,-0.929646543218628));
#31356=CARTESIAN_POINT('Ctrl Pts',(16.4123522628062,-13.9197595264192,-0.971313209885295));
#31357=CARTESIAN_POINT('Ctrl Pts',(15.5,-13.9197595264192,-1.01297987655196));
#31358=CARTESIAN_POINT('Ctrl Pts',(14.5876477371938,-13.9197595264192,-1.05464654321863));
#31359=CARTESIAN_POINT('Ctrl Pts',(14.1314716057906,-14.7098797632096,-1.0963132098853));
#31360=CARTESIAN_POINT('Ctrl Pts',(13.6752954743875,-15.5,-1.13797987655196));
#31361=CARTESIAN_POINT('Ctrl Pts',(14.1314716057906,-16.2901202367904,-1.17964654321863));
#31362=CARTESIAN_POINT('Ctrl Pts',(14.5876477371938,-17.0802404735808,-1.2213132098853));
#31363=CARTESIAN_POINT('Ctrl Pts',(15.5,-17.0802404735808,-1.26297987655196));
#31364=CARTESIAN_POINT('Ctrl Pts',(16.4123522628062,-17.0802404735808,-1.30464654321863));
#31365=CARTESIAN_POINT('Ctrl Pts',(16.8685283942094,-16.2901202367904,-1.3463132098853));
#31366=CARTESIAN_POINT('Ctrl Pts',(17.3247045256125,-15.5,-1.38797987655197));
#31367=CARTESIAN_POINT('Ctrl Pts',(16.8685283942094,-14.7098797632096,-1.42964654321863));
#31368=CARTESIAN_POINT('Ctrl Pts',(16.4123522628062,-13.9197595264192,-1.4713132098853));
#31369=CARTESIAN_POINT('Ctrl Pts',(15.5,-13.9197595264192,-1.51297987655197));
#31370=CARTESIAN_POINT('Ctrl Pts',(14.5876477371938,-13.9197595264192,-1.55464654321864));
#31371=CARTESIAN_POINT('Ctrl Pts',(14.1314716057906,-14.7098797632096,-1.5963132098853));
#31372=CARTESIAN_POINT('Ctrl Pts',(13.6752954743875,-15.5,-1.63797987655197));
#31373=CARTESIAN_POINT('Ctrl Pts',(14.1314716057906,-16.2901202367904,-1.67964654321864));
#31374=CARTESIAN_POINT('Ctrl Pts',(14.5876477371938,-17.0802404735808,-1.7213132098853));
#31375=CARTESIAN_POINT('Ctrl Pts',(15.5,-17.0802404735808,-1.76297987655197));
#31376=CARTESIAN_POINT('Ctrl Pts',(16.4123522628062,-17.0802404735808,-1.80464654321864));
#31377=CARTESIAN_POINT('Ctrl Pts',(16.8685283942094,-16.2901202367904,-1.84631320988531));
#31378=CARTESIAN_POINT('Ctrl Pts',(17.3247045256125,-15.5,-1.88797987655197));
#31379=CARTESIAN_POINT('Ctrl Pts',(16.8685283942094,-14.7098797632096,-1.92964654321864));
#31380=CARTESIAN_POINT('Ctrl Pts',(16.700583153372,-14.4189900731899,-1.94498649173085));
#31381=CARTESIAN_POINT('Ctrl Pts',(16.4288420454487,-14.2215586016756,-1.96260250461286));
#31382=CARTESIAN_POINT('Ctrl Pts',(15.3465777998745,-13.4352476007234,-2.03276185973389));
#31383=CARTESIAN_POINT('Ctrl Pts',(14.2643135543003,-12.6489365997713,-2.10292121485492));
#31384=CARTESIAN_POINT('Ctrl Pts',(15.5,-17.0802404735808,11.1745));
#31385=CARTESIAN_POINT('Ctrl Pts',(16.4123522628062,-17.0802404735808,11.1328333333333));
#31386=CARTESIAN_POINT('Ctrl Pts',(16.8685283942094,-16.2901202367904,11.0911666666667));
#31387=CARTESIAN_POINT('Ctrl Pts',(17.3247045256125,-15.5,11.0495));
#31388=CARTESIAN_POINT('Ctrl Pts',(16.8685283942094,-14.7098797632096,11.0078333333333));
#31389=CARTESIAN_POINT('Ctrl Pts',(16.4123522628062,-13.9197595264192,10.9661666666667));
#31390=CARTESIAN_POINT('Ctrl Pts',(15.5,-13.9197595264192,10.9245));
#31391=CARTESIAN_POINT('Ctrl Pts',(14.5876477371938,-13.9197595264192,10.8828333333333));
#31392=CARTESIAN_POINT('Ctrl Pts',(14.1314716057906,-14.7098797632096,10.8411666666667));
#31393=CARTESIAN_POINT('Ctrl Pts',(13.6752954743875,-15.5,10.7995));
#31394=CARTESIAN_POINT('Ctrl Pts',(14.1314716057906,-16.2901202367904,10.7578333333333));
#31395=CARTESIAN_POINT('Ctrl Pts',(14.5876477371938,-17.0802404735808,10.7161666666667));
#31396=CARTESIAN_POINT('Ctrl Pts',(15.5,-17.0802404735808,10.6745));
#31397=CARTESIAN_POINT('Ctrl Pts',(16.4123522628062,-17.0802404735808,10.6328333333333));
#31398=CARTESIAN_POINT('Ctrl Pts',(16.8685283942094,-16.2901202367904,10.5911666666667));
#31399=CARTESIAN_POINT('Ctrl Pts',(17.3247045256125,-15.5,10.5495));
#31400=CARTESIAN_POINT('Ctrl Pts',(16.8685283942094,-14.7098797632096,10.5078333333333));
#31401=CARTESIAN_POINT('Ctrl Pts',(16.4123522628062,-13.9197595264192,10.4661666666667));
#31402=CARTESIAN_POINT('Ctrl Pts',(15.5,-13.9197595264192,10.4245));
#31403=CARTESIAN_POINT('Ctrl Pts',(14.5876477371938,-13.9197595264192,10.3828333333333));
#31404=CARTESIAN_POINT('Ctrl Pts',(14.1314716057906,-14.7098797632096,10.3411666666667));
#31405=CARTESIAN_POINT('Ctrl Pts',(13.6752954743875,-15.5,10.2995));
#31406=CARTESIAN_POINT('Ctrl Pts',(14.1314716057906,-16.2901202367904,10.2578333333333));
#31407=CARTESIAN_POINT('Ctrl Pts',(14.5876477371938,-17.0802404735808,10.2161666666667));
#31408=CARTESIAN_POINT('Ctrl Pts',(15.5,-17.0802404735808,10.1745));
#31409=CARTESIAN_POINT('Ctrl Pts',(16.4123522628062,-17.0802404735808,10.1328333333333));
#31410=CARTESIAN_POINT('Ctrl Pts',(16.8685283942094,-16.2901202367904,10.0911666666667));
#31411=CARTESIAN_POINT('Ctrl Pts',(17.3247045256125,-15.5,10.0495));
#31412=CARTESIAN_POINT('Ctrl Pts',(16.8685283942094,-14.7098797632096,10.0078333333333));
#31413=CARTESIAN_POINT('Ctrl Pts',(16.4123522628062,-13.9197595264192,9.96616666666665));
#31414=CARTESIAN_POINT('Ctrl Pts',(15.5,-13.9197595264192,9.92449999999998));
#31415=CARTESIAN_POINT('Ctrl Pts',(14.5876477371938,-13.9197595264192,9.88283333333331));
#31416=CARTESIAN_POINT('Ctrl Pts',(14.1314716057906,-14.7098797632096,9.84116666666665));
#31417=CARTESIAN_POINT('Ctrl Pts',(13.6752954743875,-15.5,9.79949999999998));
#31418=CARTESIAN_POINT('Ctrl Pts',(14.1314716057906,-16.2901202367904,9.75783333333331));
#31419=CARTESIAN_POINT('Ctrl Pts',(14.5876477371938,-17.0802404735808,9.71616666666665));
#31420=CARTESIAN_POINT('Ctrl Pts',(15.5,-17.0802404735808,9.67449999999998));
#31421=CARTESIAN_POINT('Ctrl Pts',(16.4123522628062,-17.0802404735808,9.63283333333331));
#31422=CARTESIAN_POINT('Ctrl Pts',(16.8685283942094,-16.2901202367904,9.59116666666664));
#31423=CARTESIAN_POINT('Ctrl Pts',(17.3247045256125,-15.5,9.54949999999998));
#31424=CARTESIAN_POINT('Ctrl Pts',(16.8685283942094,-14.7098797632096,9.50783333333331));
#31425=CARTESIAN_POINT('Ctrl Pts',(16.4123522628062,-13.9197595264192,9.46616666666664));
#31426=CARTESIAN_POINT('Ctrl Pts',(15.5,-13.9197595264192,9.42449999999998));
#31427=CARTESIAN_POINT('Ctrl Pts',(14.5876477371938,-13.9197595264192,9.38283333333331));
#31428=CARTESIAN_POINT('Ctrl Pts',(14.1314716057906,-14.7098797632096,9.34116666666664));
#31429=CARTESIAN_POINT('Ctrl Pts',(13.6752954743875,-15.5,9.29949999999998));
#31430=CARTESIAN_POINT('Ctrl Pts',(14.1314716057906,-16.2901202367904,9.25783333333331));
#31431=CARTESIAN_POINT('Ctrl Pts',(14.5876477371938,-17.0802404735808,9.21616666666664));
#31432=CARTESIAN_POINT('Ctrl Pts',(15.5,-17.0802404735808,9.17449999999997));
#31433=CARTESIAN_POINT('Ctrl Pts',(16.4123522628062,-17.0802404735808,9.13283333333331));
#31434=CARTESIAN_POINT('Ctrl Pts',(16.8685283942094,-16.2901202367904,9.09116666666664));
#31435=CARTESIAN_POINT('Ctrl Pts',(17.3247045256125,-15.5,9.04949999999997));
#31436=CARTESIAN_POINT('Ctrl Pts',(16.8685283942094,-14.7098797632096,9.0078333333333));
#31437=CARTESIAN_POINT('Ctrl Pts',(16.4123522628062,-13.9197595264192,8.96616666666664));
#31438=CARTESIAN_POINT('Ctrl Pts',(15.5,-13.9197595264192,8.92449999999997));
#31439=CARTESIAN_POINT('Ctrl Pts',(14.5876477371938,-13.9197595264192,8.8828333333333));
#31440=CARTESIAN_POINT('Ctrl Pts',(14.1314716057906,-14.7098797632096,8.84116666666664));
#31441=CARTESIAN_POINT('Ctrl Pts',(13.6752954743875,-15.5,8.79949999999997));
#31442=CARTESIAN_POINT('Ctrl Pts',(14.1314716057906,-16.2901202367904,8.7578333333333));
#31443=CARTESIAN_POINT('Ctrl Pts',(14.5876477371938,-17.0802404735808,8.71616666666663));
#31444=CARTESIAN_POINT('Ctrl Pts',(15.5,-17.0802404735808,8.67449999999997));
#31445=CARTESIAN_POINT('Ctrl Pts',(16.4123522628062,-17.0802404735808,8.6328333333333));
#31446=CARTESIAN_POINT('Ctrl Pts',(16.8685283942094,-16.2901202367904,8.59116666666663));
#31447=CARTESIAN_POINT('Ctrl Pts',(17.3247045256125,-15.5,8.54949999999996));
#31448=CARTESIAN_POINT('Ctrl Pts',(16.8685283942094,-14.7098797632096,8.50783333333329));
#31449=CARTESIAN_POINT('Ctrl Pts',(16.4123522628062,-13.9197595264192,8.46616666666663));
#31450=CARTESIAN_POINT('Ctrl Pts',(15.5,-13.9197595264192,8.42449999999996));
#31451=CARTESIAN_POINT('Ctrl Pts',(14.5876477371938,-13.9197595264192,8.3828333333333));
#31452=CARTESIAN_POINT('Ctrl Pts',(14.1314716057906,-14.7098797632096,8.34116666666663));
#31453=CARTESIAN_POINT('Ctrl Pts',(13.6752954743875,-15.5,8.29949999999996));
#31454=CARTESIAN_POINT('Ctrl Pts',(14.1314716057906,-16.2901202367904,8.25783333333329));
#31455=CARTESIAN_POINT('Ctrl Pts',(14.5876477371938,-17.0802404735808,8.21616666666663));
#31456=CARTESIAN_POINT('Ctrl Pts',(15.5,-17.0802404735808,8.17449999999996));
#31457=CARTESIAN_POINT('Ctrl Pts',(16.4123522628062,-17.0802404735808,8.13283333333329));
#31458=CARTESIAN_POINT('Ctrl Pts',(16.8685283942094,-16.2901202367904,8.09116666666663));
#31459=CARTESIAN_POINT('Ctrl Pts',(17.3247045256125,-15.5,8.04949999999996));
#31460=CARTESIAN_POINT('Ctrl Pts',(16.8685283942094,-14.7098797632096,8.00783333333329));
#31461=CARTESIAN_POINT('Ctrl Pts',(16.4123522628062,-13.9197595264192,7.96616666666662));
#31462=CARTESIAN_POINT('Ctrl Pts',(15.5,-13.9197595264192,7.92449999999996));
#31463=CARTESIAN_POINT('Ctrl Pts',(14.5876477371938,-13.9197595264192,7.88283333333329));
#31464=CARTESIAN_POINT('Ctrl Pts',(14.1314716057906,-14.7098797632096,7.84116666666662));
#31465=CARTESIAN_POINT('Ctrl Pts',(13.6752954743875,-15.5,7.79949999999995));
#31466=CARTESIAN_POINT('Ctrl Pts',(14.1314716057906,-16.2901202367904,7.75783333333329));
#31467=CARTESIAN_POINT('Ctrl Pts',(14.5876477371938,-17.0802404735808,7.71616666666662));
#31468=CARTESIAN_POINT('Ctrl Pts',(15.5,-17.0802404735808,7.67449999999995));
#31469=CARTESIAN_POINT('Ctrl Pts',(16.4123522628062,-17.0802404735808,7.63283333333328));
#31470=CARTESIAN_POINT('Ctrl Pts',(16.8685283942094,-16.2901202367904,7.59116666666662));
#31471=CARTESIAN_POINT('Ctrl Pts',(17.3247045256125,-15.5,7.54949999999995));
#31472=CARTESIAN_POINT('Ctrl Pts',(16.8685283942094,-14.7098797632096,7.50783333333328));
#31473=CARTESIAN_POINT('Ctrl Pts',(16.4123522628062,-13.9197595264192,7.46616666666662));
#31474=CARTESIAN_POINT('Ctrl Pts',(15.5,-13.9197595264192,7.42449999999995));
#31475=CARTESIAN_POINT('Ctrl Pts',(14.5876477371938,-13.9197595264192,7.38283333333328));
#31476=CARTESIAN_POINT('Ctrl Pts',(14.1314716057906,-14.7098797632096,7.34116666666661));
#31477=CARTESIAN_POINT('Ctrl Pts',(13.6752954743875,-15.5,7.29949999999995));
#31478=CARTESIAN_POINT('Ctrl Pts',(14.1314716057906,-16.2901202367904,7.25783333333328));
#31479=CARTESIAN_POINT('Ctrl Pts',(14.5876477371938,-17.0802404735808,7.21616666666661));
#31480=CARTESIAN_POINT('Ctrl Pts',(15.5,-17.0802404735808,7.17449999999995));
#31481=CARTESIAN_POINT('Ctrl Pts',(16.4123522628062,-17.0802404735808,7.13283333333328));
#31482=CARTESIAN_POINT('Ctrl Pts',(16.8685283942094,-16.2901202367904,7.09116666666661));
#31483=CARTESIAN_POINT('Ctrl Pts',(17.3247045256125,-15.5,7.04949999999994));
#31484=CARTESIAN_POINT('Ctrl Pts',(16.8685283942094,-14.7098797632096,7.00783333333328));
#31485=CARTESIAN_POINT('Ctrl Pts',(16.4123522628062,-13.9197595264192,6.96616666666661));
#31486=CARTESIAN_POINT('Ctrl Pts',(15.5,-13.9197595264192,6.92449999999994));
#31487=CARTESIAN_POINT('Ctrl Pts',(14.5876477371938,-13.9197595264192,6.88283333333327));
#31488=CARTESIAN_POINT('Ctrl Pts',(14.1314716057906,-14.7098797632096,6.84116666666661));
#31489=CARTESIAN_POINT('Ctrl Pts',(13.6752954743875,-15.5,6.79949999999994));
#31490=CARTESIAN_POINT('Ctrl Pts',(14.1314716057906,-16.2901202367904,6.75783333333327));
#31491=CARTESIAN_POINT('Ctrl Pts',(14.5876477371938,-17.0802404735808,6.71616666666661));
#31492=CARTESIAN_POINT('Ctrl Pts',(15.5,-17.0802404735808,6.67449999999994));
#31493=CARTESIAN_POINT('Ctrl Pts',(16.4123522628062,-17.0802404735808,6.63283333333327));
#31494=CARTESIAN_POINT('Ctrl Pts',(16.8685283942094,-16.2901202367904,6.59116666666661));
#31495=CARTESIAN_POINT('Ctrl Pts',(17.3247045256125,-15.5,6.54949999999994));
#31496=CARTESIAN_POINT('Ctrl Pts',(16.8685283942094,-14.7098797632096,6.50783333333327));
#31497=CARTESIAN_POINT('Ctrl Pts',(16.4123522628062,-13.9197595264192,6.4661666666666));
#31498=CARTESIAN_POINT('Ctrl Pts',(15.5,-13.9197595264192,6.42449999999994));
#31499=CARTESIAN_POINT('Ctrl Pts',(14.5876477371938,-13.9197595264192,6.38283333333327));
#31500=CARTESIAN_POINT('Ctrl Pts',(14.1314716057906,-14.7098797632096,6.3411666666666));
#31501=CARTESIAN_POINT('Ctrl Pts',(13.6752954743875,-15.5,6.29949999999993));
#31502=CARTESIAN_POINT('Ctrl Pts',(14.1314716057906,-16.2901202367904,6.25783333333327));
#31503=CARTESIAN_POINT('Ctrl Pts',(14.5876477371938,-17.0802404735808,6.2161666666666));
#31504=CARTESIAN_POINT('Ctrl Pts',(15.5,-17.0802404735808,6.17449999999993));
#31505=CARTESIAN_POINT('Ctrl Pts',(16.4123522628062,-17.0802404735808,6.13283333333326));
#31506=CARTESIAN_POINT('Ctrl Pts',(16.8685283942094,-16.2901202367904,6.0911666666666));
#31507=CARTESIAN_POINT('Ctrl Pts',(17.3247045256125,-15.5,6.04949999999993));
#31508=CARTESIAN_POINT('Ctrl Pts',(16.8685283942094,-14.7098797632096,6.00783333333326));
#31509=CARTESIAN_POINT('Ctrl Pts',(16.4123522628062,-13.9197595264192,5.9661666666666));
#31510=CARTESIAN_POINT('Ctrl Pts',(15.5,-13.9197595264192,5.92449999999993));
#31511=CARTESIAN_POINT('Ctrl Pts',(14.5876477371938,-13.9197595264192,5.88283333333326));
#31512=CARTESIAN_POINT('Ctrl Pts',(14.1314716057906,-14.7098797632096,5.8411666666666));
#31513=CARTESIAN_POINT('Ctrl Pts',(13.6752954743875,-15.5,5.79949999999993));
#31514=CARTESIAN_POINT('Ctrl Pts',(14.1314716057906,-16.2901202367904,5.75783333333326));
#31515=CARTESIAN_POINT('Ctrl Pts',(14.5876477371938,-17.0802404735808,5.71616666666659));
#31516=CARTESIAN_POINT('Ctrl Pts',(15.5,-17.0802404735808,5.67449999999993));
#31517=CARTESIAN_POINT('Ctrl Pts',(16.4123522628062,-17.0802404735808,5.63283333333326));
#31518=CARTESIAN_POINT('Ctrl Pts',(16.8685283942094,-16.2901202367904,5.59116666666659));
#31519=CARTESIAN_POINT('Ctrl Pts',(17.3247045256125,-15.5,5.54949999999992));
#31520=CARTESIAN_POINT('Ctrl Pts',(16.8685283942094,-14.7098797632096,5.50783333333326));
#31521=CARTESIAN_POINT('Ctrl Pts',(16.4123522628062,-13.9197595264192,5.46616666666659));
#31522=CARTESIAN_POINT('Ctrl Pts',(15.5,-13.9197595264192,5.42449999999992));
#31523=CARTESIAN_POINT('Ctrl Pts',(14.5876477371938,-13.9197595264192,5.38283333333326));
#31524=CARTESIAN_POINT('Ctrl Pts',(14.1314716057906,-14.7098797632096,5.34116666666659));
#31525=CARTESIAN_POINT('Ctrl Pts',(13.6752954743875,-15.5,5.29949999999992));
#31526=CARTESIAN_POINT('Ctrl Pts',(14.1314716057906,-16.2901202367904,5.25783333333325));
#31527=CARTESIAN_POINT('Ctrl Pts',(14.5876477371938,-17.0802404735808,5.21616666666659));
#31528=CARTESIAN_POINT('Ctrl Pts',(15.5,-17.0802404735808,5.17449999999992));
#31529=CARTESIAN_POINT('Ctrl Pts',(16.4123522628062,-17.0802404735808,5.13283333333325));
#31530=CARTESIAN_POINT('Ctrl Pts',(16.8685283942094,-16.2901202367904,5.09116666666658));
#31531=CARTESIAN_POINT('Ctrl Pts',(17.3247045256125,-15.5,5.04949999999992));
#31532=CARTESIAN_POINT('Ctrl Pts',(16.8685283942094,-14.7098797632096,5.00783333333325));
#31533=CARTESIAN_POINT('Ctrl Pts',(16.4123522628062,-13.9197595264192,4.96616666666658));
#31534=CARTESIAN_POINT('Ctrl Pts',(15.5,-13.9197595264192,4.92449999999992));
#31535=CARTESIAN_POINT('Ctrl Pts',(14.5876477371938,-13.9197595264192,4.88283333333325));
#31536=CARTESIAN_POINT('Ctrl Pts',(14.1314716057906,-14.7098797632096,4.84116666666658));
#31537=CARTESIAN_POINT('Ctrl Pts',(13.6752954743875,-15.5,4.79949999999991));
#31538=CARTESIAN_POINT('Ctrl Pts',(14.1314716057906,-16.2901202367904,4.75783333333325));
#31539=CARTESIAN_POINT('Ctrl Pts',(14.5876477371938,-17.0802404735808,4.71616666666658));
#31540=CARTESIAN_POINT('Ctrl Pts',(15.5,-17.0802404735808,4.67449999999991));
#31541=CARTESIAN_POINT('Ctrl Pts',(16.4123522628062,-17.0802404735808,4.63283333333324));
#31542=CARTESIAN_POINT('Ctrl Pts',(16.8685283942094,-16.2901202367904,4.59116666666658));
#31543=CARTESIAN_POINT('Ctrl Pts',(17.3247045256125,-15.5,4.54949999999991));
#31544=CARTESIAN_POINT('Ctrl Pts',(16.8685283942094,-14.7098797632096,4.50783333333324));
#31545=CARTESIAN_POINT('Ctrl Pts',(16.4123522628062,-13.9197595264192,4.46616666666658));
#31546=CARTESIAN_POINT('Ctrl Pts',(15.5,-13.9197595264192,4.42449999999991));
#31547=CARTESIAN_POINT('Ctrl Pts',(14.5876477371938,-13.9197595264192,4.38283333333324));
#31548=CARTESIAN_POINT('Ctrl Pts',(14.1314716057906,-14.7098797632096,4.34116666666657));
#31549=CARTESIAN_POINT('Ctrl Pts',(13.6752954743875,-15.5,4.29949999999991));
#31550=CARTESIAN_POINT('Ctrl Pts',(14.1314716057906,-16.2901202367904,4.25783333333324));
#31551=CARTESIAN_POINT('Ctrl Pts',(14.5876477371938,-17.0802404735808,4.21616666666657));
#31552=CARTESIAN_POINT('Ctrl Pts',(15.5,-17.0802404735808,4.17449999999991));
#31553=CARTESIAN_POINT('Ctrl Pts',(16.4123522628062,-17.0802404735808,4.13283333333324));
#31554=CARTESIAN_POINT('Ctrl Pts',(16.8685283942094,-16.2901202367904,4.09116666666657));
#31555=CARTESIAN_POINT('Ctrl Pts',(17.3247045256125,-15.5,4.0494999999999));
#31556=CARTESIAN_POINT('Ctrl Pts',(16.8685283942094,-14.7098797632096,4.00783333333324));
#31557=CARTESIAN_POINT('Ctrl Pts',(16.4123522628062,-13.9197595264192,3.96616666666657));
#31558=CARTESIAN_POINT('Ctrl Pts',(15.5,-13.9197595264192,3.9244999999999));
#31559=CARTESIAN_POINT('Ctrl Pts',(14.5876477371938,-13.9197595264192,3.88283333333323));
#31560=CARTESIAN_POINT('Ctrl Pts',(14.1314716057906,-14.7098797632096,3.84116666666657));
#31561=CARTESIAN_POINT('Ctrl Pts',(13.6752954743875,-15.5,3.7994999999999));
#31562=CARTESIAN_POINT('Ctrl Pts',(14.1314716057906,-16.2901202367904,3.75783333333323));
#31563=CARTESIAN_POINT('Ctrl Pts',(14.5876477371938,-17.0802404735808,3.71616666666657));
#31564=CARTESIAN_POINT('Ctrl Pts',(15.5,-17.0802404735808,3.6744999999999));
#31565=CARTESIAN_POINT('Ctrl Pts',(16.4123522628062,-17.0802404735808,3.63283333333323));
#31566=CARTESIAN_POINT('Ctrl Pts',(16.8685283942094,-16.2901202367904,3.59116666666656));
#31567=CARTESIAN_POINT('Ctrl Pts',(17.3247045256125,-15.5,3.5494999999999));
#31568=CARTESIAN_POINT('Ctrl Pts',(16.8685283942094,-14.7098797632096,3.50783333333323));
#31569=CARTESIAN_POINT('Ctrl Pts',(16.4123522628062,-13.9197595264192,3.46616666666656));
#31570=CARTESIAN_POINT('Ctrl Pts',(15.5,-13.9197595264192,3.4244999999999));
#31571=CARTESIAN_POINT('Ctrl Pts',(14.5876477371938,-13.9197595264192,3.38283333333323));
#31572=CARTESIAN_POINT('Ctrl Pts',(14.1314716057906,-14.7098797632096,3.34116666666656));
#31573=CARTESIAN_POINT('Ctrl Pts',(13.6752954743875,-15.5,3.29949999999989));
#31574=CARTESIAN_POINT('Ctrl Pts',(14.1314716057906,-16.2901202367904,3.25783333333323));
#31575=CARTESIAN_POINT('Ctrl Pts',(14.5876477371938,-17.0802404735808,3.21616666666656));
#31576=CARTESIAN_POINT('Ctrl Pts',(15.5,-17.0802404735808,3.17449999999989));
#31577=CARTESIAN_POINT('Ctrl Pts',(16.4123522628062,-17.0802404735808,3.13283333333323));
#31578=CARTESIAN_POINT('Ctrl Pts',(16.8685283942094,-16.2901202367904,3.09116666666656));
#31579=CARTESIAN_POINT('Ctrl Pts',(17.3247045256125,-15.5,3.04949999999989));
#31580=CARTESIAN_POINT('Ctrl Pts',(16.8685283942094,-14.7098797632096,3.00783333333322));
#31581=CARTESIAN_POINT('Ctrl Pts',(16.4123522628062,-13.9197595264192,2.96616666666656));
#31582=CARTESIAN_POINT('Ctrl Pts',(15.5,-13.9197595264192,2.92449999999989));
#31583=CARTESIAN_POINT('Ctrl Pts',(14.5876477371938,-13.9197595264192,2.88283333333322));
#31584=CARTESIAN_POINT('Ctrl Pts',(14.1314716057906,-14.7098797632096,2.84116666666655));
#31585=CARTESIAN_POINT('Ctrl Pts',(13.6752954743875,-15.5,2.79949999999989));
#31586=CARTESIAN_POINT('Ctrl Pts',(14.1314716057906,-16.2901202367904,2.75783333333322));
#31587=CARTESIAN_POINT('Ctrl Pts',(14.5876477371938,-17.0802404735808,2.71616666666655));
#31588=CARTESIAN_POINT('Ctrl Pts',(15.5,-17.0802404735808,2.67449999999989));
#31589=CARTESIAN_POINT('Ctrl Pts',(16.4123522628062,-17.0802404735808,2.63283333333322));
#31590=CARTESIAN_POINT('Ctrl Pts',(16.8685283942094,-16.2901202367904,2.59116666666655));
#31591=CARTESIAN_POINT('Ctrl Pts',(17.3247045256125,-15.5,2.54949999999988));
#31592=CARTESIAN_POINT('Ctrl Pts',(16.8685283942094,-14.7098797632096,2.50783333333322));
#31593=CARTESIAN_POINT('Ctrl Pts',(16.4123522628062,-13.9197595264192,2.46616666666655));
#31594=CARTESIAN_POINT('Ctrl Pts',(15.5,-13.9197595264192,2.42449999999988));
#31595=CARTESIAN_POINT('Ctrl Pts',(14.5876477371938,-13.9197595264192,2.38283333333321));
#31596=CARTESIAN_POINT('Ctrl Pts',(14.1314716057906,-14.7098797632096,2.34116666666655));
#31597=CARTESIAN_POINT('Ctrl Pts',(13.6752954743875,-15.5,2.29949999999988));
#31598=CARTESIAN_POINT('Ctrl Pts',(14.1314716057906,-16.2901202367904,2.25783333333321));
#31599=CARTESIAN_POINT('Ctrl Pts',(14.5876477371938,-17.0802404735808,2.21616666666655));
#31600=CARTESIAN_POINT('Ctrl Pts',(15.5,-17.0802404735808,2.17449999999988));
#31601=CARTESIAN_POINT('Ctrl Pts',(16.4123522628062,-17.0802404735808,2.13283333333321));
#31602=CARTESIAN_POINT('Ctrl Pts',(16.8685283942094,-16.2901202367904,2.09116666666655));
#31603=CARTESIAN_POINT('Ctrl Pts',(17.3247045256125,-15.5,2.04949999999988));
#31604=CARTESIAN_POINT('Ctrl Pts',(16.8685283942094,-14.7098797632096,2.00783333333321));
#31605=CARTESIAN_POINT('Ctrl Pts',(16.4123522628062,-13.9197595264192,1.96616666666654));
#31606=CARTESIAN_POINT('Ctrl Pts',(15.5,-13.9197595264192,1.92449999999988));
#31607=CARTESIAN_POINT('Ctrl Pts',(14.5876477371938,-13.9197595264192,1.88283333333321));
#31608=CARTESIAN_POINT('Ctrl Pts',(14.1314716057906,-14.7098797632096,1.84116666666654));
#31609=CARTESIAN_POINT('Ctrl Pts',(13.6752954743875,-15.5,1.79949999999987));
#31610=CARTESIAN_POINT('Ctrl Pts',(14.1314716057906,-16.2901202367904,1.75783333333321));
#31611=CARTESIAN_POINT('Ctrl Pts',(14.5876477371938,-17.0802404735808,1.71616666666654));
#31612=CARTESIAN_POINT('Ctrl Pts',(15.5,-17.0802404735808,1.67449999999987));
#31613=CARTESIAN_POINT('Ctrl Pts',(16.4123522628062,-17.0802404735808,1.63283333333321));
#31614=CARTESIAN_POINT('Ctrl Pts',(16.8685283942094,-16.2901202367904,1.59116666666654));
#31615=CARTESIAN_POINT('Ctrl Pts',(17.3247045256125,-15.5,1.54949999999987));
#31616=CARTESIAN_POINT('Ctrl Pts',(16.8685283942094,-14.7098797632096,1.5078333333332));
#31617=CARTESIAN_POINT('Ctrl Pts',(16.4123522628062,-13.9197595264192,1.46616666666654));
#31618=CARTESIAN_POINT('Ctrl Pts',(15.5,-13.9197595264192,1.42449999999987));
#31619=CARTESIAN_POINT('Ctrl Pts',(14.5876477371938,-13.9197595264192,1.3828333333332));
#31620=CARTESIAN_POINT('Ctrl Pts',(14.1314716057906,-14.7098797632096,1.34116666666653));
#31621=CARTESIAN_POINT('Ctrl Pts',(13.6752954743875,-15.5,1.29949999999987));
#31622=CARTESIAN_POINT('Ctrl Pts',(14.1314716057906,-16.2901202367904,1.2578333333332));
#31623=CARTESIAN_POINT('Ctrl Pts',(14.5876477371938,-17.0802404735808,1.21616666666653));
#31624=CARTESIAN_POINT('Ctrl Pts',(15.5,-17.0802404735808,1.17449999999986));
#31625=CARTESIAN_POINT('Ctrl Pts',(16.4123522628062,-17.0802404735808,1.1328333333332));
#31626=CARTESIAN_POINT('Ctrl Pts',(16.8685283942094,-16.2901202367904,1.09116666666653));
#31627=CARTESIAN_POINT('Ctrl Pts',(17.3247045256125,-15.5,1.04949999999986));
#31628=CARTESIAN_POINT('Ctrl Pts',(16.8685283942094,-14.7098797632096,1.0078333333332));
#31629=CARTESIAN_POINT('Ctrl Pts',(16.4123522628062,-13.9197595264192,0.96616666666653));
#31630=CARTESIAN_POINT('Ctrl Pts',(15.5,-13.9197595264192,0.924499999999863));
#31631=CARTESIAN_POINT('Ctrl Pts',(14.5876477371938,-13.9197595264192,0.882833333333196));
#31632=CARTESIAN_POINT('Ctrl Pts',(14.1314716057906,-14.7098797632096,0.841166666666529));
#31633=CARTESIAN_POINT('Ctrl Pts',(13.6752954743875,-15.5,0.799499999999861));
#31634=CARTESIAN_POINT('Ctrl Pts',(14.1314716057906,-16.2901202367904,0.757833333333194));
#31635=CARTESIAN_POINT('Ctrl Pts',(14.5876477371938,-17.0802404735808,0.716166666666527));
#31636=CARTESIAN_POINT('Ctrl Pts',(15.5,-17.0802404735808,0.674499999999859));
#31637=CARTESIAN_POINT('Ctrl Pts',(16.4123522628062,-17.0802404735808,0.632833333333192));
#31638=CARTESIAN_POINT('Ctrl Pts',(16.8685283942094,-16.2901202367904,0.591166666666525));
#31639=CARTESIAN_POINT('Ctrl Pts',(17.3247045256125,-15.5,0.549499999999857));
#31640=CARTESIAN_POINT('Ctrl Pts',(16.8685283942094,-14.7098797632096,0.50783333333319));
#31641=CARTESIAN_POINT('Ctrl Pts',(16.4123522628062,-13.9197595264192,0.466166666666523));
#31642=CARTESIAN_POINT('Ctrl Pts',(15.5,-13.9197595264192,0.424499999999856));
#31643=CARTESIAN_POINT('Ctrl Pts',(14.5876477371938,-13.9197595264192,0.382833333333188));
#31644=CARTESIAN_POINT('Ctrl Pts',(14.1314716057906,-14.7098797632096,0.341166666666521));
#31645=CARTESIAN_POINT('Ctrl Pts',(13.6752954743875,-15.5,0.299499999999854));
#31646=CARTESIAN_POINT('Ctrl Pts',(14.1314716057906,-16.2901202367904,0.257833333333186));
#31647=CARTESIAN_POINT('Ctrl Pts',(14.5876477371938,-17.0802404735808,0.216166666666519));
#31648=CARTESIAN_POINT('Ctrl Pts',(15.5,-17.0802404735808,0.174499999999852));
#31649=CARTESIAN_POINT('Ctrl Pts',(16.4123522628062,-17.0802404735808,0.132833333333185));
#31650=CARTESIAN_POINT('Ctrl Pts',(16.8685283942094,-16.2901202367904,0.0911666666665173));
#31651=CARTESIAN_POINT('Ctrl Pts',(17.3247045256125,-15.5,0.04949999999985));
#31652=CARTESIAN_POINT('Ctrl Pts',(16.8685283942094,-14.7098797632096,0.00783333333318273));
#31653=CARTESIAN_POINT('Ctrl Pts',(16.4123522628062,-13.9197595264192,-0.0338333333334846));
#31654=CARTESIAN_POINT('Ctrl Pts',(15.5,-13.9197595264192,-0.0755000000001518));
#31655=CARTESIAN_POINT('Ctrl Pts',(14.5876477371938,-13.9197595264192,-0.117166666666817));
#31656=CARTESIAN_POINT('Ctrl Pts',(14.1314716057906,-14.7098797632096,-0.158833333333485));
#31657=CARTESIAN_POINT('Ctrl Pts',(13.6752954743875,-15.5,-0.200500000000152));
#31658=CARTESIAN_POINT('Ctrl Pts',(14.1314716057906,-16.2901202367904,-0.242166666666819));
#31659=CARTESIAN_POINT('Ctrl Pts',(14.5876477371938,-17.0802404735808,-0.283833333333486));
#31660=CARTESIAN_POINT('Ctrl Pts',(15.5,-17.0802404735808,-0.325500000000154));
#31661=CARTESIAN_POINT('Ctrl Pts',(16.4123522628062,-17.0802404735808,-0.367166666666821));
#31662=CARTESIAN_POINT('Ctrl Pts',(16.8685283942094,-16.2901202367904,-0.408833333333488));
#31663=CARTESIAN_POINT('Ctrl Pts',(17.3247045256125,-15.5,-0.450500000000156));
#31664=CARTESIAN_POINT('Ctrl Pts',(16.8685283942094,-14.7098797632096,-0.492166666666823));
#31665=CARTESIAN_POINT('Ctrl Pts',(16.4123522628062,-13.9197595264192,-0.53383333333349));
#31666=CARTESIAN_POINT('Ctrl Pts',(15.5,-13.9197595264192,-0.575500000000157));
#31667=CARTESIAN_POINT('Ctrl Pts',(14.5876477371938,-13.9197595264192,-0.617166666666825));
#31668=CARTESIAN_POINT('Ctrl Pts',(14.1314716057906,-14.7098797632096,-0.658833333333492));
#31669=CARTESIAN_POINT('Ctrl Pts',(13.6752954743875,-15.5,-0.700500000000159));
#31670=CARTESIAN_POINT('Ctrl Pts',(14.1314716057906,-16.2901202367904,-0.742166666666827));
#31671=CARTESIAN_POINT('Ctrl Pts',(14.5876477371938,-17.0802404735808,-0.783833333333494));
#31672=CARTESIAN_POINT('Ctrl Pts',(15.5,-17.0802404735808,-0.825500000000161));
#31673=CARTESIAN_POINT('Ctrl Pts',(16.4123522628062,-17.0802404735808,-0.867166666666829));
#31674=CARTESIAN_POINT('Ctrl Pts',(16.8685283942094,-16.2901202367904,-0.908833333333496));
#31675=CARTESIAN_POINT('Ctrl Pts',(17.3247045256125,-15.5,-0.950500000000163));
#31676=CARTESIAN_POINT('Ctrl Pts',(16.8685283942094,-14.7098797632096,-0.99216666666683));
#31677=CARTESIAN_POINT('Ctrl Pts',(16.4123522628062,-13.9197595264192,-1.0338333333335));
#31678=CARTESIAN_POINT('Ctrl Pts',(15.5,-13.9197595264192,-1.07550000000016));
#31679=CARTESIAN_POINT('Ctrl Pts',(14.5876477371938,-13.9197595264192,-1.11716666666683));
#31680=CARTESIAN_POINT('Ctrl Pts',(14.1314716057906,-14.7098797632096,-1.1588333333335));
#31681=CARTESIAN_POINT('Ctrl Pts',(13.6752954743875,-15.5,-1.20050000000017));
#31682=CARTESIAN_POINT('Ctrl Pts',(14.1314716057906,-16.2901202367904,-1.24216666666683));
#31683=CARTESIAN_POINT('Ctrl Pts',(14.5876477371938,-17.0802404735808,-1.2838333333335));
#31684=CARTESIAN_POINT('Ctrl Pts',(15.5,-17.0802404735808,-1.32550000000017));
#31685=CARTESIAN_POINT('Ctrl Pts',(16.4123522628062,-17.0802404735808,-1.36716666666683));
#31686=CARTESIAN_POINT('Ctrl Pts',(16.8685283942094,-16.2901202367904,-1.4088333333335));
#31687=CARTESIAN_POINT('Ctrl Pts',(17.3247045256125,-15.5,-1.45050000000017));
#31688=CARTESIAN_POINT('Ctrl Pts',(16.8685283942094,-14.7098797632096,-1.49216666666684));
#31689=CARTESIAN_POINT('Ctrl Pts',(16.4123522628062,-13.9197595264192,-1.5338333333335));
#31690=CARTESIAN_POINT('Ctrl Pts',(15.5,-13.9197595264192,-1.57550000000017));
#31691=CARTESIAN_POINT('Ctrl Pts',(14.5876477371938,-13.9197595264192,-1.61716666666684));
#31692=CARTESIAN_POINT('Ctrl Pts',(14.1314716057906,-14.7098797632096,-1.65883333333351));
#31693=CARTESIAN_POINT('Ctrl Pts',(13.6752954743875,-15.5,-1.70050000000017));
#31694=CARTESIAN_POINT('Ctrl Pts',(14.1314716057906,-16.2901202367904,-1.74216666666684));
#31695=CARTESIAN_POINT('Ctrl Pts',(14.5876477371938,-17.0802404735808,-1.78383333333351));
#31696=CARTESIAN_POINT('Ctrl Pts',(15.5,-17.0802404735808,-1.82550000000017));
#31697=CARTESIAN_POINT('Ctrl Pts',(16.4123522628062,-17.0802404735808,-1.86716666666684));
#31698=CARTESIAN_POINT('Ctrl Pts',(16.8685283942094,-16.2901202367904,-1.90883333333351));
#31699=CARTESIAN_POINT('Ctrl Pts',(17.3247045256125,-15.5,-1.95050000000018));
#31700=CARTESIAN_POINT('Ctrl Pts',(16.8685283942094,-14.7098797632096,-1.99216666666684));
#31701=CARTESIAN_POINT('Ctrl Pts',(16.700583153372,-14.4189900731899,-2.00750661517905));
#31702=CARTESIAN_POINT('Ctrl Pts',(16.4288420454487,-14.2215586016756,-2.02512262806106));
#31703=CARTESIAN_POINT('Ctrl Pts',(15.3465777998745,-13.4352476007234,-2.09528198318209));
#31704=CARTESIAN_POINT('Ctrl Pts',(14.2643135543003,-12.6489365997713,-2.16544133830312));
#31705=CARTESIAN_POINT('Ctrl Pts',(-17.0802317716412,-15.5000000000001,
11.1745050240672));
#31706=CARTESIAN_POINT('Ctrl Pts',(-17.0802317716412,-16.4123472387391,
11.1328383574005));
#31707=CARTESIAN_POINT('Ctrl Pts',(-16.2901158858206,-16.8685208581087,
11.0911716907338));
#31708=CARTESIAN_POINT('Ctrl Pts',(-15.4999999999999,-17.3246944774782,
11.0495050240672));
#31709=CARTESIAN_POINT('Ctrl Pts',(-14.7098841141793,-16.8685208581087,
11.0078383574005));
#31710=CARTESIAN_POINT('Ctrl Pts',(-13.9197682283587,-16.4123472387391,
10.9661716907338));
#31711=CARTESIAN_POINT('Ctrl Pts',(-13.9197682283587,-15.5,10.9245050240672));
#31712=CARTESIAN_POINT('Ctrl Pts',(-13.9197682283587,-14.587652761261,10.8828383574005));
#31713=CARTESIAN_POINT('Ctrl Pts',(-14.7098841141793,-14.1314791418915,
10.8411716907338));
#31714=CARTESIAN_POINT('Ctrl Pts',(-15.5,-13.6753055225219,10.7995050240672));
#31715=CARTESIAN_POINT('Ctrl Pts',(-16.2901158858206,-14.1314791418915,
10.7578383574005));
#31716=CARTESIAN_POINT('Ctrl Pts',(-17.0802317716412,-14.587652761261,10.7161716907338));
#31717=CARTESIAN_POINT('Ctrl Pts',(-17.0802317716412,-15.5000000000001,
10.6745050240672));
#31718=CARTESIAN_POINT('Ctrl Pts',(-17.0802317716412,-16.4123472387391,
10.6328383574005));
#31719=CARTESIAN_POINT('Ctrl Pts',(-16.2901158858206,-16.8685208581087,
10.5911716907338));
#31720=CARTESIAN_POINT('Ctrl Pts',(-15.4999999999999,-17.3246944774782,
10.5495050240672));
#31721=CARTESIAN_POINT('Ctrl Pts',(-14.7098841141793,-16.8685208581087,
10.5078383574005));
#31722=CARTESIAN_POINT('Ctrl Pts',(-13.9197682283587,-16.4123472387391,
10.4661716907338));
#31723=CARTESIAN_POINT('Ctrl Pts',(-13.9197682283587,-15.5,10.4245050240672));
#31724=CARTESIAN_POINT('Ctrl Pts',(-13.9197682283587,-14.587652761261,10.3828383574005));
#31725=CARTESIAN_POINT('Ctrl Pts',(-14.7098841141793,-14.1314791418915,
10.3411716907338));
#31726=CARTESIAN_POINT('Ctrl Pts',(-15.5,-13.6753055225219,10.2995050240672));
#31727=CARTESIAN_POINT('Ctrl Pts',(-16.2901158858206,-14.1314791418915,
10.2578383574005));
#31728=CARTESIAN_POINT('Ctrl Pts',(-17.0802317716412,-14.587652761261,10.2161716907338));
#31729=CARTESIAN_POINT('Ctrl Pts',(-17.0802317716412,-15.5000000000001,
10.1745050240672));
#31730=CARTESIAN_POINT('Ctrl Pts',(-17.0802317716412,-16.4123472387391,
10.1328383574005));
#31731=CARTESIAN_POINT('Ctrl Pts',(-16.2901158858206,-16.8685208581087,
10.0911716907338));
#31732=CARTESIAN_POINT('Ctrl Pts',(-15.4999999999999,-17.3246944774782,
10.0495050240672));
#31733=CARTESIAN_POINT('Ctrl Pts',(-14.7098841141793,-16.8685208581087,
10.0078383574005));
#31734=CARTESIAN_POINT('Ctrl Pts',(-13.9197682283587,-16.4123472387391,
9.96617169073382));
#31735=CARTESIAN_POINT('Ctrl Pts',(-13.9197682283587,-15.5,9.92450502406715));
#31736=CARTESIAN_POINT('Ctrl Pts',(-13.9197682283587,-14.587652761261,9.88283835740048));
#31737=CARTESIAN_POINT('Ctrl Pts',(-14.7098841141793,-14.1314791418915,
9.84117169073381));
#31738=CARTESIAN_POINT('Ctrl Pts',(-15.5,-13.6753055225219,9.79950502406715));
#31739=CARTESIAN_POINT('Ctrl Pts',(-16.2901158858206,-14.1314791418915,
9.75783835740048));
#31740=CARTESIAN_POINT('Ctrl Pts',(-17.0802317716412,-14.587652761261,9.71617169073381));
#31741=CARTESIAN_POINT('Ctrl Pts',(-17.0802317716412,-15.5000000000001,
9.67450502406715));
#31742=CARTESIAN_POINT('Ctrl Pts',(-17.0802317716412,-16.4123472387391,
9.63283835740048));
#31743=CARTESIAN_POINT('Ctrl Pts',(-16.2901158858206,-16.8685208581087,
9.59117169073381));
#31744=CARTESIAN_POINT('Ctrl Pts',(-15.4999999999999,-17.3246944774782,
9.54950502406714));
#31745=CARTESIAN_POINT('Ctrl Pts',(-14.7098841141793,-16.8685208581087,
9.50783835740048));
#31746=CARTESIAN_POINT('Ctrl Pts',(-13.9197682283587,-16.4123472387391,
9.46617169073381));
#31747=CARTESIAN_POINT('Ctrl Pts',(-13.9197682283587,-15.5,9.42450502406714));
#31748=CARTESIAN_POINT('Ctrl Pts',(-13.9197682283587,-14.587652761261,9.38283835740048));
#31749=CARTESIAN_POINT('Ctrl Pts',(-14.7098841141793,-14.1314791418915,
9.34117169073381));
#31750=CARTESIAN_POINT('Ctrl Pts',(-15.5,-13.6753055225219,9.29950502406714));
#31751=CARTESIAN_POINT('Ctrl Pts',(-16.2901158858206,-14.1314791418915,
9.25783835740048));
#31752=CARTESIAN_POINT('Ctrl Pts',(-17.0802317716412,-14.587652761261,9.21617169073381));
#31753=CARTESIAN_POINT('Ctrl Pts',(-17.0802317716412,-15.5000000000001,
9.17450502406714));
#31754=CARTESIAN_POINT('Ctrl Pts',(-17.0802317716412,-16.4123472387391,
9.13283835740048));
#31755=CARTESIAN_POINT('Ctrl Pts',(-16.2901158858206,-16.8685208581087,
9.09117169073381));
#31756=CARTESIAN_POINT('Ctrl Pts',(-15.4999999999999,-17.3246944774782,
9.04950502406714));
#31757=CARTESIAN_POINT('Ctrl Pts',(-14.7098841141793,-16.8685208581087,
9.00783835740047));
#31758=CARTESIAN_POINT('Ctrl Pts',(-13.9197682283587,-16.4123472387391,
8.9661716907338));
#31759=CARTESIAN_POINT('Ctrl Pts',(-13.9197682283587,-15.5,8.92450502406714));
#31760=CARTESIAN_POINT('Ctrl Pts',(-13.9197682283587,-14.587652761261,8.88283835740047));
#31761=CARTESIAN_POINT('Ctrl Pts',(-14.7098841141793,-14.1314791418915,
8.8411716907338));
#31762=CARTESIAN_POINT('Ctrl Pts',(-15.5,-13.6753055225219,8.79950502406714));
#31763=CARTESIAN_POINT('Ctrl Pts',(-16.2901158858206,-14.1314791418915,
8.75783835740047));
#31764=CARTESIAN_POINT('Ctrl Pts',(-17.0802317716412,-14.587652761261,8.7161716907338));
#31765=CARTESIAN_POINT('Ctrl Pts',(-17.0802317716412,-15.5000000000001,
8.67450502406713));
#31766=CARTESIAN_POINT('Ctrl Pts',(-17.0802317716412,-16.4123472387391,
8.63283835740047));
#31767=CARTESIAN_POINT('Ctrl Pts',(-16.2901158858206,-16.8685208581087,
8.5911716907338));
#31768=CARTESIAN_POINT('Ctrl Pts',(-15.4999999999999,-17.3246944774782,
8.54950502406713));
#31769=CARTESIAN_POINT('Ctrl Pts',(-14.7098841141793,-16.8685208581087,
8.50783835740046));
#31770=CARTESIAN_POINT('Ctrl Pts',(-13.9197682283587,-16.4123472387391,
8.4661716907338));
#31771=CARTESIAN_POINT('Ctrl Pts',(-13.9197682283587,-15.5,8.42450502406713));
#31772=CARTESIAN_POINT('Ctrl Pts',(-13.9197682283587,-14.587652761261,8.38283835740046));
#31773=CARTESIAN_POINT('Ctrl Pts',(-14.7098841141793,-14.1314791418915,
8.3411716907338));
#31774=CARTESIAN_POINT('Ctrl Pts',(-15.5,-13.6753055225219,8.29950502406713));
#31775=CARTESIAN_POINT('Ctrl Pts',(-16.2901158858206,-14.1314791418915,
8.25783835740046));
#31776=CARTESIAN_POINT('Ctrl Pts',(-17.0802317716412,-14.587652761261,8.21617169073379));
#31777=CARTESIAN_POINT('Ctrl Pts',(-17.0802317716412,-15.5000000000001,
8.17450502406713));
#31778=CARTESIAN_POINT('Ctrl Pts',(-17.0802317716412,-16.4123472387391,
8.13283835740046));
#31779=CARTESIAN_POINT('Ctrl Pts',(-16.2901158858206,-16.8685208581087,
8.09117169073379));
#31780=CARTESIAN_POINT('Ctrl Pts',(-15.4999999999999,-17.3246944774782,
8.04950502406713));
#31781=CARTESIAN_POINT('Ctrl Pts',(-14.7098841141793,-16.8685208581087,
8.00783835740046));
#31782=CARTESIAN_POINT('Ctrl Pts',(-13.9197682283587,-16.4123472387391,
7.96617169073379));
#31783=CARTESIAN_POINT('Ctrl Pts',(-13.9197682283587,-15.5,7.92450502406712));
#31784=CARTESIAN_POINT('Ctrl Pts',(-13.9197682283587,-14.587652761261,7.88283835740046));
#31785=CARTESIAN_POINT('Ctrl Pts',(-14.7098841141793,-14.1314791418915,
7.84117169073379));
#31786=CARTESIAN_POINT('Ctrl Pts',(-15.5,-13.6753055225219,7.79950502406712));
#31787=CARTESIAN_POINT('Ctrl Pts',(-16.2901158858206,-14.1314791418915,
7.75783835740046));
#31788=CARTESIAN_POINT('Ctrl Pts',(-17.0802317716412,-14.587652761261,7.71617169073379));
#31789=CARTESIAN_POINT('Ctrl Pts',(-17.0802317716412,-15.5000000000001,
7.67450502406712));
#31790=CARTESIAN_POINT('Ctrl Pts',(-17.0802317716412,-16.4123472387391,
7.63283835740045));
#31791=CARTESIAN_POINT('Ctrl Pts',(-16.2901158858206,-16.8685208581087,
7.59117169073379));
#31792=CARTESIAN_POINT('Ctrl Pts',(-15.4999999999999,-17.3246944774782,
7.54950502406712));
#31793=CARTESIAN_POINT('Ctrl Pts',(-14.7098841141793,-16.8685208581087,
7.50783835740045));
#31794=CARTESIAN_POINT('Ctrl Pts',(-13.9197682283587,-16.4123472387391,
7.46617169073379));
#31795=CARTESIAN_POINT('Ctrl Pts',(-13.9197682283587,-15.5,7.42450502406712));
#31796=CARTESIAN_POINT('Ctrl Pts',(-13.9197682283587,-14.587652761261,7.38283835740045));
#31797=CARTESIAN_POINT('Ctrl Pts',(-14.7098841141793,-14.1314791418915,
7.34117169073378));
#31798=CARTESIAN_POINT('Ctrl Pts',(-15.5,-13.6753055225219,7.29950502406712));
#31799=CARTESIAN_POINT('Ctrl Pts',(-16.2901158858206,-14.1314791418915,
7.25783835740045));
#31800=CARTESIAN_POINT('Ctrl Pts',(-17.0802317716412,-14.587652761261,7.21617169073378));
#31801=CARTESIAN_POINT('Ctrl Pts',(-17.0802317716412,-15.5000000000001,
7.17450502406711));
#31802=CARTESIAN_POINT('Ctrl Pts',(-17.0802317716412,-16.4123472387391,
7.13283835740044));
#31803=CARTESIAN_POINT('Ctrl Pts',(-16.2901158858206,-16.8685208581087,
7.09117169073378));
#31804=CARTESIAN_POINT('Ctrl Pts',(-15.4999999999999,-17.3246944774782,
7.04950502406711));
#31805=CARTESIAN_POINT('Ctrl Pts',(-14.7098841141793,-16.8685208581087,
7.00783835740045));
#31806=CARTESIAN_POINT('Ctrl Pts',(-13.9197682283587,-16.4123472387391,
6.96617169073378));
#31807=CARTESIAN_POINT('Ctrl Pts',(-13.9197682283587,-15.5,6.92450502406711));
#31808=CARTESIAN_POINT('Ctrl Pts',(-13.9197682283587,-14.587652761261,6.88283835740044));
#31809=CARTESIAN_POINT('Ctrl Pts',(-14.7098841141793,-14.1314791418915,
6.84117169073378));
#31810=CARTESIAN_POINT('Ctrl Pts',(-15.5,-13.6753055225219,6.79950502406711));
#31811=CARTESIAN_POINT('Ctrl Pts',(-16.2901158858206,-14.1314791418915,
6.75783835740044));
#31812=CARTESIAN_POINT('Ctrl Pts',(-17.0802317716412,-14.587652761261,6.71617169073377));
#31813=CARTESIAN_POINT('Ctrl Pts',(-17.0802317716412,-15.5000000000001,
6.67450502406711));
#31814=CARTESIAN_POINT('Ctrl Pts',(-17.0802317716412,-16.4123472387391,
6.63283835740044));
#31815=CARTESIAN_POINT('Ctrl Pts',(-16.2901158858206,-16.8685208581087,
6.59117169073377));
#31816=CARTESIAN_POINT('Ctrl Pts',(-15.4999999999999,-17.3246944774782,
6.5495050240671));
#31817=CARTESIAN_POINT('Ctrl Pts',(-14.7098841141793,-16.8685208581087,
6.50783835740044));
#31818=CARTESIAN_POINT('Ctrl Pts',(-13.9197682283587,-16.4123472387391,
6.46617169073377));
#31819=CARTESIAN_POINT('Ctrl Pts',(-13.9197682283587,-15.5,6.4245050240671));
#31820=CARTESIAN_POINT('Ctrl Pts',(-13.9197682283587,-14.587652761261,6.38283835740044));
#31821=CARTESIAN_POINT('Ctrl Pts',(-14.7098841141793,-14.1314791418915,
6.34117169073377));
#31822=CARTESIAN_POINT('Ctrl Pts',(-15.5,-13.6753055225219,6.2995050240671));
#31823=CARTESIAN_POINT('Ctrl Pts',(-16.2901158858206,-14.1314791418915,
6.25783835740044));
#31824=CARTESIAN_POINT('Ctrl Pts',(-17.0802317716412,-14.587652761261,6.21617169073377));
#31825=CARTESIAN_POINT('Ctrl Pts',(-17.0802317716412,-15.5000000000001,
6.1745050240671));
#31826=CARTESIAN_POINT('Ctrl Pts',(-17.0802317716412,-16.4123472387391,
6.13283835740043));
#31827=CARTESIAN_POINT('Ctrl Pts',(-16.2901158858206,-16.8685208581087,
6.09117169073377));
#31828=CARTESIAN_POINT('Ctrl Pts',(-15.4999999999999,-17.3246944774782,
6.0495050240671));
#31829=CARTESIAN_POINT('Ctrl Pts',(-14.7098841141793,-16.8685208581087,
6.00783835740043));
#31830=CARTESIAN_POINT('Ctrl Pts',(-13.9197682283587,-16.4123472387391,
5.96617169073376));
#31831=CARTESIAN_POINT('Ctrl Pts',(-13.9197682283587,-15.5,5.9245050240671));
#31832=CARTESIAN_POINT('Ctrl Pts',(-13.9197682283587,-14.587652761261,5.88283835740043));
#31833=CARTESIAN_POINT('Ctrl Pts',(-14.7098841141793,-14.1314791418915,
5.84117169073376));
#31834=CARTESIAN_POINT('Ctrl Pts',(-15.5,-13.6753055225219,5.79950502406709));
#31835=CARTESIAN_POINT('Ctrl Pts',(-16.2901158858206,-14.1314791418915,
5.75783835740043));
#31836=CARTESIAN_POINT('Ctrl Pts',(-17.0802317716412,-14.587652761261,5.71617169073376));
#31837=CARTESIAN_POINT('Ctrl Pts',(-17.0802317716412,-15.5000000000001,
5.67450502406709));
#31838=CARTESIAN_POINT('Ctrl Pts',(-17.0802317716412,-16.4123472387391,
5.63283835740043));
#31839=CARTESIAN_POINT('Ctrl Pts',(-16.2901158858206,-16.8685208581087,
5.59117169073376));
#31840=CARTESIAN_POINT('Ctrl Pts',(-15.4999999999999,-17.3246944774782,
5.54950502406709));
#31841=CARTESIAN_POINT('Ctrl Pts',(-14.7098841141793,-16.8685208581087,
5.50783835740043));
#31842=CARTESIAN_POINT('Ctrl Pts',(-13.9197682283587,-16.4123472387391,
5.46617169073376));
#31843=CARTESIAN_POINT('Ctrl Pts',(-13.9197682283587,-15.5,5.42450502406709));
#31844=CARTESIAN_POINT('Ctrl Pts',(-13.9197682283587,-14.587652761261,5.38283835740042));
#31845=CARTESIAN_POINT('Ctrl Pts',(-14.7098841141793,-14.1314791418915,
5.34117169073376));
#31846=CARTESIAN_POINT('Ctrl Pts',(-15.5,-13.6753055225219,5.29950502406709));
#31847=CARTESIAN_POINT('Ctrl Pts',(-16.2901158858206,-14.1314791418915,
5.25783835740042));
#31848=CARTESIAN_POINT('Ctrl Pts',(-17.0802317716412,-14.587652761261,5.21617169073375));
#31849=CARTESIAN_POINT('Ctrl Pts',(-17.0802317716412,-15.5000000000001,
5.17450502406709));
#31850=CARTESIAN_POINT('Ctrl Pts',(-17.0802317716412,-16.4123472387391,
5.13283835740042));
#31851=CARTESIAN_POINT('Ctrl Pts',(-16.2901158858206,-16.8685208581087,
5.09117169073375));
#31852=CARTESIAN_POINT('Ctrl Pts',(-15.4999999999999,-17.3246944774782,
5.04950502406708));
#31853=CARTESIAN_POINT('Ctrl Pts',(-14.7098841141793,-16.8685208581087,
5.00783835740042));
#31854=CARTESIAN_POINT('Ctrl Pts',(-13.9197682283587,-16.4123472387391,
4.96617169073375));
#31855=CARTESIAN_POINT('Ctrl Pts',(-13.9197682283587,-15.5,4.92450502406708));
#31856=CARTESIAN_POINT('Ctrl Pts',(-13.9197682283587,-14.587652761261,4.88283835740042));
#31857=CARTESIAN_POINT('Ctrl Pts',(-14.7098841141793,-14.1314791418915,
4.84117169073375));
#31858=CARTESIAN_POINT('Ctrl Pts',(-15.5,-13.6753055225219,4.79950502406708));
#31859=CARTESIAN_POINT('Ctrl Pts',(-16.2901158858206,-14.1314791418915,
4.75783835740041));
#31860=CARTESIAN_POINT('Ctrl Pts',(-17.0802317716412,-14.587652761261,4.71617169073375));
#31861=CARTESIAN_POINT('Ctrl Pts',(-17.0802317716412,-15.5000000000001,
4.67450502406708));
#31862=CARTESIAN_POINT('Ctrl Pts',(-17.0802317716412,-16.4123472387391,
4.63283835740041));
#31863=CARTESIAN_POINT('Ctrl Pts',(-16.2901158858206,-16.8685208581087,
4.59117169073374));
#31864=CARTESIAN_POINT('Ctrl Pts',(-15.4999999999999,-17.3246944774782,
4.54950502406708));
#31865=CARTESIAN_POINT('Ctrl Pts',(-14.7098841141793,-16.8685208581087,
4.50783835740041));
#31866=CARTESIAN_POINT('Ctrl Pts',(-13.9197682283587,-16.4123472387391,
4.46617169073374));
#31867=CARTESIAN_POINT('Ctrl Pts',(-13.9197682283587,-15.5,4.42450502406708));
#31868=CARTESIAN_POINT('Ctrl Pts',(-13.9197682283587,-14.587652761261,4.38283835740041));
#31869=CARTESIAN_POINT('Ctrl Pts',(-14.7098841141793,-14.1314791418915,
4.34117169073374));
#31870=CARTESIAN_POINT('Ctrl Pts',(-15.5,-13.6753055225219,4.29950502406708));
#31871=CARTESIAN_POINT('Ctrl Pts',(-16.2901158858206,-14.1314791418915,
4.25783835740041));
#31872=CARTESIAN_POINT('Ctrl Pts',(-17.0802317716412,-14.587652761261,4.21617169073374));
#31873=CARTESIAN_POINT('Ctrl Pts',(-17.0802317716412,-15.5000000000001,
4.17450502406707));
#31874=CARTESIAN_POINT('Ctrl Pts',(-17.0802317716412,-16.4123472387391,
4.13283835740041));
#31875=CARTESIAN_POINT('Ctrl Pts',(-16.2901158858206,-16.8685208581087,
4.09117169073374));
#31876=CARTESIAN_POINT('Ctrl Pts',(-15.4999999999999,-17.3246944774782,
4.04950502406707));
#31877=CARTESIAN_POINT('Ctrl Pts',(-14.7098841141793,-16.8685208581087,
4.0078383574004));
#31878=CARTESIAN_POINT('Ctrl Pts',(-13.9197682283587,-16.4123472387391,
3.96617169073374));
#31879=CARTESIAN_POINT('Ctrl Pts',(-13.9197682283587,-15.5,3.92450502406707));
#31880=CARTESIAN_POINT('Ctrl Pts',(-13.9197682283587,-14.587652761261,3.8828383574004));
#31881=CARTESIAN_POINT('Ctrl Pts',(-14.7098841141793,-14.1314791418915,
3.84117169073374));
#31882=CARTESIAN_POINT('Ctrl Pts',(-15.5,-13.6753055225219,3.79950502406707));
#31883=CARTESIAN_POINT('Ctrl Pts',(-16.2901158858206,-14.1314791418915,
3.7578383574004));
#31884=CARTESIAN_POINT('Ctrl Pts',(-17.0802317716412,-14.587652761261,3.71617169073373));
#31885=CARTESIAN_POINT('Ctrl Pts',(-17.0802317716412,-15.5000000000001,
3.67450502406707));
#31886=CARTESIAN_POINT('Ctrl Pts',(-17.0802317716412,-16.4123472387391,
3.6328383574004));
#31887=CARTESIAN_POINT('Ctrl Pts',(-16.2901158858206,-16.8685208581087,
3.59117169073373));
#31888=CARTESIAN_POINT('Ctrl Pts',(-15.4999999999999,-17.3246944774782,
3.54950502406707));
#31889=CARTESIAN_POINT('Ctrl Pts',(-14.7098841141793,-16.8685208581087,
3.5078383574004));
#31890=CARTESIAN_POINT('Ctrl Pts',(-13.9197682283587,-16.4123472387391,
3.46617169073373));
#31891=CARTESIAN_POINT('Ctrl Pts',(-13.9197682283587,-15.5,3.42450502406706));
#31892=CARTESIAN_POINT('Ctrl Pts',(-13.9197682283587,-14.587652761261,3.3828383574004));
#31893=CARTESIAN_POINT('Ctrl Pts',(-14.7098841141793,-14.1314791418915,
3.34117169073373));
#31894=CARTESIAN_POINT('Ctrl Pts',(-15.5,-13.6753055225219,3.29950502406706));
#31895=CARTESIAN_POINT('Ctrl Pts',(-16.2901158858206,-14.1314791418915,
3.2578383574004));
#31896=CARTESIAN_POINT('Ctrl Pts',(-17.0802317716412,-14.587652761261,3.21617169073373));
#31897=CARTESIAN_POINT('Ctrl Pts',(-17.0802317716412,-15.5000000000001,
3.17450502406706));
#31898=CARTESIAN_POINT('Ctrl Pts',(-17.0802317716412,-16.4123472387391,
3.13283835740039));
#31899=CARTESIAN_POINT('Ctrl Pts',(-16.2901158858206,-16.8685208581087,
3.09117169073373));
#31900=CARTESIAN_POINT('Ctrl Pts',(-15.4999999999999,-17.3246944774782,
3.04950502406706));
#31901=CARTESIAN_POINT('Ctrl Pts',(-14.7098841141793,-16.8685208581087,
3.00783835740039));
#31902=CARTESIAN_POINT('Ctrl Pts',(-13.9197682283587,-16.4123472387391,
2.96617169073372));
#31903=CARTESIAN_POINT('Ctrl Pts',(-13.9197682283587,-15.5,2.92450502406706));
#31904=CARTESIAN_POINT('Ctrl Pts',(-13.9197682283587,-14.587652761261,2.88283835740039));
#31905=CARTESIAN_POINT('Ctrl Pts',(-14.7098841141793,-14.1314791418915,
2.84117169073372));
#31906=CARTESIAN_POINT('Ctrl Pts',(-15.5,-13.6753055225219,2.79950502406705));
#31907=CARTESIAN_POINT('Ctrl Pts',(-16.2901158858206,-14.1314791418915,
2.75783835740039));
#31908=CARTESIAN_POINT('Ctrl Pts',(-17.0802317716412,-14.587652761261,2.71617169073372));
#31909=CARTESIAN_POINT('Ctrl Pts',(-17.0802317716412,-15.5000000000001,
2.67450502406705));
#31910=CARTESIAN_POINT('Ctrl Pts',(-17.0802317716412,-16.4123472387391,
2.63283835740039));
#31911=CARTESIAN_POINT('Ctrl Pts',(-16.2901158858206,-16.8685208581087,
2.59117169073372));
#31912=CARTESIAN_POINT('Ctrl Pts',(-15.4999999999999,-17.3246944774782,
2.54950502406705));
#31913=CARTESIAN_POINT('Ctrl Pts',(-14.7098841141793,-16.8685208581087,
2.50783835740038));
#31914=CARTESIAN_POINT('Ctrl Pts',(-13.9197682283587,-16.4123472387391,
2.46617169073372));
#31915=CARTESIAN_POINT('Ctrl Pts',(-13.9197682283587,-15.5,2.42450502406705));
#31916=CARTESIAN_POINT('Ctrl Pts',(-13.9197682283587,-14.587652761261,2.38283835740038));
#31917=CARTESIAN_POINT('Ctrl Pts',(-14.7098841141793,-14.1314791418915,
2.34117169073371));
#31918=CARTESIAN_POINT('Ctrl Pts',(-15.5,-13.6753055225219,2.29950502406705));
#31919=CARTESIAN_POINT('Ctrl Pts',(-16.2901158858206,-14.1314791418915,
2.25783835740038));
#31920=CARTESIAN_POINT('Ctrl Pts',(-17.0802317716412,-14.587652761261,2.21617169073371));
#31921=CARTESIAN_POINT('Ctrl Pts',(-17.0802317716412,-15.5000000000001,
2.17450502406705));
#31922=CARTESIAN_POINT('Ctrl Pts',(-17.0802317716412,-16.4123472387391,
2.13283835740038));
#31923=CARTESIAN_POINT('Ctrl Pts',(-16.2901158858206,-16.8685208581087,
2.09117169073371));
#31924=CARTESIAN_POINT('Ctrl Pts',(-15.4999999999999,-17.3246944774782,
2.04950502406705));
#31925=CARTESIAN_POINT('Ctrl Pts',(-14.7098841141793,-16.8685208581087,
2.00783835740038));
#31926=CARTESIAN_POINT('Ctrl Pts',(-13.9197682283587,-16.4123472387391,
1.96617169073371));
#31927=CARTESIAN_POINT('Ctrl Pts',(-13.9197682283587,-15.5,1.92450502406704));
#31928=CARTESIAN_POINT('Ctrl Pts',(-13.9197682283587,-14.587652761261,1.88283835740038));
#31929=CARTESIAN_POINT('Ctrl Pts',(-14.7098841141793,-14.1314791418915,
1.84117169073371));
#31930=CARTESIAN_POINT('Ctrl Pts',(-15.5,-13.6753055225219,1.79950502406704));
#31931=CARTESIAN_POINT('Ctrl Pts',(-16.2901158858206,-14.1314791418915,
1.75783835740037));
#31932=CARTESIAN_POINT('Ctrl Pts',(-17.0802317716412,-14.587652761261,1.71617169073371));
#31933=CARTESIAN_POINT('Ctrl Pts',(-17.0802317716412,-15.5000000000001,
1.67450502406704));
#31934=CARTESIAN_POINT('Ctrl Pts',(-17.0802317716412,-16.4123472387391,
1.63283835740037));
#31935=CARTESIAN_POINT('Ctrl Pts',(-16.2901158858206,-16.8685208581087,
1.59117169073371));
#31936=CARTESIAN_POINT('Ctrl Pts',(-15.4999999999999,-17.3246944774782,
1.54950502406704));
#31937=CARTESIAN_POINT('Ctrl Pts',(-14.7098841141793,-16.8685208581087,
1.50783835740037));
#31938=CARTESIAN_POINT('Ctrl Pts',(-13.9197682283587,-16.4123472387391,
1.4661716907337));
#31939=CARTESIAN_POINT('Ctrl Pts',(-13.9197682283587,-15.5,1.42450502406704));
#31940=CARTESIAN_POINT('Ctrl Pts',(-13.9197682283587,-14.587652761261,1.38283835740037));
#31941=CARTESIAN_POINT('Ctrl Pts',(-14.7098841141793,-14.1314791418915,
1.3411716907337));
#31942=CARTESIAN_POINT('Ctrl Pts',(-15.5,-13.6753055225219,1.29950502406703));
#31943=CARTESIAN_POINT('Ctrl Pts',(-16.2901158858206,-14.1314791418915,
1.25783835740037));
#31944=CARTESIAN_POINT('Ctrl Pts',(-17.0802317716412,-14.587652761261,1.2161716907337));
#31945=CARTESIAN_POINT('Ctrl Pts',(-17.0802317716412,-15.5000000000001,
1.17450502406703));
#31946=CARTESIAN_POINT('Ctrl Pts',(-17.0802317716412,-16.4123472387391,
1.13283835740037));
#31947=CARTESIAN_POINT('Ctrl Pts',(-16.2901158858206,-16.8685208581087,
1.0911716907337));
#31948=CARTESIAN_POINT('Ctrl Pts',(-15.4999999999999,-17.3246944774782,
1.04950502406703));
#31949=CARTESIAN_POINT('Ctrl Pts',(-14.7098841141793,-16.8685208581087,
1.00783835740037));
#31950=CARTESIAN_POINT('Ctrl Pts',(-13.9197682283587,-16.4123472387391,
0.966171690733698));
#31951=CARTESIAN_POINT('Ctrl Pts',(-13.9197682283587,-15.5,0.92450502406703));
#31952=CARTESIAN_POINT('Ctrl Pts',(-13.9197682283587,-14.587652761261,0.882838357400363));
#31953=CARTESIAN_POINT('Ctrl Pts',(-14.7098841141793,-14.1314791418915,
0.841171690733696));
#31954=CARTESIAN_POINT('Ctrl Pts',(-15.5,-13.6753055225219,0.799505024067029));
#31955=CARTESIAN_POINT('Ctrl Pts',(-16.2901158858206,-14.1314791418915,
0.757838357400361));
#31956=CARTESIAN_POINT('Ctrl Pts',(-17.0802317716412,-14.587652761261,0.716171690733694));
#31957=CARTESIAN_POINT('Ctrl Pts',(-17.0802317716412,-15.5000000000001,
0.674505024067027));
#31958=CARTESIAN_POINT('Ctrl Pts',(-17.0802317716412,-16.4123472387391,
0.632838357400359));
#31959=CARTESIAN_POINT('Ctrl Pts',(-16.2901158858206,-16.8685208581087,
0.591171690733692));
#31960=CARTESIAN_POINT('Ctrl Pts',(-15.4999999999999,-17.3246944774782,
0.549505024067025));
#31961=CARTESIAN_POINT('Ctrl Pts',(-14.7098841141793,-16.8685208581087,
0.507838357400358));
#31962=CARTESIAN_POINT('Ctrl Pts',(-13.9197682283587,-16.4123472387391,
0.46617169073369));
#31963=CARTESIAN_POINT('Ctrl Pts',(-13.9197682283587,-15.5,0.424505024067023));
#31964=CARTESIAN_POINT('Ctrl Pts',(-13.9197682283587,-14.587652761261,0.382838357400356));
#31965=CARTESIAN_POINT('Ctrl Pts',(-14.7098841141793,-14.1314791418915,
0.341171690733688));
#31966=CARTESIAN_POINT('Ctrl Pts',(-15.5,-13.6753055225219,0.299505024067021));
#31967=CARTESIAN_POINT('Ctrl Pts',(-16.2901158858206,-14.1314791418915,
0.257838357400354));
#31968=CARTESIAN_POINT('Ctrl Pts',(-17.0802317716412,-14.587652761261,0.216171690733687));
#31969=CARTESIAN_POINT('Ctrl Pts',(-17.0802317716412,-15.5000000000001,
0.174505024067019));
#31970=CARTESIAN_POINT('Ctrl Pts',(-17.0802317716412,-16.4123472387391,
0.132838357400352));
#31971=CARTESIAN_POINT('Ctrl Pts',(-16.2901158858206,-16.8685208581087,
0.0911716907336848));
#31972=CARTESIAN_POINT('Ctrl Pts',(-15.4999999999999,-17.3246944774782,
0.0495050240670175));
#31973=CARTESIAN_POINT('Ctrl Pts',(-14.7098841141793,-16.8685208581087,
0.0078383574003502));
#31974=CARTESIAN_POINT('Ctrl Pts',(-13.9197682283587,-16.4123472387391,
-0.0338283092663171));
#31975=CARTESIAN_POINT('Ctrl Pts',(-13.9197682283587,-15.5,-0.0754949759329844));
#31976=CARTESIAN_POINT('Ctrl Pts',(-13.9197682283587,-14.587652761261,-0.11716164259965));
#31977=CARTESIAN_POINT('Ctrl Pts',(-14.7098841141793,-14.1314791418915,
-0.158828309266317));
#31978=CARTESIAN_POINT('Ctrl Pts',(-15.5,-13.6753055225219,-0.200494975932985));
#31979=CARTESIAN_POINT('Ctrl Pts',(-16.2901158858206,-14.1314791418915,
-0.242161642599652));
#31980=CARTESIAN_POINT('Ctrl Pts',(-17.0802317716412,-14.587652761261,-0.283828309266319));
#31981=CARTESIAN_POINT('Ctrl Pts',(-17.0802317716412,-15.5000000000001,
-0.325494975932986));
#31982=CARTESIAN_POINT('Ctrl Pts',(-17.0802317716412,-16.4123472387391,
-0.367161642599654));
#31983=CARTESIAN_POINT('Ctrl Pts',(-16.2901158858206,-16.8685208581087,
-0.408828309266321));
#31984=CARTESIAN_POINT('Ctrl Pts',(-15.4999999999999,-17.3246944774782,
-0.450494975932988));
#31985=CARTESIAN_POINT('Ctrl Pts',(-14.7098841141793,-16.8685208581087,
-0.492161642599655));
#31986=CARTESIAN_POINT('Ctrl Pts',(-13.9197682283587,-16.4123472387391,
-0.533828309266323));
#31987=CARTESIAN_POINT('Ctrl Pts',(-13.9197682283587,-15.5,-0.57549497593299));
#31988=CARTESIAN_POINT('Ctrl Pts',(-13.9197682283587,-14.587652761261,-0.617161642599657));
#31989=CARTESIAN_POINT('Ctrl Pts',(-14.7098841141793,-14.1314791418915,
-0.658828309266325));
#31990=CARTESIAN_POINT('Ctrl Pts',(-15.5,-13.6753055225219,-0.700494975932992));
#31991=CARTESIAN_POINT('Ctrl Pts',(-16.2901158858206,-14.1314791418915,
-0.742161642599659));
#31992=CARTESIAN_POINT('Ctrl Pts',(-17.0802317716412,-14.587652761261,-0.783828309266327));
#31993=CARTESIAN_POINT('Ctrl Pts',(-17.0802317716412,-15.5000000000001,
-0.825494975932993));
#31994=CARTESIAN_POINT('Ctrl Pts',(-17.0802317716412,-16.4123472387391,
-0.867161642599661));
#31995=CARTESIAN_POINT('Ctrl Pts',(-16.2901158858206,-16.8685208581087,
-0.908828309266328));
#31996=CARTESIAN_POINT('Ctrl Pts',(-15.4999999999999,-17.3246944774782,
-0.950494975932996));
#31997=CARTESIAN_POINT('Ctrl Pts',(-14.7098841141793,-16.8685208581087,
-0.992161642599663));
#31998=CARTESIAN_POINT('Ctrl Pts',(-13.9197682283587,-16.4123472387391,
-1.03382830926633));
#31999=CARTESIAN_POINT('Ctrl Pts',(-13.9197682283587,-15.5,-1.075494975933));
#32000=CARTESIAN_POINT('Ctrl Pts',(-13.9197682283587,-14.587652761261,-1.11716164259966));
#32001=CARTESIAN_POINT('Ctrl Pts',(-14.7098841141793,-14.1314791418915,
-1.15882830926633));
#32002=CARTESIAN_POINT('Ctrl Pts',(-15.5,-13.6753055225219,-1.200494975933));
#32003=CARTESIAN_POINT('Ctrl Pts',(-16.2901158858206,-14.1314791418915,
-1.24216164259967));
#32004=CARTESIAN_POINT('Ctrl Pts',(-17.0802317716412,-14.587652761261,-1.28382830926633));
#32005=CARTESIAN_POINT('Ctrl Pts',(-17.0802317716412,-15.5000000000001,
-1.325494975933));
#32006=CARTESIAN_POINT('Ctrl Pts',(-17.0802317716412,-16.4123472387391,
-1.36716164259967));
#32007=CARTESIAN_POINT('Ctrl Pts',(-16.2901158858206,-16.8685208581087,
-1.40882830926633));
#32008=CARTESIAN_POINT('Ctrl Pts',(-15.4999999999999,-17.3246944774782,
-1.450494975933));
#32009=CARTESIAN_POINT('Ctrl Pts',(-14.7098841141793,-16.8685208581087,
-1.49216164259967));
#32010=CARTESIAN_POINT('Ctrl Pts',(-13.9197682283587,-16.4123472387391,
-1.53382830926634));
#32011=CARTESIAN_POINT('Ctrl Pts',(-13.9197682283587,-15.5,-1.575494975933));
#32012=CARTESIAN_POINT('Ctrl Pts',(-13.9197682283587,-14.587652761261,-1.61716164259967));
#32013=CARTESIAN_POINT('Ctrl Pts',(-14.7098841141793,-14.1314791418915,
-1.65882830926634));
#32014=CARTESIAN_POINT('Ctrl Pts',(-15.5,-13.6753055225219,-1.70049497593301));
#32015=CARTESIAN_POINT('Ctrl Pts',(-16.2901158858206,-14.1314791418915,
-1.74216164259967));
#32016=CARTESIAN_POINT('Ctrl Pts',(-17.0802317716412,-14.587652761261,-1.78382830926634));
#32017=CARTESIAN_POINT('Ctrl Pts',(-17.0802317716412,-15.5000000000001,
-1.82549497593301));
#32018=CARTESIAN_POINT('Ctrl Pts',(-17.0802317716412,-16.4123472387391,
-1.86716164259967));
#32019=CARTESIAN_POINT('Ctrl Pts',(-16.2901158858206,-16.8685208581087,
-1.90882830926634));
#32020=CARTESIAN_POINT('Ctrl Pts',(-15.4999999999999,-17.3246944774782,
-1.95049497593301));
#32021=CARTESIAN_POINT('Ctrl Pts',(-14.7098841141793,-16.8685208581087,
-1.99216164259968));
#32022=CARTESIAN_POINT('Ctrl Pts',(-14.4189893226643,-16.7005726719216,
-2.00750194461187));
#32023=CARTESIAN_POINT('Ctrl Pts',(-14.2215569357651,-16.4288249477778,
-2.02511838079831));
#32024=CARTESIAN_POINT('Ctrl Pts',(-17.4320632938682,-15.5000000000001,
10.971375));
#32025=CARTESIAN_POINT('Ctrl Pts',(-17.4320632938682,-16.6154772628063,
10.9297083333333));
#32026=CARTESIAN_POINT('Ctrl Pts',(-16.4660316469341,-17.1732158942094,
10.8880416666667));
#32027=CARTESIAN_POINT('Ctrl Pts',(-15.4999999999999,-17.7309545256125,
10.846375));
#32028=CARTESIAN_POINT('Ctrl Pts',(-14.5339683530658,-17.1732158942094,
10.8047083333333));
#32029=CARTESIAN_POINT('Ctrl Pts',(-13.5679367061317,-16.6154772628063,
10.7630416666667));
#32030=CARTESIAN_POINT('Ctrl Pts',(-13.5679367061317,-15.5,10.721375));
#32031=CARTESIAN_POINT('Ctrl Pts',(-13.5679367061317,-14.3845227371938,
10.6797083333333));
#32032=CARTESIAN_POINT('Ctrl Pts',(-14.5339683530658,-13.8267841057907,
10.6380416666667));
#32033=CARTESIAN_POINT('Ctrl Pts',(-15.5,-13.2690454743876,10.596375));
#32034=CARTESIAN_POINT('Ctrl Pts',(-16.4660316469341,-13.8267841057907,
10.5547083333333));
#32035=CARTESIAN_POINT('Ctrl Pts',(-17.4320632938682,-14.3845227371938,
10.5130416666667));
#32036=CARTESIAN_POINT('Ctrl Pts',(-17.4320632938682,-15.5000000000001,
10.471375));
#32037=CARTESIAN_POINT('Ctrl Pts',(-17.4320632938682,-16.6154772628063,
10.4297083333333));
#32038=CARTESIAN_POINT('Ctrl Pts',(-16.4660316469341,-17.1732158942094,
10.3880416666667));
#32039=CARTESIAN_POINT('Ctrl Pts',(-15.4999999999999,-17.7309545256125,
10.346375));
#32040=CARTESIAN_POINT('Ctrl Pts',(-14.5339683530658,-17.1732158942094,
10.3047083333333));
#32041=CARTESIAN_POINT('Ctrl Pts',(-13.5679367061317,-16.6154772628063,
10.2630416666667));
#32042=CARTESIAN_POINT('Ctrl Pts',(-13.5679367061317,-15.5,10.221375));
#32043=CARTESIAN_POINT('Ctrl Pts',(-13.5679367061317,-14.3845227371938,
10.1797083333333));
#32044=CARTESIAN_POINT('Ctrl Pts',(-14.5339683530658,-13.8267841057907,
10.1380416666667));
#32045=CARTESIAN_POINT('Ctrl Pts',(-15.5,-13.2690454743876,10.096375));
#32046=CARTESIAN_POINT('Ctrl Pts',(-16.4660316469341,-13.8267841057907,
10.0547083333333));
#32047=CARTESIAN_POINT('Ctrl Pts',(-17.4320632938682,-14.3845227371938,
10.0130416666666));
#32048=CARTESIAN_POINT('Ctrl Pts',(-17.4320632938682,-15.5000000000001,
9.97137499999998));
#32049=CARTESIAN_POINT('Ctrl Pts',(-17.4320632938682,-16.6154772628063,
9.92970833333332));
#32050=CARTESIAN_POINT('Ctrl Pts',(-16.4660316469341,-17.1732158942094,
9.88804166666665));
#32051=CARTESIAN_POINT('Ctrl Pts',(-15.4999999999999,-17.7309545256125,
9.84637499999998));
#32052=CARTESIAN_POINT('Ctrl Pts',(-14.5339683530658,-17.1732158942094,
9.80470833333331));
#32053=CARTESIAN_POINT('Ctrl Pts',(-13.5679367061317,-16.6154772628063,
9.76304166666665));
#32054=CARTESIAN_POINT('Ctrl Pts',(-13.5679367061317,-15.5,9.72137499999998));
#32055=CARTESIAN_POINT('Ctrl Pts',(-13.5679367061317,-14.3845227371938,
9.67970833333331));
#32056=CARTESIAN_POINT('Ctrl Pts',(-14.5339683530658,-13.8267841057907,
9.63804166666664));
#32057=CARTESIAN_POINT('Ctrl Pts',(-15.5,-13.2690454743876,9.59637499999998));
#32058=CARTESIAN_POINT('Ctrl Pts',(-16.4660316469341,-13.8267841057907,
9.55470833333331));
#32059=CARTESIAN_POINT('Ctrl Pts',(-17.4320632938682,-14.3845227371938,
9.51304166666664));
#32060=CARTESIAN_POINT('Ctrl Pts',(-17.4320632938682,-15.5000000000001,
9.47137499999998));
#32061=CARTESIAN_POINT('Ctrl Pts',(-17.4320632938682,-16.6154772628063,
9.42970833333331));
#32062=CARTESIAN_POINT('Ctrl Pts',(-16.4660316469341,-17.1732158942094,
9.38804166666664));
#32063=CARTESIAN_POINT('Ctrl Pts',(-15.4999999999999,-17.7309545256125,
9.34637499999997));
#32064=CARTESIAN_POINT('Ctrl Pts',(-14.5339683530658,-17.1732158942094,
9.30470833333331));
#32065=CARTESIAN_POINT('Ctrl Pts',(-13.5679367061317,-16.6154772628063,
9.26304166666664));
#32066=CARTESIAN_POINT('Ctrl Pts',(-13.5679367061317,-15.5,9.22137499999997));
#32067=CARTESIAN_POINT('Ctrl Pts',(-13.5679367061317,-14.3845227371938,
9.1797083333333));
#32068=CARTESIAN_POINT('Ctrl Pts',(-14.5339683530658,-13.8267841057907,
9.13804166666664));
#32069=CARTESIAN_POINT('Ctrl Pts',(-15.5,-13.2690454743876,9.09637499999997));
#32070=CARTESIAN_POINT('Ctrl Pts',(-16.4660316469341,-13.8267841057907,
9.0547083333333));
#32071=CARTESIAN_POINT('Ctrl Pts',(-17.4320632938682,-14.3845227371938,
9.01304166666664));
#32072=CARTESIAN_POINT('Ctrl Pts',(-17.4320632938682,-15.5000000000001,
8.97137499999997));
#32073=CARTESIAN_POINT('Ctrl Pts',(-17.4320632938682,-16.6154772628063,
8.9297083333333));
#32074=CARTESIAN_POINT('Ctrl Pts',(-16.4660316469341,-17.1732158942094,
8.88804166666663));
#32075=CARTESIAN_POINT('Ctrl Pts',(-15.4999999999999,-17.7309545256125,
8.84637499999997));
#32076=CARTESIAN_POINT('Ctrl Pts',(-14.5339683530658,-17.1732158942094,
8.8047083333333));
#32077=CARTESIAN_POINT('Ctrl Pts',(-13.5679367061317,-16.6154772628063,
8.76304166666663));
#32078=CARTESIAN_POINT('Ctrl Pts',(-13.5679367061317,-15.5,8.72137499999997));
#32079=CARTESIAN_POINT('Ctrl Pts',(-13.5679367061317,-14.3845227371938,
8.6797083333333));
#32080=CARTESIAN_POINT('Ctrl Pts',(-14.5339683530658,-13.8267841057907,
8.63804166666663));
#32081=CARTESIAN_POINT('Ctrl Pts',(-15.5,-13.2690454743876,8.59637499999996));
#32082=CARTESIAN_POINT('Ctrl Pts',(-16.4660316469341,-13.8267841057907,
8.5547083333333));
#32083=CARTESIAN_POINT('Ctrl Pts',(-17.4320632938682,-14.3845227371938,
8.51304166666663));
#32084=CARTESIAN_POINT('Ctrl Pts',(-17.4320632938682,-15.5000000000001,
8.47137499999996));
#32085=CARTESIAN_POINT('Ctrl Pts',(-17.4320632938682,-16.6154772628063,
8.42970833333329));
#32086=CARTESIAN_POINT('Ctrl Pts',(-16.4660316469341,-17.1732158942094,
8.38804166666663));
#32087=CARTESIAN_POINT('Ctrl Pts',(-15.4999999999999,-17.7309545256125,
8.34637499999996));
#32088=CARTESIAN_POINT('Ctrl Pts',(-14.5339683530658,-17.1732158942094,
8.30470833333329));
#32089=CARTESIAN_POINT('Ctrl Pts',(-13.5679367061317,-16.6154772628063,
8.26304166666663));
#32090=CARTESIAN_POINT('Ctrl Pts',(-13.5679367061317,-15.5,8.22137499999996));
#32091=CARTESIAN_POINT('Ctrl Pts',(-13.5679367061317,-14.3845227371938,
8.17970833333329));
#32092=CARTESIAN_POINT('Ctrl Pts',(-14.5339683530658,-13.8267841057907,
8.13804166666662));
#32093=CARTESIAN_POINT('Ctrl Pts',(-15.5,-13.2690454743876,8.09637499999996));
#32094=CARTESIAN_POINT('Ctrl Pts',(-16.4660316469341,-13.8267841057907,
8.05470833333329));
#32095=CARTESIAN_POINT('Ctrl Pts',(-17.4320632938682,-14.3845227371938,
8.01304166666662));
#32096=CARTESIAN_POINT('Ctrl Pts',(-17.4320632938682,-15.5000000000001,
7.97137499999995));
#32097=CARTESIAN_POINT('Ctrl Pts',(-17.4320632938682,-16.6154772628063,
7.92970833333329));
#32098=CARTESIAN_POINT('Ctrl Pts',(-16.4660316469341,-17.1732158942094,
7.88804166666662));
#32099=CARTESIAN_POINT('Ctrl Pts',(-15.4999999999999,-17.7309545256125,
7.84637499999995));
#32100=CARTESIAN_POINT('Ctrl Pts',(-14.5339683530658,-17.1732158942094,
7.80470833333329));
#32101=CARTESIAN_POINT('Ctrl Pts',(-13.5679367061317,-16.6154772628063,
7.76304166666662));
#32102=CARTESIAN_POINT('Ctrl Pts',(-13.5679367061317,-15.5,7.72137499999995));
#32103=CARTESIAN_POINT('Ctrl Pts',(-13.5679367061317,-14.3845227371938,
7.67970833333329));
#32104=CARTESIAN_POINT('Ctrl Pts',(-14.5339683530658,-13.8267841057907,
7.63804166666662));
#32105=CARTESIAN_POINT('Ctrl Pts',(-15.5,-13.2690454743876,7.59637499999995));
#32106=CARTESIAN_POINT('Ctrl Pts',(-16.4660316469341,-13.8267841057907,
7.55470833333328));
#32107=CARTESIAN_POINT('Ctrl Pts',(-17.4320632938682,-14.3845227371938,
7.51304166666662));
#32108=CARTESIAN_POINT('Ctrl Pts',(-17.4320632938682,-15.5000000000001,
7.47137499999995));
#32109=CARTESIAN_POINT('Ctrl Pts',(-17.4320632938682,-16.6154772628063,
7.42970833333328));
#32110=CARTESIAN_POINT('Ctrl Pts',(-16.4660316469341,-17.1732158942094,
7.38804166666661));
#32111=CARTESIAN_POINT('Ctrl Pts',(-15.4999999999999,-17.7309545256125,
7.34637499999995));
#32112=CARTESIAN_POINT('Ctrl Pts',(-14.5339683530658,-17.1732158942094,
7.30470833333328));
#32113=CARTESIAN_POINT('Ctrl Pts',(-13.5679367061317,-16.6154772628063,
7.26304166666661));
#32114=CARTESIAN_POINT('Ctrl Pts',(-13.5679367061317,-15.5,7.22137499999994));
#32115=CARTESIAN_POINT('Ctrl Pts',(-13.5679367061317,-14.3845227371938,
7.17970833333328));
#32116=CARTESIAN_POINT('Ctrl Pts',(-14.5339683530658,-13.8267841057907,
7.13804166666661));
#32117=CARTESIAN_POINT('Ctrl Pts',(-15.5,-13.2690454743876,7.09637499999995));
#32118=CARTESIAN_POINT('Ctrl Pts',(-16.4660316469341,-13.8267841057907,
7.05470833333328));
#32119=CARTESIAN_POINT('Ctrl Pts',(-17.4320632938682,-14.3845227371938,
7.01304166666661));
#32120=CARTESIAN_POINT('Ctrl Pts',(-17.4320632938682,-15.5000000000001,
6.97137499999994));
#32121=CARTESIAN_POINT('Ctrl Pts',(-17.4320632938682,-16.6154772628063,
6.92970833333328));
#32122=CARTESIAN_POINT('Ctrl Pts',(-16.4660316469341,-17.1732158942094,
6.88804166666661));
#32123=CARTESIAN_POINT('Ctrl Pts',(-15.4999999999999,-17.7309545256125,
6.84637499999994));
#32124=CARTESIAN_POINT('Ctrl Pts',(-14.5339683530658,-17.1732158942094,
6.80470833333327));
#32125=CARTESIAN_POINT('Ctrl Pts',(-13.5679367061317,-16.6154772628063,
6.76304166666661));
#32126=CARTESIAN_POINT('Ctrl Pts',(-13.5679367061317,-15.5,6.72137499999994));
#32127=CARTESIAN_POINT('Ctrl Pts',(-13.5679367061317,-14.3845227371938,
6.67970833333327));
#32128=CARTESIAN_POINT('Ctrl Pts',(-14.5339683530658,-13.8267841057907,
6.6380416666666));
#32129=CARTESIAN_POINT('Ctrl Pts',(-15.5,-13.2690454743876,6.59637499999994));
#32130=CARTESIAN_POINT('Ctrl Pts',(-16.4660316469341,-13.8267841057907,
6.55470833333327));
#32131=CARTESIAN_POINT('Ctrl Pts',(-17.4320632938682,-14.3845227371938,
6.5130416666666));
#32132=CARTESIAN_POINT('Ctrl Pts',(-17.4320632938682,-15.5000000000001,
6.47137499999994));
#32133=CARTESIAN_POINT('Ctrl Pts',(-17.4320632938682,-16.6154772628063,
6.42970833333327));
#32134=CARTESIAN_POINT('Ctrl Pts',(-16.4660316469341,-17.1732158942094,
6.3880416666666));
#32135=CARTESIAN_POINT('Ctrl Pts',(-15.4999999999999,-17.7309545256125,
6.34637499999993));
#32136=CARTESIAN_POINT('Ctrl Pts',(-14.5339683530658,-17.1732158942094,
6.30470833333327));
#32137=CARTESIAN_POINT('Ctrl Pts',(-13.5679367061317,-16.6154772628063,
6.2630416666666));
#32138=CARTESIAN_POINT('Ctrl Pts',(-13.5679367061317,-15.5,6.22137499999993));
#32139=CARTESIAN_POINT('Ctrl Pts',(-13.5679367061317,-14.3845227371938,
6.17970833333327));
#32140=CARTESIAN_POINT('Ctrl Pts',(-14.5339683530658,-13.8267841057907,
6.1380416666666));
#32141=CARTESIAN_POINT('Ctrl Pts',(-15.5,-13.2690454743876,6.09637499999993));
#32142=CARTESIAN_POINT('Ctrl Pts',(-16.4660316469341,-13.8267841057907,
6.05470833333326));
#32143=CARTESIAN_POINT('Ctrl Pts',(-17.4320632938682,-14.3845227371938,
6.0130416666666));
#32144=CARTESIAN_POINT('Ctrl Pts',(-17.4320632938682,-15.5000000000001,
5.97137499999993));
#32145=CARTESIAN_POINT('Ctrl Pts',(-17.4320632938682,-16.6154772628063,
5.92970833333326));
#32146=CARTESIAN_POINT('Ctrl Pts',(-16.4660316469341,-17.1732158942094,
5.8880416666666));
#32147=CARTESIAN_POINT('Ctrl Pts',(-15.4999999999999,-17.7309545256125,
5.84637499999993));
#32148=CARTESIAN_POINT('Ctrl Pts',(-14.5339683530658,-17.1732158942094,
5.80470833333326));
#32149=CARTESIAN_POINT('Ctrl Pts',(-13.5679367061317,-16.6154772628063,
5.76304166666659));
#32150=CARTESIAN_POINT('Ctrl Pts',(-13.5679367061317,-15.5,5.72137499999993));
#32151=CARTESIAN_POINT('Ctrl Pts',(-13.5679367061317,-14.3845227371938,
5.67970833333326));
#32152=CARTESIAN_POINT('Ctrl Pts',(-14.5339683530658,-13.8267841057907,
5.63804166666659));
#32153=CARTESIAN_POINT('Ctrl Pts',(-15.5,-13.2690454743876,5.59637499999992));
#32154=CARTESIAN_POINT('Ctrl Pts',(-16.4660316469341,-13.8267841057907,
5.55470833333326));
#32155=CARTESIAN_POINT('Ctrl Pts',(-17.4320632938682,-14.3845227371938,
5.51304166666659));
#32156=CARTESIAN_POINT('Ctrl Pts',(-17.4320632938682,-15.5000000000001,
5.47137499999992));
#32157=CARTESIAN_POINT('Ctrl Pts',(-17.4320632938682,-16.6154772628063,
5.42970833333325));
#32158=CARTESIAN_POINT('Ctrl Pts',(-16.4660316469341,-17.1732158942094,
5.38804166666659));
#32159=CARTESIAN_POINT('Ctrl Pts',(-15.4999999999999,-17.7309545256125,
5.34637499999992));
#32160=CARTESIAN_POINT('Ctrl Pts',(-14.5339683530658,-17.1732158942094,
5.30470833333325));
#32161=CARTESIAN_POINT('Ctrl Pts',(-13.5679367061317,-16.6154772628063,
5.26304166666659));
#32162=CARTESIAN_POINT('Ctrl Pts',(-13.5679367061317,-15.5,5.22137499999992));
#32163=CARTESIAN_POINT('Ctrl Pts',(-13.5679367061317,-14.3845227371938,
5.17970833333325));
#32164=CARTESIAN_POINT('Ctrl Pts',(-14.5339683530658,-13.8267841057907,
5.13804166666659));
#32165=CARTESIAN_POINT('Ctrl Pts',(-15.5,-13.2690454743876,5.09637499999992));
#32166=CARTESIAN_POINT('Ctrl Pts',(-16.4660316469341,-13.8267841057907,
5.05470833333325));
#32167=CARTESIAN_POINT('Ctrl Pts',(-17.4320632938682,-14.3845227371938,
5.01304166666658));
#32168=CARTESIAN_POINT('Ctrl Pts',(-17.4320632938682,-15.5000000000001,
4.97137499999991));
#32169=CARTESIAN_POINT('Ctrl Pts',(-17.4320632938682,-16.6154772628063,
4.92970833333325));
#32170=CARTESIAN_POINT('Ctrl Pts',(-16.4660316469341,-17.1732158942094,
4.88804166666658));
#32171=CARTESIAN_POINT('Ctrl Pts',(-15.4999999999999,-17.7309545256125,
4.84637499999991));
#32172=CARTESIAN_POINT('Ctrl Pts',(-14.5339683530658,-17.1732158942094,
4.80470833333325));
#32173=CARTESIAN_POINT('Ctrl Pts',(-13.5679367061317,-16.6154772628063,
4.76304166666658));
#32174=CARTESIAN_POINT('Ctrl Pts',(-13.5679367061317,-15.5,4.72137499999991));
#32175=CARTESIAN_POINT('Ctrl Pts',(-13.5679367061317,-14.3845227371938,
4.67970833333325));
#32176=CARTESIAN_POINT('Ctrl Pts',(-14.5339683530658,-13.8267841057907,
4.63804166666658));
#32177=CARTESIAN_POINT('Ctrl Pts',(-15.5,-13.2690454743876,4.59637499999991));
#32178=CARTESIAN_POINT('Ctrl Pts',(-16.4660316469341,-13.8267841057907,
4.55470833333324));
#32179=CARTESIAN_POINT('Ctrl Pts',(-17.4320632938682,-14.3845227371938,
4.51304166666658));
#32180=CARTESIAN_POINT('Ctrl Pts',(-17.4320632938682,-15.5000000000001,
4.47137499999991));
#32181=CARTESIAN_POINT('Ctrl Pts',(-17.4320632938682,-16.6154772628063,
4.42970833333324));
#32182=CARTESIAN_POINT('Ctrl Pts',(-16.4660316469341,-17.1732158942094,
4.38804166666657));
#32183=CARTESIAN_POINT('Ctrl Pts',(-15.4999999999999,-17.7309545256125,
4.34637499999991));
#32184=CARTESIAN_POINT('Ctrl Pts',(-14.5339683530658,-17.1732158942094,
4.30470833333324));
#32185=CARTESIAN_POINT('Ctrl Pts',(-13.5679367061317,-16.6154772628063,
4.26304166666657));
#32186=CARTESIAN_POINT('Ctrl Pts',(-13.5679367061317,-15.5,4.22137499999991));
#32187=CARTESIAN_POINT('Ctrl Pts',(-13.5679367061317,-14.3845227371938,
4.17970833333324));
#32188=CARTESIAN_POINT('Ctrl Pts',(-14.5339683530658,-13.8267841057907,
4.13804166666657));
#32189=CARTESIAN_POINT('Ctrl Pts',(-15.5,-13.2690454743876,4.0963749999999));
#32190=CARTESIAN_POINT('Ctrl Pts',(-16.4660316469341,-13.8267841057907,
4.05470833333324));
#32191=CARTESIAN_POINT('Ctrl Pts',(-17.4320632938682,-14.3845227371938,
4.01304166666657));
#32192=CARTESIAN_POINT('Ctrl Pts',(-17.4320632938682,-15.5000000000001,
3.9713749999999));
#32193=CARTESIAN_POINT('Ctrl Pts',(-17.4320632938682,-16.6154772628063,
3.92970833333323));
#32194=CARTESIAN_POINT('Ctrl Pts',(-16.4660316469341,-17.1732158942094,
3.88804166666657));
#32195=CARTESIAN_POINT('Ctrl Pts',(-15.4999999999999,-17.7309545256125,
3.8463749999999));
#32196=CARTESIAN_POINT('Ctrl Pts',(-14.5339683530658,-17.1732158942094,
3.80470833333323));
#32197=CARTESIAN_POINT('Ctrl Pts',(-13.5679367061317,-16.6154772628063,
3.76304166666656));
#32198=CARTESIAN_POINT('Ctrl Pts',(-13.5679367061317,-15.5,3.7213749999999));
#32199=CARTESIAN_POINT('Ctrl Pts',(-13.5679367061317,-14.3845227371938,
3.67970833333323));
#32200=CARTESIAN_POINT('Ctrl Pts',(-14.5339683530658,-13.8267841057907,
3.63804166666656));
#32201=CARTESIAN_POINT('Ctrl Pts',(-15.5,-13.2690454743876,3.5963749999999));
#32202=CARTESIAN_POINT('Ctrl Pts',(-16.4660316469341,-13.8267841057907,
3.55470833333323));
#32203=CARTESIAN_POINT('Ctrl Pts',(-17.4320632938682,-14.3845227371938,
3.51304166666656));
#32204=CARTESIAN_POINT('Ctrl Pts',(-17.4320632938682,-15.5000000000001,
3.4713749999999));
#32205=CARTESIAN_POINT('Ctrl Pts',(-17.4320632938682,-16.6154772628063,
3.42970833333323));
#32206=CARTESIAN_POINT('Ctrl Pts',(-16.4660316469341,-17.1732158942094,
3.38804166666656));
#32207=CARTESIAN_POINT('Ctrl Pts',(-15.4999999999999,-17.7309545256125,
3.34637499999989));
#32208=CARTESIAN_POINT('Ctrl Pts',(-14.5339683530658,-17.1732158942094,
3.30470833333323));
#32209=CARTESIAN_POINT('Ctrl Pts',(-13.5679367061317,-16.6154772628063,
3.26304166666656));
#32210=CARTESIAN_POINT('Ctrl Pts',(-13.5679367061317,-15.5,3.22137499999989));
#32211=CARTESIAN_POINT('Ctrl Pts',(-13.5679367061317,-14.3845227371938,
3.17970833333322));
#32212=CARTESIAN_POINT('Ctrl Pts',(-14.5339683530658,-13.8267841057907,
3.13804166666656));
#32213=CARTESIAN_POINT('Ctrl Pts',(-15.5,-13.2690454743876,3.09637499999989));
#32214=CARTESIAN_POINT('Ctrl Pts',(-16.4660316469341,-13.8267841057907,
3.05470833333322));
#32215=CARTESIAN_POINT('Ctrl Pts',(-17.4320632938682,-14.3845227371938,
3.01304166666656));
#32216=CARTESIAN_POINT('Ctrl Pts',(-17.4320632938682,-15.5000000000001,
2.97137499999989));
#32217=CARTESIAN_POINT('Ctrl Pts',(-17.4320632938682,-16.6154772628063,
2.92970833333322));
#32218=CARTESIAN_POINT('Ctrl Pts',(-16.4660316469341,-17.1732158942094,
2.88804166666655));
#32219=CARTESIAN_POINT('Ctrl Pts',(-15.4999999999999,-17.7309545256125,
2.84637499999989));
#32220=CARTESIAN_POINT('Ctrl Pts',(-14.5339683530658,-17.1732158942094,
2.80470833333322));
#32221=CARTESIAN_POINT('Ctrl Pts',(-13.5679367061317,-16.6154772628063,
2.76304166666655));
#32222=CARTESIAN_POINT('Ctrl Pts',(-13.5679367061317,-15.5,2.72137499999989));
#32223=CARTESIAN_POINT('Ctrl Pts',(-13.5679367061317,-14.3845227371938,
2.67970833333322));
#32224=CARTESIAN_POINT('Ctrl Pts',(-14.5339683530658,-13.8267841057907,
2.63804166666655));
#32225=CARTESIAN_POINT('Ctrl Pts',(-15.5,-13.2690454743876,2.59637499999988));
#32226=CARTESIAN_POINT('Ctrl Pts',(-16.4660316469341,-13.8267841057907,
2.55470833333322));
#32227=CARTESIAN_POINT('Ctrl Pts',(-17.4320632938682,-14.3845227371938,
2.51304166666655));
#32228=CARTESIAN_POINT('Ctrl Pts',(-17.4320632938682,-15.5000000000001,
2.47137499999988));
#32229=CARTESIAN_POINT('Ctrl Pts',(-17.4320632938682,-16.6154772628063,
2.42970833333321));
#32230=CARTESIAN_POINT('Ctrl Pts',(-16.4660316469341,-17.1732158942094,
2.38804166666655));
#32231=CARTESIAN_POINT('Ctrl Pts',(-15.4999999999999,-17.7309545256125,
2.34637499999988));
#32232=CARTESIAN_POINT('Ctrl Pts',(-14.5339683530658,-17.1732158942094,
2.30470833333321));
#32233=CARTESIAN_POINT('Ctrl Pts',(-13.5679367061317,-16.6154772628063,
2.26304166666655));
#32234=CARTESIAN_POINT('Ctrl Pts',(-13.5679367061317,-15.5,2.22137499999988));
#32235=CARTESIAN_POINT('Ctrl Pts',(-13.5679367061317,-14.3845227371938,
2.17970833333321));
#32236=CARTESIAN_POINT('Ctrl Pts',(-14.5339683530658,-13.8267841057907,
2.13804166666654));
#32237=CARTESIAN_POINT('Ctrl Pts',(-15.5,-13.2690454743876,2.09637499999988));
#32238=CARTESIAN_POINT('Ctrl Pts',(-16.4660316469341,-13.8267841057907,
2.05470833333321));
#32239=CARTESIAN_POINT('Ctrl Pts',(-17.4320632938682,-14.3845227371938,
2.01304166666654));
#32240=CARTESIAN_POINT('Ctrl Pts',(-17.4320632938682,-15.5000000000001,
1.97137499999988));
#32241=CARTESIAN_POINT('Ctrl Pts',(-17.4320632938682,-16.6154772628063,
1.92970833333321));
#32242=CARTESIAN_POINT('Ctrl Pts',(-16.4660316469341,-17.1732158942094,
1.88804166666654));
#32243=CARTESIAN_POINT('Ctrl Pts',(-15.4999999999999,-17.7309545256125,
1.84637499999987));
#32244=CARTESIAN_POINT('Ctrl Pts',(-14.5339683530658,-17.1732158942094,
1.80470833333321));
#32245=CARTESIAN_POINT('Ctrl Pts',(-13.5679367061317,-16.6154772628063,
1.76304166666654));
#32246=CARTESIAN_POINT('Ctrl Pts',(-13.5679367061317,-15.5,1.72137499999987));
#32247=CARTESIAN_POINT('Ctrl Pts',(-13.5679367061317,-14.3845227371938,
1.67970833333321));
#32248=CARTESIAN_POINT('Ctrl Pts',(-14.5339683530658,-13.8267841057907,
1.63804166666654));
#32249=CARTESIAN_POINT('Ctrl Pts',(-15.5,-13.2690454743876,1.59637499999987));
#32250=CARTESIAN_POINT('Ctrl Pts',(-16.4660316469341,-13.8267841057907,
1.5547083333332));
#32251=CARTESIAN_POINT('Ctrl Pts',(-17.4320632938682,-14.3845227371938,
1.51304166666654));
#32252=CARTESIAN_POINT('Ctrl Pts',(-17.4320632938682,-15.5000000000001,
1.47137499999987));
#32253=CARTESIAN_POINT('Ctrl Pts',(-17.4320632938682,-16.6154772628063,
1.4297083333332));
#32254=CARTESIAN_POINT('Ctrl Pts',(-16.4660316469341,-17.1732158942094,
1.38804166666653));
#32255=CARTESIAN_POINT('Ctrl Pts',(-15.4999999999999,-17.7309545256125,
1.34637499999987));
#32256=CARTESIAN_POINT('Ctrl Pts',(-14.5339683530658,-17.1732158942094,
1.3047083333332));
#32257=CARTESIAN_POINT('Ctrl Pts',(-13.5679367061317,-16.6154772628063,
1.26304166666653));
#32258=CARTESIAN_POINT('Ctrl Pts',(-13.5679367061317,-15.5,1.22137499999987));
#32259=CARTESIAN_POINT('Ctrl Pts',(-13.5679367061317,-14.3845227371938,
1.1797083333332));
#32260=CARTESIAN_POINT('Ctrl Pts',(-14.5339683530658,-13.8267841057907,
1.13804166666653));
#32261=CARTESIAN_POINT('Ctrl Pts',(-15.5,-13.2690454743876,1.09637499999986));
#32262=CARTESIAN_POINT('Ctrl Pts',(-16.4660316469341,-13.8267841057907,
1.0547083333332));
#32263=CARTESIAN_POINT('Ctrl Pts',(-17.4320632938682,-14.3845227371938,
1.01304166666653));
#32264=CARTESIAN_POINT('Ctrl Pts',(-17.4320632938682,-15.5000000000001,
0.971374999999861));
#32265=CARTESIAN_POINT('Ctrl Pts',(-17.4320632938682,-16.6154772628063,
0.929708333333194));
#32266=CARTESIAN_POINT('Ctrl Pts',(-16.4660316469341,-17.1732158942094,
0.888041666666528));
#32267=CARTESIAN_POINT('Ctrl Pts',(-15.4999999999999,-17.7309545256125,
0.846374999999861));
#32268=CARTESIAN_POINT('Ctrl Pts',(-14.5339683530658,-17.1732158942094,
0.804708333333194));
#32269=CARTESIAN_POINT('Ctrl Pts',(-13.5679367061317,-16.6154772628063,
0.763041666666526));
#32270=CARTESIAN_POINT('Ctrl Pts',(-13.5679367061317,-15.5,0.721374999999859));
#32271=CARTESIAN_POINT('Ctrl Pts',(-13.5679367061317,-14.3845227371938,
0.679708333333192));
#32272=CARTESIAN_POINT('Ctrl Pts',(-14.5339683530658,-13.8267841057907,
0.638041666666525));
#32273=CARTESIAN_POINT('Ctrl Pts',(-15.5,-13.2690454743876,0.596374999999858));
#32274=CARTESIAN_POINT('Ctrl Pts',(-16.4660316469341,-13.8267841057907,
0.55470833333319));
#32275=CARTESIAN_POINT('Ctrl Pts',(-17.4320632938682,-14.3845227371938,
0.513041666666523));
#32276=CARTESIAN_POINT('Ctrl Pts',(-17.4320632938682,-15.5000000000001,
0.471374999999856));
#32277=CARTESIAN_POINT('Ctrl Pts',(-17.4320632938682,-16.6154772628063,
0.429708333333188));
#32278=CARTESIAN_POINT('Ctrl Pts',(-16.4660316469341,-17.1732158942094,
0.388041666666521));
#32279=CARTESIAN_POINT('Ctrl Pts',(-15.4999999999999,-17.7309545256125,
0.346374999999854));
#32280=CARTESIAN_POINT('Ctrl Pts',(-14.5339683530658,-17.1732158942094,
0.304708333333186));
#32281=CARTESIAN_POINT('Ctrl Pts',(-13.5679367061317,-16.6154772628063,
0.263041666666519));
#32282=CARTESIAN_POINT('Ctrl Pts',(-13.5679367061317,-15.5,0.221374999999852));
#32283=CARTESIAN_POINT('Ctrl Pts',(-13.5679367061317,-14.3845227371938,
0.179708333333185));
#32284=CARTESIAN_POINT('Ctrl Pts',(-14.5339683530658,-13.8267841057907,
0.138041666666517));
#32285=CARTESIAN_POINT('Ctrl Pts',(-15.5,-13.2690454743876,0.0963749999998501));
#32286=CARTESIAN_POINT('Ctrl Pts',(-16.4660316469341,-13.8267841057907,
0.0547083333331828));
#32287=CARTESIAN_POINT('Ctrl Pts',(-17.4320632938682,-14.3845227371938,
0.0130416666665155));
#32288=CARTESIAN_POINT('Ctrl Pts',(-17.4320632938682,-15.5000000000001,
-0.0286250000001518));
#32289=CARTESIAN_POINT('Ctrl Pts',(-17.4320632938682,-16.6154772628063,
-0.0702916666668191));
#32290=CARTESIAN_POINT('Ctrl Pts',(-16.4660316469341,-17.1732158942094,
-0.111958333333486));
#32291=CARTESIAN_POINT('Ctrl Pts',(-15.4999999999999,-17.7309545256125,
-0.153625000000154));
#32292=CARTESIAN_POINT('Ctrl Pts',(-14.5339683530658,-17.1732158942094,
-0.195291666666821));
#32293=CARTESIAN_POINT('Ctrl Pts',(-13.5679367061317,-16.6154772628063,
-0.236958333333488));
#32294=CARTESIAN_POINT('Ctrl Pts',(-13.5679367061317,-15.5,-0.278625000000155));
#32295=CARTESIAN_POINT('Ctrl Pts',(-13.5679367061317,-14.3845227371938,
-0.320291666666821));
#32296=CARTESIAN_POINT('Ctrl Pts',(-14.5339683530658,-13.8267841057907,
-0.361958333333488));
#32297=CARTESIAN_POINT('Ctrl Pts',(-15.5,-13.2690454743876,-0.403625000000156));
#32298=CARTESIAN_POINT('Ctrl Pts',(-16.4660316469341,-13.8267841057907,
-0.445291666666823));
#32299=CARTESIAN_POINT('Ctrl Pts',(-17.4320632938682,-14.3845227371938,
-0.48695833333349));
#32300=CARTESIAN_POINT('Ctrl Pts',(-17.4320632938682,-15.5000000000001,
-0.528625000000157));
#32301=CARTESIAN_POINT('Ctrl Pts',(-17.4320632938682,-16.6154772628063,
-0.570291666666825));
#32302=CARTESIAN_POINT('Ctrl Pts',(-16.4660316469341,-17.1732158942094,
-0.611958333333492));
#32303=CARTESIAN_POINT('Ctrl Pts',(-15.4999999999999,-17.7309545256125,
-0.653625000000159));
#32304=CARTESIAN_POINT('Ctrl Pts',(-14.5339683530658,-17.1732158942094,
-0.695291666666827));
#32305=CARTESIAN_POINT('Ctrl Pts',(-13.5679367061317,-16.6154772628063,
-0.736958333333494));
#32306=CARTESIAN_POINT('Ctrl Pts',(-13.5679367061317,-15.5,-0.778625000000161));
#32307=CARTESIAN_POINT('Ctrl Pts',(-13.5679367061317,-14.3845227371938,
-0.820291666666829));
#32308=CARTESIAN_POINT('Ctrl Pts',(-14.5339683530658,-13.8267841057907,
-0.861958333333496));
#32309=CARTESIAN_POINT('Ctrl Pts',(-15.5,-13.2690454743876,-0.903625000000163));
#32310=CARTESIAN_POINT('Ctrl Pts',(-16.4660316469341,-13.8267841057907,
-0.94529166666683));
#32311=CARTESIAN_POINT('Ctrl Pts',(-17.4320632938682,-14.3845227371938,
-0.986958333333498));
#32312=CARTESIAN_POINT('Ctrl Pts',(-17.4320632938682,-15.5000000000001,
-1.02862500000016));
#32313=CARTESIAN_POINT('Ctrl Pts',(-17.4320632938682,-16.6154772628063,
-1.07029166666683));
#32314=CARTESIAN_POINT('Ctrl Pts',(-16.4660316469341,-17.1732158942094,
-1.1119583333335));
#32315=CARTESIAN_POINT('Ctrl Pts',(-15.4999999999999,-17.7309545256125,
-1.15362500000017));
#32316=CARTESIAN_POINT('Ctrl Pts',(-14.5339683530658,-17.1732158942094,
-1.19529166666683));
#32317=CARTESIAN_POINT('Ctrl Pts',(-13.5679367061317,-16.6154772628063,
-1.2369583333335));
#32318=CARTESIAN_POINT('Ctrl Pts',(-13.5679367061317,-15.5,-1.27862500000017));
#32319=CARTESIAN_POINT('Ctrl Pts',(-13.5679367061317,-14.3845227371938,
-1.32029166666684));
#32320=CARTESIAN_POINT('Ctrl Pts',(-14.5339683530658,-13.8267841057907,
-1.3619583333335));
#32321=CARTESIAN_POINT('Ctrl Pts',(-15.5,-13.2690454743876,-1.40362500000017));
#32322=CARTESIAN_POINT('Ctrl Pts',(-16.4660316469341,-13.8267841057907,
-1.44529166666684));
#32323=CARTESIAN_POINT('Ctrl Pts',(-17.4320632938682,-14.3845227371938,
-1.4869583333335));
#32324=CARTESIAN_POINT('Ctrl Pts',(-17.4320632938682,-15.5000000000001,
-1.52862500000017));
#32325=CARTESIAN_POINT('Ctrl Pts',(-17.4320632938682,-16.6154772628063,
-1.57029166666684));
#32326=CARTESIAN_POINT('Ctrl Pts',(-16.4660316469341,-17.1732158942094,
-1.61195833333351));
#32327=CARTESIAN_POINT('Ctrl Pts',(-15.4999999999999,-17.7309545256125,
-1.65362500000017));
#32328=CARTESIAN_POINT('Ctrl Pts',(-14.5339683530658,-17.1732158942094,
-1.69529166666684));
#32329=CARTESIAN_POINT('Ctrl Pts',(-13.5679367061317,-16.6154772628063,
-1.73695833333351));
#32330=CARTESIAN_POINT('Ctrl Pts',(-13.5679367061317,-15.5,-1.77862500000017));
#32331=CARTESIAN_POINT('Ctrl Pts',(-13.5679367061317,-14.3845227371938,
-1.82029166666684));
#32332=CARTESIAN_POINT('Ctrl Pts',(-14.5339683530658,-13.8267841057907,
-1.86195833333351));
#32333=CARTESIAN_POINT('Ctrl Pts',(-15.5,-13.2690454743876,-1.90362500000018));
#32334=CARTESIAN_POINT('Ctrl Pts',(-16.4660316469341,-13.8267841057907,
-1.94529166666684));
#32335=CARTESIAN_POINT('Ctrl Pts',(-17.4320632938682,-14.3845227371938,
-1.98695833333351));
#32336=CARTESIAN_POINT('Ctrl Pts',(-17.4320632938682,-15.5000000000001,
-2.02862500000018));
#32337=CARTESIAN_POINT('Ctrl Pts',(-17.4320632938682,-16.6154772628063,
-2.07029166666685));
#32338=CARTESIAN_POINT('Ctrl Pts',(-16.4660316469341,-17.1732158942094,
-2.11195833333351));
#32339=CARTESIAN_POINT('Ctrl Pts',(-15.4999999999999,-17.7309545256125,
-2.15362500000018));
#32340=CARTESIAN_POINT('Ctrl Pts',(-14.5339683530658,-17.1732158942094,
-2.19529166666685));
#32341=CARTESIAN_POINT('Ctrl Pts',(-14.1783071398503,-16.9678747970191,
-2.21063196867905));
#32342=CARTESIAN_POINT('Ctrl Pts',(-13.9369173167913,-16.6356236599184,
-2.22824840486548));
#32343=CARTESIAN_POINT('',(-14.2215513317126,-16.4288320706154,-2.0251230503213));
#32344=CARTESIAN_POINT('Ctrl Pts',(-13.9406917842496,-15.2436450846258,
10.4122404735808));
#32345=CARTESIAN_POINT('Ctrl Pts',(-14.0620451873461,-14.5054990725558,
10.3753299573543));
#32346=CARTESIAN_POINT('Ctrl Pts',(-14.7098797632095,-14.1314716057907,
10.3411666666667));
#32347=CARTESIAN_POINT('Ctrl Pts',(-15.5,-13.6752954743876,10.2995));
#32348=CARTESIAN_POINT('Ctrl Pts',(-16.2901202367904,-14.1314716057907,
10.2578333333333));
#32349=CARTESIAN_POINT('Ctrl Pts',(-17.0802404735808,-14.5876477371938,
10.2161666666667));
#32350=CARTESIAN_POINT('Ctrl Pts',(-17.0802404735808,-15.5000000000001,
10.1745));
#32351=CARTESIAN_POINT('Ctrl Pts',(-17.0802404735808,-16.4123522628063,
10.1328333333333));
#32352=CARTESIAN_POINT('Ctrl Pts',(-16.2901202367904,-16.8685283942094,
10.0911666666667));
#32353=CARTESIAN_POINT('Ctrl Pts',(-15.4999999999999,-17.3247045256125,
10.0495));
#32354=CARTESIAN_POINT('Ctrl Pts',(-14.7098797632095,-16.8685283942094,
10.0078333333333));
#32355=CARTESIAN_POINT('Ctrl Pts',(-13.9197595264191,-16.4123522628063,
9.96616666666665));
#32356=CARTESIAN_POINT('Ctrl Pts',(-13.9197595264191,-15.5,9.92449999999998));
#32357=CARTESIAN_POINT('Ctrl Pts',(-13.9197595264191,-14.5876477371938,
9.88283333333331));
#32358=CARTESIAN_POINT('Ctrl Pts',(-14.7098797632095,-14.1314716057907,
9.84116666666665));
#32359=CARTESIAN_POINT('Ctrl Pts',(-15.5,-13.6752954743876,9.79949999999998));
#32360=CARTESIAN_POINT('Ctrl Pts',(-16.2901202367904,-14.1314716057907,
9.75783333333331));
#32361=CARTESIAN_POINT('Ctrl Pts',(-17.0802404735808,-14.5876477371938,
9.71616666666665));
#32362=CARTESIAN_POINT('Ctrl Pts',(-17.0802404735808,-15.5000000000001,
9.67449999999998));
#32363=CARTESIAN_POINT('Ctrl Pts',(-17.0802404735808,-16.4123522628063,
9.63283333333331));
#32364=CARTESIAN_POINT('Ctrl Pts',(-16.2901202367904,-16.8685283942094,
9.59116666666664));
#32365=CARTESIAN_POINT('Ctrl Pts',(-15.4999999999999,-17.3247045256125,
9.54949999999998));
#32366=CARTESIAN_POINT('Ctrl Pts',(-14.7098797632095,-16.8685283942094,
9.50783333333331));
#32367=CARTESIAN_POINT('Ctrl Pts',(-13.9197595264191,-16.4123522628063,
9.46616666666664));
#32368=CARTESIAN_POINT('Ctrl Pts',(-13.9197595264191,-15.5,9.42449999999998));
#32369=CARTESIAN_POINT('Ctrl Pts',(-13.9197595264191,-14.5876477371938,
9.38283333333331));
#32370=CARTESIAN_POINT('Ctrl Pts',(-14.7098797632095,-14.1314716057907,
9.34116666666664));
#32371=CARTESIAN_POINT('Ctrl Pts',(-15.5,-13.6752954743876,9.29949999999997));
#32372=CARTESIAN_POINT('Ctrl Pts',(-16.2901202367904,-14.1314716057907,
9.25783333333331));
#32373=CARTESIAN_POINT('Ctrl Pts',(-17.0802404735808,-14.5876477371938,
9.21616666666664));
#32374=CARTESIAN_POINT('Ctrl Pts',(-17.0802404735808,-15.5000000000001,
9.17449999999997));
#32375=CARTESIAN_POINT('Ctrl Pts',(-17.0802404735808,-16.4123522628063,
9.13283333333331));
#32376=CARTESIAN_POINT('Ctrl Pts',(-16.2901202367904,-16.8685283942094,
9.09116666666664));
#32377=CARTESIAN_POINT('Ctrl Pts',(-15.4999999999999,-17.3247045256125,
9.04949999999997));
#32378=CARTESIAN_POINT('Ctrl Pts',(-14.7098797632095,-16.8685283942094,
9.0078333333333));
#32379=CARTESIAN_POINT('Ctrl Pts',(-13.9197595264191,-16.4123522628063,
8.96616666666664));
#32380=CARTESIAN_POINT('Ctrl Pts',(-13.9197595264191,-15.5,8.92449999999997));
#32381=CARTESIAN_POINT('Ctrl Pts',(-13.9197595264191,-14.5876477371938,
8.8828333333333));
#32382=CARTESIAN_POINT('Ctrl Pts',(-14.7098797632095,-14.1314716057907,
8.84116666666664));
#32383=CARTESIAN_POINT('Ctrl Pts',(-15.5,-13.6752954743876,8.79949999999997));
#32384=CARTESIAN_POINT('Ctrl Pts',(-16.2901202367904,-14.1314716057907,
8.7578333333333));
#32385=CARTESIAN_POINT('Ctrl Pts',(-17.0802404735808,-14.5876477371938,
8.71616666666663));
#32386=CARTESIAN_POINT('Ctrl Pts',(-17.0802404735808,-15.5000000000001,
8.67449999999997));
#32387=CARTESIAN_POINT('Ctrl Pts',(-17.0802404735808,-16.4123522628063,
8.6328333333333));
#32388=CARTESIAN_POINT('Ctrl Pts',(-16.2901202367904,-16.8685283942094,
8.59116666666663));
#32389=CARTESIAN_POINT('Ctrl Pts',(-15.4999999999999,-17.3247045256125,
8.54949999999996));
#32390=CARTESIAN_POINT('Ctrl Pts',(-14.7098797632095,-16.8685283942094,
8.50783333333329));
#32391=CARTESIAN_POINT('Ctrl Pts',(-13.9197595264191,-16.4123522628063,
8.46616666666663));
#32392=CARTESIAN_POINT('Ctrl Pts',(-13.9197595264191,-15.5,8.42449999999996));
#32393=CARTESIAN_POINT('Ctrl Pts',(-13.9197595264191,-14.5876477371938,
8.38283333333329));
#32394=CARTESIAN_POINT('Ctrl Pts',(-14.7098797632095,-14.1314716057907,
8.34116666666663));
#32395=CARTESIAN_POINT('Ctrl Pts',(-15.5,-13.6752954743876,8.29949999999996));
#32396=CARTESIAN_POINT('Ctrl Pts',(-16.2901202367904,-14.1314716057907,
8.25783333333329));
#32397=CARTESIAN_POINT('Ctrl Pts',(-17.0802404735808,-14.5876477371938,
8.21616666666663));
#32398=CARTESIAN_POINT('Ctrl Pts',(-17.0802404735808,-15.5000000000001,
8.17449999999996));
#32399=CARTESIAN_POINT('Ctrl Pts',(-17.0802404735808,-16.4123522628063,
8.13283333333329));
#32400=CARTESIAN_POINT('Ctrl Pts',(-16.2901202367904,-16.8685283942094,
8.09116666666663));
#32401=CARTESIAN_POINT('Ctrl Pts',(-15.4999999999999,-17.3247045256125,
8.04949999999996));
#32402=CARTESIAN_POINT('Ctrl Pts',(-14.7098797632095,-16.8685283942094,
8.00783333333329));
#32403=CARTESIAN_POINT('Ctrl Pts',(-13.9197595264191,-16.4123522628063,
7.96616666666662));
#32404=CARTESIAN_POINT('Ctrl Pts',(-13.9197595264191,-15.5,7.92449999999996));
#32405=CARTESIAN_POINT('Ctrl Pts',(-13.9197595264191,-14.5876477371938,
7.88283333333329));
#32406=CARTESIAN_POINT('Ctrl Pts',(-14.7098797632095,-14.1314716057907,
7.84116666666662));
#32407=CARTESIAN_POINT('Ctrl Pts',(-15.5,-13.6752954743876,7.79949999999995));
#32408=CARTESIAN_POINT('Ctrl Pts',(-16.2901202367904,-14.1314716057907,
7.75783333333329));
#32409=CARTESIAN_POINT('Ctrl Pts',(-17.0802404735808,-14.5876477371938,
7.71616666666662));
#32410=CARTESIAN_POINT('Ctrl Pts',(-17.0802404735808,-15.5000000000001,
7.67449999999995));
#32411=CARTESIAN_POINT('Ctrl Pts',(-17.0802404735808,-16.4123522628063,
7.63283333333328));
#32412=CARTESIAN_POINT('Ctrl Pts',(-16.2901202367904,-16.8685283942094,
7.59116666666662));
#32413=CARTESIAN_POINT('Ctrl Pts',(-15.4999999999999,-17.3247045256125,
7.54949999999995));
#32414=CARTESIAN_POINT('Ctrl Pts',(-14.7098797632095,-16.8685283942094,
7.50783333333328));
#32415=CARTESIAN_POINT('Ctrl Pts',(-13.9197595264191,-16.4123522628063,
7.46616666666662));
#32416=CARTESIAN_POINT('Ctrl Pts',(-13.9197595264191,-15.5,7.42449999999995));
#32417=CARTESIAN_POINT('Ctrl Pts',(-13.9197595264191,-14.5876477371938,
7.38283333333328));
#32418=CARTESIAN_POINT('Ctrl Pts',(-14.7098797632095,-14.1314716057907,
7.34116666666661));
#32419=CARTESIAN_POINT('Ctrl Pts',(-15.5,-13.6752954743876,7.29949999999995));
#32420=CARTESIAN_POINT('Ctrl Pts',(-16.2901202367904,-14.1314716057907,
7.25783333333328));
#32421=CARTESIAN_POINT('Ctrl Pts',(-17.0802404735808,-14.5876477371938,
7.21616666666661));
#32422=CARTESIAN_POINT('Ctrl Pts',(-17.0802404735808,-15.5000000000001,
7.17449999999995));
#32423=CARTESIAN_POINT('Ctrl Pts',(-17.0802404735808,-16.4123522628063,
7.13283333333328));
#32424=CARTESIAN_POINT('Ctrl Pts',(-16.2901202367904,-16.8685283942094,
7.09116666666661));
#32425=CARTESIAN_POINT('Ctrl Pts',(-15.4999999999999,-17.3247045256125,
7.04949999999994));
#32426=CARTESIAN_POINT('Ctrl Pts',(-14.7098797632095,-16.8685283942094,
7.00783333333328));
#32427=CARTESIAN_POINT('Ctrl Pts',(-13.9197595264191,-16.4123522628063,
6.96616666666661));
#32428=CARTESIAN_POINT('Ctrl Pts',(-13.9197595264191,-15.5,6.92449999999994));
#32429=CARTESIAN_POINT('Ctrl Pts',(-13.9197595264191,-14.5876477371938,
6.88283333333327));
#32430=CARTESIAN_POINT('Ctrl Pts',(-14.7098797632095,-14.1314716057907,
6.84116666666661));
#32431=CARTESIAN_POINT('Ctrl Pts',(-15.5,-13.6752954743876,6.79949999999994));
#32432=CARTESIAN_POINT('Ctrl Pts',(-16.2901202367904,-14.1314716057907,
6.75783333333327));
#32433=CARTESIAN_POINT('Ctrl Pts',(-17.0802404735808,-14.5876477371938,
6.71616666666661));
#32434=CARTESIAN_POINT('Ctrl Pts',(-17.0802404735808,-15.5000000000001,
6.67449999999994));
#32435=CARTESIAN_POINT('Ctrl Pts',(-17.0802404735808,-16.4123522628063,
6.63283333333327));
#32436=CARTESIAN_POINT('Ctrl Pts',(-16.2901202367904,-16.8685283942094,
6.59116666666661));
#32437=CARTESIAN_POINT('Ctrl Pts',(-15.4999999999999,-17.3247045256125,
6.54949999999994));
#32438=CARTESIAN_POINT('Ctrl Pts',(-14.7098797632095,-16.8685283942094,
6.50783333333327));
#32439=CARTESIAN_POINT('Ctrl Pts',(-13.9197595264191,-16.4123522628063,
6.4661666666666));
#32440=CARTESIAN_POINT('Ctrl Pts',(-13.9197595264191,-15.5,6.42449999999994));
#32441=CARTESIAN_POINT('Ctrl Pts',(-13.9197595264191,-14.5876477371938,
6.38283333333327));
#32442=CARTESIAN_POINT('Ctrl Pts',(-14.7098797632095,-14.1314716057907,
6.3411666666666));
#32443=CARTESIAN_POINT('Ctrl Pts',(-15.5,-13.6752954743876,6.29949999999993));
#32444=CARTESIAN_POINT('Ctrl Pts',(-16.2901202367904,-14.1314716057907,
6.25783333333327));
#32445=CARTESIAN_POINT('Ctrl Pts',(-17.0802404735808,-14.5876477371938,
6.2161666666666));
#32446=CARTESIAN_POINT('Ctrl Pts',(-17.0802404735808,-15.5000000000001,
6.17449999999993));
#32447=CARTESIAN_POINT('Ctrl Pts',(-17.0802404735808,-16.4123522628063,
6.13283333333326));
#32448=CARTESIAN_POINT('Ctrl Pts',(-16.2901202367904,-16.8685283942094,
6.0911666666666));
#32449=CARTESIAN_POINT('Ctrl Pts',(-15.4999999999999,-17.3247045256125,
6.04949999999993));
#32450=CARTESIAN_POINT('Ctrl Pts',(-14.7098797632095,-16.8685283942094,
6.00783333333326));
#32451=CARTESIAN_POINT('Ctrl Pts',(-13.9197595264191,-16.4123522628063,
5.9661666666666));
#32452=CARTESIAN_POINT('Ctrl Pts',(-13.9197595264191,-15.5,5.92449999999993));
#32453=CARTESIAN_POINT('Ctrl Pts',(-13.9197595264191,-14.5876477371938,
5.88283333333326));
#32454=CARTESIAN_POINT('Ctrl Pts',(-14.7098797632095,-14.1314716057907,
5.8411666666666));
#32455=CARTESIAN_POINT('Ctrl Pts',(-15.5,-13.6752954743876,5.79949999999993));
#32456=CARTESIAN_POINT('Ctrl Pts',(-16.2901202367904,-14.1314716057907,
5.75783333333326));
#32457=CARTESIAN_POINT('Ctrl Pts',(-17.0802404735808,-14.5876477371938,
5.71616666666659));
#32458=CARTESIAN_POINT('Ctrl Pts',(-17.0802404735808,-15.5000000000001,
5.67449999999993));
#32459=CARTESIAN_POINT('Ctrl Pts',(-17.0802404735808,-16.4123522628063,
5.63283333333326));
#32460=CARTESIAN_POINT('Ctrl Pts',(-16.2901202367904,-16.8685283942094,
5.59116666666659));
#32461=CARTESIAN_POINT('Ctrl Pts',(-15.4999999999999,-17.3247045256125,
5.54949999999992));
#32462=CARTESIAN_POINT('Ctrl Pts',(-14.7098797632095,-16.8685283942094,
5.50783333333326));
#32463=CARTESIAN_POINT('Ctrl Pts',(-13.9197595264191,-16.4123522628063,
5.46616666666659));
#32464=CARTESIAN_POINT('Ctrl Pts',(-13.9197595264191,-15.5,5.42449999999992));
#32465=CARTESIAN_POINT('Ctrl Pts',(-13.9197595264191,-14.5876477371938,
5.38283333333326));
#32466=CARTESIAN_POINT('Ctrl Pts',(-14.7098797632095,-14.1314716057907,
5.34116666666659));
#32467=CARTESIAN_POINT('Ctrl Pts',(-15.5,-13.6752954743876,5.29949999999992));
#32468=CARTESIAN_POINT('Ctrl Pts',(-16.2901202367904,-14.1314716057907,
5.25783333333325));
#32469=CARTESIAN_POINT('Ctrl Pts',(-17.0802404735808,-14.5876477371938,
5.21616666666659));
#32470=CARTESIAN_POINT('Ctrl Pts',(-17.0802404735808,-15.5000000000001,
5.17449999999992));
#32471=CARTESIAN_POINT('Ctrl Pts',(-17.0802404735808,-16.4123522628063,
5.13283333333325));
#32472=CARTESIAN_POINT('Ctrl Pts',(-16.2901202367904,-16.8685283942094,
5.09116666666658));
#32473=CARTESIAN_POINT('Ctrl Pts',(-15.4999999999999,-17.3247045256125,
5.04949999999992));
#32474=CARTESIAN_POINT('Ctrl Pts',(-14.7098797632095,-16.8685283942094,
5.00783333333325));
#32475=CARTESIAN_POINT('Ctrl Pts',(-13.9197595264191,-16.4123522628063,
4.96616666666658));
#32476=CARTESIAN_POINT('Ctrl Pts',(-13.9197595264191,-15.5,4.92449999999992));
#32477=CARTESIAN_POINT('Ctrl Pts',(-13.9197595264191,-14.5876477371938,
4.88283333333325));
#32478=CARTESIAN_POINT('Ctrl Pts',(-14.7098797632095,-14.1314716057907,
4.84116666666658));
#32479=CARTESIAN_POINT('Ctrl Pts',(-15.5,-13.6752954743876,4.79949999999991));
#32480=CARTESIAN_POINT('Ctrl Pts',(-16.2901202367904,-14.1314716057907,
4.75783333333325));
#32481=CARTESIAN_POINT('Ctrl Pts',(-17.0802404735808,-14.5876477371938,
4.71616666666658));
#32482=CARTESIAN_POINT('Ctrl Pts',(-17.0802404735808,-15.5000000000001,
4.67449999999991));
#32483=CARTESIAN_POINT('Ctrl Pts',(-17.0802404735808,-16.4123522628063,
4.63283333333325));
#32484=CARTESIAN_POINT('Ctrl Pts',(-16.2901202367904,-16.8685283942094,
4.59116666666658));
#32485=CARTESIAN_POINT('Ctrl Pts',(-15.4999999999999,-17.3247045256125,
4.54949999999991));
#32486=CARTESIAN_POINT('Ctrl Pts',(-14.7098797632095,-16.8685283942094,
4.50783333333324));
#32487=CARTESIAN_POINT('Ctrl Pts',(-13.9197595264191,-16.4123522628063,
4.46616666666658));
#32488=CARTESIAN_POINT('Ctrl Pts',(-13.9197595264191,-15.5,4.42449999999991));
#32489=CARTESIAN_POINT('Ctrl Pts',(-13.9197595264191,-14.5876477371938,
4.38283333333324));
#32490=CARTESIAN_POINT('Ctrl Pts',(-14.7098797632095,-14.1314716057907,
4.34116666666657));
#32491=CARTESIAN_POINT('Ctrl Pts',(-15.5,-13.6752954743876,4.29949999999991));
#32492=CARTESIAN_POINT('Ctrl Pts',(-16.2901202367904,-14.1314716057907,
4.25783333333324));
#32493=CARTESIAN_POINT('Ctrl Pts',(-17.0802404735808,-14.5876477371938,
4.21616666666657));
#32494=CARTESIAN_POINT('Ctrl Pts',(-17.0802404735808,-15.5000000000001,
4.17449999999991));
#32495=CARTESIAN_POINT('Ctrl Pts',(-17.0802404735808,-16.4123522628063,
4.13283333333324));
#32496=CARTESIAN_POINT('Ctrl Pts',(-16.2901202367904,-16.8685283942094,
4.09116666666657));
#32497=CARTESIAN_POINT('Ctrl Pts',(-15.4999999999999,-17.3247045256125,
4.0494999999999));
#32498=CARTESIAN_POINT('Ctrl Pts',(-14.7098797632095,-16.8685283942094,
4.00783333333324));
#32499=CARTESIAN_POINT('Ctrl Pts',(-13.9197595264191,-16.4123522628063,
3.96616666666657));
#32500=CARTESIAN_POINT('Ctrl Pts',(-13.9197595264191,-15.5,3.9244999999999));
#32501=CARTESIAN_POINT('Ctrl Pts',(-13.9197595264191,-14.5876477371938,
3.88283333333323));
#32502=CARTESIAN_POINT('Ctrl Pts',(-14.7098797632095,-14.1314716057907,
3.84116666666657));
#32503=CARTESIAN_POINT('Ctrl Pts',(-15.5,-13.6752954743876,3.7994999999999));
#32504=CARTESIAN_POINT('Ctrl Pts',(-16.2901202367904,-14.1314716057907,
3.75783333333323));
#32505=CARTESIAN_POINT('Ctrl Pts',(-17.0802404735808,-14.5876477371938,
3.71616666666657));
#32506=CARTESIAN_POINT('Ctrl Pts',(-17.0802404735808,-15.5000000000001,
3.6744999999999));
#32507=CARTESIAN_POINT('Ctrl Pts',(-17.0802404735808,-16.4123522628063,
3.63283333333323));
#32508=CARTESIAN_POINT('Ctrl Pts',(-16.2901202367904,-16.8685283942094,
3.59116666666656));
#32509=CARTESIAN_POINT('Ctrl Pts',(-15.4999999999999,-17.3247045256125,
3.5494999999999));
#32510=CARTESIAN_POINT('Ctrl Pts',(-14.7098797632095,-16.8685283942094,
3.50783333333323));
#32511=CARTESIAN_POINT('Ctrl Pts',(-13.9197595264191,-16.4123522628063,
3.46616666666656));
#32512=CARTESIAN_POINT('Ctrl Pts',(-13.9197595264191,-15.5,3.4244999999999));
#32513=CARTESIAN_POINT('Ctrl Pts',(-13.9197595264191,-14.5876477371938,
3.38283333333323));
#32514=CARTESIAN_POINT('Ctrl Pts',(-14.7098797632095,-14.1314716057907,
3.34116666666656));
#32515=CARTESIAN_POINT('Ctrl Pts',(-15.5,-13.6752954743876,3.29949999999989));
#32516=CARTESIAN_POINT('Ctrl Pts',(-16.2901202367904,-14.1314716057907,
3.25783333333323));
#32517=CARTESIAN_POINT('Ctrl Pts',(-17.0802404735808,-14.5876477371938,
3.21616666666656));
#32518=CARTESIAN_POINT('Ctrl Pts',(-17.0802404735808,-15.5000000000001,
3.17449999999989));
#32519=CARTESIAN_POINT('Ctrl Pts',(-17.0802404735808,-16.4123522628063,
3.13283333333323));
#32520=CARTESIAN_POINT('Ctrl Pts',(-16.2901202367904,-16.8685283942094,
3.09116666666656));
#32521=CARTESIAN_POINT('Ctrl Pts',(-15.4999999999999,-17.3247045256125,
3.04949999999989));
#32522=CARTESIAN_POINT('Ctrl Pts',(-14.7098797632095,-16.8685283942094,
3.00783333333322));
#32523=CARTESIAN_POINT('Ctrl Pts',(-13.9197595264191,-16.4123522628063,
2.96616666666656));
#32524=CARTESIAN_POINT('Ctrl Pts',(-13.9197595264191,-15.5,2.92449999999989));
#32525=CARTESIAN_POINT('Ctrl Pts',(-13.9197595264191,-14.5876477371938,
2.88283333333322));
#32526=CARTESIAN_POINT('Ctrl Pts',(-14.7098797632095,-14.1314716057907,
2.84116666666655));
#32527=CARTESIAN_POINT('Ctrl Pts',(-15.5,-13.6752954743876,2.79949999999989));
#32528=CARTESIAN_POINT('Ctrl Pts',(-16.2901202367904,-14.1314716057907,
2.75783333333322));
#32529=CARTESIAN_POINT('Ctrl Pts',(-17.0802404735808,-14.5876477371938,
2.71616666666655));
#32530=CARTESIAN_POINT('Ctrl Pts',(-17.0802404735808,-15.5000000000001,
2.67449999999989));
#32531=CARTESIAN_POINT('Ctrl Pts',(-17.0802404735808,-16.4123522628063,
2.63283333333322));
#32532=CARTESIAN_POINT('Ctrl Pts',(-16.2901202367904,-16.8685283942094,
2.59116666666655));
#32533=CARTESIAN_POINT('Ctrl Pts',(-15.4999999999999,-17.3247045256125,
2.54949999999988));
#32534=CARTESIAN_POINT('Ctrl Pts',(-14.7098797632095,-16.8685283942094,
2.50783333333322));
#32535=CARTESIAN_POINT('Ctrl Pts',(-13.9197595264191,-16.4123522628063,
2.46616666666655));
#32536=CARTESIAN_POINT('Ctrl Pts',(-13.9197595264191,-15.5,2.42449999999988));
#32537=CARTESIAN_POINT('Ctrl Pts',(-13.9197595264191,-14.5876477371938,
2.38283333333321));
#32538=CARTESIAN_POINT('Ctrl Pts',(-14.7098797632095,-14.1314716057907,
2.34116666666655));
#32539=CARTESIAN_POINT('Ctrl Pts',(-15.5,-13.6752954743876,2.29949999999988));
#32540=CARTESIAN_POINT('Ctrl Pts',(-16.2901202367904,-14.1314716057907,
2.25783333333321));
#32541=CARTESIAN_POINT('Ctrl Pts',(-17.0802404735808,-14.5876477371938,
2.21616666666655));
#32542=CARTESIAN_POINT('Ctrl Pts',(-17.0802404735808,-15.5000000000001,
2.17449999999988));
#32543=CARTESIAN_POINT('Ctrl Pts',(-17.0802404735808,-16.4123522628063,
2.13283333333321));
#32544=CARTESIAN_POINT('Ctrl Pts',(-16.2901202367904,-16.8685283942094,
2.09116666666655));
#32545=CARTESIAN_POINT('Ctrl Pts',(-15.4999999999999,-17.3247045256125,
2.04949999999988));
#32546=CARTESIAN_POINT('Ctrl Pts',(-14.7098797632095,-16.8685283942094,
2.00783333333321));
#32547=CARTESIAN_POINT('Ctrl Pts',(-13.9197595264191,-16.4123522628063,
1.96616666666654));
#32548=CARTESIAN_POINT('Ctrl Pts',(-13.9197595264191,-15.5,1.92449999999988));
#32549=CARTESIAN_POINT('Ctrl Pts',(-13.9197595264191,-14.5876477371938,
1.88283333333321));
#32550=CARTESIAN_POINT('Ctrl Pts',(-14.7098797632095,-14.1314716057907,
1.84116666666654));
#32551=CARTESIAN_POINT('Ctrl Pts',(-15.5,-13.6752954743876,1.79949999999987));
#32552=CARTESIAN_POINT('Ctrl Pts',(-16.2901202367904,-14.1314716057907,
1.75783333333321));
#32553=CARTESIAN_POINT('Ctrl Pts',(-17.0802404735808,-14.5876477371938,
1.71616666666654));
#32554=CARTESIAN_POINT('Ctrl Pts',(-17.0802404735808,-15.5000000000001,
1.67449999999987));
#32555=CARTESIAN_POINT('Ctrl Pts',(-17.0802404735808,-16.4123522628063,
1.63283333333321));
#32556=CARTESIAN_POINT('Ctrl Pts',(-16.2901202367904,-16.8685283942094,
1.59116666666654));
#32557=CARTESIAN_POINT('Ctrl Pts',(-15.4999999999999,-17.3247045256125,
1.54949999999987));
#32558=CARTESIAN_POINT('Ctrl Pts',(-14.7098797632095,-16.8685283942094,
1.5078333333332));
#32559=CARTESIAN_POINT('Ctrl Pts',(-13.9197595264191,-16.4123522628063,
1.46616666666654));
#32560=CARTESIAN_POINT('Ctrl Pts',(-13.9197595264191,-15.5,1.42449999999987));
#32561=CARTESIAN_POINT('Ctrl Pts',(-13.9197595264191,-14.5876477371938,
1.3828333333332));
#32562=CARTESIAN_POINT('Ctrl Pts',(-14.7098797632095,-14.1314716057907,
1.34116666666653));
#32563=CARTESIAN_POINT('Ctrl Pts',(-15.5,-13.6752954743876,1.29949999999987));
#32564=CARTESIAN_POINT('Ctrl Pts',(-16.2901202367904,-14.1314716057907,
1.2578333333332));
#32565=CARTESIAN_POINT('Ctrl Pts',(-17.0802404735808,-14.5876477371938,
1.21616666666653));
#32566=CARTESIAN_POINT('Ctrl Pts',(-17.0802404735808,-15.5000000000001,
1.17449999999986));
#32567=CARTESIAN_POINT('Ctrl Pts',(-17.0802404735808,-16.4123522628063,
1.1328333333332));
#32568=CARTESIAN_POINT('Ctrl Pts',(-16.2901202367904,-16.8685283942094,
1.09116666666653));
#32569=CARTESIAN_POINT('Ctrl Pts',(-15.4999999999999,-17.3247045256125,
1.04949999999987));
#32570=CARTESIAN_POINT('Ctrl Pts',(-14.7098797632095,-16.8685283942094,
1.0078333333332));
#32571=CARTESIAN_POINT('Ctrl Pts',(-13.9197595264191,-16.4123522628063,
0.96616666666653));
#32572=CARTESIAN_POINT('Ctrl Pts',(-13.9197595264191,-15.5,0.924499999999863));
#32573=CARTESIAN_POINT('Ctrl Pts',(-13.9197595264191,-14.5876477371938,
0.882833333333196));
#32574=CARTESIAN_POINT('Ctrl Pts',(-14.7098797632095,-14.1314716057907,
0.841166666666529));
#32575=CARTESIAN_POINT('Ctrl Pts',(-15.5,-13.6752954743876,0.799499999999861));
#32576=CARTESIAN_POINT('Ctrl Pts',(-16.2901202367904,-14.1314716057907,
0.757833333333194));
#32577=CARTESIAN_POINT('Ctrl Pts',(-17.0802404735808,-14.5876477371938,
0.716166666666527));
#32578=CARTESIAN_POINT('Ctrl Pts',(-17.0802404735808,-15.5000000000001,
0.674499999999859));
#32579=CARTESIAN_POINT('Ctrl Pts',(-17.0802404735808,-16.4123522628063,
0.632833333333192));
#32580=CARTESIAN_POINT('Ctrl Pts',(-16.2901202367904,-16.8685283942094,
0.591166666666525));
#32581=CARTESIAN_POINT('Ctrl Pts',(-15.4999999999999,-17.3247045256125,
0.549499999999857));
#32582=CARTESIAN_POINT('Ctrl Pts',(-14.7098797632095,-16.8685283942094,
0.50783333333319));
#32583=CARTESIAN_POINT('Ctrl Pts',(-13.9197595264191,-16.4123522628063,
0.466166666666523));
#32584=CARTESIAN_POINT('Ctrl Pts',(-13.9197595264191,-15.5,0.424499999999856));
#32585=CARTESIAN_POINT('Ctrl Pts',(-13.9197595264191,-14.5876477371938,
0.382833333333188));
#32586=CARTESIAN_POINT('Ctrl Pts',(-14.7098797632095,-14.1314716057907,
0.341166666666521));
#32587=CARTESIAN_POINT('Ctrl Pts',(-15.5,-13.6752954743876,0.299499999999854));
#32588=CARTESIAN_POINT('Ctrl Pts',(-16.2901202367904,-14.1314716057907,
0.257833333333186));
#32589=CARTESIAN_POINT('Ctrl Pts',(-17.0802404735808,-14.5876477371938,
0.216166666666519));
#32590=CARTESIAN_POINT('Ctrl Pts',(-17.0802404735808,-15.5000000000001,
0.174499999999852));
#32591=CARTESIAN_POINT('Ctrl Pts',(-17.0802404735808,-16.4123522628063,
0.132833333333185));
#32592=CARTESIAN_POINT('Ctrl Pts',(-16.2901202367904,-16.8685283942094,
0.0911666666665173));
#32593=CARTESIAN_POINT('Ctrl Pts',(-15.4999999999999,-17.3247045256125,
0.04949999999985));
#32594=CARTESIAN_POINT('Ctrl Pts',(-14.7098797632095,-16.8685283942094,
0.00783333333318273));
#32595=CARTESIAN_POINT('Ctrl Pts',(-13.9197595264191,-16.4123522628063,
-0.0338333333334846));
#32596=CARTESIAN_POINT('Ctrl Pts',(-13.9197595264191,-15.5,-0.0755000000001518));
#32597=CARTESIAN_POINT('Ctrl Pts',(-13.9197595264191,-14.5876477371938,
-0.117166666666817));
#32598=CARTESIAN_POINT('Ctrl Pts',(-14.7098797632095,-14.1314716057907,
-0.158833333333485));
#32599=CARTESIAN_POINT('Ctrl Pts',(-15.5,-13.6752954743876,-0.200500000000152));
#32600=CARTESIAN_POINT('Ctrl Pts',(-16.2901202367904,-14.1314716057907,
-0.242166666666819));
#32601=CARTESIAN_POINT('Ctrl Pts',(-17.0802404735808,-14.5876477371938,
-0.283833333333487));
#32602=CARTESIAN_POINT('Ctrl Pts',(-17.0802404735808,-15.5000000000001,
-0.325500000000154));
#32603=CARTESIAN_POINT('Ctrl Pts',(-17.0802404735808,-16.4123522628063,
-0.367166666666821));
#32604=CARTESIAN_POINT('Ctrl Pts',(-16.2901202367904,-16.8685283942094,
-0.408833333333488));
#32605=CARTESIAN_POINT('Ctrl Pts',(-15.4999999999999,-17.3247045256125,
-0.450500000000156));
#32606=CARTESIAN_POINT('Ctrl Pts',(-14.7098797632095,-16.8685283942094,
-0.492166666666823));
#32607=CARTESIAN_POINT('Ctrl Pts',(-13.9197595264191,-16.4123522628063,
-0.53383333333349));
#32608=CARTESIAN_POINT('Ctrl Pts',(-13.9197595264191,-15.5,-0.575500000000157));
#32609=CARTESIAN_POINT('Ctrl Pts',(-13.9197595264191,-14.5876477371938,
-0.617166666666825));
#32610=CARTESIAN_POINT('Ctrl Pts',(-14.7098797632095,-14.1314716057907,
-0.658833333333492));
#32611=CARTESIAN_POINT('Ctrl Pts',(-15.5,-13.6752954743876,-0.700500000000159));
#32612=CARTESIAN_POINT('Ctrl Pts',(-16.2901202367904,-14.1314716057907,
-0.742166666666827));
#32613=CARTESIAN_POINT('Ctrl Pts',(-17.0802404735808,-14.5876477371938,
-0.783833333333494));
#32614=CARTESIAN_POINT('Ctrl Pts',(-17.0802404735808,-15.5000000000001,
-0.825500000000161));
#32615=CARTESIAN_POINT('Ctrl Pts',(-17.0802404735808,-16.4123522628063,
-0.867166666666829));
#32616=CARTESIAN_POINT('Ctrl Pts',(-16.2901202367904,-16.8685283942094,
-0.908833333333496));
#32617=CARTESIAN_POINT('Ctrl Pts',(-15.4999999999999,-17.3247045256125,
-0.950500000000163));
#32618=CARTESIAN_POINT('Ctrl Pts',(-14.7098797632095,-16.8685283942094,
-0.99216666666683));
#32619=CARTESIAN_POINT('Ctrl Pts',(-13.9197595264191,-16.4123522628063,
-1.0338333333335));
#32620=CARTESIAN_POINT('Ctrl Pts',(-13.9197595264191,-15.5,-1.07550000000016));
#32621=CARTESIAN_POINT('Ctrl Pts',(-13.9197595264191,-14.5876477371938,
-1.11716666666683));
#32622=CARTESIAN_POINT('Ctrl Pts',(-14.7098797632095,-14.1314716057907,
-1.1588333333335));
#32623=CARTESIAN_POINT('Ctrl Pts',(-15.5,-13.6752954743876,-1.20050000000017));
#32624=CARTESIAN_POINT('Ctrl Pts',(-16.2901202367904,-14.1314716057907,
-1.24216666666683));
#32625=CARTESIAN_POINT('Ctrl Pts',(-17.0802404735808,-14.5876477371938,
-1.2838333333335));
#32626=CARTESIAN_POINT('Ctrl Pts',(-17.0802404735808,-15.5000000000001,
-1.32550000000017));
#32627=CARTESIAN_POINT('Ctrl Pts',(-17.0802404735808,-16.4123522628063,
-1.36716666666683));
#32628=CARTESIAN_POINT('Ctrl Pts',(-16.2901202367904,-16.8685283942094,
-1.4088333333335));
#32629=CARTESIAN_POINT('Ctrl Pts',(-15.4999999999999,-17.3247045256125,
-1.45050000000017));
#32630=CARTESIAN_POINT('Ctrl Pts',(-14.7098797632095,-16.8685283942094,
-1.49216666666684));
#32631=CARTESIAN_POINT('Ctrl Pts',(-13.9197595264191,-16.4123522628063,
-1.5338333333335));
#32632=CARTESIAN_POINT('Ctrl Pts',(-13.9197595264191,-15.5,-1.57550000000017));
#32633=CARTESIAN_POINT('Ctrl Pts',(-13.9197595264191,-14.5876477371938,
-1.61716666666684));
#32634=CARTESIAN_POINT('Ctrl Pts',(-14.7098797632095,-14.1314716057907,
-1.65883333333351));
#32635=CARTESIAN_POINT('Ctrl Pts',(-15.5,-13.6752954743876,-1.70050000000017));
#32636=CARTESIAN_POINT('Ctrl Pts',(-16.2901202367904,-14.1314716057907,
-1.74216666666684));
#32637=CARTESIAN_POINT('Ctrl Pts',(-17.0802404735808,-14.5876477371938,
-1.78383333333351));
#32638=CARTESIAN_POINT('Ctrl Pts',(-17.0802404735808,-15.5000000000001,
-1.82550000000017));
#32639=CARTESIAN_POINT('Ctrl Pts',(-17.0802404735808,-16.4123522628063,
-1.86716666666684));
#32640=CARTESIAN_POINT('Ctrl Pts',(-16.2901202367904,-16.8685283942094,
-1.90883333333351));
#32641=CARTESIAN_POINT('Ctrl Pts',(-15.4999999999999,-17.3247045256125,
-1.95050000000018));
#32642=CARTESIAN_POINT('Ctrl Pts',(-14.7098797632095,-16.8685283942094,
-1.99216666666684));
#32643=CARTESIAN_POINT('Ctrl Pts',(-14.4189900731849,-16.7005831533692,
-2.00750661517932));
#32644=CARTESIAN_POINT('Ctrl Pts',(-14.2215542486879,-16.4288360540162,
-2.02512301646327));
#32645=CARTESIAN_POINT('',(-13.9369173167913,-16.6356236599184,-2.22824840486548));
#32646=CARTESIAN_POINT('Ctrl Pts',(-17.4320632938682,-15.5000000000001,
11.440125));
#32647=CARTESIAN_POINT('Ctrl Pts',(-17.4320632938682,-16.6154772628063,
11.3984583333333));
#32648=CARTESIAN_POINT('Ctrl Pts',(-16.4660316469341,-17.1732158942094,
11.3567916666667));
#32649=CARTESIAN_POINT('Ctrl Pts',(-15.4999999999999,-17.7309545256125,
11.315125));
#32650=CARTESIAN_POINT('Ctrl Pts',(-14.5339683530658,-17.1732158942094,
11.2734583333333));
#32651=CARTESIAN_POINT('Ctrl Pts',(-13.5679367061317,-16.6154772628063,
11.2317916666667));
#32652=CARTESIAN_POINT('Ctrl Pts',(-13.5679367061317,-15.5,11.190125));
#32653=CARTESIAN_POINT('Ctrl Pts',(-13.5679367061317,-14.3845227371938,
11.1484583333333));
#32654=CARTESIAN_POINT('Ctrl Pts',(-14.5339683530658,-13.8267841057907,
11.1067916666667));
#32655=CARTESIAN_POINT('Ctrl Pts',(-15.5,-13.2690454743876,11.065125));
#32656=CARTESIAN_POINT('Ctrl Pts',(-16.4660316469341,-13.8267841057907,
11.0234583333333));
#32657=CARTESIAN_POINT('Ctrl Pts',(-17.4320632938682,-14.3845227371938,
10.9817916666667));
#32658=CARTESIAN_POINT('Ctrl Pts',(-17.4320632938682,-15.5000000000001,
10.940125));
#32659=CARTESIAN_POINT('Ctrl Pts',(-17.4320632938682,-16.6154772628063,
10.8984583333333));
#32660=CARTESIAN_POINT('Ctrl Pts',(-16.4660316469341,-17.1732158942094,
10.8567916666667));
#32661=CARTESIAN_POINT('Ctrl Pts',(-15.4999999999999,-17.7309545256125,
10.815125));
#32662=CARTESIAN_POINT('Ctrl Pts',(-14.5339683530658,-17.1732158942094,
10.7734583333333));
#32663=CARTESIAN_POINT('Ctrl Pts',(-13.5679367061317,-16.6154772628063,
10.7317916666667));
#32664=CARTESIAN_POINT('Ctrl Pts',(-13.5679367061317,-15.5,10.690125));
#32665=CARTESIAN_POINT('Ctrl Pts',(-13.5679367061317,-14.3845227371938,
10.6484583333333));
#32666=CARTESIAN_POINT('Ctrl Pts',(-14.5339683530658,-13.8267841057907,
10.6067916666667));
#32667=CARTESIAN_POINT('Ctrl Pts',(-15.5,-13.2690454743876,10.565125));
#32668=CARTESIAN_POINT('Ctrl Pts',(-16.4660316469341,-13.8267841057907,
10.5234583333333));
#32669=CARTESIAN_POINT('Ctrl Pts',(-17.4320632938682,-14.3845227371938,
10.4817916666667));
#32670=CARTESIAN_POINT('Ctrl Pts',(-17.4320632938682,-15.5000000000001,
10.440125));
#32671=CARTESIAN_POINT('Ctrl Pts',(-17.4320632938682,-16.6154772628063,
10.3984583333333));
#32672=CARTESIAN_POINT('Ctrl Pts',(-16.4660316469341,-17.1732158942094,
10.3567916666667));
#32673=CARTESIAN_POINT('Ctrl Pts',(-15.4999999999999,-17.7309545256125,
10.315125));
#32674=CARTESIAN_POINT('Ctrl Pts',(-14.5339683530658,-17.1732158942094,
10.2734583333333));
#32675=CARTESIAN_POINT('Ctrl Pts',(-13.5679367061317,-16.6154772628063,
10.2317916666667));
#32676=CARTESIAN_POINT('Ctrl Pts',(-13.5679367061317,-15.5,10.190125));
#32677=CARTESIAN_POINT('Ctrl Pts',(-13.5679367061317,-14.3845227371938,
10.1484583333333));
#32678=CARTESIAN_POINT('Ctrl Pts',(-14.5339683530658,-13.8267841057907,
10.1067916666666));
#32679=CARTESIAN_POINT('Ctrl Pts',(-15.5,-13.2690454743876,10.065125));
#32680=CARTESIAN_POINT('Ctrl Pts',(-16.4660316469341,-13.8267841057907,
10.0234583333333));
#32681=CARTESIAN_POINT('Ctrl Pts',(-17.4320632938682,-14.3845227371938,
9.98179166666664));
#32682=CARTESIAN_POINT('Ctrl Pts',(-17.4320632938682,-15.5000000000001,
9.94012499999998));
#32683=CARTESIAN_POINT('Ctrl Pts',(-17.4320632938682,-16.6154772628063,
9.89845833333331));
#32684=CARTESIAN_POINT('Ctrl Pts',(-16.4660316469341,-17.1732158942094,
9.85679166666664));
#32685=CARTESIAN_POINT('Ctrl Pts',(-15.4999999999999,-17.7309545256125,
9.81512499999998));
#32686=CARTESIAN_POINT('Ctrl Pts',(-14.5339683530658,-17.1732158942094,
9.77345833333331));
#32687=CARTESIAN_POINT('Ctrl Pts',(-13.5679367061317,-16.6154772628063,
9.73179166666664));
#32688=CARTESIAN_POINT('Ctrl Pts',(-13.5679367061317,-15.5,9.69012499999998));
#32689=CARTESIAN_POINT('Ctrl Pts',(-13.5679367061317,-14.3845227371938,
9.64845833333331));
#32690=CARTESIAN_POINT('Ctrl Pts',(-14.5339683530658,-13.8267841057907,
9.60679166666664));
#32691=CARTESIAN_POINT('Ctrl Pts',(-15.5,-13.2690454743876,9.56512499999998));
#32692=CARTESIAN_POINT('Ctrl Pts',(-16.4660316469341,-13.8267841057907,
9.52345833333331));
#32693=CARTESIAN_POINT('Ctrl Pts',(-17.4320632938682,-14.3845227371938,
9.48179166666664));
#32694=CARTESIAN_POINT('Ctrl Pts',(-17.4320632938682,-15.5000000000001,
9.44012499999997));
#32695=CARTESIAN_POINT('Ctrl Pts',(-17.4320632938682,-16.6154772628063,
9.39845833333331));
#32696=CARTESIAN_POINT('Ctrl Pts',(-16.4660316469341,-17.1732158942094,
9.35679166666664));
#32697=CARTESIAN_POINT('Ctrl Pts',(-15.4999999999999,-17.7309545256125,
9.31512499999997));
#32698=CARTESIAN_POINT('Ctrl Pts',(-14.5339683530658,-17.1732158942094,
9.2734583333333));
#32699=CARTESIAN_POINT('Ctrl Pts',(-13.5679367061317,-16.6154772628063,
9.23179166666664));
#32700=CARTESIAN_POINT('Ctrl Pts',(-13.5679367061317,-15.5,9.19012499999997));
#32701=CARTESIAN_POINT('Ctrl Pts',(-13.5679367061317,-14.3845227371938,
9.1484583333333));
#32702=CARTESIAN_POINT('Ctrl Pts',(-14.5339683530658,-13.8267841057907,
9.10679166666664));
#32703=CARTESIAN_POINT('Ctrl Pts',(-15.5,-13.2690454743876,9.06512499999997));
#32704=CARTESIAN_POINT('Ctrl Pts',(-16.4660316469341,-13.8267841057907,
9.0234583333333));
#32705=CARTESIAN_POINT('Ctrl Pts',(-17.4320632938682,-14.3845227371938,
8.98179166666663));
#32706=CARTESIAN_POINT('Ctrl Pts',(-17.4320632938682,-15.5000000000001,
8.94012499999997));
#32707=CARTESIAN_POINT('Ctrl Pts',(-17.4320632938682,-16.6154772628063,
8.8984583333333));
#32708=CARTESIAN_POINT('Ctrl Pts',(-16.4660316469341,-17.1732158942094,
8.85679166666663));
#32709=CARTESIAN_POINT('Ctrl Pts',(-15.4999999999999,-17.7309545256125,
8.81512499999996));
#32710=CARTESIAN_POINT('Ctrl Pts',(-14.5339683530658,-17.1732158942094,
8.7734583333333));
#32711=CARTESIAN_POINT('Ctrl Pts',(-13.5679367061317,-16.6154772628063,
8.73179166666663));
#32712=CARTESIAN_POINT('Ctrl Pts',(-13.5679367061317,-15.5,8.69012499999996));
#32713=CARTESIAN_POINT('Ctrl Pts',(-13.5679367061317,-14.3845227371938,
8.64845833333329));
#32714=CARTESIAN_POINT('Ctrl Pts',(-14.5339683530658,-13.8267841057907,
8.60679166666663));
#32715=CARTESIAN_POINT('Ctrl Pts',(-15.5,-13.2690454743876,8.56512499999996));
#32716=CARTESIAN_POINT('Ctrl Pts',(-16.4660316469341,-13.8267841057907,
8.52345833333329));
#32717=CARTESIAN_POINT('Ctrl Pts',(-17.4320632938682,-14.3845227371938,
8.48179166666663));
#32718=CARTESIAN_POINT('Ctrl Pts',(-17.4320632938682,-15.5000000000001,
8.44012499999996));
#32719=CARTESIAN_POINT('Ctrl Pts',(-17.4320632938682,-16.6154772628063,
8.39845833333329));
#32720=CARTESIAN_POINT('Ctrl Pts',(-16.4660316469341,-17.1732158942094,
8.35679166666662));
#32721=CARTESIAN_POINT('Ctrl Pts',(-15.4999999999999,-17.7309545256125,
8.31512499999996));
#32722=CARTESIAN_POINT('Ctrl Pts',(-14.5339683530658,-17.1732158942094,
8.27345833333329));
#32723=CARTESIAN_POINT('Ctrl Pts',(-13.5679367061317,-16.6154772628063,
8.23179166666662));
#32724=CARTESIAN_POINT('Ctrl Pts',(-13.5679367061317,-15.5,8.19012499999996));
#32725=CARTESIAN_POINT('Ctrl Pts',(-13.5679367061317,-14.3845227371938,
8.14845833333329));
#32726=CARTESIAN_POINT('Ctrl Pts',(-14.5339683530658,-13.8267841057907,
8.10679166666662));
#32727=CARTESIAN_POINT('Ctrl Pts',(-15.5,-13.2690454743876,8.06512499999995));
#32728=CARTESIAN_POINT('Ctrl Pts',(-16.4660316469341,-13.8267841057907,
8.02345833333329));
#32729=CARTESIAN_POINT('Ctrl Pts',(-17.4320632938682,-14.3845227371938,
7.98179166666662));
#32730=CARTESIAN_POINT('Ctrl Pts',(-17.4320632938682,-15.5000000000001,
7.94012499999995));
#32731=CARTESIAN_POINT('Ctrl Pts',(-17.4320632938682,-16.6154772628063,
7.89845833333329));
#32732=CARTESIAN_POINT('Ctrl Pts',(-16.4660316469341,-17.1732158942094,
7.85679166666662));
#32733=CARTESIAN_POINT('Ctrl Pts',(-15.4999999999999,-17.7309545256125,
7.81512499999995));
#32734=CARTESIAN_POINT('Ctrl Pts',(-14.5339683530658,-17.1732158942094,
7.77345833333328));
#32735=CARTESIAN_POINT('Ctrl Pts',(-13.5679367061317,-16.6154772628063,
7.73179166666662));
#32736=CARTESIAN_POINT('Ctrl Pts',(-13.5679367061317,-15.5,7.69012499999995));
#32737=CARTESIAN_POINT('Ctrl Pts',(-13.5679367061317,-14.3845227371938,
7.64845833333328));
#32738=CARTESIAN_POINT('Ctrl Pts',(-14.5339683530658,-13.8267841057907,
7.60679166666661));
#32739=CARTESIAN_POINT('Ctrl Pts',(-15.5,-13.2690454743876,7.56512499999995));
#32740=CARTESIAN_POINT('Ctrl Pts',(-16.4660316469341,-13.8267841057907,
7.52345833333328));
#32741=CARTESIAN_POINT('Ctrl Pts',(-17.4320632938682,-14.3845227371938,
7.48179166666661));
#32742=CARTESIAN_POINT('Ctrl Pts',(-17.4320632938682,-15.5000000000001,
7.44012499999995));
#32743=CARTESIAN_POINT('Ctrl Pts',(-17.4320632938682,-16.6154772628063,
7.39845833333328));
#32744=CARTESIAN_POINT('Ctrl Pts',(-16.4660316469341,-17.1732158942094,
7.35679166666661));
#32745=CARTESIAN_POINT('Ctrl Pts',(-15.4999999999999,-17.7309545256125,
7.31512499999995));
#32746=CARTESIAN_POINT('Ctrl Pts',(-14.5339683530658,-17.1732158942094,
7.27345833333328));
#32747=CARTESIAN_POINT('Ctrl Pts',(-13.5679367061317,-16.6154772628063,
7.23179166666661));
#32748=CARTESIAN_POINT('Ctrl Pts',(-13.5679367061317,-15.5,7.19012499999994));
#32749=CARTESIAN_POINT('Ctrl Pts',(-13.5679367061317,-14.3845227371938,
7.14845833333328));
#32750=CARTESIAN_POINT('Ctrl Pts',(-14.5339683530658,-13.8267841057907,
7.10679166666661));
#32751=CARTESIAN_POINT('Ctrl Pts',(-15.5,-13.2690454743876,7.06512499999994));
#32752=CARTESIAN_POINT('Ctrl Pts',(-16.4660316469341,-13.8267841057907,
7.02345833333327));
#32753=CARTESIAN_POINT('Ctrl Pts',(-17.4320632938682,-14.3845227371938,
6.98179166666661));
#32754=CARTESIAN_POINT('Ctrl Pts',(-17.4320632938682,-15.5000000000001,
6.94012499999994));
#32755=CARTESIAN_POINT('Ctrl Pts',(-17.4320632938682,-16.6154772628063,
6.89845833333327));
#32756=CARTESIAN_POINT('Ctrl Pts',(-16.4660316469341,-17.1732158942094,
6.8567916666666));
#32757=CARTESIAN_POINT('Ctrl Pts',(-15.4999999999999,-17.7309545256125,
6.81512499999994));
#32758=CARTESIAN_POINT('Ctrl Pts',(-14.5339683530658,-17.1732158942094,
6.77345833333327));
#32759=CARTESIAN_POINT('Ctrl Pts',(-13.5679367061317,-16.6154772628063,
6.7317916666666));
#32760=CARTESIAN_POINT('Ctrl Pts',(-13.5679367061317,-15.5,6.69012499999994));
#32761=CARTESIAN_POINT('Ctrl Pts',(-13.5679367061317,-14.3845227371938,
6.64845833333327));
#32762=CARTESIAN_POINT('Ctrl Pts',(-14.5339683530658,-13.8267841057907,
6.6067916666666));
#32763=CARTESIAN_POINT('Ctrl Pts',(-15.5,-13.2690454743876,6.56512499999993));
#32764=CARTESIAN_POINT('Ctrl Pts',(-16.4660316469341,-13.8267841057907,
6.52345833333327));
#32765=CARTESIAN_POINT('Ctrl Pts',(-17.4320632938682,-14.3845227371938,
6.4817916666666));
#32766=CARTESIAN_POINT('Ctrl Pts',(-17.4320632938682,-15.5000000000001,
6.44012499999993));
#32767=CARTESIAN_POINT('Ctrl Pts',(-17.4320632938682,-16.6154772628063,
6.39845833333327));
#32768=CARTESIAN_POINT('Ctrl Pts',(-16.4660316469341,-17.1732158942094,
6.3567916666666));
#32769=CARTESIAN_POINT('Ctrl Pts',(-15.4999999999999,-17.7309545256125,
6.31512499999993));
#32770=CARTESIAN_POINT('Ctrl Pts',(-14.5339683530658,-17.1732158942094,
6.27345833333326));
#32771=CARTESIAN_POINT('Ctrl Pts',(-13.5679367061317,-16.6154772628063,
6.2317916666666));
#32772=CARTESIAN_POINT('Ctrl Pts',(-13.5679367061317,-15.5,6.19012499999993));
#32773=CARTESIAN_POINT('Ctrl Pts',(-13.5679367061317,-14.3845227371938,
6.14845833333326));
#32774=CARTESIAN_POINT('Ctrl Pts',(-14.5339683530658,-13.8267841057907,
6.10679166666659));
#32775=CARTESIAN_POINT('Ctrl Pts',(-15.5,-13.2690454743876,6.06512499999993));
#32776=CARTESIAN_POINT('Ctrl Pts',(-16.4660316469341,-13.8267841057907,
6.02345833333326));
#32777=CARTESIAN_POINT('Ctrl Pts',(-17.4320632938682,-14.3845227371938,
5.98179166666659));
#32778=CARTESIAN_POINT('Ctrl Pts',(-17.4320632938682,-15.5000000000001,
5.94012499999993));
#32779=CARTESIAN_POINT('Ctrl Pts',(-17.4320632938682,-16.6154772628063,
5.89845833333326));
#32780=CARTESIAN_POINT('Ctrl Pts',(-16.4660316469341,-17.1732158942094,
5.85679166666659));
#32781=CARTESIAN_POINT('Ctrl Pts',(-15.4999999999999,-17.7309545256125,
5.81512499999992));
#32782=CARTESIAN_POINT('Ctrl Pts',(-14.5339683530658,-17.1732158942094,
5.77345833333326));
#32783=CARTESIAN_POINT('Ctrl Pts',(-13.5679367061317,-16.6154772628063,
5.73179166666659));
#32784=CARTESIAN_POINT('Ctrl Pts',(-13.5679367061317,-15.5,5.69012499999992));
#32785=CARTESIAN_POINT('Ctrl Pts',(-13.5679367061317,-14.3845227371938,
5.64845833333326));
#32786=CARTESIAN_POINT('Ctrl Pts',(-14.5339683530658,-13.8267841057907,
5.60679166666659));
#32787=CARTESIAN_POINT('Ctrl Pts',(-15.5,-13.2690454743876,5.56512499999992));
#32788=CARTESIAN_POINT('Ctrl Pts',(-16.4660316469341,-13.8267841057907,
5.52345833333325));
#32789=CARTESIAN_POINT('Ctrl Pts',(-17.4320632938682,-14.3845227371938,
5.48179166666659));
#32790=CARTESIAN_POINT('Ctrl Pts',(-17.4320632938682,-15.5000000000001,
5.44012499999992));
#32791=CARTESIAN_POINT('Ctrl Pts',(-17.4320632938682,-16.6154772628063,
5.39845833333325));
#32792=CARTESIAN_POINT('Ctrl Pts',(-16.4660316469341,-17.1732158942094,
5.35679166666658));
#32793=CARTESIAN_POINT('Ctrl Pts',(-15.4999999999999,-17.7309545256125,
5.31512499999992));
#32794=CARTESIAN_POINT('Ctrl Pts',(-14.5339683530658,-17.1732158942094,
5.27345833333325));
#32795=CARTESIAN_POINT('Ctrl Pts',(-13.5679367061317,-16.6154772628063,
5.23179166666658));
#32796=CARTESIAN_POINT('Ctrl Pts',(-13.5679367061317,-15.5,5.19012499999992));
#32797=CARTESIAN_POINT('Ctrl Pts',(-13.5679367061317,-14.3845227371938,
5.14845833333325));
#32798=CARTESIAN_POINT('Ctrl Pts',(-14.5339683530658,-13.8267841057907,
5.10679166666658));
#32799=CARTESIAN_POINT('Ctrl Pts',(-15.5,-13.2690454743876,5.06512499999991));
#32800=CARTESIAN_POINT('Ctrl Pts',(-16.4660316469341,-13.8267841057907,
5.02345833333325));
#32801=CARTESIAN_POINT('Ctrl Pts',(-17.4320632938682,-14.3845227371938,
4.98179166666658));
#32802=CARTESIAN_POINT('Ctrl Pts',(-17.4320632938682,-15.5000000000001,
4.94012499999991));
#32803=CARTESIAN_POINT('Ctrl Pts',(-17.4320632938682,-16.6154772628063,
4.89845833333325));
#32804=CARTESIAN_POINT('Ctrl Pts',(-16.4660316469341,-17.1732158942094,
4.85679166666658));
#32805=CARTESIAN_POINT('Ctrl Pts',(-15.4999999999999,-17.7309545256125,
4.81512499999991));
#32806=CARTESIAN_POINT('Ctrl Pts',(-14.5339683530658,-17.1732158942094,
4.77345833333324));
#32807=CARTESIAN_POINT('Ctrl Pts',(-13.5679367061317,-16.6154772628063,
4.73179166666658));
#32808=CARTESIAN_POINT('Ctrl Pts',(-13.5679367061317,-15.5,4.69012499999991));
#32809=CARTESIAN_POINT('Ctrl Pts',(-13.5679367061317,-14.3845227371938,
4.64845833333324));
#32810=CARTESIAN_POINT('Ctrl Pts',(-14.5339683530658,-13.8267841057907,
4.60679166666657));
#32811=CARTESIAN_POINT('Ctrl Pts',(-15.5,-13.2690454743876,4.56512499999991));
#32812=CARTESIAN_POINT('Ctrl Pts',(-16.4660316469341,-13.8267841057907,
4.52345833333324));
#32813=CARTESIAN_POINT('Ctrl Pts',(-17.4320632938682,-14.3845227371938,
4.48179166666657));
#32814=CARTESIAN_POINT('Ctrl Pts',(-17.4320632938682,-15.5000000000001,
4.44012499999991));
#32815=CARTESIAN_POINT('Ctrl Pts',(-17.4320632938682,-16.6154772628063,
4.39845833333324));
#32816=CARTESIAN_POINT('Ctrl Pts',(-16.4660316469341,-17.1732158942094,
4.35679166666657));
#32817=CARTESIAN_POINT('Ctrl Pts',(-15.4999999999999,-17.7309545256125,
4.31512499999991));
#32818=CARTESIAN_POINT('Ctrl Pts',(-14.5339683530658,-17.1732158942094,
4.27345833333324));
#32819=CARTESIAN_POINT('Ctrl Pts',(-13.5679367061317,-16.6154772628063,
4.23179166666657));
#32820=CARTESIAN_POINT('Ctrl Pts',(-13.5679367061317,-15.5,4.1901249999999));
#32821=CARTESIAN_POINT('Ctrl Pts',(-13.5679367061317,-14.3845227371938,
4.14845833333324));
#32822=CARTESIAN_POINT('Ctrl Pts',(-14.5339683530658,-13.8267841057907,
4.10679166666657));
#32823=CARTESIAN_POINT('Ctrl Pts',(-15.5,-13.2690454743876,4.0651249999999));
#32824=CARTESIAN_POINT('Ctrl Pts',(-16.4660316469341,-13.8267841057907,
4.02345833333323));
#32825=CARTESIAN_POINT('Ctrl Pts',(-17.4320632938682,-14.3845227371938,
3.98179166666657));
#32826=CARTESIAN_POINT('Ctrl Pts',(-17.4320632938682,-15.5000000000001,
3.9401249999999));
#32827=CARTESIAN_POINT('Ctrl Pts',(-17.4320632938682,-16.6154772628063,
3.89845833333323));
#32828=CARTESIAN_POINT('Ctrl Pts',(-16.4660316469341,-17.1732158942094,
3.85679166666657));
#32829=CARTESIAN_POINT('Ctrl Pts',(-15.4999999999999,-17.7309545256125,
3.8151249999999));
#32830=CARTESIAN_POINT('Ctrl Pts',(-14.5339683530658,-17.1732158942094,
3.77345833333323));
#32831=CARTESIAN_POINT('Ctrl Pts',(-13.5679367061317,-16.6154772628063,
3.73179166666656));
#32832=CARTESIAN_POINT('Ctrl Pts',(-13.5679367061317,-15.5,3.6901249999999));
#32833=CARTESIAN_POINT('Ctrl Pts',(-13.5679367061317,-14.3845227371938,
3.64845833333323));
#32834=CARTESIAN_POINT('Ctrl Pts',(-14.5339683530658,-13.8267841057907,
3.60679166666656));
#32835=CARTESIAN_POINT('Ctrl Pts',(-15.5,-13.2690454743876,3.5651249999999));
#32836=CARTESIAN_POINT('Ctrl Pts',(-16.4660316469341,-13.8267841057907,
3.52345833333323));
#32837=CARTESIAN_POINT('Ctrl Pts',(-17.4320632938682,-14.3845227371938,
3.48179166666656));
#32838=CARTESIAN_POINT('Ctrl Pts',(-17.4320632938682,-15.5000000000001,
3.44012499999989));
#32839=CARTESIAN_POINT('Ctrl Pts',(-17.4320632938682,-16.6154772628063,
3.39845833333323));
#32840=CARTESIAN_POINT('Ctrl Pts',(-16.4660316469341,-17.1732158942094,
3.35679166666656));
#32841=CARTESIAN_POINT('Ctrl Pts',(-15.4999999999999,-17.7309545256125,
3.31512499999989));
#32842=CARTESIAN_POINT('Ctrl Pts',(-14.5339683530658,-17.1732158942094,
3.27345833333322));
#32843=CARTESIAN_POINT('Ctrl Pts',(-13.5679367061317,-16.6154772628063,
3.23179166666656));
#32844=CARTESIAN_POINT('Ctrl Pts',(-13.5679367061317,-15.5,3.19012499999989));
#32845=CARTESIAN_POINT('Ctrl Pts',(-13.5679367061317,-14.3845227371938,
3.14845833333322));
#32846=CARTESIAN_POINT('Ctrl Pts',(-14.5339683530658,-13.8267841057907,
3.10679166666655));
#32847=CARTESIAN_POINT('Ctrl Pts',(-15.5,-13.2690454743876,3.06512499999989));
#32848=CARTESIAN_POINT('Ctrl Pts',(-16.4660316469341,-13.8267841057907,
3.02345833333322));
#32849=CARTESIAN_POINT('Ctrl Pts',(-17.4320632938682,-14.3845227371938,
2.98179166666655));
#32850=CARTESIAN_POINT('Ctrl Pts',(-17.4320632938682,-15.5000000000001,
2.94012499999989));
#32851=CARTESIAN_POINT('Ctrl Pts',(-17.4320632938682,-16.6154772628063,
2.89845833333322));
#32852=CARTESIAN_POINT('Ctrl Pts',(-16.4660316469341,-17.1732158942094,
2.85679166666655));
#32853=CARTESIAN_POINT('Ctrl Pts',(-15.4999999999999,-17.7309545256125,
2.81512499999988));
#32854=CARTESIAN_POINT('Ctrl Pts',(-14.5339683530658,-17.1732158942094,
2.77345833333322));
#32855=CARTESIAN_POINT('Ctrl Pts',(-13.5679367061317,-16.6154772628063,
2.73179166666655));
#32856=CARTESIAN_POINT('Ctrl Pts',(-13.5679367061317,-15.5,2.69012499999988));
#32857=CARTESIAN_POINT('Ctrl Pts',(-13.5679367061317,-14.3845227371938,
2.64845833333321));
#32858=CARTESIAN_POINT('Ctrl Pts',(-14.5339683530658,-13.8267841057907,
2.60679166666655));
#32859=CARTESIAN_POINT('Ctrl Pts',(-15.5,-13.2690454743876,2.56512499999988));
#32860=CARTESIAN_POINT('Ctrl Pts',(-16.4660316469341,-13.8267841057907,
2.52345833333321));
#32861=CARTESIAN_POINT('Ctrl Pts',(-17.4320632938682,-14.3845227371938,
2.48179166666655));
#32862=CARTESIAN_POINT('Ctrl Pts',(-17.4320632938682,-15.5000000000001,
2.44012499999988));
#32863=CARTESIAN_POINT('Ctrl Pts',(-17.4320632938682,-16.6154772628063,
2.39845833333321));
#32864=CARTESIAN_POINT('Ctrl Pts',(-16.4660316469341,-17.1732158942094,
2.35679166666655));
#32865=CARTESIAN_POINT('Ctrl Pts',(-15.4999999999999,-17.7309545256125,
2.31512499999988));
#32866=CARTESIAN_POINT('Ctrl Pts',(-14.5339683530658,-17.1732158942094,
2.27345833333321));
#32867=CARTESIAN_POINT('Ctrl Pts',(-13.5679367061317,-16.6154772628063,
2.23179166666654));
#32868=CARTESIAN_POINT('Ctrl Pts',(-13.5679367061317,-15.5,2.19012499999988));
#32869=CARTESIAN_POINT('Ctrl Pts',(-13.5679367061317,-14.3845227371938,
2.14845833333321));
#32870=CARTESIAN_POINT('Ctrl Pts',(-14.5339683530658,-13.8267841057907,
2.10679166666654));
#32871=CARTESIAN_POINT('Ctrl Pts',(-15.5,-13.2690454743876,2.06512499999987));
#32872=CARTESIAN_POINT('Ctrl Pts',(-16.4660316469341,-13.8267841057907,
2.02345833333321));
#32873=CARTESIAN_POINT('Ctrl Pts',(-17.4320632938682,-14.3845227371938,
1.98179166666654));
#32874=CARTESIAN_POINT('Ctrl Pts',(-17.4320632938682,-15.5000000000001,
1.94012499999987));
#32875=CARTESIAN_POINT('Ctrl Pts',(-17.4320632938682,-16.6154772628063,
1.89845833333321));
#32876=CARTESIAN_POINT('Ctrl Pts',(-16.4660316469341,-17.1732158942094,
1.85679166666654));
#32877=CARTESIAN_POINT('Ctrl Pts',(-15.4999999999999,-17.7309545256125,
1.81512499999987));
#32878=CARTESIAN_POINT('Ctrl Pts',(-14.5339683530658,-17.1732158942094,
1.7734583333332));
#32879=CARTESIAN_POINT('Ctrl Pts',(-13.5679367061317,-16.6154772628063,
1.73179166666654));
#32880=CARTESIAN_POINT('Ctrl Pts',(-13.5679367061317,-15.5,1.69012499999987));
#32881=CARTESIAN_POINT('Ctrl Pts',(-13.5679367061317,-14.3845227371938,
1.6484583333332));
#32882=CARTESIAN_POINT('Ctrl Pts',(-14.5339683530658,-13.8267841057907,
1.60679166666653));
#32883=CARTESIAN_POINT('Ctrl Pts',(-15.5,-13.2690454743876,1.56512499999987));
#32884=CARTESIAN_POINT('Ctrl Pts',(-16.4660316469341,-13.8267841057907,
1.5234583333332));
#32885=CARTESIAN_POINT('Ctrl Pts',(-17.4320632938682,-14.3845227371938,
1.48179166666653));
#32886=CARTESIAN_POINT('Ctrl Pts',(-17.4320632938682,-15.5000000000001,
1.44012499999987));
#32887=CARTESIAN_POINT('Ctrl Pts',(-17.4320632938682,-16.6154772628063,
1.3984583333332));
#32888=CARTESIAN_POINT('Ctrl Pts',(-16.4660316469341,-17.1732158942094,
1.35679166666653));
#32889=CARTESIAN_POINT('Ctrl Pts',(-15.4999999999999,-17.7309545256125,
1.31512499999987));
#32890=CARTESIAN_POINT('Ctrl Pts',(-14.5339683530658,-17.1732158942094,
1.2734583333332));
#32891=CARTESIAN_POINT('Ctrl Pts',(-13.5679367061317,-16.6154772628063,
1.23179166666653));
#32892=CARTESIAN_POINT('Ctrl Pts',(-13.5679367061317,-15.5,1.19012499999986));
#32893=CARTESIAN_POINT('Ctrl Pts',(-13.5679367061317,-14.3845227371938,
1.1484583333332));
#32894=CARTESIAN_POINT('Ctrl Pts',(-14.5339683530658,-13.8267841057907,
1.10679166666653));
#32895=CARTESIAN_POINT('Ctrl Pts',(-15.5,-13.2690454743876,1.06512499999986));
#32896=CARTESIAN_POINT('Ctrl Pts',(-16.4660316469341,-13.8267841057907,
1.02345833333319));
#32897=CARTESIAN_POINT('Ctrl Pts',(-17.4320632938682,-14.3845227371938,
0.981791666666527));
#32898=CARTESIAN_POINT('Ctrl Pts',(-17.4320632938682,-15.5000000000001,
0.94012499999986));
#32899=CARTESIAN_POINT('Ctrl Pts',(-17.4320632938682,-16.6154772628063,
0.898458333333192));
#32900=CARTESIAN_POINT('Ctrl Pts',(-16.4660316469341,-17.1732158942094,
0.856791666666525));
#32901=CARTESIAN_POINT('Ctrl Pts',(-15.4999999999999,-17.7309545256125,
0.815124999999858));
#32902=CARTESIAN_POINT('Ctrl Pts',(-14.5339683530658,-17.1732158942094,
0.77345833333319));
#32903=CARTESIAN_POINT('Ctrl Pts',(-13.5679367061317,-16.6154772628063,
0.731791666666523));
#32904=CARTESIAN_POINT('Ctrl Pts',(-13.5679367061317,-15.5,0.690124999999856));
#32905=CARTESIAN_POINT('Ctrl Pts',(-13.5679367061317,-14.3845227371938,
0.648458333333188));
#32906=CARTESIAN_POINT('Ctrl Pts',(-14.5339683530658,-13.8267841057907,
0.606791666666521));
#32907=CARTESIAN_POINT('Ctrl Pts',(-15.5,-13.2690454743876,0.565124999999854));
#32908=CARTESIAN_POINT('Ctrl Pts',(-16.4660316469341,-13.8267841057907,
0.523458333333187));
#32909=CARTESIAN_POINT('Ctrl Pts',(-17.4320632938682,-14.3845227371938,
0.481791666666519));
#32910=CARTESIAN_POINT('Ctrl Pts',(-17.4320632938682,-15.5000000000001,
0.440124999999852));
#32911=CARTESIAN_POINT('Ctrl Pts',(-17.4320632938682,-16.6154772628063,
0.398458333333185));
#32912=CARTESIAN_POINT('Ctrl Pts',(-16.4660316469341,-17.1732158942094,
0.356791666666518));
#32913=CARTESIAN_POINT('Ctrl Pts',(-15.4999999999999,-17.7309545256125,
0.31512499999985));
#32914=CARTESIAN_POINT('Ctrl Pts',(-14.5339683530658,-17.1732158942094,
0.273458333333183));
#32915=CARTESIAN_POINT('Ctrl Pts',(-13.5679367061317,-16.6154772628063,
0.231791666666516));
#32916=CARTESIAN_POINT('Ctrl Pts',(-13.5679367061317,-15.5,0.190124999999848));
#32917=CARTESIAN_POINT('Ctrl Pts',(-13.5679367061317,-14.3845227371938,
0.148458333333183));
#32918=CARTESIAN_POINT('Ctrl Pts',(-14.5339683530658,-13.8267841057907,
0.106791666666516));
#32919=CARTESIAN_POINT('Ctrl Pts',(-15.5,-13.2690454743876,0.0651249999998483));
#32920=CARTESIAN_POINT('Ctrl Pts',(-16.4660316469341,-13.8267841057907,
0.023458333333181));
#32921=CARTESIAN_POINT('Ctrl Pts',(-17.4320632938682,-14.3845227371938,
-0.0182083333334863));
#32922=CARTESIAN_POINT('Ctrl Pts',(-17.4320632938682,-15.5000000000001,
-0.0598750000001536));
#32923=CARTESIAN_POINT('Ctrl Pts',(-17.4320632938682,-16.6154772628063,
-0.101541666666821));
#32924=CARTESIAN_POINT('Ctrl Pts',(-16.4660316469341,-17.1732158942094,
-0.143208333333488));
#32925=CARTESIAN_POINT('Ctrl Pts',(-15.4999999999999,-17.7309545256125,
-0.184875000000155));
#32926=CARTESIAN_POINT('Ctrl Pts',(-14.5339683530658,-17.1732158942094,
-0.226541666666823));
#32927=CARTESIAN_POINT('Ctrl Pts',(-13.5679367061317,-16.6154772628063,
-0.26820833333349));
#32928=CARTESIAN_POINT('Ctrl Pts',(-13.5679367061317,-15.5,-0.309875000000157));
#32929=CARTESIAN_POINT('Ctrl Pts',(-13.5679367061317,-14.3845227371938,
-0.351541666666825));
#32930=CARTESIAN_POINT('Ctrl Pts',(-14.5339683530658,-13.8267841057907,
-0.393208333333492));
#32931=CARTESIAN_POINT('Ctrl Pts',(-15.5,-13.2690454743876,-0.434875000000159));
#32932=CARTESIAN_POINT('Ctrl Pts',(-16.4660316469341,-13.8267841057907,
-0.476541666666826));
#32933=CARTESIAN_POINT('Ctrl Pts',(-17.4320632938682,-14.3845227371938,
-0.518208333333494));
#32934=CARTESIAN_POINT('Ctrl Pts',(-17.4320632938682,-15.5000000000001,
-0.559875000000161));
#32935=CARTESIAN_POINT('Ctrl Pts',(-17.4320632938682,-16.6154772628063,
-0.601541666666828));
#32936=CARTESIAN_POINT('Ctrl Pts',(-16.4660316469341,-17.1732158942094,
-0.643208333333495));
#32937=CARTESIAN_POINT('Ctrl Pts',(-15.4999999999999,-17.7309545256125,
-0.684875000000163));
#32938=CARTESIAN_POINT('Ctrl Pts',(-14.5339683530658,-17.1732158942094,
-0.72654166666683));
#32939=CARTESIAN_POINT('Ctrl Pts',(-13.5679367061317,-16.6154772628063,
-0.768208333333497));
#32940=CARTESIAN_POINT('Ctrl Pts',(-13.5679367061317,-15.5,-0.809875000000165));
#32941=CARTESIAN_POINT('Ctrl Pts',(-13.5679367061317,-14.3845227371938,
-0.851541666666832));
#32942=CARTESIAN_POINT('Ctrl Pts',(-14.5339683530658,-13.8267841057907,
-0.893208333333499));
#32943=CARTESIAN_POINT('Ctrl Pts',(-15.5,-13.2690454743876,-0.934875000000167));
#32944=CARTESIAN_POINT('Ctrl Pts',(-16.4660316469341,-13.8267841057907,
-0.976541666666834));
#32945=CARTESIAN_POINT('Ctrl Pts',(-17.4320632938682,-14.3845227371938,
-1.0182083333335));
#32946=CARTESIAN_POINT('Ctrl Pts',(-17.4320632938682,-15.5000000000001,
-1.05987500000017));
#32947=CARTESIAN_POINT('Ctrl Pts',(-17.4320632938682,-16.6154772628063,
-1.10154166666683));
#32948=CARTESIAN_POINT('Ctrl Pts',(-16.4660316469341,-17.1732158942094,
-1.1432083333335));
#32949=CARTESIAN_POINT('Ctrl Pts',(-15.4999999999999,-17.7309545256125,
-1.18487500000017));
#32950=CARTESIAN_POINT('Ctrl Pts',(-14.5339683530658,-17.1732158942094,
-1.22654166666684));
#32951=CARTESIAN_POINT('Ctrl Pts',(-13.5679367061317,-16.6154772628063,
-1.2682083333335));
#32952=CARTESIAN_POINT('Ctrl Pts',(-13.5679367061317,-15.5,-1.30987500000017));
#32953=CARTESIAN_POINT('Ctrl Pts',(-13.5679367061317,-14.3845227371938,
-1.35154166666684));
#32954=CARTESIAN_POINT('Ctrl Pts',(-14.5339683530658,-13.8267841057907,
-1.3932083333335));
#32955=CARTESIAN_POINT('Ctrl Pts',(-15.5,-13.2690454743876,-1.43487500000017));
#32956=CARTESIAN_POINT('Ctrl Pts',(-16.4660316469341,-13.8267841057907,
-1.47654166666684));
#32957=CARTESIAN_POINT('Ctrl Pts',(-17.4320632938682,-14.3845227371938,
-1.51820833333351));
#32958=CARTESIAN_POINT('Ctrl Pts',(-17.4320632938682,-15.5000000000001,
-1.55987500000017));
#32959=CARTESIAN_POINT('Ctrl Pts',(-17.4320632938682,-16.6154772628063,
-1.60154166666684));
#32960=CARTESIAN_POINT('Ctrl Pts',(-16.4660316469341,-17.1732158942094,
-1.64320833333351));
#32961=CARTESIAN_POINT('Ctrl Pts',(-15.4999999999999,-17.7309545256125,
-1.68487500000018));
#32962=CARTESIAN_POINT('Ctrl Pts',(-14.5339683530658,-17.1732158942094,
-1.72654166666684));
#32963=CARTESIAN_POINT('Ctrl Pts',(-14.1783081829977,-16.9678753992806,
-1.74188192368624));
#32964=CARTESIAN_POINT('Ctrl Pts',(-13.9369186715641,-16.6356255246376,
-1.75949830599533));
#32965=CARTESIAN_POINT('Ctrl Pts',(-17.0802357869868,-15.5000000000001,
11.2369972941937));
#32966=CARTESIAN_POINT('Ctrl Pts',(-17.0802357869868,-16.412349557,11.195330627527));
#32967=CARTESIAN_POINT('Ctrl Pts',(-16.2901178934934,-16.8685243355,11.1536639608604));
#32968=CARTESIAN_POINT('Ctrl Pts',(-15.4999999999999,-17.324699114,11.1119972941937));
#32969=CARTESIAN_POINT('Ctrl Pts',(-14.7098821065065,-16.8685243355,11.070330627527));
#32970=CARTESIAN_POINT('Ctrl Pts',(-13.9197642130131,-16.412349557,11.0286639608604));
#32971=CARTESIAN_POINT('Ctrl Pts',(-13.9197642130131,-15.5,10.9869972941937));
#32972=CARTESIAN_POINT('Ctrl Pts',(-13.9197642130131,-14.5876504430001,
10.945330627527));
#32973=CARTESIAN_POINT('Ctrl Pts',(-14.7098821065065,-14.1314756645001,
10.9036639608604));
#32974=CARTESIAN_POINT('Ctrl Pts',(-15.5,-13.6753008860002,10.8619972941937));
#32975=CARTESIAN_POINT('Ctrl Pts',(-16.2901178934934,-14.1314756645001,
10.820330627527));
#32976=CARTESIAN_POINT('Ctrl Pts',(-17.0802357869868,-14.5876504430001,
10.7786639608604));
#32977=CARTESIAN_POINT('Ctrl Pts',(-17.0802357869868,-15.5000000000001,
10.7369972941937));
#32978=CARTESIAN_POINT('Ctrl Pts',(-17.0802357869868,-16.412349557,10.695330627527));
#32979=CARTESIAN_POINT('Ctrl Pts',(-16.2901178934934,-16.8685243355,10.6536639608604));
#32980=CARTESIAN_POINT('Ctrl Pts',(-15.4999999999999,-17.324699114,10.6119972941937));
#32981=CARTESIAN_POINT('Ctrl Pts',(-14.7098821065065,-16.8685243355,10.570330627527));
#32982=CARTESIAN_POINT('Ctrl Pts',(-13.9197642130131,-16.412349557,10.5286639608604));
#32983=CARTESIAN_POINT('Ctrl Pts',(-13.9197642130131,-15.5,10.4869972941937));
#32984=CARTESIAN_POINT('Ctrl Pts',(-13.9197642130131,-14.5876504430001,
10.445330627527));
#32985=CARTESIAN_POINT('Ctrl Pts',(-14.7098821065065,-14.1314756645001,
10.4036639608604));
#32986=CARTESIAN_POINT('Ctrl Pts',(-15.5,-13.6753008860002,10.3619972941937));
#32987=CARTESIAN_POINT('Ctrl Pts',(-16.2901178934934,-14.1314756645001,
10.320330627527));
#32988=CARTESIAN_POINT('Ctrl Pts',(-17.0802357869868,-14.5876504430001,
10.2786639608604));
#32989=CARTESIAN_POINT('Ctrl Pts',(-17.0802357869868,-15.5000000000001,
10.2369972941937));
#32990=CARTESIAN_POINT('Ctrl Pts',(-17.0802357869868,-16.412349557,10.195330627527));
#32991=CARTESIAN_POINT('Ctrl Pts',(-16.2901178934934,-16.8685243355,10.1536639608604));
#32992=CARTESIAN_POINT('Ctrl Pts',(-15.4999999999999,-17.324699114,10.1119972941937));
#32993=CARTESIAN_POINT('Ctrl Pts',(-14.7098821065065,-16.8685243355,10.070330627527));
#32994=CARTESIAN_POINT('Ctrl Pts',(-13.9197642130131,-16.412349557,10.0286639608604));
#32995=CARTESIAN_POINT('Ctrl Pts',(-13.9197642130131,-15.5,9.98699729419369));
#32996=CARTESIAN_POINT('Ctrl Pts',(-13.9197642130131,-14.5876504430001,
9.94533062752702));
#32997=CARTESIAN_POINT('Ctrl Pts',(-14.7098821065065,-14.1314756645001,
9.90366396086035));
#32998=CARTESIAN_POINT('Ctrl Pts',(-15.5,-13.6753008860002,9.86199729419368));
#32999=CARTESIAN_POINT('Ctrl Pts',(-16.2901178934934,-14.1314756645001,
9.82033062752702));
#33000=CARTESIAN_POINT('Ctrl Pts',(-17.0802357869868,-14.5876504430001,
9.77866396086035));
#33001=CARTESIAN_POINT('Ctrl Pts',(-17.0802357869868,-15.5000000000001,
9.73699729419368));
#33002=CARTESIAN_POINT('Ctrl Pts',(-17.0802357869868,-16.412349557,9.69533062752702));
#33003=CARTESIAN_POINT('Ctrl Pts',(-16.2901178934934,-16.8685243355,9.65366396086035));
#33004=CARTESIAN_POINT('Ctrl Pts',(-15.4999999999999,-17.324699114,9.61199729419368));
#33005=CARTESIAN_POINT('Ctrl Pts',(-14.7098821065065,-16.8685243355,9.57033062752701));
#33006=CARTESIAN_POINT('Ctrl Pts',(-13.9197642130131,-16.412349557,9.52866396086034));
#33007=CARTESIAN_POINT('Ctrl Pts',(-13.9197642130131,-15.5,9.48699729419368));
#33008=CARTESIAN_POINT('Ctrl Pts',(-13.9197642130131,-14.5876504430001,
9.44533062752701));
#33009=CARTESIAN_POINT('Ctrl Pts',(-14.7098821065065,-14.1314756645001,
9.40366396086034));
#33010=CARTESIAN_POINT('Ctrl Pts',(-15.5,-13.6753008860002,9.36199729419368));
#33011=CARTESIAN_POINT('Ctrl Pts',(-16.2901178934934,-14.1314756645001,
9.32033062752701));
#33012=CARTESIAN_POINT('Ctrl Pts',(-17.0802357869868,-14.5876504430001,
9.27866396086035));
#33013=CARTESIAN_POINT('Ctrl Pts',(-17.0802357869868,-15.5000000000001,
9.23699729419368));
#33014=CARTESIAN_POINT('Ctrl Pts',(-17.0802357869868,-16.412349557,9.19533062752701));
#33015=CARTESIAN_POINT('Ctrl Pts',(-16.2901178934934,-16.8685243355,9.15366396086034));
#33016=CARTESIAN_POINT('Ctrl Pts',(-15.4999999999999,-17.324699114,9.11199729419368));
#33017=CARTESIAN_POINT('Ctrl Pts',(-14.7098821065065,-16.8685243355,9.07033062752701));
#33018=CARTESIAN_POINT('Ctrl Pts',(-13.9197642130131,-16.412349557,9.02866396086034));
#33019=CARTESIAN_POINT('Ctrl Pts',(-13.9197642130131,-15.5,8.98699729419367));
#33020=CARTESIAN_POINT('Ctrl Pts',(-13.9197642130131,-14.5876504430001,
8.94533062752701));
#33021=CARTESIAN_POINT('Ctrl Pts',(-14.7098821065065,-14.1314756645001,
8.90366396086034));
#33022=CARTESIAN_POINT('Ctrl Pts',(-15.5,-13.6753008860002,8.86199729419367));
#33023=CARTESIAN_POINT('Ctrl Pts',(-16.2901178934934,-14.1314756645001,
8.820330627527));
#33024=CARTESIAN_POINT('Ctrl Pts',(-17.0802357869868,-14.5876504430001,
8.77866396086034));
#33025=CARTESIAN_POINT('Ctrl Pts',(-17.0802357869868,-15.5000000000001,
8.73699729419367));
#33026=CARTESIAN_POINT('Ctrl Pts',(-17.0802357869868,-16.412349557,8.695330627527));
#33027=CARTESIAN_POINT('Ctrl Pts',(-16.2901178934934,-16.8685243355,8.65366396086033));
#33028=CARTESIAN_POINT('Ctrl Pts',(-15.4999999999999,-17.324699114,8.61199729419367));
#33029=CARTESIAN_POINT('Ctrl Pts',(-14.7098821065065,-16.8685243355,8.570330627527));
#33030=CARTESIAN_POINT('Ctrl Pts',(-13.9197642130131,-16.412349557,8.52866396086033));
#33031=CARTESIAN_POINT('Ctrl Pts',(-13.9197642130131,-15.5,8.48699729419366));
#33032=CARTESIAN_POINT('Ctrl Pts',(-13.9197642130131,-14.5876504430001,
8.445330627527));
#33033=CARTESIAN_POINT('Ctrl Pts',(-14.7098821065065,-14.1314756645001,
8.40366396086033));
#33034=CARTESIAN_POINT('Ctrl Pts',(-15.5,-13.6753008860002,8.36199729419366));
#33035=CARTESIAN_POINT('Ctrl Pts',(-16.2901178934934,-14.1314756645001,
8.320330627527));
#33036=CARTESIAN_POINT('Ctrl Pts',(-17.0802357869868,-14.5876504430001,
8.27866396086033));
#33037=CARTESIAN_POINT('Ctrl Pts',(-17.0802357869868,-15.5000000000001,
8.23699729419366));
#33038=CARTESIAN_POINT('Ctrl Pts',(-17.0802357869868,-16.412349557,8.19533062752699));
#33039=CARTESIAN_POINT('Ctrl Pts',(-16.2901178934934,-16.8685243355,8.15366396086033));
#33040=CARTESIAN_POINT('Ctrl Pts',(-15.4999999999999,-17.324699114,8.11199729419366));
#33041=CARTESIAN_POINT('Ctrl Pts',(-14.7098821065065,-16.8685243355,8.07033062752699));
#33042=CARTESIAN_POINT('Ctrl Pts',(-13.9197642130131,-16.412349557,8.02866396086033));
#33043=CARTESIAN_POINT('Ctrl Pts',(-13.9197642130131,-15.5,7.98699729419366));
#33044=CARTESIAN_POINT('Ctrl Pts',(-13.9197642130131,-14.5876504430001,
7.94533062752699));
#33045=CARTESIAN_POINT('Ctrl Pts',(-14.7098821065065,-14.1314756645001,
7.90366396086032));
#33046=CARTESIAN_POINT('Ctrl Pts',(-15.5,-13.6753008860002,7.86199729419366));
#33047=CARTESIAN_POINT('Ctrl Pts',(-16.2901178934934,-14.1314756645001,
7.82033062752699));
#33048=CARTESIAN_POINT('Ctrl Pts',(-17.0802357869868,-14.5876504430001,
7.77866396086032));
#33049=CARTESIAN_POINT('Ctrl Pts',(-17.0802357869868,-15.5000000000001,
7.73699729419366));
#33050=CARTESIAN_POINT('Ctrl Pts',(-17.0802357869868,-16.412349557,7.69533062752699));
#33051=CARTESIAN_POINT('Ctrl Pts',(-16.2901178934934,-16.8685243355,7.65366396086032));
#33052=CARTESIAN_POINT('Ctrl Pts',(-15.4999999999999,-17.324699114,7.61199729419365));
#33053=CARTESIAN_POINT('Ctrl Pts',(-14.7098821065065,-16.8685243355,7.57033062752699));
#33054=CARTESIAN_POINT('Ctrl Pts',(-13.9197642130131,-16.412349557,7.52866396086032));
#33055=CARTESIAN_POINT('Ctrl Pts',(-13.9197642130131,-15.5,7.48699729419365));
#33056=CARTESIAN_POINT('Ctrl Pts',(-13.9197642130131,-14.5876504430001,
7.44533062752699));
#33057=CARTESIAN_POINT('Ctrl Pts',(-14.7098821065065,-14.1314756645001,
7.40366396086032));
#33058=CARTESIAN_POINT('Ctrl Pts',(-15.5,-13.6753008860002,7.36199729419365));
#33059=CARTESIAN_POINT('Ctrl Pts',(-16.2901178934934,-14.1314756645001,
7.32033062752699));
#33060=CARTESIAN_POINT('Ctrl Pts',(-17.0802357869868,-14.5876504430001,
7.27866396086032));
#33061=CARTESIAN_POINT('Ctrl Pts',(-17.0802357869868,-15.5000000000001,
7.23699729419365));
#33062=CARTESIAN_POINT('Ctrl Pts',(-17.0802357869868,-16.412349557,7.19533062752698));
#33063=CARTESIAN_POINT('Ctrl Pts',(-16.2901178934934,-16.8685243355,7.15366396086031));
#33064=CARTESIAN_POINT('Ctrl Pts',(-15.4999999999999,-17.324699114,7.11199729419365));
#33065=CARTESIAN_POINT('Ctrl Pts',(-14.7098821065065,-16.8685243355,7.07033062752698));
#33066=CARTESIAN_POINT('Ctrl Pts',(-13.9197642130131,-16.412349557,7.02866396086031));
#33067=CARTESIAN_POINT('Ctrl Pts',(-13.9197642130131,-15.5,6.98699729419364));
#33068=CARTESIAN_POINT('Ctrl Pts',(-13.9197642130131,-14.5876504430001,
6.94533062752698));
#33069=CARTESIAN_POINT('Ctrl Pts',(-14.7098821065065,-14.1314756645001,
6.90366396086031));
#33070=CARTESIAN_POINT('Ctrl Pts',(-15.5,-13.6753008860002,6.86199729419364));
#33071=CARTESIAN_POINT('Ctrl Pts',(-16.2901178934934,-14.1314756645001,
6.82033062752698));
#33072=CARTESIAN_POINT('Ctrl Pts',(-17.0802357869868,-14.5876504430001,
6.77866396086031));
#33073=CARTESIAN_POINT('Ctrl Pts',(-17.0802357869868,-15.5000000000001,
6.73699729419364));
#33074=CARTESIAN_POINT('Ctrl Pts',(-17.0802357869868,-16.412349557,6.69533062752697));
#33075=CARTESIAN_POINT('Ctrl Pts',(-16.2901178934934,-16.8685243355,6.65366396086031));
#33076=CARTESIAN_POINT('Ctrl Pts',(-15.4999999999999,-17.324699114,6.61199729419364));
#33077=CARTESIAN_POINT('Ctrl Pts',(-14.7098821065065,-16.8685243355,6.57033062752697));
#33078=CARTESIAN_POINT('Ctrl Pts',(-13.9197642130131,-16.412349557,6.52866396086031));
#33079=CARTESIAN_POINT('Ctrl Pts',(-13.9197642130131,-15.5,6.48699729419364));
#33080=CARTESIAN_POINT('Ctrl Pts',(-13.9197642130131,-14.5876504430001,
6.44533062752697));
#33081=CARTESIAN_POINT('Ctrl Pts',(-14.7098821065065,-14.1314756645001,
6.40366396086031));
#33082=CARTESIAN_POINT('Ctrl Pts',(-15.5,-13.6753008860002,6.36199729419364));
#33083=CARTESIAN_POINT('Ctrl Pts',(-16.2901178934934,-14.1314756645001,
6.32033062752697));
#33084=CARTESIAN_POINT('Ctrl Pts',(-17.0802357869868,-14.5876504430001,
6.2786639608603));
#33085=CARTESIAN_POINT('Ctrl Pts',(-17.0802357869868,-15.5000000000001,
6.23699729419364));
#33086=CARTESIAN_POINT('Ctrl Pts',(-17.0802357869868,-16.412349557,6.19533062752697));
#33087=CARTESIAN_POINT('Ctrl Pts',(-16.2901178934934,-16.8685243355,6.1536639608603));
#33088=CARTESIAN_POINT('Ctrl Pts',(-15.4999999999999,-17.324699114,6.11199729419363));
#33089=CARTESIAN_POINT('Ctrl Pts',(-14.7098821065065,-16.8685243355,6.07033062752697));
#33090=CARTESIAN_POINT('Ctrl Pts',(-13.9197642130131,-16.412349557,6.0286639608603));
#33091=CARTESIAN_POINT('Ctrl Pts',(-13.9197642130131,-15.5,5.98699729419363));
#33092=CARTESIAN_POINT('Ctrl Pts',(-13.9197642130131,-14.5876504430001,
5.94533062752696));
#33093=CARTESIAN_POINT('Ctrl Pts',(-14.7098821065065,-14.1314756645001,
5.9036639608603));
#33094=CARTESIAN_POINT('Ctrl Pts',(-15.5,-13.6753008860002,5.86199729419363));
#33095=CARTESIAN_POINT('Ctrl Pts',(-16.2901178934934,-14.1314756645001,
5.82033062752696));
#33096=CARTESIAN_POINT('Ctrl Pts',(-17.0802357869868,-14.5876504430001,
5.7786639608603));
#33097=CARTESIAN_POINT('Ctrl Pts',(-17.0802357869868,-15.5000000000001,
5.73699729419363));
#33098=CARTESIAN_POINT('Ctrl Pts',(-17.0802357869868,-16.412349557,5.69533062752696));
#33099=CARTESIAN_POINT('Ctrl Pts',(-16.2901178934934,-16.8685243355,5.65366396086029));
#33100=CARTESIAN_POINT('Ctrl Pts',(-15.4999999999999,-17.324699114,5.61199729419363));
#33101=CARTESIAN_POINT('Ctrl Pts',(-14.7098821065065,-16.8685243355,5.57033062752696));
#33102=CARTESIAN_POINT('Ctrl Pts',(-13.9197642130131,-16.412349557,5.52866396086029));
#33103=CARTESIAN_POINT('Ctrl Pts',(-13.9197642130131,-15.5,5.48699729419363));
#33104=CARTESIAN_POINT('Ctrl Pts',(-13.9197642130131,-14.5876504430001,
5.44533062752696));
#33105=CARTESIAN_POINT('Ctrl Pts',(-14.7098821065065,-14.1314756645001,
5.40366396086029));
#33106=CARTESIAN_POINT('Ctrl Pts',(-15.5,-13.6753008860002,5.36199729419362));
#33107=CARTESIAN_POINT('Ctrl Pts',(-16.2901178934934,-14.1314756645001,
5.32033062752696));
#33108=CARTESIAN_POINT('Ctrl Pts',(-17.0802357869868,-14.5876504430001,
5.27866396086029));
#33109=CARTESIAN_POINT('Ctrl Pts',(-17.0802357869868,-15.5000000000001,
5.23699729419362));
#33110=CARTESIAN_POINT('Ctrl Pts',(-17.0802357869868,-16.412349557,5.19533062752695));
#33111=CARTESIAN_POINT('Ctrl Pts',(-16.2901178934934,-16.8685243355,5.15366396086029));
#33112=CARTESIAN_POINT('Ctrl Pts',(-15.4999999999999,-17.324699114,5.11199729419362));
#33113=CARTESIAN_POINT('Ctrl Pts',(-14.7098821065065,-16.8685243355,5.07033062752695));
#33114=CARTESIAN_POINT('Ctrl Pts',(-13.9197642130131,-16.412349557,5.02866396086029));
#33115=CARTESIAN_POINT('Ctrl Pts',(-13.9197642130131,-15.5,4.98699729419362));
#33116=CARTESIAN_POINT('Ctrl Pts',(-13.9197642130131,-14.5876504430001,
4.94533062752695));
#33117=CARTESIAN_POINT('Ctrl Pts',(-14.7098821065065,-14.1314756645001,
4.90366396086028));
#33118=CARTESIAN_POINT('Ctrl Pts',(-15.5,-13.6753008860002,4.86199729419362));
#33119=CARTESIAN_POINT('Ctrl Pts',(-16.2901178934934,-14.1314756645001,
4.82033062752695));
#33120=CARTESIAN_POINT('Ctrl Pts',(-17.0802357869868,-14.5876504430001,
4.77866396086028));
#33121=CARTESIAN_POINT('Ctrl Pts',(-17.0802357869868,-15.5000000000001,
4.73699729419362));
#33122=CARTESIAN_POINT('Ctrl Pts',(-17.0802357869868,-16.412349557,4.69533062752695));
#33123=CARTESIAN_POINT('Ctrl Pts',(-16.2901178934934,-16.8685243355,4.65366396086028));
#33124=CARTESIAN_POINT('Ctrl Pts',(-15.4999999999999,-17.324699114,4.61199729419361));
#33125=CARTESIAN_POINT('Ctrl Pts',(-14.7098821065065,-16.8685243355,4.57033062752695));
#33126=CARTESIAN_POINT('Ctrl Pts',(-13.9197642130131,-16.412349557,4.52866396086028));
#33127=CARTESIAN_POINT('Ctrl Pts',(-13.9197642130131,-15.5,4.48699729419361));
#33128=CARTESIAN_POINT('Ctrl Pts',(-13.9197642130131,-14.5876504430001,
4.44533062752694));
#33129=CARTESIAN_POINT('Ctrl Pts',(-14.7098821065065,-14.1314756645001,
4.40366396086028));
#33130=CARTESIAN_POINT('Ctrl Pts',(-15.5,-13.6753008860002,4.36199729419361));
#33131=CARTESIAN_POINT('Ctrl Pts',(-16.2901178934934,-14.1314756645001,
4.32033062752694));
#33132=CARTESIAN_POINT('Ctrl Pts',(-17.0802357869868,-14.5876504430001,
4.27866396086028));
#33133=CARTESIAN_POINT('Ctrl Pts',(-17.0802357869868,-15.5000000000001,
4.23699729419361));
#33134=CARTESIAN_POINT('Ctrl Pts',(-17.0802357869868,-16.412349557,4.19533062752694));
#33135=CARTESIAN_POINT('Ctrl Pts',(-16.2901178934934,-16.8685243355,4.15366396086027));
#33136=CARTESIAN_POINT('Ctrl Pts',(-15.4999999999999,-17.324699114,4.11199729419361));
#33137=CARTESIAN_POINT('Ctrl Pts',(-14.7098821065065,-16.8685243355,4.07033062752694));
#33138=CARTESIAN_POINT('Ctrl Pts',(-13.9197642130131,-16.412349557,4.02866396086027));
#33139=CARTESIAN_POINT('Ctrl Pts',(-13.9197642130131,-15.5,3.9869972941936));
#33140=CARTESIAN_POINT('Ctrl Pts',(-13.9197642130131,-14.5876504430001,
3.94533062752694));
#33141=CARTESIAN_POINT('Ctrl Pts',(-14.7098821065065,-14.1314756645001,
3.90366396086027));
#33142=CARTESIAN_POINT('Ctrl Pts',(-15.5,-13.6753008860002,3.8619972941936));
#33143=CARTESIAN_POINT('Ctrl Pts',(-16.2901178934934,-14.1314756645001,
3.82033062752694));
#33144=CARTESIAN_POINT('Ctrl Pts',(-17.0802357869868,-14.5876504430001,
3.77866396086027));
#33145=CARTESIAN_POINT('Ctrl Pts',(-17.0802357869868,-15.5000000000001,
3.7369972941936));
#33146=CARTESIAN_POINT('Ctrl Pts',(-17.0802357869868,-16.412349557,3.69533062752693));
#33147=CARTESIAN_POINT('Ctrl Pts',(-16.2901178934934,-16.8685243355,3.65366396086027));
#33148=CARTESIAN_POINT('Ctrl Pts',(-15.4999999999999,-17.324699114,3.6119972941936));
#33149=CARTESIAN_POINT('Ctrl Pts',(-14.7098821065065,-16.8685243355,3.57033062752693));
#33150=CARTESIAN_POINT('Ctrl Pts',(-13.9197642130131,-16.412349557,3.52866396086027));
#33151=CARTESIAN_POINT('Ctrl Pts',(-13.9197642130131,-15.5,3.4869972941936));
#33152=CARTESIAN_POINT('Ctrl Pts',(-13.9197642130131,-14.5876504430001,
3.44533062752693));
#33153=CARTESIAN_POINT('Ctrl Pts',(-14.7098821065065,-14.1314756645001,
3.40366396086026));
#33154=CARTESIAN_POINT('Ctrl Pts',(-15.5,-13.6753008860002,3.3619972941936));
#33155=CARTESIAN_POINT('Ctrl Pts',(-16.2901178934934,-14.1314756645001,
3.32033062752693));
#33156=CARTESIAN_POINT('Ctrl Pts',(-17.0802357869868,-14.5876504430001,
3.27866396086026));
#33157=CARTESIAN_POINT('Ctrl Pts',(-17.0802357869868,-15.5000000000001,
3.2369972941936));
#33158=CARTESIAN_POINT('Ctrl Pts',(-17.0802357869868,-16.412349557,3.19533062752693));
#33159=CARTESIAN_POINT('Ctrl Pts',(-16.2901178934934,-16.8685243355,3.15366396086026));
#33160=CARTESIAN_POINT('Ctrl Pts',(-15.4999999999999,-17.324699114,3.11199729419359));
#33161=CARTESIAN_POINT('Ctrl Pts',(-14.7098821065065,-16.8685243355,3.07033062752693));
#33162=CARTESIAN_POINT('Ctrl Pts',(-13.9197642130131,-16.412349557,3.02866396086026));
#33163=CARTESIAN_POINT('Ctrl Pts',(-13.9197642130131,-15.5,2.98699729419359));
#33164=CARTESIAN_POINT('Ctrl Pts',(-13.9197642130131,-14.5876504430001,
2.94533062752692));
#33165=CARTESIAN_POINT('Ctrl Pts',(-14.7098821065065,-14.1314756645001,
2.90366396086026));
#33166=CARTESIAN_POINT('Ctrl Pts',(-15.5,-13.6753008860002,2.86199729419359));
#33167=CARTESIAN_POINT('Ctrl Pts',(-16.2901178934934,-14.1314756645001,
2.82033062752692));
#33168=CARTESIAN_POINT('Ctrl Pts',(-17.0802357869868,-14.5876504430001,
2.77866396086026));
#33169=CARTESIAN_POINT('Ctrl Pts',(-17.0802357869868,-15.5000000000001,
2.73699729419359));
#33170=CARTESIAN_POINT('Ctrl Pts',(-17.0802357869868,-16.412349557,2.69533062752692));
#33171=CARTESIAN_POINT('Ctrl Pts',(-16.2901178934934,-16.8685243355,2.65366396086025));
#33172=CARTESIAN_POINT('Ctrl Pts',(-15.4999999999999,-17.324699114,2.61199729419359));
#33173=CARTESIAN_POINT('Ctrl Pts',(-14.7098821065065,-16.8685243355,2.57033062752692));
#33174=CARTESIAN_POINT('Ctrl Pts',(-13.9197642130131,-16.412349557,2.52866396086025));
#33175=CARTESIAN_POINT('Ctrl Pts',(-13.9197642130131,-15.5,2.48699729419358));
#33176=CARTESIAN_POINT('Ctrl Pts',(-13.9197642130131,-14.5876504430001,
2.44533062752692));
#33177=CARTESIAN_POINT('Ctrl Pts',(-14.7098821065065,-14.1314756645001,
2.40366396086025));
#33178=CARTESIAN_POINT('Ctrl Pts',(-15.5,-13.6753008860002,2.36199729419358));
#33179=CARTESIAN_POINT('Ctrl Pts',(-16.2901178934934,-14.1314756645001,
2.32033062752692));
#33180=CARTESIAN_POINT('Ctrl Pts',(-17.0802357869868,-14.5876504430001,
2.27866396086025));
#33181=CARTESIAN_POINT('Ctrl Pts',(-17.0802357869868,-15.5000000000001,
2.23699729419358));
#33182=CARTESIAN_POINT('Ctrl Pts',(-17.0802357869868,-16.412349557,2.19533062752692));
#33183=CARTESIAN_POINT('Ctrl Pts',(-16.2901178934934,-16.8685243355,2.15366396086025));
#33184=CARTESIAN_POINT('Ctrl Pts',(-15.4999999999999,-17.324699114,2.11199729419358));
#33185=CARTESIAN_POINT('Ctrl Pts',(-14.7098821065065,-16.8685243355,2.07033062752691));
#33186=CARTESIAN_POINT('Ctrl Pts',(-13.9197642130131,-16.412349557,2.02866396086025));
#33187=CARTESIAN_POINT('Ctrl Pts',(-13.9197642130131,-15.5,1.98699729419358));
#33188=CARTESIAN_POINT('Ctrl Pts',(-13.9197642130131,-14.5876504430001,
1.94533062752691));
#33189=CARTESIAN_POINT('Ctrl Pts',(-14.7098821065065,-14.1314756645001,
1.90366396086024));
#33190=CARTESIAN_POINT('Ctrl Pts',(-15.5,-13.6753008860002,1.86199729419358));
#33191=CARTESIAN_POINT('Ctrl Pts',(-16.2901178934934,-14.1314756645001,
1.82033062752691));
#33192=CARTESIAN_POINT('Ctrl Pts',(-17.0802357869868,-14.5876504430001,
1.77866396086024));
#33193=CARTESIAN_POINT('Ctrl Pts',(-17.0802357869868,-15.5000000000001,
1.73699729419358));
#33194=CARTESIAN_POINT('Ctrl Pts',(-17.0802357869868,-16.412349557,1.69533062752691));
#33195=CARTESIAN_POINT('Ctrl Pts',(-16.2901178934934,-16.8685243355,1.65366396086024));
#33196=CARTESIAN_POINT('Ctrl Pts',(-15.4999999999999,-17.324699114,1.61199729419357));
#33197=CARTESIAN_POINT('Ctrl Pts',(-14.7098821065065,-16.8685243355,1.57033062752691));
#33198=CARTESIAN_POINT('Ctrl Pts',(-13.9197642130131,-16.412349557,1.52866396086024));
#33199=CARTESIAN_POINT('Ctrl Pts',(-13.9197642130131,-15.5,1.48699729419357));
#33200=CARTESIAN_POINT('Ctrl Pts',(-13.9197642130131,-14.5876504430001,
1.4453306275269));
#33201=CARTESIAN_POINT('Ctrl Pts',(-14.7098821065065,-14.1314756645001,
1.40366396086024));
#33202=CARTESIAN_POINT('Ctrl Pts',(-15.5,-13.6753008860002,1.36199729419357));
#33203=CARTESIAN_POINT('Ctrl Pts',(-16.2901178934934,-14.1314756645001,
1.3203306275269));
#33204=CARTESIAN_POINT('Ctrl Pts',(-17.0802357869868,-14.5876504430001,
1.27866396086024));
#33205=CARTESIAN_POINT('Ctrl Pts',(-17.0802357869868,-15.5000000000001,
1.23699729419357));
#33206=CARTESIAN_POINT('Ctrl Pts',(-17.0802357869868,-16.412349557,1.1953306275269));
#33207=CARTESIAN_POINT('Ctrl Pts',(-16.2901178934934,-16.8685243355,1.15366396086024));
#33208=CARTESIAN_POINT('Ctrl Pts',(-15.4999999999999,-17.324699114,1.11199729419357));
#33209=CARTESIAN_POINT('Ctrl Pts',(-14.7098821065065,-16.8685243355,1.0703306275269));
#33210=CARTESIAN_POINT('Ctrl Pts',(-13.9197642130131,-16.412349557,1.02866396086023));
#33211=CARTESIAN_POINT('Ctrl Pts',(-13.9197642130131,-15.5,0.986997294193569));
#33212=CARTESIAN_POINT('Ctrl Pts',(-13.9197642130131,-14.5876504430001,
0.945330627526902));
#33213=CARTESIAN_POINT('Ctrl Pts',(-14.7098821065065,-14.1314756645001,
0.903663960860235));
#33214=CARTESIAN_POINT('Ctrl Pts',(-15.5,-13.6753008860002,0.861997294193567));
#33215=CARTESIAN_POINT('Ctrl Pts',(-16.2901178934934,-14.1314756645001,
0.8203306275269));
#33216=CARTESIAN_POINT('Ctrl Pts',(-17.0802357869868,-14.5876504430001,
0.778663960860232));
#33217=CARTESIAN_POINT('Ctrl Pts',(-17.0802357869868,-15.5000000000001,
0.736997294193565));
#33218=CARTESIAN_POINT('Ctrl Pts',(-17.0802357869868,-16.412349557,0.695330627526898));
#33219=CARTESIAN_POINT('Ctrl Pts',(-16.2901178934934,-16.8685243355,0.653663960860231));
#33220=CARTESIAN_POINT('Ctrl Pts',(-15.4999999999999,-17.324699114,0.611997294193563));
#33221=CARTESIAN_POINT('Ctrl Pts',(-14.7098821065065,-16.8685243355,0.570330627526896));
#33222=CARTESIAN_POINT('Ctrl Pts',(-13.9197642130131,-16.412349557,0.528663960860229));
#33223=CARTESIAN_POINT('Ctrl Pts',(-13.9197642130131,-15.5,0.486997294193562));
#33224=CARTESIAN_POINT('Ctrl Pts',(-13.9197642130131,-14.5876504430001,
0.445330627526894));
#33225=CARTESIAN_POINT('Ctrl Pts',(-14.7098821065065,-14.1314756645001,
0.403663960860227));
#33226=CARTESIAN_POINT('Ctrl Pts',(-15.5,-13.6753008860002,0.36199729419356));
#33227=CARTESIAN_POINT('Ctrl Pts',(-16.2901178934934,-14.1314756645001,
0.320330627526892));
#33228=CARTESIAN_POINT('Ctrl Pts',(-17.0802357869868,-14.5876504430001,
0.278663960860225));
#33229=CARTESIAN_POINT('Ctrl Pts',(-17.0802357869868,-15.5000000000001,
0.236997294193558));
#33230=CARTESIAN_POINT('Ctrl Pts',(-17.0802357869868,-16.412349557,0.195330627526891));
#33231=CARTESIAN_POINT('Ctrl Pts',(-16.2901178934934,-16.8685243355,0.153663960860223));
#33232=CARTESIAN_POINT('Ctrl Pts',(-15.4999999999999,-17.324699114,0.111997294193556));
#33233=CARTESIAN_POINT('Ctrl Pts',(-14.7098821065065,-16.8685243355,0.0703306275268884));
#33234=CARTESIAN_POINT('Ctrl Pts',(-13.9197642130131,-16.412349557,0.0286639608602211));
#33235=CARTESIAN_POINT('Ctrl Pts',(-13.9197642130131,-15.5,-0.0130027058064461));
#33236=CARTESIAN_POINT('Ctrl Pts',(-13.9197642130131,-14.5876504430001,
-0.0546693724731117));
#33237=CARTESIAN_POINT('Ctrl Pts',(-14.7098821065065,-14.1314756645001,
-0.096336039139779));
#33238=CARTESIAN_POINT('Ctrl Pts',(-15.5,-13.6753008860002,-0.138002705806446));
#33239=CARTESIAN_POINT('Ctrl Pts',(-16.2901178934934,-14.1314756645001,
-0.179669372473113));
#33240=CARTESIAN_POINT('Ctrl Pts',(-17.0802357869868,-14.5876504430001,
-0.221336039139781));
#33241=CARTESIAN_POINT('Ctrl Pts',(-17.0802357869868,-15.5000000000001,
-0.263002705806448));
#33242=CARTESIAN_POINT('Ctrl Pts',(-17.0802357869868,-16.412349557,-0.304669372473115));
#33243=CARTESIAN_POINT('Ctrl Pts',(-16.2901178934934,-16.8685243355,-0.346336039139782));
#33244=CARTESIAN_POINT('Ctrl Pts',(-15.4999999999999,-17.324699114,-0.38800270580645));
#33245=CARTESIAN_POINT('Ctrl Pts',(-14.7098821065065,-16.8685243355,-0.429669372473117));
#33246=CARTESIAN_POINT('Ctrl Pts',(-13.9197642130131,-16.412349557,-0.471336039139784));
#33247=CARTESIAN_POINT('Ctrl Pts',(-13.9197642130131,-15.5,-0.513002705806452));
#33248=CARTESIAN_POINT('Ctrl Pts',(-13.9197642130131,-14.5876504430001,
-0.554669372473119));
#33249=CARTESIAN_POINT('Ctrl Pts',(-14.7098821065065,-14.1314756645001,
-0.596336039139786));
#33250=CARTESIAN_POINT('Ctrl Pts',(-15.5,-13.6753008860002,-0.638002705806453));
#33251=CARTESIAN_POINT('Ctrl Pts',(-16.2901178934934,-14.1314756645001,
-0.679669372473122));
#33252=CARTESIAN_POINT('Ctrl Pts',(-17.0802357869868,-14.5876504430001,
-0.721336039139788));
#33253=CARTESIAN_POINT('Ctrl Pts',(-17.0802357869868,-15.5000000000001,
-0.763002705806455));
#33254=CARTESIAN_POINT('Ctrl Pts',(-17.0802357869868,-16.412349557,-0.804669372473123));
#33255=CARTESIAN_POINT('Ctrl Pts',(-16.2901178934934,-16.8685243355,-0.84633603913979));
#33256=CARTESIAN_POINT('Ctrl Pts',(-15.4999999999999,-17.324699114,-0.888002705806457));
#33257=CARTESIAN_POINT('Ctrl Pts',(-14.7098821065065,-16.8685243355,-0.929669372473124));
#33258=CARTESIAN_POINT('Ctrl Pts',(-13.9197642130131,-16.412349557,-0.971336039139791));
#33259=CARTESIAN_POINT('Ctrl Pts',(-13.9197642130131,-15.5,-1.01300270580646));
#33260=CARTESIAN_POINT('Ctrl Pts',(-13.9197642130131,-14.5876504430001,
-1.05466937247313));
#33261=CARTESIAN_POINT('Ctrl Pts',(-14.7098821065065,-14.1314756645001,
-1.0963360391398));
#33262=CARTESIAN_POINT('Ctrl Pts',(-15.5,-13.6753008860002,-1.13800270580646));
#33263=CARTESIAN_POINT('Ctrl Pts',(-16.2901178934934,-14.1314756645001,
-1.17966937247313));
#33264=CARTESIAN_POINT('Ctrl Pts',(-17.0802357869868,-14.5876504430001,
-1.2213360391398));
#33265=CARTESIAN_POINT('Ctrl Pts',(-17.0802357869868,-15.5000000000001,
-1.26300270580646));
#33266=CARTESIAN_POINT('Ctrl Pts',(-17.0802357869868,-16.412349557,-1.30466937247313));
#33267=CARTESIAN_POINT('Ctrl Pts',(-16.2901178934934,-16.8685243355,-1.3463360391398));
#33268=CARTESIAN_POINT('Ctrl Pts',(-15.4999999999999,-17.324699114,-1.38800270580647));
#33269=CARTESIAN_POINT('Ctrl Pts',(-14.7098821065065,-16.8685243355,-1.42966937247313));
#33270=CARTESIAN_POINT('Ctrl Pts',(-13.9197642130131,-16.412349557,-1.4713360391398));
#33271=CARTESIAN_POINT('Ctrl Pts',(-13.9197642130131,-15.5,-1.51300270580647));
#33272=CARTESIAN_POINT('Ctrl Pts',(-13.9197642130131,-14.5876504430001,
-1.55466937247313));
#33273=CARTESIAN_POINT('Ctrl Pts',(-14.7098821065065,-14.1314756645001,
-1.5963360391398));
#33274=CARTESIAN_POINT('Ctrl Pts',(-15.5,-13.6753008860002,-1.63800270580647));
#33275=CARTESIAN_POINT('Ctrl Pts',(-16.2901178934934,-14.1314756645001,
-1.67966937247314));
#33276=CARTESIAN_POINT('Ctrl Pts',(-17.0802357869868,-14.5876504430001,
-1.7213360391398));
#33277=CARTESIAN_POINT('Ctrl Pts',(-17.0802357869868,-15.5000000000001,
-1.76300270580647));
#33278=CARTESIAN_POINT('Ctrl Pts',(-17.0802357869868,-16.412349557,-1.80466937247314));
#33279=CARTESIAN_POINT('Ctrl Pts',(-16.2901178934934,-16.8685243355,-1.84633603913981));
#33280=CARTESIAN_POINT('Ctrl Pts',(-15.4999999999999,-17.324699114,-1.88800270580647));
#33281=CARTESIAN_POINT('Ctrl Pts',(-14.7098821065065,-16.8685243355,-1.92966937247314));
#33282=CARTESIAN_POINT('Ctrl Pts',(-14.4189874290231,-16.700576215149,-1.94500962949253));
#33283=CARTESIAN_POINT('Ctrl Pts',(-14.2215547953297,-16.4288288330633,
-1.96262601180163));
#33284=CARTESIAN_POINT('',(-14.2215509627456,-16.4288315898517,-1.96262324186735));
#33285=CARTESIAN_POINT('',(-14.2215500160356,-16.4288304039466,-1.96262332703659));
#33286=CARTESIAN_POINT('Ctrl Pts',(-14.5577749122402,-14.2313898004749,
10.4122404735808));
#33287=CARTESIAN_POINT('Ctrl Pts',(-14.6309457974487,-14.1770441521709,
10.407829216981));
#33288=CARTESIAN_POINT('Ctrl Pts',(-14.7098797632095,-14.1314716057907,
10.4036666666667));
#33289=CARTESIAN_POINT('Ctrl Pts',(-15.5,-13.6752954743876,10.362));
#33290=CARTESIAN_POINT('Ctrl Pts',(-16.2901202367904,-14.1314716057907,
10.3203333333333));
#33291=CARTESIAN_POINT('Ctrl Pts',(-17.0802404735808,-14.5876477371938,
10.2786666666667));
#33292=CARTESIAN_POINT('Ctrl Pts',(-17.0802404735808,-15.5000000000001,
10.237));
#33293=CARTESIAN_POINT('Ctrl Pts',(-17.0802404735808,-16.4123522628063,
10.1953333333333));
#33294=CARTESIAN_POINT('Ctrl Pts',(-16.2901202367904,-16.8685283942094,
10.1536666666667));
#33295=CARTESIAN_POINT('Ctrl Pts',(-15.4999999999999,-17.3247045256125,
10.112));
#33296=CARTESIAN_POINT('Ctrl Pts',(-14.7098797632095,-16.8685283942094,
10.0703333333333));
#33297=CARTESIAN_POINT('Ctrl Pts',(-13.9197595264191,-16.4123522628063,
10.0286666666667));
#33298=CARTESIAN_POINT('Ctrl Pts',(-13.9197595264191,-15.5,9.98699999999998));
#33299=CARTESIAN_POINT('Ctrl Pts',(-13.9197595264191,-14.5876477371938,
9.94533333333331));
#33300=CARTESIAN_POINT('Ctrl Pts',(-14.7098797632095,-14.1314716057907,
9.90366666666665));
#33301=CARTESIAN_POINT('Ctrl Pts',(-15.5,-13.6752954743876,9.86199999999998));
#33302=CARTESIAN_POINT('Ctrl Pts',(-16.2901202367904,-14.1314716057907,
9.82033333333331));
#33303=CARTESIAN_POINT('Ctrl Pts',(-17.0802404735808,-14.5876477371938,
9.77866666666665));
#33304=CARTESIAN_POINT('Ctrl Pts',(-17.0802404735808,-15.5000000000001,
9.73699999999998));
#33305=CARTESIAN_POINT('Ctrl Pts',(-17.0802404735808,-16.4123522628063,
9.69533333333331));
#33306=CARTESIAN_POINT('Ctrl Pts',(-16.2901202367904,-16.8685283942094,
9.65366666666664));
#33307=CARTESIAN_POINT('Ctrl Pts',(-15.4999999999999,-17.3247045256125,
9.61199999999998));
#33308=CARTESIAN_POINT('Ctrl Pts',(-14.7098797632095,-16.8685283942094,
9.57033333333331));
#33309=CARTESIAN_POINT('Ctrl Pts',(-13.9197595264191,-16.4123522628063,
9.52866666666664));
#33310=CARTESIAN_POINT('Ctrl Pts',(-13.9197595264191,-15.5,9.48699999999998));
#33311=CARTESIAN_POINT('Ctrl Pts',(-13.9197595264191,-14.5876477371938,
9.44533333333331));
#33312=CARTESIAN_POINT('Ctrl Pts',(-14.7098797632095,-14.1314716057907,
9.40366666666664));
#33313=CARTESIAN_POINT('Ctrl Pts',(-15.5,-13.6752954743876,9.36199999999998));
#33314=CARTESIAN_POINT('Ctrl Pts',(-16.2901202367904,-14.1314716057907,
9.32033333333331));
#33315=CARTESIAN_POINT('Ctrl Pts',(-17.0802404735808,-14.5876477371938,
9.27866666666664));
#33316=CARTESIAN_POINT('Ctrl Pts',(-17.0802404735808,-15.5000000000001,
9.23699999999997));
#33317=CARTESIAN_POINT('Ctrl Pts',(-17.0802404735808,-16.4123522628063,
9.19533333333331));
#33318=CARTESIAN_POINT('Ctrl Pts',(-16.2901202367904,-16.8685283942094,
9.15366666666664));
#33319=CARTESIAN_POINT('Ctrl Pts',(-15.4999999999999,-17.3247045256125,
9.11199999999997));
#33320=CARTESIAN_POINT('Ctrl Pts',(-14.7098797632095,-16.8685283942094,
9.0703333333333));
#33321=CARTESIAN_POINT('Ctrl Pts',(-13.9197595264191,-16.4123522628063,
9.02866666666664));
#33322=CARTESIAN_POINT('Ctrl Pts',(-13.9197595264191,-15.5,8.98699999999997));
#33323=CARTESIAN_POINT('Ctrl Pts',(-13.9197595264191,-14.5876477371938,
8.9453333333333));
#33324=CARTESIAN_POINT('Ctrl Pts',(-14.7098797632095,-14.1314716057907,
8.90366666666664));
#33325=CARTESIAN_POINT('Ctrl Pts',(-15.5,-13.6752954743876,8.86199999999997));
#33326=CARTESIAN_POINT('Ctrl Pts',(-16.2901202367904,-14.1314716057907,
8.8203333333333));
#33327=CARTESIAN_POINT('Ctrl Pts',(-17.0802404735808,-14.5876477371938,
8.77866666666663));
#33328=CARTESIAN_POINT('Ctrl Pts',(-17.0802404735808,-15.5000000000001,
8.73699999999997));
#33329=CARTESIAN_POINT('Ctrl Pts',(-17.0802404735808,-16.4123522628063,
8.6953333333333));
#33330=CARTESIAN_POINT('Ctrl Pts',(-16.2901202367904,-16.8685283942094,
8.65366666666663));
#33331=CARTESIAN_POINT('Ctrl Pts',(-15.4999999999999,-17.3247045256125,
8.61199999999996));
#33332=CARTESIAN_POINT('Ctrl Pts',(-14.7098797632095,-16.8685283942094,
8.57033333333329));
#33333=CARTESIAN_POINT('Ctrl Pts',(-13.9197595264191,-16.4123522628063,
8.52866666666663));
#33334=CARTESIAN_POINT('Ctrl Pts',(-13.9197595264191,-15.5,8.48699999999996));
#33335=CARTESIAN_POINT('Ctrl Pts',(-13.9197595264191,-14.5876477371938,
8.44533333333329));
#33336=CARTESIAN_POINT('Ctrl Pts',(-14.7098797632095,-14.1314716057907,
8.40366666666663));
#33337=CARTESIAN_POINT('Ctrl Pts',(-15.5,-13.6752954743876,8.36199999999996));
#33338=CARTESIAN_POINT('Ctrl Pts',(-16.2901202367904,-14.1314716057907,
8.32033333333329));
#33339=CARTESIAN_POINT('Ctrl Pts',(-17.0802404735808,-14.5876477371938,
8.27866666666663));
#33340=CARTESIAN_POINT('Ctrl Pts',(-17.0802404735808,-15.5000000000001,
8.23699999999996));
#33341=CARTESIAN_POINT('Ctrl Pts',(-17.0802404735808,-16.4123522628063,
8.19533333333329));
#33342=CARTESIAN_POINT('Ctrl Pts',(-16.2901202367904,-16.8685283942094,
8.15366666666663));
#33343=CARTESIAN_POINT('Ctrl Pts',(-15.4999999999999,-17.3247045256125,
8.11199999999996));
#33344=CARTESIAN_POINT('Ctrl Pts',(-14.7098797632095,-16.8685283942094,
8.07033333333329));
#33345=CARTESIAN_POINT('Ctrl Pts',(-13.9197595264191,-16.4123522628063,
8.02866666666662));
#33346=CARTESIAN_POINT('Ctrl Pts',(-13.9197595264191,-15.5,7.98699999999996));
#33347=CARTESIAN_POINT('Ctrl Pts',(-13.9197595264191,-14.5876477371938,
7.94533333333329));
#33348=CARTESIAN_POINT('Ctrl Pts',(-14.7098797632095,-14.1314716057907,
7.90366666666662));
#33349=CARTESIAN_POINT('Ctrl Pts',(-15.5,-13.6752954743876,7.86199999999995));
#33350=CARTESIAN_POINT('Ctrl Pts',(-16.2901202367904,-14.1314716057907,
7.82033333333329));
#33351=CARTESIAN_POINT('Ctrl Pts',(-17.0802404735808,-14.5876477371938,
7.77866666666662));
#33352=CARTESIAN_POINT('Ctrl Pts',(-17.0802404735808,-15.5000000000001,
7.73699999999995));
#33353=CARTESIAN_POINT('Ctrl Pts',(-17.0802404735808,-16.4123522628063,
7.69533333333329));
#33354=CARTESIAN_POINT('Ctrl Pts',(-16.2901202367904,-16.8685283942094,
7.65366666666662));
#33355=CARTESIAN_POINT('Ctrl Pts',(-15.4999999999999,-17.3247045256125,
7.61199999999995));
#33356=CARTESIAN_POINT('Ctrl Pts',(-14.7098797632095,-16.8685283942094,
7.57033333333328));
#33357=CARTESIAN_POINT('Ctrl Pts',(-13.9197595264191,-16.4123522628063,
7.52866666666662));
#33358=CARTESIAN_POINT('Ctrl Pts',(-13.9197595264191,-15.5,7.48699999999995));
#33359=CARTESIAN_POINT('Ctrl Pts',(-13.9197595264191,-14.5876477371938,
7.44533333333328));
#33360=CARTESIAN_POINT('Ctrl Pts',(-14.7098797632095,-14.1314716057907,
7.40366666666661));
#33361=CARTESIAN_POINT('Ctrl Pts',(-15.5,-13.6752954743876,7.36199999999995));
#33362=CARTESIAN_POINT('Ctrl Pts',(-16.2901202367904,-14.1314716057907,
7.32033333333328));
#33363=CARTESIAN_POINT('Ctrl Pts',(-17.0802404735808,-14.5876477371938,
7.27866666666661));
#33364=CARTESIAN_POINT('Ctrl Pts',(-17.0802404735808,-15.5000000000001,
7.23699999999995));
#33365=CARTESIAN_POINT('Ctrl Pts',(-17.0802404735808,-16.4123522628063,
7.19533333333328));
#33366=CARTESIAN_POINT('Ctrl Pts',(-16.2901202367904,-16.8685283942094,
7.15366666666661));
#33367=CARTESIAN_POINT('Ctrl Pts',(-15.4999999999999,-17.3247045256125,
7.11199999999994));
#33368=CARTESIAN_POINT('Ctrl Pts',(-14.7098797632095,-16.8685283942094,
7.07033333333328));
#33369=CARTESIAN_POINT('Ctrl Pts',(-13.9197595264191,-16.4123522628063,
7.02866666666661));
#33370=CARTESIAN_POINT('Ctrl Pts',(-13.9197595264191,-15.5,6.98699999999994));
#33371=CARTESIAN_POINT('Ctrl Pts',(-13.9197595264191,-14.5876477371938,
6.94533333333327));
#33372=CARTESIAN_POINT('Ctrl Pts',(-14.7098797632095,-14.1314716057907,
6.90366666666661));
#33373=CARTESIAN_POINT('Ctrl Pts',(-15.5,-13.6752954743876,6.86199999999994));
#33374=CARTESIAN_POINT('Ctrl Pts',(-16.2901202367904,-14.1314716057907,
6.82033333333327));
#33375=CARTESIAN_POINT('Ctrl Pts',(-17.0802404735808,-14.5876477371938,
6.77866666666661));
#33376=CARTESIAN_POINT('Ctrl Pts',(-17.0802404735808,-15.5000000000001,
6.73699999999994));
#33377=CARTESIAN_POINT('Ctrl Pts',(-17.0802404735808,-16.4123522628063,
6.69533333333327));
#33378=CARTESIAN_POINT('Ctrl Pts',(-16.2901202367904,-16.8685283942094,
6.65366666666661));
#33379=CARTESIAN_POINT('Ctrl Pts',(-15.4999999999999,-17.3247045256125,
6.61199999999994));
#33380=CARTESIAN_POINT('Ctrl Pts',(-14.7098797632095,-16.8685283942094,
6.57033333333327));
#33381=CARTESIAN_POINT('Ctrl Pts',(-13.9197595264191,-16.4123522628063,
6.5286666666666));
#33382=CARTESIAN_POINT('Ctrl Pts',(-13.9197595264191,-15.5,6.48699999999994));
#33383=CARTESIAN_POINT('Ctrl Pts',(-13.9197595264191,-14.5876477371938,
6.44533333333327));
#33384=CARTESIAN_POINT('Ctrl Pts',(-14.7098797632095,-14.1314716057907,
6.4036666666666));
#33385=CARTESIAN_POINT('Ctrl Pts',(-15.5,-13.6752954743876,6.36199999999993));
#33386=CARTESIAN_POINT('Ctrl Pts',(-16.2901202367904,-14.1314716057907,
6.32033333333327));
#33387=CARTESIAN_POINT('Ctrl Pts',(-17.0802404735808,-14.5876477371938,
6.2786666666666));
#33388=CARTESIAN_POINT('Ctrl Pts',(-17.0802404735808,-15.5000000000001,
6.23699999999993));
#33389=CARTESIAN_POINT('Ctrl Pts',(-17.0802404735808,-16.4123522628063,
6.19533333333326));
#33390=CARTESIAN_POINT('Ctrl Pts',(-16.2901202367904,-16.8685283942094,
6.1536666666666));
#33391=CARTESIAN_POINT('Ctrl Pts',(-15.4999999999999,-17.3247045256125,
6.11199999999993));
#33392=CARTESIAN_POINT('Ctrl Pts',(-14.7098797632095,-16.8685283942094,
6.07033333333326));
#33393=CARTESIAN_POINT('Ctrl Pts',(-13.9197595264191,-16.4123522628063,
6.0286666666666));
#33394=CARTESIAN_POINT('Ctrl Pts',(-13.9197595264191,-15.5,5.98699999999993));
#33395=CARTESIAN_POINT('Ctrl Pts',(-13.9197595264191,-14.5876477371938,
5.94533333333326));
#33396=CARTESIAN_POINT('Ctrl Pts',(-14.7098797632095,-14.1314716057907,
5.9036666666666));
#33397=CARTESIAN_POINT('Ctrl Pts',(-15.5,-13.6752954743876,5.86199999999993));
#33398=CARTESIAN_POINT('Ctrl Pts',(-16.2901202367904,-14.1314716057907,
5.82033333333326));
#33399=CARTESIAN_POINT('Ctrl Pts',(-17.0802404735808,-14.5876477371938,
5.77866666666659));
#33400=CARTESIAN_POINT('Ctrl Pts',(-17.0802404735808,-15.5000000000001,
5.73699999999993));
#33401=CARTESIAN_POINT('Ctrl Pts',(-17.0802404735808,-16.4123522628063,
5.69533333333326));
#33402=CARTESIAN_POINT('Ctrl Pts',(-16.2901202367904,-16.8685283942094,
5.65366666666659));
#33403=CARTESIAN_POINT('Ctrl Pts',(-15.4999999999999,-17.3247045256125,
5.61199999999992));
#33404=CARTESIAN_POINT('Ctrl Pts',(-14.7098797632095,-16.8685283942094,
5.57033333333326));
#33405=CARTESIAN_POINT('Ctrl Pts',(-13.9197595264191,-16.4123522628063,
5.52866666666659));
#33406=CARTESIAN_POINT('Ctrl Pts',(-13.9197595264191,-15.5,5.48699999999992));
#33407=CARTESIAN_POINT('Ctrl Pts',(-13.9197595264191,-14.5876477371938,
5.44533333333326));
#33408=CARTESIAN_POINT('Ctrl Pts',(-14.7098797632095,-14.1314716057907,
5.40366666666659));
#33409=CARTESIAN_POINT('Ctrl Pts',(-15.5,-13.6752954743876,5.36199999999992));
#33410=CARTESIAN_POINT('Ctrl Pts',(-16.2901202367904,-14.1314716057907,
5.32033333333325));
#33411=CARTESIAN_POINT('Ctrl Pts',(-17.0802404735808,-14.5876477371938,
5.27866666666659));
#33412=CARTESIAN_POINT('Ctrl Pts',(-17.0802404735808,-15.5000000000001,
5.23699999999992));
#33413=CARTESIAN_POINT('Ctrl Pts',(-17.0802404735808,-16.4123522628063,
5.19533333333325));
#33414=CARTESIAN_POINT('Ctrl Pts',(-16.2901202367904,-16.8685283942094,
5.15366666666658));
#33415=CARTESIAN_POINT('Ctrl Pts',(-15.4999999999999,-17.3247045256125,
5.11199999999992));
#33416=CARTESIAN_POINT('Ctrl Pts',(-14.7098797632095,-16.8685283942094,
5.07033333333325));
#33417=CARTESIAN_POINT('Ctrl Pts',(-13.9197595264191,-16.4123522628063,
5.02866666666658));
#33418=CARTESIAN_POINT('Ctrl Pts',(-13.9197595264191,-15.5,4.98699999999992));
#33419=CARTESIAN_POINT('Ctrl Pts',(-13.9197595264191,-14.5876477371938,
4.94533333333325));
#33420=CARTESIAN_POINT('Ctrl Pts',(-14.7098797632095,-14.1314716057907,
4.90366666666658));
#33421=CARTESIAN_POINT('Ctrl Pts',(-15.5,-13.6752954743876,4.86199999999991));
#33422=CARTESIAN_POINT('Ctrl Pts',(-16.2901202367904,-14.1314716057907,
4.82033333333325));
#33423=CARTESIAN_POINT('Ctrl Pts',(-17.0802404735808,-14.5876477371938,
4.77866666666658));
#33424=CARTESIAN_POINT('Ctrl Pts',(-17.0802404735808,-15.5000000000001,
4.73699999999991));
#33425=CARTESIAN_POINT('Ctrl Pts',(-17.0802404735808,-16.4123522628063,
4.69533333333325));
#33426=CARTESIAN_POINT('Ctrl Pts',(-16.2901202367904,-16.8685283942094,
4.65366666666658));
#33427=CARTESIAN_POINT('Ctrl Pts',(-15.4999999999999,-17.3247045256125,
4.61199999999991));
#33428=CARTESIAN_POINT('Ctrl Pts',(-14.7098797632095,-16.8685283942094,
4.57033333333324));
#33429=CARTESIAN_POINT('Ctrl Pts',(-13.9197595264191,-16.4123522628063,
4.52866666666658));
#33430=CARTESIAN_POINT('Ctrl Pts',(-13.9197595264191,-15.5,4.48699999999991));
#33431=CARTESIAN_POINT('Ctrl Pts',(-13.9197595264191,-14.5876477371938,
4.44533333333324));
#33432=CARTESIAN_POINT('Ctrl Pts',(-14.7098797632095,-14.1314716057907,
4.40366666666658));
#33433=CARTESIAN_POINT('Ctrl Pts',(-15.5,-13.6752954743876,4.36199999999991));
#33434=CARTESIAN_POINT('Ctrl Pts',(-16.2901202367904,-14.1314716057907,
4.32033333333324));
#33435=CARTESIAN_POINT('Ctrl Pts',(-17.0802404735808,-14.5876477371938,
4.27866666666657));
#33436=CARTESIAN_POINT('Ctrl Pts',(-17.0802404735808,-15.5000000000001,
4.23699999999991));
#33437=CARTESIAN_POINT('Ctrl Pts',(-17.0802404735808,-16.4123522628063,
4.19533333333324));
#33438=CARTESIAN_POINT('Ctrl Pts',(-16.2901202367904,-16.8685283942094,
4.15366666666657));
#33439=CARTESIAN_POINT('Ctrl Pts',(-15.4999999999999,-17.3247045256125,
4.1119999999999));
#33440=CARTESIAN_POINT('Ctrl Pts',(-14.7098797632095,-16.8685283942094,
4.07033333333324));
#33441=CARTESIAN_POINT('Ctrl Pts',(-13.9197595264191,-16.4123522628063,
4.02866666666657));
#33442=CARTESIAN_POINT('Ctrl Pts',(-13.9197595264191,-15.5,3.9869999999999));
#33443=CARTESIAN_POINT('Ctrl Pts',(-13.9197595264191,-14.5876477371938,
3.94533333333323));
#33444=CARTESIAN_POINT('Ctrl Pts',(-14.7098797632095,-14.1314716057907,
3.90366666666657));
#33445=CARTESIAN_POINT('Ctrl Pts',(-15.5,-13.6752954743876,3.8619999999999));
#33446=CARTESIAN_POINT('Ctrl Pts',(-16.2901202367904,-14.1314716057907,
3.82033333333323));
#33447=CARTESIAN_POINT('Ctrl Pts',(-17.0802404735808,-14.5876477371938,
3.77866666666657));
#33448=CARTESIAN_POINT('Ctrl Pts',(-17.0802404735808,-15.5000000000001,
3.7369999999999));
#33449=CARTESIAN_POINT('Ctrl Pts',(-17.0802404735808,-16.4123522628063,
3.69533333333323));
#33450=CARTESIAN_POINT('Ctrl Pts',(-16.2901202367904,-16.8685283942094,
3.65366666666656));
#33451=CARTESIAN_POINT('Ctrl Pts',(-15.4999999999999,-17.3247045256125,
3.6119999999999));
#33452=CARTESIAN_POINT('Ctrl Pts',(-14.7098797632095,-16.8685283942094,
3.57033333333323));
#33453=CARTESIAN_POINT('Ctrl Pts',(-13.9197595264191,-16.4123522628063,
3.52866666666656));
#33454=CARTESIAN_POINT('Ctrl Pts',(-13.9197595264191,-15.5,3.4869999999999));
#33455=CARTESIAN_POINT('Ctrl Pts',(-13.9197595264191,-14.5876477371938,
3.44533333333323));
#33456=CARTESIAN_POINT('Ctrl Pts',(-14.7098797632095,-14.1314716057907,
3.40366666666656));
#33457=CARTESIAN_POINT('Ctrl Pts',(-15.5,-13.6752954743876,3.36199999999989));
#33458=CARTESIAN_POINT('Ctrl Pts',(-16.2901202367904,-14.1314716057907,
3.32033333333323));
#33459=CARTESIAN_POINT('Ctrl Pts',(-17.0802404735808,-14.5876477371938,
3.27866666666656));
#33460=CARTESIAN_POINT('Ctrl Pts',(-17.0802404735808,-15.5000000000001,
3.23699999999989));
#33461=CARTESIAN_POINT('Ctrl Pts',(-17.0802404735808,-16.4123522628063,
3.19533333333323));
#33462=CARTESIAN_POINT('Ctrl Pts',(-16.2901202367904,-16.8685283942094,
3.15366666666656));
#33463=CARTESIAN_POINT('Ctrl Pts',(-15.4999999999999,-17.3247045256125,
3.11199999999989));
#33464=CARTESIAN_POINT('Ctrl Pts',(-14.7098797632095,-16.8685283942094,
3.07033333333322));
#33465=CARTESIAN_POINT('Ctrl Pts',(-13.9197595264191,-16.4123522628063,
3.02866666666656));
#33466=CARTESIAN_POINT('Ctrl Pts',(-13.9197595264191,-15.5,2.98699999999989));
#33467=CARTESIAN_POINT('Ctrl Pts',(-13.9197595264191,-14.5876477371938,
2.94533333333322));
#33468=CARTESIAN_POINT('Ctrl Pts',(-14.7098797632095,-14.1314716057907,
2.90366666666656));
#33469=CARTESIAN_POINT('Ctrl Pts',(-15.5,-13.6752954743876,2.86199999999989));
#33470=CARTESIAN_POINT('Ctrl Pts',(-16.2901202367904,-14.1314716057907,
2.82033333333322));
#33471=CARTESIAN_POINT('Ctrl Pts',(-17.0802404735808,-14.5876477371938,
2.77866666666655));
#33472=CARTESIAN_POINT('Ctrl Pts',(-17.0802404735808,-15.5000000000001,
2.73699999999989));
#33473=CARTESIAN_POINT('Ctrl Pts',(-17.0802404735808,-16.4123522628063,
2.69533333333322));
#33474=CARTESIAN_POINT('Ctrl Pts',(-16.2901202367904,-16.8685283942094,
2.65366666666655));
#33475=CARTESIAN_POINT('Ctrl Pts',(-15.4999999999999,-17.3247045256125,
2.61199999999988));
#33476=CARTESIAN_POINT('Ctrl Pts',(-14.7098797632095,-16.8685283942094,
2.57033333333322));
#33477=CARTESIAN_POINT('Ctrl Pts',(-13.9197595264191,-16.4123522628063,
2.52866666666655));
#33478=CARTESIAN_POINT('Ctrl Pts',(-13.9197595264191,-15.5,2.48699999999988));
#33479=CARTESIAN_POINT('Ctrl Pts',(-13.9197595264191,-14.5876477371938,
2.44533333333321));
#33480=CARTESIAN_POINT('Ctrl Pts',(-14.7098797632095,-14.1314716057907,
2.40366666666655));
#33481=CARTESIAN_POINT('Ctrl Pts',(-15.5,-13.6752954743876,2.36199999999988));
#33482=CARTESIAN_POINT('Ctrl Pts',(-16.2901202367904,-14.1314716057907,
2.32033333333321));
#33483=CARTESIAN_POINT('Ctrl Pts',(-17.0802404735808,-14.5876477371938,
2.27866666666655));
#33484=CARTESIAN_POINT('Ctrl Pts',(-17.0802404735808,-15.5000000000001,
2.23699999999988));
#33485=CARTESIAN_POINT('Ctrl Pts',(-17.0802404735808,-16.4123522628063,
2.19533333333321));
#33486=CARTESIAN_POINT('Ctrl Pts',(-16.2901202367904,-16.8685283942094,
2.15366666666655));
#33487=CARTESIAN_POINT('Ctrl Pts',(-15.4999999999999,-17.3247045256125,
2.11199999999988));
#33488=CARTESIAN_POINT('Ctrl Pts',(-14.7098797632095,-16.8685283942094,
2.07033333333321));
#33489=CARTESIAN_POINT('Ctrl Pts',(-13.9197595264191,-16.4123522628063,
2.02866666666654));
#33490=CARTESIAN_POINT('Ctrl Pts',(-13.9197595264191,-15.5,1.98699999999988));
#33491=CARTESIAN_POINT('Ctrl Pts',(-13.9197595264191,-14.5876477371938,
1.94533333333321));
#33492=CARTESIAN_POINT('Ctrl Pts',(-14.7098797632095,-14.1314716057907,
1.90366666666654));
#33493=CARTESIAN_POINT('Ctrl Pts',(-15.5,-13.6752954743876,1.86199999999987));
#33494=CARTESIAN_POINT('Ctrl Pts',(-16.2901202367904,-14.1314716057907,
1.82033333333321));
#33495=CARTESIAN_POINT('Ctrl Pts',(-17.0802404735808,-14.5876477371938,
1.77866666666654));
#33496=CARTESIAN_POINT('Ctrl Pts',(-17.0802404735808,-15.5000000000001,
1.73699999999987));
#33497=CARTESIAN_POINT('Ctrl Pts',(-17.0802404735808,-16.4123522628063,
1.6953333333332));
#33498=CARTESIAN_POINT('Ctrl Pts',(-16.2901202367904,-16.8685283942094,
1.65366666666654));
#33499=CARTESIAN_POINT('Ctrl Pts',(-15.4999999999999,-17.3247045256125,
1.61199999999987));
#33500=CARTESIAN_POINT('Ctrl Pts',(-14.7098797632095,-16.8685283942094,
1.5703333333332));
#33501=CARTESIAN_POINT('Ctrl Pts',(-13.9197595264191,-16.4123522628063,
1.52866666666654));
#33502=CARTESIAN_POINT('Ctrl Pts',(-13.9197595264191,-15.5,1.48699999999987));
#33503=CARTESIAN_POINT('Ctrl Pts',(-13.9197595264191,-14.5876477371938,
1.4453333333332));
#33504=CARTESIAN_POINT('Ctrl Pts',(-14.7098797632095,-14.1314716057907,
1.40366666666653));
#33505=CARTESIAN_POINT('Ctrl Pts',(-15.5,-13.6752954743876,1.36199999999987));
#33506=CARTESIAN_POINT('Ctrl Pts',(-16.2901202367904,-14.1314716057907,
1.3203333333332));
#33507=CARTESIAN_POINT('Ctrl Pts',(-17.0802404735808,-14.5876477371938,
1.27866666666653));
#33508=CARTESIAN_POINT('Ctrl Pts',(-17.0802404735808,-15.5000000000001,
1.23699999999987));
#33509=CARTESIAN_POINT('Ctrl Pts',(-17.0802404735808,-16.4123522628063,
1.1953333333332));
#33510=CARTESIAN_POINT('Ctrl Pts',(-16.2901202367904,-16.8685283942094,
1.15366666666653));
#33511=CARTESIAN_POINT('Ctrl Pts',(-15.4999999999999,-17.3247045256125,
1.11199999999986));
#33512=CARTESIAN_POINT('Ctrl Pts',(-14.7098797632095,-16.8685283942094,
1.0703333333332));
#33513=CARTESIAN_POINT('Ctrl Pts',(-13.9197595264191,-16.4123522628063,
1.02866666666653));
#33514=CARTESIAN_POINT('Ctrl Pts',(-13.9197595264191,-15.5,0.986999999999863));
#33515=CARTESIAN_POINT('Ctrl Pts',(-13.9197595264191,-14.5876477371938,
0.945333333333196));
#33516=CARTESIAN_POINT('Ctrl Pts',(-14.7098797632095,-14.1314716057907,
0.903666666666529));
#33517=CARTESIAN_POINT('Ctrl Pts',(-15.5,-13.6752954743876,0.861999999999861));
#33518=CARTESIAN_POINT('Ctrl Pts',(-16.2901202367904,-14.1314716057907,
0.820333333333194));
#33519=CARTESIAN_POINT('Ctrl Pts',(-17.0802404735808,-14.5876477371938,
0.778666666666527));
#33520=CARTESIAN_POINT('Ctrl Pts',(-17.0802404735808,-15.5000000000001,
0.736999999999859));
#33521=CARTESIAN_POINT('Ctrl Pts',(-17.0802404735808,-16.4123522628063,
0.695333333333192));
#33522=CARTESIAN_POINT('Ctrl Pts',(-16.2901202367904,-16.8685283942094,
0.653666666666525));
#33523=CARTESIAN_POINT('Ctrl Pts',(-15.4999999999999,-17.3247045256125,
0.611999999999858));
#33524=CARTESIAN_POINT('Ctrl Pts',(-14.7098797632095,-16.8685283942094,
0.57033333333319));
#33525=CARTESIAN_POINT('Ctrl Pts',(-13.9197595264191,-16.4123522628063,
0.528666666666523));
#33526=CARTESIAN_POINT('Ctrl Pts',(-13.9197595264191,-15.5,0.486999999999856));
#33527=CARTESIAN_POINT('Ctrl Pts',(-13.9197595264191,-14.5876477371938,
0.445333333333188));
#33528=CARTESIAN_POINT('Ctrl Pts',(-14.7098797632095,-14.1314716057907,
0.403666666666521));
#33529=CARTESIAN_POINT('Ctrl Pts',(-15.5,-13.6752954743876,0.361999999999854));
#33530=CARTESIAN_POINT('Ctrl Pts',(-16.2901202367904,-14.1314716057907,
0.320333333333186));
#33531=CARTESIAN_POINT('Ctrl Pts',(-17.0802404735808,-14.5876477371938,
0.278666666666519));
#33532=CARTESIAN_POINT('Ctrl Pts',(-17.0802404735808,-15.5000000000001,
0.236999999999852));
#33533=CARTESIAN_POINT('Ctrl Pts',(-17.0802404735808,-16.4123522628063,
0.195333333333185));
#33534=CARTESIAN_POINT('Ctrl Pts',(-16.2901202367904,-16.8685283942094,
0.153666666666517));
#33535=CARTESIAN_POINT('Ctrl Pts',(-15.4999999999999,-17.3247045256125,
0.11199999999985));
#33536=CARTESIAN_POINT('Ctrl Pts',(-14.7098797632095,-16.8685283942094,
0.0703333333331828));
#33537=CARTESIAN_POINT('Ctrl Pts',(-13.9197595264191,-16.4123522628063,
0.0286666666665155));
#33538=CARTESIAN_POINT('Ctrl Pts',(-13.9197595264191,-15.5,-0.0130000000001518));
#33539=CARTESIAN_POINT('Ctrl Pts',(-13.9197595264191,-14.5876477371938,
-0.0546666666668173));
#33540=CARTESIAN_POINT('Ctrl Pts',(-14.7098797632095,-14.1314716057907,
-0.0963333333334846));
#33541=CARTESIAN_POINT('Ctrl Pts',(-15.5,-13.6752954743876,-0.138000000000152));
#33542=CARTESIAN_POINT('Ctrl Pts',(-16.2901202367904,-14.1314716057907,
-0.179666666666819));
#33543=CARTESIAN_POINT('Ctrl Pts',(-17.0802404735808,-14.5876477371938,
-0.221333333333486));
#33544=CARTESIAN_POINT('Ctrl Pts',(-17.0802404735808,-15.5000000000001,
-0.263000000000154));
#33545=CARTESIAN_POINT('Ctrl Pts',(-17.0802404735808,-16.4123522628063,
-0.304666666666821));
#33546=CARTESIAN_POINT('Ctrl Pts',(-16.2901202367904,-16.8685283942094,
-0.346333333333488));
#33547=CARTESIAN_POINT('Ctrl Pts',(-15.4999999999999,-17.3247045256125,
-0.388000000000156));
#33548=CARTESIAN_POINT('Ctrl Pts',(-14.7098797632095,-16.8685283942094,
-0.429666666666823));
#33549=CARTESIAN_POINT('Ctrl Pts',(-13.9197595264191,-16.4123522628063,
-0.47133333333349));
#33550=CARTESIAN_POINT('Ctrl Pts',(-13.9197595264191,-15.5,-0.513000000000157));
#33551=CARTESIAN_POINT('Ctrl Pts',(-13.9197595264191,-14.5876477371938,
-0.554666666666825));
#33552=CARTESIAN_POINT('Ctrl Pts',(-14.7098797632095,-14.1314716057907,
-0.596333333333492));
#33553=CARTESIAN_POINT('Ctrl Pts',(-15.5,-13.6752954743876,-0.638000000000159));
#33554=CARTESIAN_POINT('Ctrl Pts',(-16.2901202367904,-14.1314716057907,
-0.679666666666827));
#33555=CARTESIAN_POINT('Ctrl Pts',(-17.0802404735808,-14.5876477371938,
-0.721333333333494));
#33556=CARTESIAN_POINT('Ctrl Pts',(-17.0802404735808,-15.5000000000001,
-0.763000000000161));
#33557=CARTESIAN_POINT('Ctrl Pts',(-17.0802404735808,-16.4123522628063,
-0.804666666666829));
#33558=CARTESIAN_POINT('Ctrl Pts',(-16.2901202367904,-16.8685283942094,
-0.846333333333496));
#33559=CARTESIAN_POINT('Ctrl Pts',(-15.4999999999999,-17.3247045256125,
-0.888000000000163));
#33560=CARTESIAN_POINT('Ctrl Pts',(-14.7098797632095,-16.8685283942094,
-0.92966666666683));
#33561=CARTESIAN_POINT('Ctrl Pts',(-13.9197595264191,-16.4123522628063,
-0.971333333333498));
#33562=CARTESIAN_POINT('Ctrl Pts',(-13.9197595264191,-15.5,-1.01300000000016));
#33563=CARTESIAN_POINT('Ctrl Pts',(-13.9197595264191,-14.5876477371938,
-1.05466666666683));
#33564=CARTESIAN_POINT('Ctrl Pts',(-14.7098797632095,-14.1314716057907,
-1.0963333333335));
#33565=CARTESIAN_POINT('Ctrl Pts',(-15.5,-13.6752954743876,-1.13800000000017));
#33566=CARTESIAN_POINT('Ctrl Pts',(-16.2901202367904,-14.1314716057907,
-1.17966666666683));
#33567=CARTESIAN_POINT('Ctrl Pts',(-17.0802404735808,-14.5876477371938,
-1.2213333333335));
#33568=CARTESIAN_POINT('Ctrl Pts',(-17.0802404735808,-15.5000000000001,
-1.26300000000017));
#33569=CARTESIAN_POINT('Ctrl Pts',(-17.0802404735808,-16.4123522628063,
-1.30466666666683));
#33570=CARTESIAN_POINT('Ctrl Pts',(-16.2901202367904,-16.8685283942094,
-1.3463333333335));
#33571=CARTESIAN_POINT('Ctrl Pts',(-15.4999999999999,-17.3247045256125,
-1.38800000000017));
#33572=CARTESIAN_POINT('Ctrl Pts',(-14.7098797632095,-16.8685283942094,
-1.42966666666684));
#33573=CARTESIAN_POINT('Ctrl Pts',(-13.9197595264191,-16.4123522628063,
-1.4713333333335));
#33574=CARTESIAN_POINT('Ctrl Pts',(-13.9197595264191,-15.5,-1.51300000000017));
#33575=CARTESIAN_POINT('Ctrl Pts',(-13.9197595264191,-14.5876477371938,
-1.55466666666684));
#33576=CARTESIAN_POINT('Ctrl Pts',(-14.7098797632095,-14.1314716057907,
-1.59633333333351));
#33577=CARTESIAN_POINT('Ctrl Pts',(-15.5,-13.6752954743876,-1.63800000000017));
#33578=CARTESIAN_POINT('Ctrl Pts',(-16.2901202367904,-14.1314716057907,
-1.67966666666684));
#33579=CARTESIAN_POINT('Ctrl Pts',(-17.0802404735808,-14.5876477371938,
-1.72133333333351));
#33580=CARTESIAN_POINT('Ctrl Pts',(-17.0802404735808,-15.5000000000001,
-1.76300000000017));
#33581=CARTESIAN_POINT('Ctrl Pts',(-17.0802404735808,-16.4123522628063,
-1.80466666666684));
#33582=CARTESIAN_POINT('Ctrl Pts',(-16.2901202367904,-16.8685283942094,
-1.84633333333351));
#33583=CARTESIAN_POINT('Ctrl Pts',(-15.4999999999999,-17.3247045256125,
-1.88800000000018));
#33584=CARTESIAN_POINT('Ctrl Pts',(-14.7098797632095,-16.8685283942094,
-1.92966666666684));
#33585=CARTESIAN_POINT('Ctrl Pts',(-14.4189900731898,-16.7005831533721,
-1.94500661517905));
#33586=CARTESIAN_POINT('Ctrl Pts',(-14.2215527726061,-16.42883402237,-1.96262314816781));
#33587=CARTESIAN_POINT('Origin',(-14.0080754615185,-16.5839252605847,-2.17746715486548));
#33588=CARTESIAN_POINT('',(-14.2215498957103,-16.4288300625789,-2.02512301642217));
#33589=CARTESIAN_POINT('Ctrl Pts',(-17.0802404735808,-15.5000000000001,
11.2370201234482));
#33590=CARTESIAN_POINT('Ctrl Pts',(-17.0802404735808,-16.4123522628063,
11.1953534567815));
#33591=CARTESIAN_POINT('Ctrl Pts',(-16.2901202367904,-16.8685283942094,
11.1536867901149));
#33592=CARTESIAN_POINT('Ctrl Pts',(-15.4999999999999,-17.3247045256125,
11.1120201234482));
#33593=CARTESIAN_POINT('Ctrl Pts',(-14.7098797632095,-16.8685283942094,
11.0703534567815));
#33594=CARTESIAN_POINT('Ctrl Pts',(-13.9197595264191,-16.4123522628063,
11.0286867901149));
#33595=CARTESIAN_POINT('Ctrl Pts',(-13.9197595264191,-15.5,10.9870201234482));
#33596=CARTESIAN_POINT('Ctrl Pts',(-13.9197595264191,-14.5876477371938,
10.9453534567815));
#33597=CARTESIAN_POINT('Ctrl Pts',(-14.7098797632095,-14.1314716057907,
10.9036867901149));
#33598=CARTESIAN_POINT('Ctrl Pts',(-15.5,-13.6752954743876,10.8620201234482));
#33599=CARTESIAN_POINT('Ctrl Pts',(-16.2901202367904,-14.1314716057907,
10.8203534567815));
#33600=CARTESIAN_POINT('Ctrl Pts',(-17.0802404735808,-14.5876477371938,
10.7786867901149));
#33601=CARTESIAN_POINT('Ctrl Pts',(-17.0802404735808,-15.5000000000001,
10.7370201234482));
#33602=CARTESIAN_POINT('Ctrl Pts',(-17.0802404735808,-16.4123522628063,
10.6953534567815));
#33603=CARTESIAN_POINT('Ctrl Pts',(-16.2901202367904,-16.8685283942094,
10.6536867901149));
#33604=CARTESIAN_POINT('Ctrl Pts',(-15.4999999999999,-17.3247045256125,
10.6120201234482));
#33605=CARTESIAN_POINT('Ctrl Pts',(-14.7098797632095,-16.8685283942094,
10.5703534567815));
#33606=CARTESIAN_POINT('Ctrl Pts',(-13.9197595264191,-16.4123522628063,
10.5286867901149));
#33607=CARTESIAN_POINT('Ctrl Pts',(-13.9197595264191,-15.5,10.4870201234482));
#33608=CARTESIAN_POINT('Ctrl Pts',(-13.9197595264191,-14.5876477371938,
10.4453534567815));
#33609=CARTESIAN_POINT('Ctrl Pts',(-14.7098797632095,-14.1314716057907,
10.4036867901149));
#33610=CARTESIAN_POINT('Ctrl Pts',(-15.5,-13.6752954743876,10.3620201234482));
#33611=CARTESIAN_POINT('Ctrl Pts',(-16.2901202367904,-14.1314716057907,
10.3203534567815));
#33612=CARTESIAN_POINT('Ctrl Pts',(-17.0802404735808,-14.5876477371938,
10.2786867901149));
#33613=CARTESIAN_POINT('Ctrl Pts',(-17.0802404735808,-15.5000000000001,
10.2370201234482));
#33614=CARTESIAN_POINT('Ctrl Pts',(-17.0802404735808,-16.4123522628063,
10.1953534567815));
#33615=CARTESIAN_POINT('Ctrl Pts',(-16.2901202367904,-16.8685283942094,
10.1536867901149));
#33616=CARTESIAN_POINT('Ctrl Pts',(-15.4999999999999,-17.3247045256125,
10.1120201234482));
#33617=CARTESIAN_POINT('Ctrl Pts',(-14.7098797632095,-16.8685283942094,
10.0703534567815));
#33618=CARTESIAN_POINT('Ctrl Pts',(-13.9197595264191,-16.4123522628063,
10.0286867901149));
#33619=CARTESIAN_POINT('Ctrl Pts',(-13.9197595264191,-15.5,9.98702012344819));
#33620=CARTESIAN_POINT('Ctrl Pts',(-13.9197595264191,-14.5876477371938,
9.94535345678152));
#33621=CARTESIAN_POINT('Ctrl Pts',(-14.7098797632095,-14.1314716057907,
9.90368679011485));
#33622=CARTESIAN_POINT('Ctrl Pts',(-15.5,-13.6752954743876,9.86202012344818));
#33623=CARTESIAN_POINT('Ctrl Pts',(-16.2901202367904,-14.1314716057907,
9.82035345678151));
#33624=CARTESIAN_POINT('Ctrl Pts',(-17.0802404735808,-14.5876477371938,
9.77868679011485));
#33625=CARTESIAN_POINT('Ctrl Pts',(-17.0802404735808,-15.5000000000001,
9.73702012344818));
#33626=CARTESIAN_POINT('Ctrl Pts',(-17.0802404735808,-16.4123522628063,
9.69535345678152));
#33627=CARTESIAN_POINT('Ctrl Pts',(-16.2901202367904,-16.8685283942094,
9.65368679011485));
#33628=CARTESIAN_POINT('Ctrl Pts',(-15.4999999999999,-17.3247045256125,
9.61202012344818));
#33629=CARTESIAN_POINT('Ctrl Pts',(-14.7098797632095,-16.8685283942094,
9.57035345678151));
#33630=CARTESIAN_POINT('Ctrl Pts',(-13.9197595264191,-16.4123522628063,
9.52868679011484));
#33631=CARTESIAN_POINT('Ctrl Pts',(-13.9197595264191,-15.5,9.48702012344818));
#33632=CARTESIAN_POINT('Ctrl Pts',(-13.9197595264191,-14.5876477371938,
9.44535345678151));
#33633=CARTESIAN_POINT('Ctrl Pts',(-14.7098797632095,-14.1314716057907,
9.40368679011484));
#33634=CARTESIAN_POINT('Ctrl Pts',(-15.5,-13.6752954743876,9.36202012344818));
#33635=CARTESIAN_POINT('Ctrl Pts',(-16.2901202367904,-14.1314716057907,
9.32035345678151));
#33636=CARTESIAN_POINT('Ctrl Pts',(-17.0802404735808,-14.5876477371938,
9.27868679011484));
#33637=CARTESIAN_POINT('Ctrl Pts',(-17.0802404735808,-15.5000000000001,
9.23702012344818));
#33638=CARTESIAN_POINT('Ctrl Pts',(-17.0802404735808,-16.4123522628063,
9.19535345678151));
#33639=CARTESIAN_POINT('Ctrl Pts',(-16.2901202367904,-16.8685283942094,
9.15368679011484));
#33640=CARTESIAN_POINT('Ctrl Pts',(-15.4999999999999,-17.3247045256125,
9.11202012344818));
#33641=CARTESIAN_POINT('Ctrl Pts',(-14.7098797632095,-16.8685283942094,
9.07035345678151));
#33642=CARTESIAN_POINT('Ctrl Pts',(-13.9197595264191,-16.4123522628063,
9.02868679011484));
#33643=CARTESIAN_POINT('Ctrl Pts',(-13.9197595264191,-15.5,8.98702012344817));
#33644=CARTESIAN_POINT('Ctrl Pts',(-13.9197595264191,-14.5876477371938,
8.9453534567815));
#33645=CARTESIAN_POINT('Ctrl Pts',(-14.7098797632095,-14.1314716057907,
8.90368679011484));
#33646=CARTESIAN_POINT('Ctrl Pts',(-15.5,-13.6752954743876,8.86202012344817));
#33647=CARTESIAN_POINT('Ctrl Pts',(-16.2901202367904,-14.1314716057907,
8.8203534567815));
#33648=CARTESIAN_POINT('Ctrl Pts',(-17.0802404735808,-14.5876477371938,
8.77868679011484));
#33649=CARTESIAN_POINT('Ctrl Pts',(-17.0802404735808,-15.5000000000001,
8.73702012344817));
#33650=CARTESIAN_POINT('Ctrl Pts',(-17.0802404735808,-16.4123522628063,
8.6953534567815));
#33651=CARTESIAN_POINT('Ctrl Pts',(-16.2901202367904,-16.8685283942094,
8.65368679011483));
#33652=CARTESIAN_POINT('Ctrl Pts',(-15.4999999999999,-17.3247045256125,
8.61202012344817));
#33653=CARTESIAN_POINT('Ctrl Pts',(-14.7098797632095,-16.8685283942094,
8.5703534567815));
#33654=CARTESIAN_POINT('Ctrl Pts',(-13.9197595264191,-16.4123522628063,
8.52868679011483));
#33655=CARTESIAN_POINT('Ctrl Pts',(-13.9197595264191,-15.5,8.48702012344816));
#33656=CARTESIAN_POINT('Ctrl Pts',(-13.9197595264191,-14.5876477371938,
8.4453534567815));
#33657=CARTESIAN_POINT('Ctrl Pts',(-14.7098797632095,-14.1314716057907,
8.40368679011483));
#33658=CARTESIAN_POINT('Ctrl Pts',(-15.5,-13.6752954743876,8.36202012344816));
#33659=CARTESIAN_POINT('Ctrl Pts',(-16.2901202367904,-14.1314716057907,
8.3203534567815));
#33660=CARTESIAN_POINT('Ctrl Pts',(-17.0802404735808,-14.5876477371938,
8.27868679011483));
#33661=CARTESIAN_POINT('Ctrl Pts',(-17.0802404735808,-15.5000000000001,
8.23702012344816));
#33662=CARTESIAN_POINT('Ctrl Pts',(-17.0802404735808,-16.4123522628063,
8.19535345678149));
#33663=CARTESIAN_POINT('Ctrl Pts',(-16.2901202367904,-16.8685283942094,
8.15368679011483));
#33664=CARTESIAN_POINT('Ctrl Pts',(-15.4999999999999,-17.3247045256125,
8.11202012344816));
#33665=CARTESIAN_POINT('Ctrl Pts',(-14.7098797632095,-16.8685283942094,
8.07035345678149));
#33666=CARTESIAN_POINT('Ctrl Pts',(-13.9197595264191,-16.4123522628063,
8.02868679011483));
#33667=CARTESIAN_POINT('Ctrl Pts',(-13.9197595264191,-15.5,7.98702012344816));
#33668=CARTESIAN_POINT('Ctrl Pts',(-13.9197595264191,-14.5876477371938,
7.94535345678149));
#33669=CARTESIAN_POINT('Ctrl Pts',(-14.7098797632095,-14.1314716057907,
7.90368679011482));
#33670=CARTESIAN_POINT('Ctrl Pts',(-15.5,-13.6752954743876,7.86202012344816));
#33671=CARTESIAN_POINT('Ctrl Pts',(-16.2901202367904,-14.1314716057907,
7.82035345678149));
#33672=CARTESIAN_POINT('Ctrl Pts',(-17.0802404735808,-14.5876477371938,
7.77868679011482));
#33673=CARTESIAN_POINT('Ctrl Pts',(-17.0802404735808,-15.5000000000001,
7.73702012344816));
#33674=CARTESIAN_POINT('Ctrl Pts',(-17.0802404735808,-16.4123522628063,
7.69535345678149));
#33675=CARTESIAN_POINT('Ctrl Pts',(-16.2901202367904,-16.8685283942094,
7.65368679011482));
#33676=CARTESIAN_POINT('Ctrl Pts',(-15.4999999999999,-17.3247045256125,
7.61202012344815));
#33677=CARTESIAN_POINT('Ctrl Pts',(-14.7098797632095,-16.8685283942094,
7.57035345678149));
#33678=CARTESIAN_POINT('Ctrl Pts',(-13.9197595264191,-16.4123522628063,
7.52868679011482));
#33679=CARTESIAN_POINT('Ctrl Pts',(-13.9197595264191,-15.5,7.48702012344815));
#33680=CARTESIAN_POINT('Ctrl Pts',(-13.9197595264191,-14.5876477371938,
7.44535345678149));
#33681=CARTESIAN_POINT('Ctrl Pts',(-14.7098797632095,-14.1314716057907,
7.40368679011482));
#33682=CARTESIAN_POINT('Ctrl Pts',(-15.5,-13.6752954743876,7.36202012344815));
#33683=CARTESIAN_POINT('Ctrl Pts',(-16.2901202367904,-14.1314716057907,
7.32035345678148));
#33684=CARTESIAN_POINT('Ctrl Pts',(-17.0802404735808,-14.5876477371938,
7.27868679011482));
#33685=CARTESIAN_POINT('Ctrl Pts',(-17.0802404735808,-15.5000000000001,
7.23702012344815));
#33686=CARTESIAN_POINT('Ctrl Pts',(-17.0802404735808,-16.4123522628063,
7.19535345678148));
#33687=CARTESIAN_POINT('Ctrl Pts',(-16.2901202367904,-16.8685283942094,
7.15368679011481));
#33688=CARTESIAN_POINT('Ctrl Pts',(-15.4999999999999,-17.3247045256125,
7.11202012344815));
#33689=CARTESIAN_POINT('Ctrl Pts',(-14.7098797632095,-16.8685283942094,
7.07035345678148));
#33690=CARTESIAN_POINT('Ctrl Pts',(-13.9197595264191,-16.4123522628063,
7.02868679011481));
#33691=CARTESIAN_POINT('Ctrl Pts',(-13.9197595264191,-15.5,6.98702012344815));
#33692=CARTESIAN_POINT('Ctrl Pts',(-13.9197595264191,-14.5876477371938,
6.94535345678148));
#33693=CARTESIAN_POINT('Ctrl Pts',(-14.7098797632095,-14.1314716057907,
6.90368679011481));
#33694=CARTESIAN_POINT('Ctrl Pts',(-15.5,-13.6752954743876,6.86202012344814));
#33695=CARTESIAN_POINT('Ctrl Pts',(-16.2901202367904,-14.1314716057907,
6.82035345678148));
#33696=CARTESIAN_POINT('Ctrl Pts',(-17.0802404735808,-14.5876477371938,
6.77868679011481));
#33697=CARTESIAN_POINT('Ctrl Pts',(-17.0802404735808,-15.5000000000001,
6.73702012344814));
#33698=CARTESIAN_POINT('Ctrl Pts',(-17.0802404735808,-16.4123522628063,
6.69535345678147));
#33699=CARTESIAN_POINT('Ctrl Pts',(-16.2901202367904,-16.8685283942094,
6.65368679011481));
#33700=CARTESIAN_POINT('Ctrl Pts',(-15.4999999999999,-17.3247045256125,
6.61202012344814));
#33701=CARTESIAN_POINT('Ctrl Pts',(-14.7098797632095,-16.8685283942094,
6.57035345678147));
#33702=CARTESIAN_POINT('Ctrl Pts',(-13.9197595264191,-16.4123522628063,
6.52868679011481));
#33703=CARTESIAN_POINT('Ctrl Pts',(-13.9197595264191,-15.5,6.48702012344814));
#33704=CARTESIAN_POINT('Ctrl Pts',(-13.9197595264191,-14.5876477371938,
6.44535345678147));
#33705=CARTESIAN_POINT('Ctrl Pts',(-14.7098797632095,-14.1314716057907,
6.4036867901148));
#33706=CARTESIAN_POINT('Ctrl Pts',(-15.5,-13.6752954743876,6.36202012344814));
#33707=CARTESIAN_POINT('Ctrl Pts',(-16.2901202367904,-14.1314716057907,
6.32035345678147));
#33708=CARTESIAN_POINT('Ctrl Pts',(-17.0802404735808,-14.5876477371938,
6.2786867901148));
#33709=CARTESIAN_POINT('Ctrl Pts',(-17.0802404735808,-15.5000000000001,
6.23702012344813));
#33710=CARTESIAN_POINT('Ctrl Pts',(-17.0802404735808,-16.4123522628063,
6.19535345678147));
#33711=CARTESIAN_POINT('Ctrl Pts',(-16.2901202367904,-16.8685283942094,
6.1536867901148));
#33712=CARTESIAN_POINT('Ctrl Pts',(-15.4999999999999,-17.3247045256125,
6.11202012344813));
#33713=CARTESIAN_POINT('Ctrl Pts',(-14.7098797632095,-16.8685283942094,
6.07035345678146));
#33714=CARTESIAN_POINT('Ctrl Pts',(-13.9197595264191,-16.4123522628063,
6.0286867901148));
#33715=CARTESIAN_POINT('Ctrl Pts',(-13.9197595264191,-15.5,5.98702012344813));
#33716=CARTESIAN_POINT('Ctrl Pts',(-13.9197595264191,-14.5876477371938,
5.94535345678146));
#33717=CARTESIAN_POINT('Ctrl Pts',(-14.7098797632095,-14.1314716057907,
5.9036867901148));
#33718=CARTESIAN_POINT('Ctrl Pts',(-15.5,-13.6752954743876,5.86202012344813));
#33719=CARTESIAN_POINT('Ctrl Pts',(-16.2901202367904,-14.1314716057907,
5.82035345678146));
#33720=CARTESIAN_POINT('Ctrl Pts',(-17.0802404735808,-14.5876477371938,
5.77868679011479));
#33721=CARTESIAN_POINT('Ctrl Pts',(-17.0802404735808,-15.5000000000001,
5.73702012344813));
#33722=CARTESIAN_POINT('Ctrl Pts',(-17.0802404735808,-16.4123522628063,
5.69535345678146));
#33723=CARTESIAN_POINT('Ctrl Pts',(-16.2901202367904,-16.8685283942094,
5.65368679011479));
#33724=CARTESIAN_POINT('Ctrl Pts',(-15.4999999999999,-17.3247045256125,
5.61202012344813));
#33725=CARTESIAN_POINT('Ctrl Pts',(-14.7098797632095,-16.8685283942094,
5.57035345678146));
#33726=CARTESIAN_POINT('Ctrl Pts',(-13.9197595264191,-16.4123522628063,
5.52868679011479));
#33727=CARTESIAN_POINT('Ctrl Pts',(-13.9197595264191,-15.5,5.48702012344813));
#33728=CARTESIAN_POINT('Ctrl Pts',(-13.9197595264191,-14.5876477371938,
5.44535345678146));
#33729=CARTESIAN_POINT('Ctrl Pts',(-14.7098797632095,-14.1314716057907,
5.40368679011479));
#33730=CARTESIAN_POINT('Ctrl Pts',(-15.5,-13.6752954743876,5.36202012344812));
#33731=CARTESIAN_POINT('Ctrl Pts',(-16.2901202367904,-14.1314716057907,
5.32035345678146));
#33732=CARTESIAN_POINT('Ctrl Pts',(-17.0802404735808,-14.5876477371938,
5.27868679011479));
#33733=CARTESIAN_POINT('Ctrl Pts',(-17.0802404735808,-15.5000000000001,
5.23702012344812));
#33734=CARTESIAN_POINT('Ctrl Pts',(-17.0802404735808,-16.4123522628063,
5.19535345678145));
#33735=CARTESIAN_POINT('Ctrl Pts',(-16.2901202367904,-16.8685283942094,
5.15368679011479));
#33736=CARTESIAN_POINT('Ctrl Pts',(-15.4999999999999,-17.3247045256125,
5.11202012344812));
#33737=CARTESIAN_POINT('Ctrl Pts',(-14.7098797632095,-16.8685283942094,
5.07035345678145));
#33738=CARTESIAN_POINT('Ctrl Pts',(-13.9197595264191,-16.4123522628063,
5.02868679011479));
#33739=CARTESIAN_POINT('Ctrl Pts',(-13.9197595264191,-15.5,4.98702012344812));
#33740=CARTESIAN_POINT('Ctrl Pts',(-13.9197595264191,-14.5876477371938,
4.94535345678145));
#33741=CARTESIAN_POINT('Ctrl Pts',(-14.7098797632095,-14.1314716057907,
4.90368679011478));
#33742=CARTESIAN_POINT('Ctrl Pts',(-15.5,-13.6752954743876,4.86202012344812));
#33743=CARTESIAN_POINT('Ctrl Pts',(-16.2901202367904,-14.1314716057907,
4.82035345678145));
#33744=CARTESIAN_POINT('Ctrl Pts',(-17.0802404735808,-14.5876477371938,
4.77868679011478));
#33745=CARTESIAN_POINT('Ctrl Pts',(-17.0802404735808,-15.5000000000001,
4.73702012344812));
#33746=CARTESIAN_POINT('Ctrl Pts',(-17.0802404735808,-16.4123522628063,
4.69535345678145));
#33747=CARTESIAN_POINT('Ctrl Pts',(-16.2901202367904,-16.8685283942094,
4.65368679011478));
#33748=CARTESIAN_POINT('Ctrl Pts',(-15.4999999999999,-17.3247045256125,
4.61202012344811));
#33749=CARTESIAN_POINT('Ctrl Pts',(-14.7098797632095,-16.8685283942094,
4.57035345678145));
#33750=CARTESIAN_POINT('Ctrl Pts',(-13.9197595264191,-16.4123522628063,
4.52868679011478));
#33751=CARTESIAN_POINT('Ctrl Pts',(-13.9197595264191,-15.5,4.48702012344811));
#33752=CARTESIAN_POINT('Ctrl Pts',(-13.9197595264191,-14.5876477371938,
4.44535345678144));
#33753=CARTESIAN_POINT('Ctrl Pts',(-14.7098797632095,-14.1314716057907,
4.40368679011478));
#33754=CARTESIAN_POINT('Ctrl Pts',(-15.5,-13.6752954743876,4.36202012344811));
#33755=CARTESIAN_POINT('Ctrl Pts',(-16.2901202367904,-14.1314716057907,
4.32035345678144));
#33756=CARTESIAN_POINT('Ctrl Pts',(-17.0802404735808,-14.5876477371938,
4.27868679011477));
#33757=CARTESIAN_POINT('Ctrl Pts',(-17.0802404735808,-15.5000000000001,
4.23702012344811));
#33758=CARTESIAN_POINT('Ctrl Pts',(-17.0802404735808,-16.4123522628063,
4.19535345678144));
#33759=CARTESIAN_POINT('Ctrl Pts',(-16.2901202367904,-16.8685283942094,
4.15368679011477));
#33760=CARTESIAN_POINT('Ctrl Pts',(-15.4999999999999,-17.3247045256125,
4.11202012344811));
#33761=CARTESIAN_POINT('Ctrl Pts',(-14.7098797632095,-16.8685283942094,
4.07035345678144));
#33762=CARTESIAN_POINT('Ctrl Pts',(-13.9197595264191,-16.4123522628063,
4.02868679011477));
#33763=CARTESIAN_POINT('Ctrl Pts',(-13.9197595264191,-15.5,3.9870201234481));
#33764=CARTESIAN_POINT('Ctrl Pts',(-13.9197595264191,-14.5876477371938,
3.94535345678144));
#33765=CARTESIAN_POINT('Ctrl Pts',(-14.7098797632095,-14.1314716057907,
3.90368679011477));
#33766=CARTESIAN_POINT('Ctrl Pts',(-15.5,-13.6752954743876,3.8620201234481));
#33767=CARTESIAN_POINT('Ctrl Pts',(-16.2901202367904,-14.1314716057907,
3.82035345678144));
#33768=CARTESIAN_POINT('Ctrl Pts',(-17.0802404735808,-14.5876477371938,
3.77868679011477));
#33769=CARTESIAN_POINT('Ctrl Pts',(-17.0802404735808,-15.5000000000001,
3.7370201234481));
#33770=CARTESIAN_POINT('Ctrl Pts',(-17.0802404735808,-16.4123522628063,
3.69535345678143));
#33771=CARTESIAN_POINT('Ctrl Pts',(-16.2901202367904,-16.8685283942094,
3.65368679011477));
#33772=CARTESIAN_POINT('Ctrl Pts',(-15.4999999999999,-17.3247045256125,
3.6120201234481));
#33773=CARTESIAN_POINT('Ctrl Pts',(-14.7098797632095,-16.8685283942094,
3.57035345678143));
#33774=CARTESIAN_POINT('Ctrl Pts',(-13.9197595264191,-16.4123522628063,
3.52868679011477));
#33775=CARTESIAN_POINT('Ctrl Pts',(-13.9197595264191,-15.5,3.4870201234481));
#33776=CARTESIAN_POINT('Ctrl Pts',(-13.9197595264191,-14.5876477371938,
3.44535345678143));
#33777=CARTESIAN_POINT('Ctrl Pts',(-14.7098797632095,-14.1314716057907,
3.40368679011476));
#33778=CARTESIAN_POINT('Ctrl Pts',(-15.5,-13.6752954743876,3.3620201234481));
#33779=CARTESIAN_POINT('Ctrl Pts',(-16.2901202367904,-14.1314716057907,
3.32035345678143));
#33780=CARTESIAN_POINT('Ctrl Pts',(-17.0802404735808,-14.5876477371938,
3.27868679011476));
#33781=CARTESIAN_POINT('Ctrl Pts',(-17.0802404735808,-15.5000000000001,
3.2370201234481));
#33782=CARTESIAN_POINT('Ctrl Pts',(-17.0802404735808,-16.4123522628063,
3.19535345678143));
#33783=CARTESIAN_POINT('Ctrl Pts',(-16.2901202367904,-16.8685283942094,
3.15368679011476));
#33784=CARTESIAN_POINT('Ctrl Pts',(-15.4999999999999,-17.3247045256125,
3.11202012344809));
#33785=CARTESIAN_POINT('Ctrl Pts',(-14.7098797632095,-16.8685283942094,
3.07035345678143));
#33786=CARTESIAN_POINT('Ctrl Pts',(-13.9197595264191,-16.4123522628063,
3.02868679011476));
#33787=CARTESIAN_POINT('Ctrl Pts',(-13.9197595264191,-15.5,2.98702012344809));
#33788=CARTESIAN_POINT('Ctrl Pts',(-13.9197595264191,-14.5876477371938,
2.94535345678143));
#33789=CARTESIAN_POINT('Ctrl Pts',(-14.7098797632095,-14.1314716057907,
2.90368679011476));
#33790=CARTESIAN_POINT('Ctrl Pts',(-15.5,-13.6752954743876,2.86202012344809));
#33791=CARTESIAN_POINT('Ctrl Pts',(-16.2901202367904,-14.1314716057907,
2.82035345678142));
#33792=CARTESIAN_POINT('Ctrl Pts',(-17.0802404735808,-14.5876477371938,
2.77868679011475));
#33793=CARTESIAN_POINT('Ctrl Pts',(-17.0802404735808,-15.5000000000001,
2.73702012344809));
#33794=CARTESIAN_POINT('Ctrl Pts',(-17.0802404735808,-16.4123522628063,
2.69535345678142));
#33795=CARTESIAN_POINT('Ctrl Pts',(-16.2901202367904,-16.8685283942094,
2.65368679011475));
#33796=CARTESIAN_POINT('Ctrl Pts',(-15.4999999999999,-17.3247045256125,
2.61202012344809));
#33797=CARTESIAN_POINT('Ctrl Pts',(-14.7098797632095,-16.8685283942094,
2.57035345678142));
#33798=CARTESIAN_POINT('Ctrl Pts',(-13.9197595264191,-16.4123522628063,
2.52868679011475));
#33799=CARTESIAN_POINT('Ctrl Pts',(-13.9197595264191,-15.5,2.48702012344808));
#33800=CARTESIAN_POINT('Ctrl Pts',(-13.9197595264191,-14.5876477371938,
2.44535345678142));
#33801=CARTESIAN_POINT('Ctrl Pts',(-14.7098797632095,-14.1314716057907,
2.40368679011475));
#33802=CARTESIAN_POINT('Ctrl Pts',(-15.5,-13.6752954743876,2.36202012344808));
#33803=CARTESIAN_POINT('Ctrl Pts',(-16.2901202367904,-14.1314716057907,
2.32035345678142));
#33804=CARTESIAN_POINT('Ctrl Pts',(-17.0802404735808,-14.5876477371938,
2.27868679011475));
#33805=CARTESIAN_POINT('Ctrl Pts',(-17.0802404735808,-15.5000000000001,
2.23702012344808));
#33806=CARTESIAN_POINT('Ctrl Pts',(-17.0802404735808,-16.4123522628063,
2.19535345678142));
#33807=CARTESIAN_POINT('Ctrl Pts',(-16.2901202367904,-16.8685283942094,
2.15368679011475));
#33808=CARTESIAN_POINT('Ctrl Pts',(-15.4999999999999,-17.3247045256125,
2.11202012344808));
#33809=CARTESIAN_POINT('Ctrl Pts',(-14.7098797632095,-16.8685283942094,
2.07035345678141));
#33810=CARTESIAN_POINT('Ctrl Pts',(-13.9197595264191,-16.4123522628063,
2.02868679011475));
#33811=CARTESIAN_POINT('Ctrl Pts',(-13.9197595264191,-15.5,1.98702012344808));
#33812=CARTESIAN_POINT('Ctrl Pts',(-13.9197595264191,-14.5876477371938,
1.94535345678141));
#33813=CARTESIAN_POINT('Ctrl Pts',(-14.7098797632095,-14.1314716057907,
1.90368679011474));
#33814=CARTESIAN_POINT('Ctrl Pts',(-15.5,-13.6752954743876,1.86202012344808));
#33815=CARTESIAN_POINT('Ctrl Pts',(-16.2901202367904,-14.1314716057907,
1.82035345678141));
#33816=CARTESIAN_POINT('Ctrl Pts',(-17.0802404735808,-14.5876477371938,
1.77868679011474));
#33817=CARTESIAN_POINT('Ctrl Pts',(-17.0802404735808,-15.5000000000001,
1.73702012344808));
#33818=CARTESIAN_POINT('Ctrl Pts',(-17.0802404735808,-16.4123522628063,
1.69535345678141));
#33819=CARTESIAN_POINT('Ctrl Pts',(-16.2901202367904,-16.8685283942094,
1.65368679011474));
#33820=CARTESIAN_POINT('Ctrl Pts',(-15.4999999999999,-17.3247045256125,
1.61202012344807));
#33821=CARTESIAN_POINT('Ctrl Pts',(-14.7098797632095,-16.8685283942094,
1.57035345678141));
#33822=CARTESIAN_POINT('Ctrl Pts',(-13.9197595264191,-16.4123522628063,
1.52868679011474));
#33823=CARTESIAN_POINT('Ctrl Pts',(-13.9197595264191,-15.5,1.48702012344807));
#33824=CARTESIAN_POINT('Ctrl Pts',(-13.9197595264191,-14.5876477371938,
1.4453534567814));
#33825=CARTESIAN_POINT('Ctrl Pts',(-14.7098797632095,-14.1314716057907,
1.40368679011474));
#33826=CARTESIAN_POINT('Ctrl Pts',(-15.5,-13.6752954743876,1.36202012344807));
#33827=CARTESIAN_POINT('Ctrl Pts',(-16.2901202367904,-14.1314716057907,
1.3203534567814));
#33828=CARTESIAN_POINT('Ctrl Pts',(-17.0802404735808,-14.5876477371938,
1.27868679011473));
#33829=CARTESIAN_POINT('Ctrl Pts',(-17.0802404735808,-15.5000000000001,
1.23702012344807));
#33830=CARTESIAN_POINT('Ctrl Pts',(-17.0802404735808,-16.4123522628063,
1.1953534567814));
#33831=CARTESIAN_POINT('Ctrl Pts',(-16.2901202367904,-16.8685283942094,
1.15368679011473));
#33832=CARTESIAN_POINT('Ctrl Pts',(-15.4999999999999,-17.3247045256125,
1.11202012344807));
#33833=CARTESIAN_POINT('Ctrl Pts',(-14.7098797632095,-16.8685283942094,
1.0703534567814));
#33834=CARTESIAN_POINT('Ctrl Pts',(-13.9197595264191,-16.4123522628063,
1.02868679011473));
#33835=CARTESIAN_POINT('Ctrl Pts',(-13.9197595264191,-15.5,0.987020123448066));
#33836=CARTESIAN_POINT('Ctrl Pts',(-13.9197595264191,-14.5876477371938,
0.945353456781398));
#33837=CARTESIAN_POINT('Ctrl Pts',(-14.7098797632095,-14.1314716057907,
0.903686790114731));
#33838=CARTESIAN_POINT('Ctrl Pts',(-15.5,-13.6752954743876,0.862020123448064));
#33839=CARTESIAN_POINT('Ctrl Pts',(-16.2901202367904,-14.1314716057907,
0.820353456781396));
#33840=CARTESIAN_POINT('Ctrl Pts',(-17.0802404735808,-14.5876477371938,
0.778686790114729));
#33841=CARTESIAN_POINT('Ctrl Pts',(-17.0802404735808,-15.5000000000001,
0.737020123448062));
#33842=CARTESIAN_POINT('Ctrl Pts',(-17.0802404735808,-16.4123522628063,
0.695353456781395));
#33843=CARTESIAN_POINT('Ctrl Pts',(-16.2901202367904,-16.8685283942094,
0.653686790114727));
#33844=CARTESIAN_POINT('Ctrl Pts',(-15.4999999999999,-17.3247045256125,
0.61202012344806));
#33845=CARTESIAN_POINT('Ctrl Pts',(-14.7098797632095,-16.8685283942094,
0.570353456781393));
#33846=CARTESIAN_POINT('Ctrl Pts',(-13.9197595264191,-16.4123522628063,
0.528686790114725));
#33847=CARTESIAN_POINT('Ctrl Pts',(-13.9197595264191,-15.5,0.487020123448058));
#33848=CARTESIAN_POINT('Ctrl Pts',(-13.9197595264191,-14.5876477371938,
0.445353456781391));
#33849=CARTESIAN_POINT('Ctrl Pts',(-14.7098797632095,-14.1314716057907,
0.403686790114724));
#33850=CARTESIAN_POINT('Ctrl Pts',(-15.5,-13.6752954743876,0.362020123448056));
#33851=CARTESIAN_POINT('Ctrl Pts',(-16.2901202367904,-14.1314716057907,
0.320353456781389));
#33852=CARTESIAN_POINT('Ctrl Pts',(-17.0802404735808,-14.5876477371938,
0.278686790114722));
#33853=CARTESIAN_POINT('Ctrl Pts',(-17.0802404735808,-15.5000000000001,
0.237020123448054));
#33854=CARTESIAN_POINT('Ctrl Pts',(-17.0802404735808,-16.4123522628063,
0.195353456781387));
#33855=CARTESIAN_POINT('Ctrl Pts',(-16.2901202367904,-16.8685283942094,
0.15368679011472));
#33856=CARTESIAN_POINT('Ctrl Pts',(-15.4999999999999,-17.3247045256125,
0.112020123448053));
#33857=CARTESIAN_POINT('Ctrl Pts',(-14.7098797632095,-16.8685283942094,
0.0703534567813853));
#33858=CARTESIAN_POINT('Ctrl Pts',(-13.9197595264191,-16.4123522628063,
0.028686790114718));
#33859=CARTESIAN_POINT('Ctrl Pts',(-13.9197595264191,-15.5,-0.0129798765519493));
#33860=CARTESIAN_POINT('Ctrl Pts',(-13.9197595264191,-14.5876477371938,
-0.0546465432186148));
#33861=CARTESIAN_POINT('Ctrl Pts',(-14.7098797632095,-14.1314716057907,
-0.0963132098852821));
#33862=CARTESIAN_POINT('Ctrl Pts',(-15.5,-13.6752954743876,-0.137979876551949));
#33863=CARTESIAN_POINT('Ctrl Pts',(-16.2901202367904,-14.1314716057907,
-0.179646543218617));
#33864=CARTESIAN_POINT('Ctrl Pts',(-17.0802404735808,-14.5876477371938,
-0.221313209885284));
#33865=CARTESIAN_POINT('Ctrl Pts',(-17.0802404735808,-15.5000000000001,
-0.262979876551951));
#33866=CARTESIAN_POINT('Ctrl Pts',(-17.0802404735808,-16.4123522628063,
-0.304646543218619));
#33867=CARTESIAN_POINT('Ctrl Pts',(-16.2901202367904,-16.8685283942094,
-0.346313209885286));
#33868=CARTESIAN_POINT('Ctrl Pts',(-15.4999999999999,-17.3247045256125,
-0.387979876551953));
#33869=CARTESIAN_POINT('Ctrl Pts',(-14.7098797632095,-16.8685283942094,
-0.42964654321862));
#33870=CARTESIAN_POINT('Ctrl Pts',(-13.9197595264191,-16.4123522628063,
-0.471313209885288));
#33871=CARTESIAN_POINT('Ctrl Pts',(-13.9197595264191,-15.5,-0.512979876551955));
#33872=CARTESIAN_POINT('Ctrl Pts',(-13.9197595264191,-14.5876477371938,
-0.554646543218622));
#33873=CARTESIAN_POINT('Ctrl Pts',(-14.7098797632095,-14.1314716057907,
-0.596313209885289));
#33874=CARTESIAN_POINT('Ctrl Pts',(-15.5,-13.6752954743876,-0.637979876551957));
#33875=CARTESIAN_POINT('Ctrl Pts',(-16.2901202367904,-14.1314716057907,
-0.679646543218624));
#33876=CARTESIAN_POINT('Ctrl Pts',(-17.0802404735808,-14.5876477371938,
-0.721313209885291));
#33877=CARTESIAN_POINT('Ctrl Pts',(-17.0802404735808,-15.5000000000001,
-0.762979876551959));
#33878=CARTESIAN_POINT('Ctrl Pts',(-17.0802404735808,-16.4123522628063,
-0.804646543218626));
#33879=CARTESIAN_POINT('Ctrl Pts',(-16.2901202367904,-16.8685283942094,
-0.846313209885293));
#33880=CARTESIAN_POINT('Ctrl Pts',(-15.4999999999999,-17.3247045256125,
-0.88797987655196));
#33881=CARTESIAN_POINT('Ctrl Pts',(-14.7098797632095,-16.8685283942094,
-0.929646543218628));
#33882=CARTESIAN_POINT('Ctrl Pts',(-13.9197595264191,-16.4123522628063,
-0.971313209885295));
#33883=CARTESIAN_POINT('Ctrl Pts',(-13.9197595264191,-15.5,-1.01297987655196));
#33884=CARTESIAN_POINT('Ctrl Pts',(-13.9197595264191,-14.5876477371938,
-1.05464654321863));
#33885=CARTESIAN_POINT('Ctrl Pts',(-14.7098797632095,-14.1314716057907,
-1.0963132098853));
#33886=CARTESIAN_POINT('Ctrl Pts',(-15.5,-13.6752954743876,-1.13797987655196));
#33887=CARTESIAN_POINT('Ctrl Pts',(-16.2901202367904,-14.1314716057907,
-1.17964654321863));
#33888=CARTESIAN_POINT('Ctrl Pts',(-17.0802404735808,-14.5876477371938,
-1.2213132098853));
#33889=CARTESIAN_POINT('Ctrl Pts',(-17.0802404735808,-15.5000000000001,
-1.26297987655196));
#33890=CARTESIAN_POINT('Ctrl Pts',(-17.0802404735808,-16.4123522628063,
-1.30464654321863));
#33891=CARTESIAN_POINT('Ctrl Pts',(-16.2901202367904,-16.8685283942094,
-1.3463132098853));
#33892=CARTESIAN_POINT('Ctrl Pts',(-15.4999999999999,-17.3247045256125,
-1.38797987655197));
#33893=CARTESIAN_POINT('Ctrl Pts',(-14.7098797632095,-16.8685283942094,
-1.42964654321863));
#33894=CARTESIAN_POINT('Ctrl Pts',(-13.9197595264191,-16.4123522628063,
-1.4713132098853));
#33895=CARTESIAN_POINT('Ctrl Pts',(-13.9197595264191,-15.5,-1.51297987655197));
#33896=CARTESIAN_POINT('Ctrl Pts',(-13.9197595264191,-14.5876477371938,
-1.55464654321864));
#33897=CARTESIAN_POINT('Ctrl Pts',(-14.7098797632095,-14.1314716057907,
-1.5963132098853));
#33898=CARTESIAN_POINT('Ctrl Pts',(-15.5,-13.6752954743876,-1.63797987655197));
#33899=CARTESIAN_POINT('Ctrl Pts',(-16.2901202367904,-14.1314716057907,
-1.67964654321864));
#33900=CARTESIAN_POINT('Ctrl Pts',(-17.0802404735808,-14.5876477371938,
-1.7213132098853));
#33901=CARTESIAN_POINT('Ctrl Pts',(-17.0802404735808,-15.5000000000001,
-1.76297987655197));
#33902=CARTESIAN_POINT('Ctrl Pts',(-17.0802404735808,-16.4123522628063,
-1.80464654321864));
#33903=CARTESIAN_POINT('Ctrl Pts',(-16.2901202367904,-16.8685283942094,
-1.84631320988531));
#33904=CARTESIAN_POINT('Ctrl Pts',(-15.4999999999999,-17.3247045256125,
-1.88797987655197));
#33905=CARTESIAN_POINT('Ctrl Pts',(-14.7098797632095,-16.8685283942094,
-1.92964654321864));
#33906=CARTESIAN_POINT('Ctrl Pts',(-14.4189900731898,-16.7005831533721,
-1.94498649173085));
#33907=CARTESIAN_POINT('Ctrl Pts',(-14.2215586016756,-16.4288420454488,
-1.96260250461286));
#33908=CARTESIAN_POINT('Ctrl Pts',(-13.4352476007234,-15.3465777998746,
-2.03276185973389));
#33909=CARTESIAN_POINT('Ctrl Pts',(-12.6489365997712,-14.2643135543004,
-2.10292121485492));
#33910=CARTESIAN_POINT('Ctrl Pts',(-17.0802404735808,-15.5000000000001,
11.1745));
#33911=CARTESIAN_POINT('Ctrl Pts',(-17.0802404735808,-16.4123522628063,
11.1328333333333));
#33912=CARTESIAN_POINT('Ctrl Pts',(-16.2901202367904,-16.8685283942094,
11.0911666666667));
#33913=CARTESIAN_POINT('Ctrl Pts',(-15.4999999999999,-17.3247045256125,
11.0495));
#33914=CARTESIAN_POINT('Ctrl Pts',(-14.7098797632095,-16.8685283942094,
11.0078333333333));
#33915=CARTESIAN_POINT('Ctrl Pts',(-13.9197595264191,-16.4123522628063,
10.9661666666667));
#33916=CARTESIAN_POINT('Ctrl Pts',(-13.9197595264191,-15.5,10.9245));
#33917=CARTESIAN_POINT('Ctrl Pts',(-13.9197595264191,-14.5876477371938,
10.8828333333333));
#33918=CARTESIAN_POINT('Ctrl Pts',(-14.7098797632095,-14.1314716057907,
10.8411666666667));
#33919=CARTESIAN_POINT('Ctrl Pts',(-15.5,-13.6752954743876,10.7995));
#33920=CARTESIAN_POINT('Ctrl Pts',(-16.2901202367904,-14.1314716057907,
10.7578333333333));
#33921=CARTESIAN_POINT('Ctrl Pts',(-17.0802404735808,-14.5876477371938,
10.7161666666667));
#33922=CARTESIAN_POINT('Ctrl Pts',(-17.0802404735808,-15.5000000000001,
10.6745));
#33923=CARTESIAN_POINT('Ctrl Pts',(-17.0802404735808,-16.4123522628063,
10.6328333333333));
#33924=CARTESIAN_POINT('Ctrl Pts',(-16.2901202367904,-16.8685283942094,
10.5911666666667));
#33925=CARTESIAN_POINT('Ctrl Pts',(-15.4999999999999,-17.3247045256125,
10.5495));
#33926=CARTESIAN_POINT('Ctrl Pts',(-14.7098797632095,-16.8685283942094,
10.5078333333333));
#33927=CARTESIAN_POINT('Ctrl Pts',(-13.9197595264191,-16.4123522628063,
10.4661666666667));
#33928=CARTESIAN_POINT('Ctrl Pts',(-13.9197595264191,-15.5,10.4245));
#33929=CARTESIAN_POINT('Ctrl Pts',(-13.9197595264191,-14.5876477371938,
10.3828333333333));
#33930=CARTESIAN_POINT('Ctrl Pts',(-14.7098797632095,-14.1314716057907,
10.3411666666667));
#33931=CARTESIAN_POINT('Ctrl Pts',(-15.5,-13.6752954743876,10.2995));
#33932=CARTESIAN_POINT('Ctrl Pts',(-16.2901202367904,-14.1314716057907,
10.2578333333333));
#33933=CARTESIAN_POINT('Ctrl Pts',(-17.0802404735808,-14.5876477371938,
10.2161666666667));
#33934=CARTESIAN_POINT('Ctrl Pts',(-17.0802404735808,-15.5000000000001,
10.1745));
#33935=CARTESIAN_POINT('Ctrl Pts',(-17.0802404735808,-16.4123522628063,
10.1328333333333));
#33936=CARTESIAN_POINT('Ctrl Pts',(-16.2901202367904,-16.8685283942094,
10.0911666666667));
#33937=CARTESIAN_POINT('Ctrl Pts',(-15.4999999999999,-17.3247045256125,
10.0495));
#33938=CARTESIAN_POINT('Ctrl Pts',(-14.7098797632095,-16.8685283942094,
10.0078333333333));
#33939=CARTESIAN_POINT('Ctrl Pts',(-13.9197595264191,-16.4123522628063,
9.96616666666665));
#33940=CARTESIAN_POINT('Ctrl Pts',(-13.9197595264191,-15.5,9.92449999999998));
#33941=CARTESIAN_POINT('Ctrl Pts',(-13.9197595264191,-14.5876477371938,
9.88283333333331));
#33942=CARTESIAN_POINT('Ctrl Pts',(-14.7098797632095,-14.1314716057907,
9.84116666666665));
#33943=CARTESIAN_POINT('Ctrl Pts',(-15.5,-13.6752954743876,9.79949999999998));
#33944=CARTESIAN_POINT('Ctrl Pts',(-16.2901202367904,-14.1314716057907,
9.75783333333331));
#33945=CARTESIAN_POINT('Ctrl Pts',(-17.0802404735808,-14.5876477371938,
9.71616666666665));
#33946=CARTESIAN_POINT('Ctrl Pts',(-17.0802404735808,-15.5000000000001,
9.67449999999998));
#33947=CARTESIAN_POINT('Ctrl Pts',(-17.0802404735808,-16.4123522628063,
9.63283333333331));
#33948=CARTESIAN_POINT('Ctrl Pts',(-16.2901202367904,-16.8685283942094,
9.59116666666664));
#33949=CARTESIAN_POINT('Ctrl Pts',(-15.4999999999999,-17.3247045256125,
9.54949999999998));
#33950=CARTESIAN_POINT('Ctrl Pts',(-14.7098797632095,-16.8685283942094,
9.50783333333331));
#33951=CARTESIAN_POINT('Ctrl Pts',(-13.9197595264191,-16.4123522628063,
9.46616666666664));
#33952=CARTESIAN_POINT('Ctrl Pts',(-13.9197595264191,-15.5,9.42449999999998));
#33953=CARTESIAN_POINT('Ctrl Pts',(-13.9197595264191,-14.5876477371938,
9.38283333333331));
#33954=CARTESIAN_POINT('Ctrl Pts',(-14.7098797632095,-14.1314716057907,
9.34116666666664));
#33955=CARTESIAN_POINT('Ctrl Pts',(-15.5,-13.6752954743876,9.29949999999998));
#33956=CARTESIAN_POINT('Ctrl Pts',(-16.2901202367904,-14.1314716057907,
9.25783333333331));
#33957=CARTESIAN_POINT('Ctrl Pts',(-17.0802404735808,-14.5876477371938,
9.21616666666664));
#33958=CARTESIAN_POINT('Ctrl Pts',(-17.0802404735808,-15.5000000000001,
9.17449999999997));
#33959=CARTESIAN_POINT('Ctrl Pts',(-17.0802404735808,-16.4123522628063,
9.13283333333331));
#33960=CARTESIAN_POINT('Ctrl Pts',(-16.2901202367904,-16.8685283942094,
9.09116666666664));
#33961=CARTESIAN_POINT('Ctrl Pts',(-15.4999999999999,-17.3247045256125,
9.04949999999997));
#33962=CARTESIAN_POINT('Ctrl Pts',(-14.7098797632095,-16.8685283942094,
9.0078333333333));
#33963=CARTESIAN_POINT('Ctrl Pts',(-13.9197595264191,-16.4123522628063,
8.96616666666664));
#33964=CARTESIAN_POINT('Ctrl Pts',(-13.9197595264191,-15.5,8.92449999999997));
#33965=CARTESIAN_POINT('Ctrl Pts',(-13.9197595264191,-14.5876477371938,
8.8828333333333));
#33966=CARTESIAN_POINT('Ctrl Pts',(-14.7098797632095,-14.1314716057907,
8.84116666666664));
#33967=CARTESIAN_POINT('Ctrl Pts',(-15.5,-13.6752954743876,8.79949999999997));
#33968=CARTESIAN_POINT('Ctrl Pts',(-16.2901202367904,-14.1314716057907,
8.7578333333333));
#33969=CARTESIAN_POINT('Ctrl Pts',(-17.0802404735808,-14.5876477371938,
8.71616666666663));
#33970=CARTESIAN_POINT('Ctrl Pts',(-17.0802404735808,-15.5000000000001,
8.67449999999997));
#33971=CARTESIAN_POINT('Ctrl Pts',(-17.0802404735808,-16.4123522628063,
8.6328333333333));
#33972=CARTESIAN_POINT('Ctrl Pts',(-16.2901202367904,-16.8685283942094,
8.59116666666663));
#33973=CARTESIAN_POINT('Ctrl Pts',(-15.4999999999999,-17.3247045256125,
8.54949999999996));
#33974=CARTESIAN_POINT('Ctrl Pts',(-14.7098797632095,-16.8685283942094,
8.50783333333329));
#33975=CARTESIAN_POINT('Ctrl Pts',(-13.9197595264191,-16.4123522628063,
8.46616666666663));
#33976=CARTESIAN_POINT('Ctrl Pts',(-13.9197595264191,-15.5,8.42449999999996));
#33977=CARTESIAN_POINT('Ctrl Pts',(-13.9197595264191,-14.5876477371938,
8.3828333333333));
#33978=CARTESIAN_POINT('Ctrl Pts',(-14.7098797632095,-14.1314716057907,
8.34116666666663));
#33979=CARTESIAN_POINT('Ctrl Pts',(-15.5,-13.6752954743876,8.29949999999996));
#33980=CARTESIAN_POINT('Ctrl Pts',(-16.2901202367904,-14.1314716057907,
8.25783333333329));
#33981=CARTESIAN_POINT('Ctrl Pts',(-17.0802404735808,-14.5876477371938,
8.21616666666663));
#33982=CARTESIAN_POINT('Ctrl Pts',(-17.0802404735808,-15.5000000000001,
8.17449999999996));
#33983=CARTESIAN_POINT('Ctrl Pts',(-17.0802404735808,-16.4123522628063,
8.13283333333329));
#33984=CARTESIAN_POINT('Ctrl Pts',(-16.2901202367904,-16.8685283942094,
8.09116666666663));
#33985=CARTESIAN_POINT('Ctrl Pts',(-15.4999999999999,-17.3247045256125,
8.04949999999996));
#33986=CARTESIAN_POINT('Ctrl Pts',(-14.7098797632095,-16.8685283942094,
8.00783333333329));
#33987=CARTESIAN_POINT('Ctrl Pts',(-13.9197595264191,-16.4123522628063,
7.96616666666662));
#33988=CARTESIAN_POINT('Ctrl Pts',(-13.9197595264191,-15.5,7.92449999999996));
#33989=CARTESIAN_POINT('Ctrl Pts',(-13.9197595264191,-14.5876477371938,
7.88283333333329));
#33990=CARTESIAN_POINT('Ctrl Pts',(-14.7098797632095,-14.1314716057907,
7.84116666666662));
#33991=CARTESIAN_POINT('Ctrl Pts',(-15.5,-13.6752954743876,7.79949999999995));
#33992=CARTESIAN_POINT('Ctrl Pts',(-16.2901202367904,-14.1314716057907,
7.75783333333329));
#33993=CARTESIAN_POINT('Ctrl Pts',(-17.0802404735808,-14.5876477371938,
7.71616666666662));
#33994=CARTESIAN_POINT('Ctrl Pts',(-17.0802404735808,-15.5000000000001,
7.67449999999995));
#33995=CARTESIAN_POINT('Ctrl Pts',(-17.0802404735808,-16.4123522628063,
7.63283333333328));
#33996=CARTESIAN_POINT('Ctrl Pts',(-16.2901202367904,-16.8685283942094,
7.59116666666662));
#33997=CARTESIAN_POINT('Ctrl Pts',(-15.4999999999999,-17.3247045256125,
7.54949999999995));
#33998=CARTESIAN_POINT('Ctrl Pts',(-14.7098797632095,-16.8685283942094,
7.50783333333328));
#33999=CARTESIAN_POINT('Ctrl Pts',(-13.9197595264191,-16.4123522628063,
7.46616666666662));
#34000=CARTESIAN_POINT('Ctrl Pts',(-13.9197595264191,-15.5,7.42449999999995));
#34001=CARTESIAN_POINT('Ctrl Pts',(-13.9197595264191,-14.5876477371938,
7.38283333333328));
#34002=CARTESIAN_POINT('Ctrl Pts',(-14.7098797632095,-14.1314716057907,
7.34116666666661));
#34003=CARTESIAN_POINT('Ctrl Pts',(-15.5,-13.6752954743876,7.29949999999995));
#34004=CARTESIAN_POINT('Ctrl Pts',(-16.2901202367904,-14.1314716057907,
7.25783333333328));
#34005=CARTESIAN_POINT('Ctrl Pts',(-17.0802404735808,-14.5876477371938,
7.21616666666661));
#34006=CARTESIAN_POINT('Ctrl Pts',(-17.0802404735808,-15.5000000000001,
7.17449999999995));
#34007=CARTESIAN_POINT('Ctrl Pts',(-17.0802404735808,-16.4123522628063,
7.13283333333328));
#34008=CARTESIAN_POINT('Ctrl Pts',(-16.2901202367904,-16.8685283942094,
7.09116666666661));
#34009=CARTESIAN_POINT('Ctrl Pts',(-15.4999999999999,-17.3247045256125,
7.04949999999994));
#34010=CARTESIAN_POINT('Ctrl Pts',(-14.7098797632095,-16.8685283942094,
7.00783333333328));
#34011=CARTESIAN_POINT('Ctrl Pts',(-13.9197595264191,-16.4123522628063,
6.96616666666661));
#34012=CARTESIAN_POINT('Ctrl Pts',(-13.9197595264191,-15.5,6.92449999999994));
#34013=CARTESIAN_POINT('Ctrl Pts',(-13.9197595264191,-14.5876477371938,
6.88283333333327));
#34014=CARTESIAN_POINT('Ctrl Pts',(-14.7098797632095,-14.1314716057907,
6.84116666666661));
#34015=CARTESIAN_POINT('Ctrl Pts',(-15.5,-13.6752954743876,6.79949999999994));
#34016=CARTESIAN_POINT('Ctrl Pts',(-16.2901202367904,-14.1314716057907,
6.75783333333327));
#34017=CARTESIAN_POINT('Ctrl Pts',(-17.0802404735808,-14.5876477371938,
6.71616666666661));
#34018=CARTESIAN_POINT('Ctrl Pts',(-17.0802404735808,-15.5000000000001,
6.67449999999994));
#34019=CARTESIAN_POINT('Ctrl Pts',(-17.0802404735808,-16.4123522628063,
6.63283333333327));
#34020=CARTESIAN_POINT('Ctrl Pts',(-16.2901202367904,-16.8685283942094,
6.59116666666661));
#34021=CARTESIAN_POINT('Ctrl Pts',(-15.4999999999999,-17.3247045256125,
6.54949999999994));
#34022=CARTESIAN_POINT('Ctrl Pts',(-14.7098797632095,-16.8685283942094,
6.50783333333327));
#34023=CARTESIAN_POINT('Ctrl Pts',(-13.9197595264191,-16.4123522628063,
6.4661666666666));
#34024=CARTESIAN_POINT('Ctrl Pts',(-13.9197595264191,-15.5,6.42449999999994));
#34025=CARTESIAN_POINT('Ctrl Pts',(-13.9197595264191,-14.5876477371938,
6.38283333333327));
#34026=CARTESIAN_POINT('Ctrl Pts',(-14.7098797632095,-14.1314716057907,
6.3411666666666));
#34027=CARTESIAN_POINT('Ctrl Pts',(-15.5,-13.6752954743876,6.29949999999993));
#34028=CARTESIAN_POINT('Ctrl Pts',(-16.2901202367904,-14.1314716057907,
6.25783333333327));
#34029=CARTESIAN_POINT('Ctrl Pts',(-17.0802404735808,-14.5876477371938,
6.2161666666666));
#34030=CARTESIAN_POINT('Ctrl Pts',(-17.0802404735808,-15.5000000000001,
6.17449999999993));
#34031=CARTESIAN_POINT('Ctrl Pts',(-17.0802404735808,-16.4123522628063,
6.13283333333326));
#34032=CARTESIAN_POINT('Ctrl Pts',(-16.2901202367904,-16.8685283942094,
6.0911666666666));
#34033=CARTESIAN_POINT('Ctrl Pts',(-15.4999999999999,-17.3247045256125,
6.04949999999993));
#34034=CARTESIAN_POINT('Ctrl Pts',(-14.7098797632095,-16.8685283942094,
6.00783333333326));
#34035=CARTESIAN_POINT('Ctrl Pts',(-13.9197595264191,-16.4123522628063,
5.9661666666666));
#34036=CARTESIAN_POINT('Ctrl Pts',(-13.9197595264191,-15.5,5.92449999999993));
#34037=CARTESIAN_POINT('Ctrl Pts',(-13.9197595264191,-14.5876477371938,
5.88283333333326));
#34038=CARTESIAN_POINT('Ctrl Pts',(-14.7098797632095,-14.1314716057907,
5.8411666666666));
#34039=CARTESIAN_POINT('Ctrl Pts',(-15.5,-13.6752954743876,5.79949999999993));
#34040=CARTESIAN_POINT('Ctrl Pts',(-16.2901202367904,-14.1314716057907,
5.75783333333326));
#34041=CARTESIAN_POINT('Ctrl Pts',(-17.0802404735808,-14.5876477371938,
5.71616666666659));
#34042=CARTESIAN_POINT('Ctrl Pts',(-17.0802404735808,-15.5000000000001,
5.67449999999993));
#34043=CARTESIAN_POINT('Ctrl Pts',(-17.0802404735808,-16.4123522628063,
5.63283333333326));
#34044=CARTESIAN_POINT('Ctrl Pts',(-16.2901202367904,-16.8685283942094,
5.59116666666659));
#34045=CARTESIAN_POINT('Ctrl Pts',(-15.4999999999999,-17.3247045256125,
5.54949999999992));
#34046=CARTESIAN_POINT('Ctrl Pts',(-14.7098797632095,-16.8685283942094,
5.50783333333326));
#34047=CARTESIAN_POINT('Ctrl Pts',(-13.9197595264191,-16.4123522628063,
5.46616666666659));
#34048=CARTESIAN_POINT('Ctrl Pts',(-13.9197595264191,-15.5,5.42449999999992));
#34049=CARTESIAN_POINT('Ctrl Pts',(-13.9197595264191,-14.5876477371938,
5.38283333333326));
#34050=CARTESIAN_POINT('Ctrl Pts',(-14.7098797632095,-14.1314716057907,
5.34116666666659));
#34051=CARTESIAN_POINT('Ctrl Pts',(-15.5,-13.6752954743876,5.29949999999992));
#34052=CARTESIAN_POINT('Ctrl Pts',(-16.2901202367904,-14.1314716057907,
5.25783333333325));
#34053=CARTESIAN_POINT('Ctrl Pts',(-17.0802404735808,-14.5876477371938,
5.21616666666659));
#34054=CARTESIAN_POINT('Ctrl Pts',(-17.0802404735808,-15.5000000000001,
5.17449999999992));
#34055=CARTESIAN_POINT('Ctrl Pts',(-17.0802404735808,-16.4123522628063,
5.13283333333325));
#34056=CARTESIAN_POINT('Ctrl Pts',(-16.2901202367904,-16.8685283942094,
5.09116666666658));
#34057=CARTESIAN_POINT('Ctrl Pts',(-15.4999999999999,-17.3247045256125,
5.04949999999992));
#34058=CARTESIAN_POINT('Ctrl Pts',(-14.7098797632095,-16.8685283942094,
5.00783333333325));
#34059=CARTESIAN_POINT('Ctrl Pts',(-13.9197595264191,-16.4123522628063,
4.96616666666658));
#34060=CARTESIAN_POINT('Ctrl Pts',(-13.9197595264191,-15.5,4.92449999999992));
#34061=CARTESIAN_POINT('Ctrl Pts',(-13.9197595264191,-14.5876477371938,
4.88283333333325));
#34062=CARTESIAN_POINT('Ctrl Pts',(-14.7098797632095,-14.1314716057907,
4.84116666666658));
#34063=CARTESIAN_POINT('Ctrl Pts',(-15.5,-13.6752954743876,4.79949999999991));
#34064=CARTESIAN_POINT('Ctrl Pts',(-16.2901202367904,-14.1314716057907,
4.75783333333325));
#34065=CARTESIAN_POINT('Ctrl Pts',(-17.0802404735808,-14.5876477371938,
4.71616666666658));
#34066=CARTESIAN_POINT('Ctrl Pts',(-17.0802404735808,-15.5000000000001,
4.67449999999991));
#34067=CARTESIAN_POINT('Ctrl Pts',(-17.0802404735808,-16.4123522628063,
4.63283333333324));
#34068=CARTESIAN_POINT('Ctrl Pts',(-16.2901202367904,-16.8685283942094,
4.59116666666658));
#34069=CARTESIAN_POINT('Ctrl Pts',(-15.4999999999999,-17.3247045256125,
4.54949999999991));
#34070=CARTESIAN_POINT('Ctrl Pts',(-14.7098797632095,-16.8685283942094,
4.50783333333324));
#34071=CARTESIAN_POINT('Ctrl Pts',(-13.9197595264191,-16.4123522628063,
4.46616666666658));
#34072=CARTESIAN_POINT('Ctrl Pts',(-13.9197595264191,-15.5,4.42449999999991));
#34073=CARTESIAN_POINT('Ctrl Pts',(-13.9197595264191,-14.5876477371938,
4.38283333333324));
#34074=CARTESIAN_POINT('Ctrl Pts',(-14.7098797632095,-14.1314716057907,
4.34116666666657));
#34075=CARTESIAN_POINT('Ctrl Pts',(-15.5,-13.6752954743876,4.29949999999991));
#34076=CARTESIAN_POINT('Ctrl Pts',(-16.2901202367904,-14.1314716057907,
4.25783333333324));
#34077=CARTESIAN_POINT('Ctrl Pts',(-17.0802404735808,-14.5876477371938,
4.21616666666657));
#34078=CARTESIAN_POINT('Ctrl Pts',(-17.0802404735808,-15.5000000000001,
4.17449999999991));
#34079=CARTESIAN_POINT('Ctrl Pts',(-17.0802404735808,-16.4123522628063,
4.13283333333324));
#34080=CARTESIAN_POINT('Ctrl Pts',(-16.2901202367904,-16.8685283942094,
4.09116666666657));
#34081=CARTESIAN_POINT('Ctrl Pts',(-15.4999999999999,-17.3247045256125,
4.0494999999999));
#34082=CARTESIAN_POINT('Ctrl Pts',(-14.7098797632095,-16.8685283942094,
4.00783333333324));
#34083=CARTESIAN_POINT('Ctrl Pts',(-13.9197595264191,-16.4123522628063,
3.96616666666657));
#34084=CARTESIAN_POINT('Ctrl Pts',(-13.9197595264191,-15.5,3.9244999999999));
#34085=CARTESIAN_POINT('Ctrl Pts',(-13.9197595264191,-14.5876477371938,
3.88283333333323));
#34086=CARTESIAN_POINT('Ctrl Pts',(-14.7098797632095,-14.1314716057907,
3.84116666666657));
#34087=CARTESIAN_POINT('Ctrl Pts',(-15.5,-13.6752954743876,3.7994999999999));
#34088=CARTESIAN_POINT('Ctrl Pts',(-16.2901202367904,-14.1314716057907,
3.75783333333323));
#34089=CARTESIAN_POINT('Ctrl Pts',(-17.0802404735808,-14.5876477371938,
3.71616666666657));
#34090=CARTESIAN_POINT('Ctrl Pts',(-17.0802404735808,-15.5000000000001,
3.6744999999999));
#34091=CARTESIAN_POINT('Ctrl Pts',(-17.0802404735808,-16.4123522628063,
3.63283333333323));
#34092=CARTESIAN_POINT('Ctrl Pts',(-16.2901202367904,-16.8685283942094,
3.59116666666656));
#34093=CARTESIAN_POINT('Ctrl Pts',(-15.4999999999999,-17.3247045256125,
3.5494999999999));
#34094=CARTESIAN_POINT('Ctrl Pts',(-14.7098797632095,-16.8685283942094,
3.50783333333323));
#34095=CARTESIAN_POINT('Ctrl Pts',(-13.9197595264191,-16.4123522628063,
3.46616666666656));
#34096=CARTESIAN_POINT('Ctrl Pts',(-13.9197595264191,-15.5,3.4244999999999));
#34097=CARTESIAN_POINT('Ctrl Pts',(-13.9197595264191,-14.5876477371938,
3.38283333333323));
#34098=CARTESIAN_POINT('Ctrl Pts',(-14.7098797632095,-14.1314716057907,
3.34116666666656));
#34099=CARTESIAN_POINT('Ctrl Pts',(-15.5,-13.6752954743876,3.29949999999989));
#34100=CARTESIAN_POINT('Ctrl Pts',(-16.2901202367904,-14.1314716057907,
3.25783333333323));
#34101=CARTESIAN_POINT('Ctrl Pts',(-17.0802404735808,-14.5876477371938,
3.21616666666656));
#34102=CARTESIAN_POINT('Ctrl Pts',(-17.0802404735808,-15.5000000000001,
3.17449999999989));
#34103=CARTESIAN_POINT('Ctrl Pts',(-17.0802404735808,-16.4123522628063,
3.13283333333323));
#34104=CARTESIAN_POINT('Ctrl Pts',(-16.2901202367904,-16.8685283942094,
3.09116666666656));
#34105=CARTESIAN_POINT('Ctrl Pts',(-15.4999999999999,-17.3247045256125,
3.04949999999989));
#34106=CARTESIAN_POINT('Ctrl Pts',(-14.7098797632095,-16.8685283942094,
3.00783333333322));
#34107=CARTESIAN_POINT('Ctrl Pts',(-13.9197595264191,-16.4123522628063,
2.96616666666656));
#34108=CARTESIAN_POINT('Ctrl Pts',(-13.9197595264191,-15.5,2.92449999999989));
#34109=CARTESIAN_POINT('Ctrl Pts',(-13.9197595264191,-14.5876477371938,
2.88283333333322));
#34110=CARTESIAN_POINT('Ctrl Pts',(-14.7098797632095,-14.1314716057907,
2.84116666666655));
#34111=CARTESIAN_POINT('Ctrl Pts',(-15.5,-13.6752954743876,2.79949999999989));
#34112=CARTESIAN_POINT('Ctrl Pts',(-16.2901202367904,-14.1314716057907,
2.75783333333322));
#34113=CARTESIAN_POINT('Ctrl Pts',(-17.0802404735808,-14.5876477371938,
2.71616666666655));
#34114=CARTESIAN_POINT('Ctrl Pts',(-17.0802404735808,-15.5000000000001,
2.67449999999989));
#34115=CARTESIAN_POINT('Ctrl Pts',(-17.0802404735808,-16.4123522628063,
2.63283333333322));
#34116=CARTESIAN_POINT('Ctrl Pts',(-16.2901202367904,-16.8685283942094,
2.59116666666655));
#34117=CARTESIAN_POINT('Ctrl Pts',(-15.4999999999999,-17.3247045256125,
2.54949999999988));
#34118=CARTESIAN_POINT('Ctrl Pts',(-14.7098797632095,-16.8685283942094,
2.50783333333322));
#34119=CARTESIAN_POINT('Ctrl Pts',(-13.9197595264191,-16.4123522628063,
2.46616666666655));
#34120=CARTESIAN_POINT('Ctrl Pts',(-13.9197595264191,-15.5,2.42449999999988));
#34121=CARTESIAN_POINT('Ctrl Pts',(-13.9197595264191,-14.5876477371938,
2.38283333333321));
#34122=CARTESIAN_POINT('Ctrl Pts',(-14.7098797632095,-14.1314716057907,
2.34116666666655));
#34123=CARTESIAN_POINT('Ctrl Pts',(-15.5,-13.6752954743876,2.29949999999988));
#34124=CARTESIAN_POINT('Ctrl Pts',(-16.2901202367904,-14.1314716057907,
2.25783333333321));
#34125=CARTESIAN_POINT('Ctrl Pts',(-17.0802404735808,-14.5876477371938,
2.21616666666655));
#34126=CARTESIAN_POINT('Ctrl Pts',(-17.0802404735808,-15.5000000000001,
2.17449999999988));
#34127=CARTESIAN_POINT('Ctrl Pts',(-17.0802404735808,-16.4123522628063,
2.13283333333321));
#34128=CARTESIAN_POINT('Ctrl Pts',(-16.2901202367904,-16.8685283942094,
2.09116666666655));
#34129=CARTESIAN_POINT('Ctrl Pts',(-15.4999999999999,-17.3247045256125,
2.04949999999988));
#34130=CARTESIAN_POINT('Ctrl Pts',(-14.7098797632095,-16.8685283942094,
2.00783333333321));
#34131=CARTESIAN_POINT('Ctrl Pts',(-13.9197595264191,-16.4123522628063,
1.96616666666654));
#34132=CARTESIAN_POINT('Ctrl Pts',(-13.9197595264191,-15.5,1.92449999999988));
#34133=CARTESIAN_POINT('Ctrl Pts',(-13.9197595264191,-14.5876477371938,
1.88283333333321));
#34134=CARTESIAN_POINT('Ctrl Pts',(-14.7098797632095,-14.1314716057907,
1.84116666666654));
#34135=CARTESIAN_POINT('Ctrl Pts',(-15.5,-13.6752954743876,1.79949999999987));
#34136=CARTESIAN_POINT('Ctrl Pts',(-16.2901202367904,-14.1314716057907,
1.75783333333321));
#34137=CARTESIAN_POINT('Ctrl Pts',(-17.0802404735808,-14.5876477371938,
1.71616666666654));
#34138=CARTESIAN_POINT('Ctrl Pts',(-17.0802404735808,-15.5000000000001,
1.67449999999987));
#34139=CARTESIAN_POINT('Ctrl Pts',(-17.0802404735808,-16.4123522628063,
1.63283333333321));
#34140=CARTESIAN_POINT('Ctrl Pts',(-16.2901202367904,-16.8685283942094,
1.59116666666654));
#34141=CARTESIAN_POINT('Ctrl Pts',(-15.4999999999999,-17.3247045256125,
1.54949999999987));
#34142=CARTESIAN_POINT('Ctrl Pts',(-14.7098797632095,-16.8685283942094,
1.5078333333332));
#34143=CARTESIAN_POINT('Ctrl Pts',(-13.9197595264191,-16.4123522628063,
1.46616666666654));
#34144=CARTESIAN_POINT('Ctrl Pts',(-13.9197595264191,-15.5,1.42449999999987));
#34145=CARTESIAN_POINT('Ctrl Pts',(-13.9197595264191,-14.5876477371938,
1.3828333333332));
#34146=CARTESIAN_POINT('Ctrl Pts',(-14.7098797632095,-14.1314716057907,
1.34116666666653));
#34147=CARTESIAN_POINT('Ctrl Pts',(-15.5,-13.6752954743876,1.29949999999987));
#34148=CARTESIAN_POINT('Ctrl Pts',(-16.2901202367904,-14.1314716057907,
1.2578333333332));
#34149=CARTESIAN_POINT('Ctrl Pts',(-17.0802404735808,-14.5876477371938,
1.21616666666653));
#34150=CARTESIAN_POINT('Ctrl Pts',(-17.0802404735808,-15.5000000000001,
1.17449999999986));
#34151=CARTESIAN_POINT('Ctrl Pts',(-17.0802404735808,-16.4123522628063,
1.1328333333332));
#34152=CARTESIAN_POINT('Ctrl Pts',(-16.2901202367904,-16.8685283942094,
1.09116666666653));
#34153=CARTESIAN_POINT('Ctrl Pts',(-15.4999999999999,-17.3247045256125,
1.04949999999986));
#34154=CARTESIAN_POINT('Ctrl Pts',(-14.7098797632095,-16.8685283942094,
1.0078333333332));
#34155=CARTESIAN_POINT('Ctrl Pts',(-13.9197595264191,-16.4123522628063,
0.96616666666653));
#34156=CARTESIAN_POINT('Ctrl Pts',(-13.9197595264191,-15.5,0.924499999999863));
#34157=CARTESIAN_POINT('Ctrl Pts',(-13.9197595264191,-14.5876477371938,
0.882833333333196));
#34158=CARTESIAN_POINT('Ctrl Pts',(-14.7098797632095,-14.1314716057907,
0.841166666666529));
#34159=CARTESIAN_POINT('Ctrl Pts',(-15.5,-13.6752954743876,0.799499999999861));
#34160=CARTESIAN_POINT('Ctrl Pts',(-16.2901202367904,-14.1314716057907,
0.757833333333194));
#34161=CARTESIAN_POINT('Ctrl Pts',(-17.0802404735808,-14.5876477371938,
0.716166666666527));
#34162=CARTESIAN_POINT('Ctrl Pts',(-17.0802404735808,-15.5000000000001,
0.674499999999859));
#34163=CARTESIAN_POINT('Ctrl Pts',(-17.0802404735808,-16.4123522628063,
0.632833333333192));
#34164=CARTESIAN_POINT('Ctrl Pts',(-16.2901202367904,-16.8685283942094,
0.591166666666525));
#34165=CARTESIAN_POINT('Ctrl Pts',(-15.4999999999999,-17.3247045256125,
0.549499999999857));
#34166=CARTESIAN_POINT('Ctrl Pts',(-14.7098797632095,-16.8685283942094,
0.50783333333319));
#34167=CARTESIAN_POINT('Ctrl Pts',(-13.9197595264191,-16.4123522628063,
0.466166666666523));
#34168=CARTESIAN_POINT('Ctrl Pts',(-13.9197595264191,-15.5,0.424499999999856));
#34169=CARTESIAN_POINT('Ctrl Pts',(-13.9197595264191,-14.5876477371938,
0.382833333333188));
#34170=CARTESIAN_POINT('Ctrl Pts',(-14.7098797632095,-14.1314716057907,
0.341166666666521));
#34171=CARTESIAN_POINT('Ctrl Pts',(-15.5,-13.6752954743876,0.299499999999854));
#34172=CARTESIAN_POINT('Ctrl Pts',(-16.2901202367904,-14.1314716057907,
0.257833333333186));
#34173=CARTESIAN_POINT('Ctrl Pts',(-17.0802404735808,-14.5876477371938,
0.216166666666519));
#34174=CARTESIAN_POINT('Ctrl Pts',(-17.0802404735808,-15.5000000000001,
0.174499999999852));
#34175=CARTESIAN_POINT('Ctrl Pts',(-17.0802404735808,-16.4123522628063,
0.132833333333185));
#34176=CARTESIAN_POINT('Ctrl Pts',(-16.2901202367904,-16.8685283942094,
0.0911666666665173));
#34177=CARTESIAN_POINT('Ctrl Pts',(-15.4999999999999,-17.3247045256125,
0.04949999999985));
#34178=CARTESIAN_POINT('Ctrl Pts',(-14.7098797632095,-16.8685283942094,
0.00783333333318273));
#34179=CARTESIAN_POINT('Ctrl Pts',(-13.9197595264191,-16.4123522628063,
-0.0338333333334846));
#34180=CARTESIAN_POINT('Ctrl Pts',(-13.9197595264191,-15.5,-0.0755000000001518));
#34181=CARTESIAN_POINT('Ctrl Pts',(-13.9197595264191,-14.5876477371938,
-0.117166666666817));
#34182=CARTESIAN_POINT('Ctrl Pts',(-14.7098797632095,-14.1314716057907,
-0.158833333333485));
#34183=CARTESIAN_POINT('Ctrl Pts',(-15.5,-13.6752954743876,-0.200500000000152));
#34184=CARTESIAN_POINT('Ctrl Pts',(-16.2901202367904,-14.1314716057907,
-0.242166666666819));
#34185=CARTESIAN_POINT('Ctrl Pts',(-17.0802404735808,-14.5876477371938,
-0.283833333333486));
#34186=CARTESIAN_POINT('Ctrl Pts',(-17.0802404735808,-15.5000000000001,
-0.325500000000154));
#34187=CARTESIAN_POINT('Ctrl Pts',(-17.0802404735808,-16.4123522628063,
-0.367166666666821));
#34188=CARTESIAN_POINT('Ctrl Pts',(-16.2901202367904,-16.8685283942094,
-0.408833333333488));
#34189=CARTESIAN_POINT('Ctrl Pts',(-15.4999999999999,-17.3247045256125,
-0.450500000000156));
#34190=CARTESIAN_POINT('Ctrl Pts',(-14.7098797632095,-16.8685283942094,
-0.492166666666823));
#34191=CARTESIAN_POINT('Ctrl Pts',(-13.9197595264191,-16.4123522628063,
-0.53383333333349));
#34192=CARTESIAN_POINT('Ctrl Pts',(-13.9197595264191,-15.5,-0.575500000000157));
#34193=CARTESIAN_POINT('Ctrl Pts',(-13.9197595264191,-14.5876477371938,
-0.617166666666825));
#34194=CARTESIAN_POINT('Ctrl Pts',(-14.7098797632095,-14.1314716057907,
-0.658833333333492));
#34195=CARTESIAN_POINT('Ctrl Pts',(-15.5,-13.6752954743876,-0.700500000000159));
#34196=CARTESIAN_POINT('Ctrl Pts',(-16.2901202367904,-14.1314716057907,
-0.742166666666827));
#34197=CARTESIAN_POINT('Ctrl Pts',(-17.0802404735808,-14.5876477371938,
-0.783833333333494));
#34198=CARTESIAN_POINT('Ctrl Pts',(-17.0802404735808,-15.5000000000001,
-0.825500000000161));
#34199=CARTESIAN_POINT('Ctrl Pts',(-17.0802404735808,-16.4123522628063,
-0.867166666666829));
#34200=CARTESIAN_POINT('Ctrl Pts',(-16.2901202367904,-16.8685283942094,
-0.908833333333496));
#34201=CARTESIAN_POINT('Ctrl Pts',(-15.4999999999999,-17.3247045256125,
-0.950500000000163));
#34202=CARTESIAN_POINT('Ctrl Pts',(-14.7098797632095,-16.8685283942094,
-0.99216666666683));
#34203=CARTESIAN_POINT('Ctrl Pts',(-13.9197595264191,-16.4123522628063,
-1.0338333333335));
#34204=CARTESIAN_POINT('Ctrl Pts',(-13.9197595264191,-15.5,-1.07550000000016));
#34205=CARTESIAN_POINT('Ctrl Pts',(-13.9197595264191,-14.5876477371938,
-1.11716666666683));
#34206=CARTESIAN_POINT('Ctrl Pts',(-14.7098797632095,-14.1314716057907,
-1.1588333333335));
#34207=CARTESIAN_POINT('Ctrl Pts',(-15.5,-13.6752954743876,-1.20050000000017));
#34208=CARTESIAN_POINT('Ctrl Pts',(-16.2901202367904,-14.1314716057907,
-1.24216666666683));
#34209=CARTESIAN_POINT('Ctrl Pts',(-17.0802404735808,-14.5876477371938,
-1.2838333333335));
#34210=CARTESIAN_POINT('Ctrl Pts',(-17.0802404735808,-15.5000000000001,
-1.32550000000017));
#34211=CARTESIAN_POINT('Ctrl Pts',(-17.0802404735808,-16.4123522628063,
-1.36716666666683));
#34212=CARTESIAN_POINT('Ctrl Pts',(-16.2901202367904,-16.8685283942094,
-1.4088333333335));
#34213=CARTESIAN_POINT('Ctrl Pts',(-15.4999999999999,-17.3247045256125,
-1.45050000000017));
#34214=CARTESIAN_POINT('Ctrl Pts',(-14.7098797632095,-16.8685283942094,
-1.49216666666684));
#34215=CARTESIAN_POINT('Ctrl Pts',(-13.9197595264191,-16.4123522628063,
-1.5338333333335));
#34216=CARTESIAN_POINT('Ctrl Pts',(-13.9197595264191,-15.5,-1.57550000000017));
#34217=CARTESIAN_POINT('Ctrl Pts',(-13.9197595264191,-14.5876477371938,
-1.61716666666684));
#34218=CARTESIAN_POINT('Ctrl Pts',(-14.7098797632095,-14.1314716057907,
-1.65883333333351));
#34219=CARTESIAN_POINT('Ctrl Pts',(-15.5,-13.6752954743876,-1.70050000000017));
#34220=CARTESIAN_POINT('Ctrl Pts',(-16.2901202367904,-14.1314716057907,
-1.74216666666684));
#34221=CARTESIAN_POINT('Ctrl Pts',(-17.0802404735808,-14.5876477371938,
-1.78383333333351));
#34222=CARTESIAN_POINT('Ctrl Pts',(-17.0802404735808,-15.5000000000001,
-1.82550000000017));
#34223=CARTESIAN_POINT('Ctrl Pts',(-17.0802404735808,-16.4123522628063,
-1.86716666666684));
#34224=CARTESIAN_POINT('Ctrl Pts',(-16.2901202367904,-16.8685283942094,
-1.90883333333351));
#34225=CARTESIAN_POINT('Ctrl Pts',(-15.4999999999999,-17.3247045256125,
-1.95050000000018));
#34226=CARTESIAN_POINT('Ctrl Pts',(-14.7098797632095,-16.8685283942094,
-1.99216666666684));
#34227=CARTESIAN_POINT('Ctrl Pts',(-14.4189900731898,-16.7005831533721,
-2.00750661517905));
#34228=CARTESIAN_POINT('Ctrl Pts',(-14.2215586016756,-16.4288420454488,
-2.02512262806106));
#34229=CARTESIAN_POINT('Ctrl Pts',(-13.4352476007234,-15.3465777998746,
-2.09528198318209));
#34230=CARTESIAN_POINT('Ctrl Pts',(-12.6489365997712,-14.2643135543004,
-2.16544133830312));
#34231=CARTESIAN_POINT('Origin',(0.,0.,6.669));
#34232=CARTESIAN_POINT('Origin',(0.,0.,13.019));
#34233=CARTESIAN_POINT('Origin',(-16.96,21.2,10.987));
#34234=CARTESIAN_POINT('',(-21.2,16.96,10.225));
#34235=CARTESIAN_POINT('',(-21.2,16.96,10.987));
#34236=CARTESIAN_POINT('',(-16.96,21.2,10.225));
#34237=CARTESIAN_POINT('',(-16.96,21.2,10.225));
#34238=CARTESIAN_POINT('',(-16.96,21.2,10.987));
#34239=CARTESIAN_POINT('Origin',(-21.2,-16.96,10.987));
#34240=CARTESIAN_POINT('',(-21.2,-16.96,10.225));
#34241=CARTESIAN_POINT('',(-21.2,-16.96,10.987));
#34242=CARTESIAN_POINT('',(-21.2,-16.96,10.225));
#34243=CARTESIAN_POINT('Origin',(-18.5411846327358,18.541184632736,10.225));
#34244=CARTESIAN_POINT('',(-20.438,16.6443692654717,10.987));
#34245=CARTESIAN_POINT('Origin',(-20.4379999999999,16.6443692654717,10.2249999999998));
#34246=CARTESIAN_POINT('',(-16.6443692654717,20.438,10.987));
#34247=CARTESIAN_POINT('',(-18.5411846327358,18.541184632736,10.987));
#34248=CARTESIAN_POINT('Origin',(-16.6443692654718,20.4380000000003,10.2250000000004));
#34249=CARTESIAN_POINT('Origin',(-16.96,21.2,10.987));
#34250=CARTESIAN_POINT('',(16.96,21.2,10.225));
#34251=CARTESIAN_POINT('',(-16.96,21.2,10.225));
#34252=CARTESIAN_POINT('',(16.96,21.2,10.987));
#34253=CARTESIAN_POINT('Origin',(-16.96,-21.2,10.987));
#34254=CARTESIAN_POINT('',(-16.96,-21.2,10.225));
#34255=CARTESIAN_POINT('',(-16.96,-21.2,10.987));
#34256=CARTESIAN_POINT('',(-16.96,-21.2,10.225));
#34257=CARTESIAN_POINT('Origin',(-20.438,-2.09046452842063E-15,10.225));
#34258=CARTESIAN_POINT('',(-20.438,-16.6443692654717,10.987));
#34259=CARTESIAN_POINT('Origin',(-20.4380000000003,-16.6443692654719,10.2250000000003));
#34260=CARTESIAN_POINT('',(-20.438,-2.09046452842063E-15,10.987));
#34261=CARTESIAN_POINT('Origin',(16.96,-21.2,10.987));
#34262=CARTESIAN_POINT('',(16.96,-21.2,10.225));
#34263=CARTESIAN_POINT('',(16.96,-21.2,10.987));
#34264=CARTESIAN_POINT('',(16.96,-21.2,10.225));
#34265=CARTESIAN_POINT('Origin',(-18.5411846327358,-18.541184632736,10.225));
#34266=CARTESIAN_POINT('',(-16.6443692654717,-20.438,10.987));
#34267=CARTESIAN_POINT('Origin',(-16.6443692654716,-20.4379999999998,10.2249999999998));
#34268=CARTESIAN_POINT('',(-18.5411846327358,-18.541184632736,10.987));
#34269=CARTESIAN_POINT('Origin',(16.96,-21.2,10.987));
#34270=CARTESIAN_POINT('',(21.2,-16.96,10.225));
#34271=CARTESIAN_POINT('',(21.2,-16.96,10.987));
#34272=CARTESIAN_POINT('',(16.96,-21.2,10.225));
#34273=CARTESIAN_POINT('Origin',(4.18092905684127E-15,-20.438,10.225));
#34274=CARTESIAN_POINT('',(16.6443692654717,-20.438,10.987));
#34275=CARTESIAN_POINT('Origin',(16.6443692654717,-20.4380000000001,10.2250000000001));
#34276=CARTESIAN_POINT('',(4.18092905684127E-15,-20.438,10.987));
#34277=CARTESIAN_POINT('Origin',(21.2,16.96,10.987));
#34278=CARTESIAN_POINT('',(21.2,16.96,10.225));
#34279=CARTESIAN_POINT('',(21.2,16.96,10.987));
#34280=CARTESIAN_POINT('',(21.2,16.96,10.225));
#34281=CARTESIAN_POINT('Origin',(18.5411846327358,-18.541184632736,10.225));
#34282=CARTESIAN_POINT('',(20.438,-16.6443692654717,10.987));
#34283=CARTESIAN_POINT('Origin',(20.4380000000001,-16.6443692654718,10.2250000000002));
#34284=CARTESIAN_POINT('',(18.5411846327358,-18.541184632736,10.987));
#34285=CARTESIAN_POINT('Origin',(16.96,21.2,10.987));
#34286=CARTESIAN_POINT('',(16.96,21.2,10.225));
#34287=CARTESIAN_POINT('Origin',(20.438,0.,10.225));
#34288=CARTESIAN_POINT('',(20.438,16.6443692654717,10.987));
#34289=CARTESIAN_POINT('Origin',(20.4380000000004,16.6443692654719,10.2250000000004));
#34290=CARTESIAN_POINT('',(20.438,0.,10.987));
#34291=CARTESIAN_POINT('Origin',(18.5411846327358,18.541184632736,10.225));
#34292=CARTESIAN_POINT('',(16.6443692654717,20.438,10.987));
#34293=CARTESIAN_POINT('Origin',(16.6443692654718,20.4380000000003,10.2250000000003));
#34294=CARTESIAN_POINT('',(18.5411846327358,18.541184632736,10.987));
#34295=CARTESIAN_POINT('Origin',(0.,20.438,10.225));
#34296=CARTESIAN_POINT('',(0.,20.438,10.987));
#34297=CARTESIAN_POINT('Origin',(0.,0.,10.987));
#34298=CARTESIAN_POINT('Origin',(0.,0.,37.019));
#34299=CARTESIAN_POINT('',(2.50000000000186,-3.06161699787066E-16,36.5109999999982));
#34300=CARTESIAN_POINT('',(1.99199999999996,-2.43949642390148E-16,37.0190000000001));
#34301=CARTESIAN_POINT('',(1.99200000000004,-2.43949642390158E-16,37.019));
#34302=CARTESIAN_POINT('',(1.51060782468515,1.99199999999999,36.511));
#34303=CARTESIAN_POINT('Origin',(0.,0.,36.511));
#34304=CARTESIAN_POINT('',(0.,1.99200000000004,37.019));
#34305=CARTESIAN_POINT('Ctrl Pts',(2.79900555615041E-16,1.99199999999998,
37.0190000000001));
#34306=CARTESIAN_POINT('Ctrl Pts',(0.669886639976148,1.99199999999998,37.0190000000001));
#34307=CARTESIAN_POINT('Ctrl Pts',(1.51060782468516,1.99199999999998,36.5110000000001));
#34308=CARTESIAN_POINT('Origin',(0.,0.,37.019));
#34309=CARTESIAN_POINT('Origin',(0.,0.,37.019));
#34310=CARTESIAN_POINT('Origin',(0.,0.,37.019));
#34311=CARTESIAN_POINT('',(-1.51060782468517,1.99199999999999,36.511));
#34312=CARTESIAN_POINT('Ctrl Pts',(-1.51060782468828,1.99199999999998,36.5109999999982));
#34313=CARTESIAN_POINT('Ctrl Pts',(-0.669886639977248,1.99199999999998,
37.0190000000001));
#34314=CARTESIAN_POINT('Ctrl Pts',(2.79900555615041E-16,1.99199999999998,
37.0190000000001));
#34315=CARTESIAN_POINT('Origin',(0.,0.,36.511));
#34316=CARTESIAN_POINT('Origin',(0.,0.,37.019));
#34317=CARTESIAN_POINT('',(0.,0.,36.043));
#34318=CARTESIAN_POINT('',(-0.975999999999995,1.19525527596781E-16,37.019));
#34319=CARTESIAN_POINT('',(-0.975999999999995,-1.19525527596781E-16,37.019));
#34320=CARTESIAN_POINT('Origin',(0.,0.,37.019));
#34321=CARTESIAN_POINT('Origin',(0.,0.,37.019));
#34322=CARTESIAN_POINT('',(2.5,-3.06161699786838E-16,-31.939));
#34323=CARTESIAN_POINT('Origin',(0.,0.,-31.939));
#34324=CARTESIAN_POINT('',(2.5,-3.06161699786838E-16,37.019));
#34325=CARTESIAN_POINT('',(-1.51060782468515,1.99199999999999,16.719));
#34326=CARTESIAN_POINT('',(-1.51060782468515,1.99199999999999,37.019));
#34327=CARTESIAN_POINT('',(1.51060782468515,1.99199999999999,16.719));
#34328=CARTESIAN_POINT('Origin',(0.,0.,16.719));
#34329=CARTESIAN_POINT('',(1.51060782468515,1.99199999999999,37.019));
#34330=CARTESIAN_POINT('Origin',(0.,0.,37.019));
#34331=CARTESIAN_POINT('Origin',(0.,0.,-31.939));
#34332=CARTESIAN_POINT('Origin',(-21.2,3.008,16.719));
#34333=CARTESIAN_POINT('',(-21.2,1.99199999999999,16.719));
#34334=CARTESIAN_POINT('Origin',(-21.2,1.99199999999999,37.019));
#34335=CARTESIAN_POINT('Origin',(0.,0.,-32.574));
#34336=CARTESIAN_POINT('',(5.16699999999999,-6.32775001119437E-16,-32.574));
#34337=CARTESIAN_POINT('Origin',(0.,0.,-32.574));
#34338=CARTESIAN_POINT('',(5.16699999999999,-6.32775001119437E-16,-37.019));
#34339=CARTESIAN_POINT('',(5.16699999999999,-6.32775001119436E-16,-32.574));
#34340=CARTESIAN_POINT('Origin',(0.,0.,-37.019));
#34341=CARTESIAN_POINT('Origin',(-15.5,-15.5,-36.765));
#34342=CARTESIAN_POINT('',(-12.325,-15.5,-36.765));
#34343=CARTESIAN_POINT('Origin',(-15.5,-15.5,-36.765));
#34344=CARTESIAN_POINT('',(-12.071,-15.5,-37.019));
#34345=CARTESIAN_POINT('',(-12.325,-15.5,-36.765));
#34346=CARTESIAN_POINT('Origin',(-15.5,-15.5,-37.019));
#34347=CARTESIAN_POINT('Origin',(15.5,-15.5,-36.765));
#34348=CARTESIAN_POINT('',(18.675,-15.5,-36.765));
#34349=CARTESIAN_POINT('Origin',(15.5,-15.5,-36.765));
#34350=CARTESIAN_POINT('',(18.929,-15.5,-37.019));
#34351=CARTESIAN_POINT('',(18.675,-15.5,-36.765));
#34352=CARTESIAN_POINT('Origin',(15.5,-15.5,-37.019));
#34353=CARTESIAN_POINT('Origin',(15.5,15.5,-36.765));
#34354=CARTESIAN_POINT('',(18.675,15.5,-36.765));
#34355=CARTESIAN_POINT('Origin',(15.5,15.5,-36.765));
#34356=CARTESIAN_POINT('',(18.929,15.5,-37.019));
#34357=CARTESIAN_POINT('',(18.675,15.5,-36.765));
#34358=CARTESIAN_POINT('Origin',(15.5,15.5,-37.019));
#34359=CARTESIAN_POINT('Origin',(-15.5,15.5,-36.765));
#34360=CARTESIAN_POINT('',(-12.325,15.5,-36.765));
#34361=CARTESIAN_POINT('Origin',(-15.5,15.5,-36.765));
#34362=CARTESIAN_POINT('',(-12.071,15.5,-37.019));
#34363=CARTESIAN_POINT('',(-12.325,15.5,-36.765));
#34364=CARTESIAN_POINT('Origin',(-15.5,15.5,-37.019));
#34365=CARTESIAN_POINT('Origin',(-15.5,-15.5,-33.844));
#34366=CARTESIAN_POINT('',(-12.325,-15.5,-33.844));
#34367=CARTESIAN_POINT('Origin',(-15.5,-15.5,-33.844));
#34368=CARTESIAN_POINT('',(-12.325,-15.5,-33.844));
#34369=CARTESIAN_POINT('Origin',(15.5,-15.5,-33.844));
#34370=CARTESIAN_POINT('',(18.675,-15.5,-33.844));
#34371=CARTESIAN_POINT('Origin',(15.5,-15.5,-33.844));
#34372=CARTESIAN_POINT('',(18.675,-15.5,-33.844));
#34373=CARTESIAN_POINT('Origin',(15.5,15.5,-33.844));
#34374=CARTESIAN_POINT('',(18.675,15.5,-33.844));
#34375=CARTESIAN_POINT('Origin',(15.5,15.5,-33.844));
#34376=CARTESIAN_POINT('',(18.675,15.5,-33.844));
#34377=CARTESIAN_POINT('Origin',(-15.5,15.5,-33.844));
#34378=CARTESIAN_POINT('',(-12.325,15.5,-33.844));
#34379=CARTESIAN_POINT('Origin',(-15.5,15.5,-33.844));
#34380=CARTESIAN_POINT('',(-12.325,15.5,-33.844));
#34381=CARTESIAN_POINT('Origin',(0.,0.,-37.019));
#34382=CARTESIAN_POINT('',(-2.62699999999999,-3.21714714136009E-16,-32.574));
#34383=CARTESIAN_POINT('Origin',(0.,0.,-32.574));
#34384=CARTESIAN_POINT('',(-2.62699999999999,-3.21714714136009E-16,-27.4178));
#34385=CARTESIAN_POINT('',(-2.62699999999999,-3.21714714136008E-16,-37.019));
#34386=CARTESIAN_POINT('Origin',(0.,0.,-27.4178));
#34387=CARTESIAN_POINT('Origin',(-15.5,15.5,-33.844));
#34388=CARTESIAN_POINT('Origin',(15.5,15.5,-33.844));
#34389=CARTESIAN_POINT('Origin',(15.5,-15.5,-33.844));
#34390=CARTESIAN_POINT('Origin',(-15.5,-15.5,-33.844));
#34391=CARTESIAN_POINT('Origin',(0.,14.342,0.));
#34392=CARTESIAN_POINT('',(-4.445,14.342,-28.9418));
#34393=CARTESIAN_POINT('',(4.445,14.342,-28.9418));
#34394=CARTESIAN_POINT('',(-4.445,14.342,-28.9418));
#34395=CARTESIAN_POINT('',(4.445,14.342,-35.495));
#34396=CARTESIAN_POINT('',(4.445,14.342,-28.9418));
#34397=CARTESIAN_POINT('',(-4.445,14.342,-35.495));
#34398=CARTESIAN_POINT('',(4.445,14.342,-35.495));
#34399=CARTESIAN_POINT('',(-4.445,14.342,-35.495));
#34400=CARTESIAN_POINT('Origin',(4.445,14.342,-35.495));
#34401=CARTESIAN_POINT('',(4.445,21.962,-35.495));
#34402=CARTESIAN_POINT('',(-4.445,21.962,-35.495));
#34403=CARTESIAN_POINT('',(4.445,21.962,-35.495));
#34404=CARTESIAN_POINT('',(-4.445,14.342,-35.495));
#34405=CARTESIAN_POINT('',(4.445,14.342,-35.495));
#34406=CARTESIAN_POINT('Origin',(-4.445,14.342,-35.495));
#34407=CARTESIAN_POINT('',(-4.445,21.962,-28.9418));
#34408=CARTESIAN_POINT('',(-4.445,21.962,-35.495));
#34409=CARTESIAN_POINT('',(-4.445,14.342,-28.9418));
#34410=CARTESIAN_POINT('Origin',(-4.445,14.342,-28.9418));
#34411=CARTESIAN_POINT('',(4.445,21.962,-28.9418));
#34412=CARTESIAN_POINT('',(-4.445,21.962,-28.9418));
#34413=CARTESIAN_POINT('',(4.445,14.342,-28.9418));
#34414=CARTESIAN_POINT('Origin',(4.445,14.342,-28.9418));
#34415=CARTESIAN_POINT('',(4.445,21.962,-28.9418));
#34416=CARTESIAN_POINT('Origin',(0.,21.962,0.));
#34417=CARTESIAN_POINT('',(5.715,21.962,-27.6718));
#34418=CARTESIAN_POINT('',(5.715,21.962,-36.765));
#34419=CARTESIAN_POINT('',(5.715,21.962,-27.6718));
#34420=CARTESIAN_POINT('',(-5.715,21.962,-36.765));
#34421=CARTESIAN_POINT('',(-5.715,21.962,-36.765));
#34422=CARTESIAN_POINT('',(-5.715,21.962,-27.6718));
#34423=CARTESIAN_POINT('',(-5.715,21.962,-27.6718));
#34424=CARTESIAN_POINT('',(-5.715,21.962,-27.6718));
#34425=CARTESIAN_POINT('Origin',(-5.715,21.962,-36.765));
#34426=CARTESIAN_POINT('',(5.715,21.0059612662849,-36.765));
#34427=CARTESIAN_POINT('',(5.715,21.962,-36.765));
#34428=CARTESIAN_POINT('',(-5.715,21.0059612662849,-36.765));
#34429=CARTESIAN_POINT('',(5.715,21.0059612662849,-36.765));
#34430=CARTESIAN_POINT('',(-5.715,21.962,-36.765));
#34431=CARTESIAN_POINT('Origin',(0.,0.,-37.019));
#34432=CARTESIAN_POINT('',(16.6443692654717,-20.438,-37.019));
#34433=CARTESIAN_POINT('',(-16.6443692654717,-20.438,-37.019));
#34434=CARTESIAN_POINT('',(-16.96,-20.438,-37.019));
#34435=CARTESIAN_POINT('',(-20.438,-16.6443692654717,-37.019));
#34436=CARTESIAN_POINT('',(-20.6611846327359,-16.4211846327359,-37.019));
#34437=CARTESIAN_POINT('',(-20.438,16.6443692654717,-37.019));
#34438=CARTESIAN_POINT('',(-20.438,16.96,-37.019));
#34439=CARTESIAN_POINT('',(-16.6443692654717,20.438,-37.019));
#34440=CARTESIAN_POINT('',(-16.4211846327359,20.6611846327359,-37.019));
#34441=CARTESIAN_POINT('',(16.6443692654717,20.438,-37.019));
#34442=CARTESIAN_POINT('',(16.96,20.438,-37.019));
#34443=CARTESIAN_POINT('',(20.438,16.6443692654717,-37.019));
#34444=CARTESIAN_POINT('',(20.6611846327359,16.4211846327359,-37.019));
#34445=CARTESIAN_POINT('',(20.438,-16.6443692654717,-37.019));
#34446=CARTESIAN_POINT('',(20.438,-16.96,-37.019));
#34447=CARTESIAN_POINT('',(16.4211846327359,-20.6611846327358,-37.019));
#34448=CARTESIAN_POINT('Origin',(-16.4211846327359,20.6611846327359,-36.257));
#34449=CARTESIAN_POINT('',(-16.96,21.2,-36.257));
#34450=CARTESIAN_POINT('Origin',(-16.6443692654719,20.4380000000006,-36.2570000000005));
#34451=CARTESIAN_POINT('',(-21.2,16.96,-36.257));
#34452=CARTESIAN_POINT('Origin',(-20.4380000000008,16.6443692654721,-36.2570000000008));
#34453=CARTESIAN_POINT('',(-21.2,16.96,-36.257));
#34454=CARTESIAN_POINT('Origin',(-20.438,-16.96,-36.257));
#34455=CARTESIAN_POINT('',(-21.2,-16.96,-36.257));
#34456=CARTESIAN_POINT('Origin',(-20.4380000000006,-16.644369265472,-36.2570000000005));
#34457=CARTESIAN_POINT('',(-21.2,-16.96,-36.257));
#34458=CARTESIAN_POINT('Origin',(-16.4211846327358,-20.6611846327359,-36.257));
#34459=CARTESIAN_POINT('',(-16.96,-21.2,-36.257));
#34460=CARTESIAN_POINT('Origin',(-16.6443692654721,-20.4380000000011,-36.257000000001));
#34461=CARTESIAN_POINT('',(-16.96,-21.2,-36.257));
#34462=CARTESIAN_POINT('Origin',(-21.2,-16.96,10.987));
#34463=CARTESIAN_POINT('',(-21.2,16.96,-27.4178));
#34464=CARTESIAN_POINT('',(-21.2,16.96,10.987));
#34465=CARTESIAN_POINT('',(-21.2,-16.96,-27.4178));
#34466=CARTESIAN_POINT('',(-21.2,-16.96,10.987));
#34467=CARTESIAN_POINT('',(-21.2,21.2,-27.4178));
#34468=CARTESIAN_POINT('Origin',(16.96,-20.438,-36.257));
#34469=CARTESIAN_POINT('',(16.96,-21.2,-36.257));
#34470=CARTESIAN_POINT('Origin',(16.6443692654718,-20.4380000000002,-36.2570000000002));
#34471=CARTESIAN_POINT('',(16.96,-21.2,-36.257));
#34472=CARTESIAN_POINT('Origin',(-16.96,-21.2,10.987));
#34473=CARTESIAN_POINT('',(-16.96,-21.2,-27.4178));
#34474=CARTESIAN_POINT('',(-16.96,-21.2,10.987));
#34475=CARTESIAN_POINT('',(-16.96,-21.2,-27.4178));
#34476=CARTESIAN_POINT('Origin',(16.4211846327359,-20.6611846327358,-36.257));
#34477=CARTESIAN_POINT('',(21.2,-16.96,-36.257));
#34478=CARTESIAN_POINT('Origin',(20.4380000000003,-16.6443692654718,-36.2570000000003));
#34479=CARTESIAN_POINT('',(21.2,-16.96,-36.257));
#34480=CARTESIAN_POINT('Origin',(16.96,-21.2,10.987));
#34481=CARTESIAN_POINT('',(16.96,-21.2,-27.4178));
#34482=CARTESIAN_POINT('',(16.96,-21.2,10.987));
#34483=CARTESIAN_POINT('',(-21.2,-21.2,-27.4178));
#34484=CARTESIAN_POINT('Origin',(20.438,16.96,-36.257));
#34485=CARTESIAN_POINT('',(21.2,16.96,-36.257));
#34486=CARTESIAN_POINT('Origin',(20.4379999999998,16.6443692654717,-36.2569999999998));
#34487=CARTESIAN_POINT('',(21.2,16.96,-36.257));
#34488=CARTESIAN_POINT('Origin',(16.96,-21.2,10.987));
#34489=CARTESIAN_POINT('',(21.2,-16.96,-27.4178));
#34490=CARTESIAN_POINT('',(21.2,-16.96,10.987));
#34491=CARTESIAN_POINT('',(16.96,-21.2,-27.4178));
#34492=CARTESIAN_POINT('Origin',(16.4211846327359,20.6611846327359,-36.257));
#34493=CARTESIAN_POINT('',(16.96,21.2,-36.257));
#34494=CARTESIAN_POINT('Origin',(16.6443692654716,20.4379999999997,-36.2569999999998));
#34495=CARTESIAN_POINT('',(16.96,21.2,-36.257));
#34496=CARTESIAN_POINT('Origin',(21.2,16.96,10.987));
#34497=CARTESIAN_POINT('',(21.2,16.96,-27.4178));
#34498=CARTESIAN_POINT('',(21.2,16.96,10.987));
#34499=CARTESIAN_POINT('',(21.2,21.2,-27.4178));
#34500=CARTESIAN_POINT('Origin',(-16.96,21.2,10.987));
#34501=CARTESIAN_POINT('',(-16.96,21.2,-27.4178));
#34502=CARTESIAN_POINT('',(-16.96,21.2,10.987));
#34503=CARTESIAN_POINT('',(-16.96,21.2,-27.4178));
#34504=CARTESIAN_POINT('Origin',(-5.715,21.962,-27.6718));
#34505=CARTESIAN_POINT('',(-5.715,21.2,-36.257));
#34506=CARTESIAN_POINT('Origin',(-5.715,20.438,-36.257));
#34507=CARTESIAN_POINT('',(-5.715,21.2,-27.6718));
#34508=CARTESIAN_POINT('',(-5.715,21.2,-27.6718));
#34509=CARTESIAN_POINT('',(-5.715,21.962,-27.6718));
#34510=CARTESIAN_POINT('Origin',(-5.715,21.962,-27.6718));
#34511=CARTESIAN_POINT('',(5.715,21.2,-27.6718));
#34512=CARTESIAN_POINT('',(-5.715,21.2,-27.6718));
#34513=CARTESIAN_POINT('',(5.715,21.962,-27.6718));
#34514=CARTESIAN_POINT('Origin',(5.715,21.962,-27.6718));
#34515=CARTESIAN_POINT('',(5.715,21.2,-36.257));
#34516=CARTESIAN_POINT('',(5.715,21.2,-27.6718));
#34517=CARTESIAN_POINT('Origin',(5.715,20.438,-36.257));
#34518=CARTESIAN_POINT('Origin',(-16.96,20.438,-36.257));
#34519=CARTESIAN_POINT('',(-16.96,21.2,-36.257));
#34520=CARTESIAN_POINT('',(-16.96,21.2,-36.257));
#34521=CARTESIAN_POINT('Origin',(16.96,21.2,10.987));
#34522=CARTESIAN_POINT('',(16.96,21.2,-27.4178));
#34523=CARTESIAN_POINT('',(16.96,21.2,10.987));
#34524=CARTESIAN_POINT('',(16.96,21.2,-27.4178));
#34525=CARTESIAN_POINT('Origin',(-16.96,21.2,10.987));
#34526=CARTESIAN_POINT('',(-21.2,21.2,-27.4178));
#34527=CARTESIAN_POINT('Origin',(-21.2,16.96,-27.4178));
#34528=CARTESIAN_POINT('Origin',(0.,0.,-32.574));
#34529=CARTESIAN_POINT('Origin',(0.,0.,-37.019));
#34530=CARTESIAN_POINT('',(-2.62699999999999,-3.21714714136009E-16,-27.4178));
#34531=CARTESIAN_POINT('Origin',(0.,0.,-27.4178));
#34532=CARTESIAN_POINT('',(-2.62699999999999,-3.21714714136009E-16,1.3858));
#34533=CARTESIAN_POINT('',(-2.62699999999999,-3.21714714136008E-16,-37.019));
#34534=CARTESIAN_POINT('Origin',(0.,0.,1.3858));
#34535=CARTESIAN_POINT('Origin',(15.5,-15.5,-1.713));
#34536=CARTESIAN_POINT('',(13.595,-15.5,-1.713));
#34537=CARTESIAN_POINT('Origin',(15.5,-15.5,-1.713));
#34538=CARTESIAN_POINT('',(13.595,-15.5,1.3858));
#34539=CARTESIAN_POINT('',(13.595,-15.5,-1.713));
#34540=CARTESIAN_POINT('Origin',(15.5,-15.5,1.3858));
#34541=CARTESIAN_POINT('Origin',(-15.5,15.5,-1.713));
#34542=CARTESIAN_POINT('',(-17.405,15.5,-1.713));
#34543=CARTESIAN_POINT('Origin',(-15.5,15.5,-1.713));
#34544=CARTESIAN_POINT('',(-17.405,15.5,1.3858));
#34545=CARTESIAN_POINT('',(-17.405,15.5,-1.713));
#34546=CARTESIAN_POINT('Origin',(-15.5,15.5,1.3858));
#34547=CARTESIAN_POINT('Origin',(15.5,15.5,-1.713));
#34548=CARTESIAN_POINT('',(13.595,15.5,-1.713));
#34549=CARTESIAN_POINT('Origin',(15.5,15.5,-1.713));
#34550=CARTESIAN_POINT('',(13.595,15.5,1.3858));
#34551=CARTESIAN_POINT('',(13.595,15.5,-1.713));
#34552=CARTESIAN_POINT('Origin',(15.5,15.5,1.3858));
#34553=CARTESIAN_POINT('Origin',(-15.5,-15.5,-1.713));
#34554=CARTESIAN_POINT('',(-17.405,-15.5,-1.713));
#34555=CARTESIAN_POINT('Origin',(-15.5,-15.5,-1.713));
#34556=CARTESIAN_POINT('',(-17.405,-15.5,1.3858));
#34557=CARTESIAN_POINT('',(-17.405,-15.5,-1.713));
#34558=CARTESIAN_POINT('Origin',(-15.5,-15.5,1.3858));
#34559=CARTESIAN_POINT('Origin',(-21.2,16.96,-27.4178));
#34560=CARTESIAN_POINT('',(14.5199231636792,20.946,-27.4178));
#34561=CARTESIAN_POINT('',(20.946,14.5199231636793,-27.4178));
#34562=CARTESIAN_POINT('',(15.6129615818396,19.8529615818396,-27.4178));
#34563=CARTESIAN_POINT('',(20.946,-14.5199231636793,-27.4178));
#34564=CARTESIAN_POINT('',(20.946,14.5199231636793,-27.4178));
#34565=CARTESIAN_POINT('',(14.5199231636792,-20.946,-27.4178));
#34566=CARTESIAN_POINT('',(20.946,-14.5199231636793,-27.4178));
#34567=CARTESIAN_POINT('',(-14.5199231636792,-20.946,-27.4178));
#34568=CARTESIAN_POINT('',(-14.5199231636792,-20.946,-27.4178));
#34569=CARTESIAN_POINT('',(-20.946,-14.5199231636793,-27.4178));
#34570=CARTESIAN_POINT('',(-15.6129615818396,-19.8529615818396,-27.4178));
#34571=CARTESIAN_POINT('',(-20.946,14.5199231636793,-27.4178));
#34572=CARTESIAN_POINT('',(-20.946,14.5199231636793,-27.4178));
#34573=CARTESIAN_POINT('',(-14.5199231636792,20.946,-27.4178));
#34574=CARTESIAN_POINT('',(-15.6129615818396,19.8529615818396,-27.4178));
#34575=CARTESIAN_POINT('',(-14.5199231636792,20.946,-27.4178));
#34576=CARTESIAN_POINT('Origin',(16.96,21.2,1.3858));
#34577=CARTESIAN_POINT('',(14.5199231636792,20.946,1.3858));
#34578=CARTESIAN_POINT('',(20.946,14.5199231636793,1.3858));
#34579=CARTESIAN_POINT('',(20.946,14.5199231636793,1.3858));
#34580=CARTESIAN_POINT('',(-14.5199231636792,20.946,1.3858));
#34581=CARTESIAN_POINT('',(-14.5199231636792,20.946,1.3858));
#34582=CARTESIAN_POINT('',(-20.946,14.5199231636793,1.3858));
#34583=CARTESIAN_POINT('',(-15.6129615818396,19.8529615818396,1.3858));
#34584=CARTESIAN_POINT('',(-20.946,-14.5199231636793,1.3858));
#34585=CARTESIAN_POINT('',(-20.946,14.5199231636793,1.3858));
#34586=CARTESIAN_POINT('',(-14.5199231636792,-20.946,1.3858));
#34587=CARTESIAN_POINT('',(-20.946,-14.5199231636793,1.3858));
#34588=CARTESIAN_POINT('',(14.5199231636792,-20.946,1.3858));
#34589=CARTESIAN_POINT('',(-14.5199231636792,-20.946,1.3858));
#34590=CARTESIAN_POINT('',(20.946,-14.5199231636793,1.3858));
#34591=CARTESIAN_POINT('',(15.6129615818396,-19.8529615818396,1.3858));
#34592=CARTESIAN_POINT('',(20.946,14.5199231636793,1.3858));
#34593=CARTESIAN_POINT('Origin',(-14.5199231636792,20.946,-27.4178));
#34594=CARTESIAN_POINT('',(14.5199231636792,20.946,-27.4178));
#34595=CARTESIAN_POINT('',(-14.5199231636792,20.946,-27.4178));
#34596=CARTESIAN_POINT('Origin',(20.946,14.5199231636793,-27.4178));
#34597=CARTESIAN_POINT('',(20.946,14.5199231636793,-27.4178));
#34598=CARTESIAN_POINT('Origin',(-15.6129615818396,19.8529615818396,-27.4178));
#34599=CARTESIAN_POINT('',(-20.946,14.5199231636793,-27.4178));
#34600=CARTESIAN_POINT('Origin',(15.6129615818396,-19.8529615818396,-27.4178));
#34601=CARTESIAN_POINT('',(14.5199231636792,-20.946,-27.4178));
#34602=CARTESIAN_POINT('',(20.946,-14.5199231636793,-27.4178));
#34603=CARTESIAN_POINT('Origin',(-20.946,-14.5199231636793,-27.4178));
#34604=CARTESIAN_POINT('',(-20.946,-14.5199231636793,-27.4178));
#34605=CARTESIAN_POINT('',(-14.5199231636792,-20.946,-27.4178));
#34606=CARTESIAN_POINT('Origin',(-20.946,14.5199231636793,-27.4178));
#34607=CARTESIAN_POINT('Origin',(-14.5199231636792,-20.946,-27.4178));
#34608=CARTESIAN_POINT('Origin',(20.946,14.5199231636793,-27.4178));
#34609=CARTESIAN_POINT('Origin',(15.5,-15.5,-1.713));
#34610=CARTESIAN_POINT('Origin',(-15.5,15.5,-1.713));
#34611=CARTESIAN_POINT('Origin',(15.5,15.5,-1.713));
#34612=CARTESIAN_POINT('Origin',(-15.5,-15.5,-1.713));
#36430=UNCERTAINTY_MEASURE_WITH_UNIT(LENGTH_MEASURE(0.01),#36461,
'DISTANCE_ACCURACY_VALUE',
'Maximum model space distance between geometric entities at asserted c
onnectivities');
#36444=UNCERTAINTY_MEASURE_WITH_UNIT(LENGTH_MEASURE(0.01),#36461,
'DISTANCE_ACCURACY_VALUE',
'Maximum model space distance between geometric entities at asserted c
onnectivities');
#36446=(
GEOMETRIC_REPRESENTATION_CONTEXT(3)
GLOBAL_UNCERTAINTY_ASSIGNED_CONTEXT((#36430))
GLOBAL_UNIT_ASSIGNED_CONTEXT((#36461,#36463,#36464))
REPRESENTATION_CONTEXT('','3D')
);
#36460=(
GEOMETRIC_REPRESENTATION_CONTEXT(3)
GLOBAL_UNCERTAINTY_ASSIGNED_CONTEXT((#36444))
GLOBAL_UNIT_ASSIGNED_CONTEXT((#36461,#36463,#36464))
REPRESENTATION_CONTEXT('','3D')
);
#36461=(
LENGTH_UNIT()
NAMED_UNIT(*)
SI_UNIT(.MILLI.,.METRE.)
);
#36463=(
NAMED_UNIT(*)
PLANE_ANGLE_UNIT()
SI_UNIT($,.RADIAN.)
);
#36464=(
NAMED_UNIT(*)
SI_UNIT($,.STERADIAN.)
SOLID_ANGLE_UNIT()
);
#36466=SHAPE_DEFINITION_REPRESENTATION(#36481,#36517);
#36481=PRODUCT_DEFINITION_SHAPE('',$,#36533);
#36517=SHAPE_REPRESENTATION('',(#11439),#36446);
#36531=PRODUCT_DEFINITION_CONTEXT('part definition',#36578,'design');
#36533=PRODUCT_DEFINITION('Reference_design_envelope_Motor',
'Reference_design_envelope_Motor',#36548,#36531);
#36548=PRODUCT_DEFINITION_FORMATION('',$,#36581);
#36578=APPLICATION_CONTEXT(
'Core Data for Automotive Mechanical Design Process');
#36579=PRODUCT_CONTEXT('part definition',#36578,'mechanical');
#36581=PRODUCT('Reference_design_envelope_Motor',
'Reference_design_envelope_Motor',$,(#36579));
#36596=PRESENTATION_STYLE_ASSIGNMENT((#36601));
#36601=SURFACE_STYLE_USAGE(.BOTH.,#36606);
#36606=SURFACE_SIDE_STYLE('',(#36611));
#36611=SURFACE_STYLE_FILL_AREA(#36616);
#36616=FILL_AREA_STYLE('Opaque(160,160,160)',(#36621));
#36621=FILL_AREA_STYLE_COLOUR('Opaque(160,160,160)',#36626);
#36626=COLOUR_RGB('Opaque(160,160,160)', 0.09019608, 0.27058824, 0.51372549);
ENDSEC;
END-ISO-10303-21;
